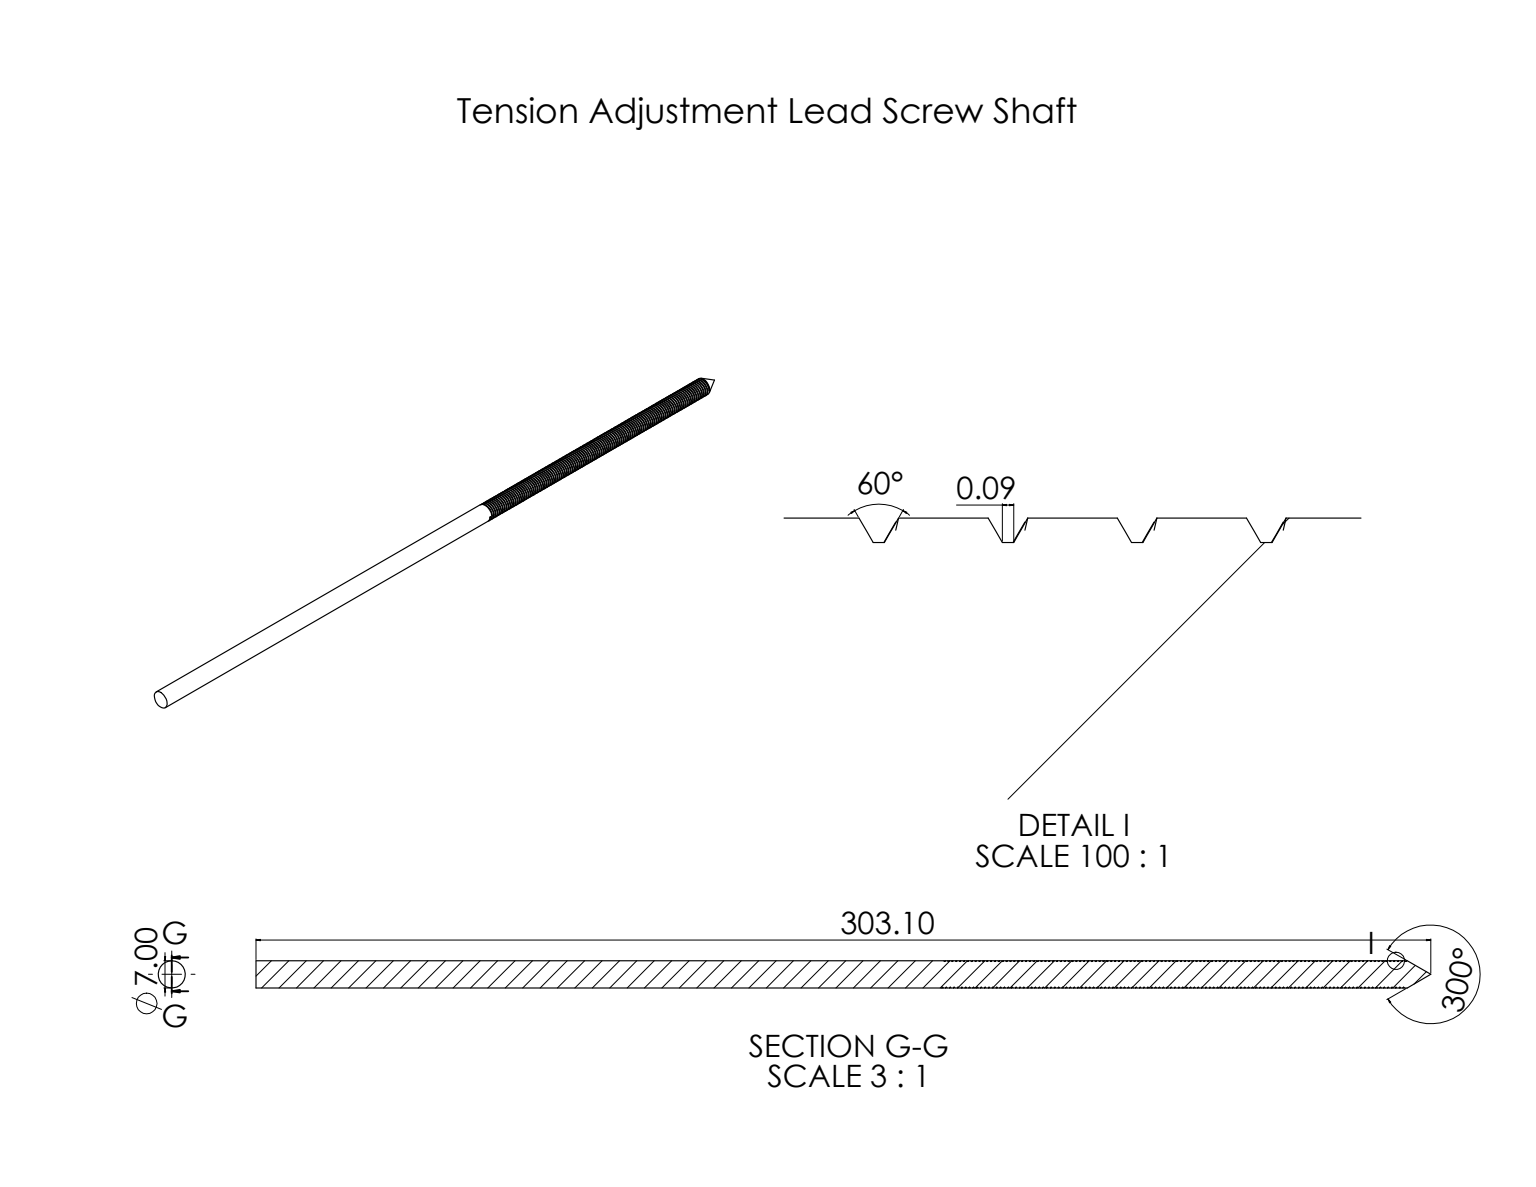
ISO-10303-21;
HEADER;
FILE_DESCRIPTION (('STEP AP214'),
    '1' );
FILE_NAME ('Tension Adjustment Lead Screw Shaft.step',
    '2026-10-25T21:42:00',
    ( '' ),
    ( '' ),
    'SwSTEP 2.0',
    'SolidWorks 2025',
    '' );
FILE_SCHEMA (( 'AUTOMOTIVE_DESIGN' ));
ENDSEC;

DATA;
#4=CARTESIAN_POINT ( 'NONE',  ( 1.655278471874998436, 14.63297358603754539, -90.43077246956613635 ) ) ;
#5=ORIENTED_EDGE ( 'NONE', *, *, #18600, .F. ) ;
#7=EDGE_LOOP ( 'NONE', ( #23173, #23553, #33553, #33564 ) ) ;
#9=CARTESIAN_POINT ( 'NONE',  ( -1.394453263437886604E-15, 14.00000000000001776, -84.40473080337743284 ) ) ;
#12=( BOUNDED_CURVE ( )  B_SPLINE_CURVE ( 2, ( #12979, #41701, #6799, #32739, #418, #13394, #26374, #31903, #3401 ),
 .UNSPECIFIED., .F., .F. ) 
 B_SPLINE_CURVE_WITH_KNOTS ( ( 3, 2, 2, 2, 3 ),
 ( 0.5229166666666666963, 0.5236111111111111382, 0.5250000000000000222, 0.5263888888888889062, 0.5270833333333333481 ),
 .UNSPECIFIED. ) 
 CURVE ( )  GEOMETRIC_REPRESENTATION_ITEM ( )  RATIONAL_B_SPLINE_CURVE ( ( 0.9330127018922194093, 0.9330127018922194093, 1.000000000000000000, 0.8660254037844387076, 1.000000000000000000, 0.8660254037844387076, 1.000000000000000000, 0.9330127018922194093, 0.9330127018922194093 ) ) 
 REPRESENTATION_ITEM ( '' )  );
#13=CARTESIAN_POINT ( 'NONE',  ( -0.9378221735089310451, 14.00000000000002309, -127.4493890021159359 ) ) ;
#14=CARTESIAN_POINT ( 'NONE',  ( 1.749999999999998224, 14.46891108675448656, -129.6276474690881741 ) ) ;
#15=CARTESIAN_POINT ( 'NONE',  ( -1.655278471874999990, 20.36702641396249902, -133.9307724695661364 ) ) ;
#17=CARTESIAN_POINT ( 'NONE',  ( 0.9378221735089302680, 14.00000000000002132, -139.3600726046389013 ) ) ;
#18=CARTESIAN_POINT ( 'NONE',  ( -3.310556943750002645, 15.58864905735837780, -117.7682724695661420 ) ) ;
#19=CARTESIAN_POINT ( 'NONE',  ( 3.310556943749999981, 15.58864905735836182, -51.43493913623279923 ) ) ;
#21=CARTESIAN_POINT ( 'NONE',  ( -3.500000000000000888, 19.52072594216371826, -128.7380641367107614 ) ) ;
#22=VECTOR ( 'NONE', #20923, 1000.000000000000000 ) ;
#23=CARTESIAN_POINT ( 'NONE',  ( 3.310556943750001313, 17.50000000000001421, -72.35160580289947063 ) ) ;
#24=CARTESIAN_POINT ( 'NONE',  ( 2.474675557024783212E-16, 21.54145188432740099, -122.2109808024215170 ) ) ;
#25=CARTESIAN_POINT ( 'NONE',  ( -1.655278471875002211, 14.63297358603754894, -108.5974391362328078 ) ) ;
#26=CARTESIAN_POINT ( 'NONE',  ( 1.750000000000001110, 20.53108891324555429, -92.98806413671076143 ) ) ;
#29=CARTESIAN_POINT ( 'NONE',  ( 3.500000000000001776, 19.52072594216371115, -75.37764746908818836 ) ) ;
#31=CARTESIAN_POINT ( 'NONE',  ( 3.310556943749999981, 15.58864905735836182, -44.34743913623280065 ) ) ;
#33=CARTESIAN_POINT ( 'NONE',  ( 1.655278471874998436, 14.63297358603754716, -97.51827246956612782 ) ) ;
#34=CARTESIAN_POINT ( 'NONE',  ( 0.9378221735089300459, 21.00000000000001421, -67.94938900211596433 ) ) ;
#35=CARTESIAN_POINT ( 'NONE',  ( 1.749999999999998224, 14.46891108675447768, -62.32139747004410424 ) ) ;
#38=CARTESIAN_POINT ( 'NONE',  ( 3.310556943750001313, 19.41135094264166838, -117.2682724695661278 ) ) ;
#44=CARTESIAN_POINT ( 'NONE',  ( 3.310556943750001313, 17.50000000000001776, -99.26410580289947916 ) ) ;
#45=CARTESIAN_POINT ( 'NONE',  ( 4.648177544792955347E-16, 21.00000000000001421, -63.21098080242150274 ) ) ;
#47=ORIENTED_EDGE ( 'NONE', *, *, #33783, .T. ) ;
#48=CARTESIAN_POINT ( 'NONE',  ( -7.460324959392693302E-14, 21.00000000000001776, -87.90473080337741862 ) ) ;
#49=CARTESIAN_POINT ( 'NONE',  ( -3.500000000000001332, 17.50000000000002132, -126.9609808024215170 ) ) ;
#50=DIRECTION ( 'NONE',  ( -0.000000000000000000, 1.259100132267607459E-16, -1.000000000000000000 ) ) ;
#53=CARTESIAN_POINT ( 'NONE',  ( 1.655278471875001101, 20.36702641396248481, -33.09743913623280775 ) ) ;
#54=CARTESIAN_POINT ( 'NONE',  ( -0.9378221735089310451, 14.00000000000002309, -109.4493890021159359 ) ) ;
#60=LINE ( 'NONE', #6452, #31415 ) ;
#61=( BOUNDED_CURVE ( )  B_SPLINE_CURVE ( 2, ( #20657, #17472, #30432, #1301, #10233, #7041, #1713, #24475, #37444 ),
 .UNSPECIFIED., .F., .T. ) 
 B_SPLINE_CURVE_WITH_KNOTS ( ( 3, 2, 2, 2, 3 ),
 ( 0.8270833333333332815, 0.8277777777777777235, 0.8291666666666667185, 0.8305555555555556024, 0.8312500000000000444 ),
 .UNSPECIFIED. ) 
 CURVE ( )  GEOMETRIC_REPRESENTATION_ITEM ( )  RATIONAL_B_SPLINE_CURVE ( ( 0.9330127018922194093, 0.9330127018922194093, 1.000000000000000000, 0.8660254037844387076, 1.000000000000000000, 0.8660254037844387076, 1.000000000000000000, 0.9330127018922194093, 0.9330127018922194093 ) ) 
 REPRESENTATION_ITEM ( '' )  );
#63=CARTESIAN_POINT ( 'NONE',  ( 4.648177544792955347E-16, 21.00000000000002132, -115.2109808024215027 ) ) ;
#64=CARTESIAN_POINT ( 'NONE',  ( 3.500000000000001332, 17.50000000000002487, -140.4609808024215170 ) ) ;
#65=CARTESIAN_POINT ( 'NONE',  ( -7.424026671074350129E-16, 13.45854811567263987, -118.4047308033774328 ) ) ;
#67=CARTESIAN_POINT ( 'NONE',  ( -1.655278471875002211, 14.63297358603755249, -134.6849391362327992 ) ) ;
#68=CARTESIAN_POINT ( 'NONE',  ( -3.500000000000000888, 19.52072594216370405, -34.04431413575484555 ) ) ;
#71=CARTESIAN_POINT ( 'NONE',  ( -1.394453263437886604E-15, 14.00000000000001421, -65.40473080337743284 ) ) ;
#73=CARTESIAN_POINT ( 'NONE',  ( -3.500000000000000888, 19.52072594216372181, -138.0443141357548598 ) ) ;
#74=CARTESIAN_POINT ( 'NONE',  ( 1.655278471874998436, 14.63297358603755072, -123.4307724695661506 ) ) ;
#77=CARTESIAN_POINT ( 'NONE',  ( -1.394453263437886604E-15, 14.00000000000001066, -46.40473080337741862 ) ) ;
#78=CARTESIAN_POINT ( 'NONE',  ( 1.749999999999998224, 14.46891108675448123, -92.62764746908815994 ) ) ;
#79=CARTESIAN_POINT ( 'NONE',  ( -3.500000000000001332, 17.50000000000001066, -45.65473080337742573 ) ) ;
#80=CARTESIAN_POINT ( 'NONE',  ( 3.310556943750001313, 17.50000000000001421, -58.26410580289947916 ) ) ;
#81=CARTESIAN_POINT ( 'NONE',  ( 1.655278471874998436, 14.63297358603754894, -119.5182724695661278 ) ) ;
#83=CARTESIAN_POINT ( 'NONE',  ( -3.500000000000002220, 15.47927405783632082, -30.57139747004410069 ) ) ;
#86=CARTESIAN_POINT ( 'NONE',  ( -7.022189441860112050E-16, 13.67729811471672896, -132.6016058028994564 ) ) ;
#90=CARTESIAN_POINT ( 'NONE',  ( -7.022189441860112050E-16, 13.67729811471672186, -70.60160580289947063 ) ) ;
#92=CARTESIAN_POINT ( 'NONE',  ( 3.310556943750001313, 17.50000000000001421, -65.26410580289946495 ) ) ;
#93=ORIENTED_EDGE ( 'NONE', *, *, #26909, .T. ) ;
#95=CARTESIAN_POINT ( 'NONE',  ( -1.655278471875002211, 14.63297358603754716, -83.68493913623278502 ) ) ;
#97=CARTESIAN_POINT ( 'NONE',  ( -1.394453263437886604E-15, 14.00000000000001066, -36.40473080337743284 ) ) ;
#99=CARTESIAN_POINT ( 'NONE',  ( -1.655278471874999990, 20.36702641396248836, -47.93077246956614346 ) ) ;
#100=EDGE_CURVE ( 'NONE', #30193, #39728, #5168, .T. ) ;
#102=CARTESIAN_POINT ( 'NONE',  ( 2.340729813953370519E-16, 21.32270188528331900, -105.0141058028994649 ) ) ;
#103=CARTESIAN_POINT ( 'NONE',  ( -3.500000000000000000, 19.52072594216370405, -36.04431413575484555 ) ) ;
#104=VERTEX_POINT ( 'NONE', #20780 ) ;
#109=CARTESIAN_POINT ( 'NONE',  ( 2.340729813953370519E-16, 21.32270188528330834, -56.01410580289947916 ) ) ;
#110=ORIENTED_EDGE ( 'NONE', *, *, #41716, .T. ) ;
#111=ORIENTED_EDGE ( 'NONE', *, *, #16123, .F. ) ;
#113=CARTESIAN_POINT ( 'NONE',  ( 4.648177544792955347E-16, 21.00000000000001421, -55.21098080242150274 ) ) ;
#116=CARTESIAN_POINT ( 'NONE',  ( -1.750000000000002220, 14.46891108675449011, -138.7943141357548313 ) ) ;
#117=CARTESIAN_POINT ( 'NONE',  ( -3.310556943750002201, 15.58864905735837780, -126.6807724695661364 ) ) ;
#118=EDGE_CURVE ( 'NONE', #7389, #10255, #33314, .T. ) ;
#120=VECTOR ( 'NONE', #13547, 1000.000000000000000 ) ;
#121=EDGE_CURVE ( 'NONE', #3869, #17551, #1003, .T. ) ;
#123=CARTESIAN_POINT ( 'NONE',  ( -3.310556943750002645, 15.58864905735836537, -33.76827246956613493 ) ) ;
#124=CARTESIAN_POINT ( 'NONE',  ( 1.655278471874998436, 14.63297358603753651, -25.51827246956613138 ) ) ;
#125=CARTESIAN_POINT ( 'NONE',  ( 3.310556943750001313, 19.41135094264166483, -85.26827246956612782 ) ) ;
#126=CARTESIAN_POINT ( 'NONE',  ( -3.310556943750000425, 19.41135094264167549, -139.8474391362327935 ) ) ;
#128=CARTESIAN_POINT ( 'NONE',  ( 3.405278471875001323, 17.50000000000001066, -23.20941830313845600 ) ) ;
#129=CARTESIAN_POINT ( 'NONE',  ( -1.394453263437886604E-15, 14.00000000000001421, -66.71098080242148853 ) ) ;
#130=CARTESIAN_POINT ( 'NONE',  ( -3.310556943750000425, 19.41135094264167549, -134.9349391362328277 ) ) ;
#131=CARTESIAN_POINT ( 'NONE',  ( 3.500000000000000000, 15.47927405783632437, -56.54431413575483845 ) ) ;
#132=CARTESIAN_POINT ( 'NONE',  ( 2.340729813953370519E-16, 21.32270188528331190, -94.01410580289947916 ) ) ;
#134=CARTESIAN_POINT ( 'NONE',  ( -0.9378221735089291577, 21.00000000000001776, -93.16632260368298546 ) ) ;
#135=CARTESIAN_POINT ( 'NONE',  ( 3.500000000000001776, 19.52072594216371115, -76.07139747004410424 ) ) ;
#136=AXIS2_PLACEMENT_3D ( 'NONE', #21819, #34790, #18632 ) ;
#137=CARTESIAN_POINT ( 'NONE',  ( -1.655278471874999990, 20.36702641396248836, -59.01827246956613493 ) ) ;
#141=AXIS2_PLACEMENT_3D ( 'NONE', #11011, #30148, #20585 ) ;
#142=CARTESIAN_POINT ( 'NONE',  ( 2.340729813953370519E-16, 21.32270188528331190, -84.10160580289945642 ) ) ;
#144=CARTESIAN_POINT ( 'NONE',  ( -1.655278471875002211, 14.63297358603755072, -115.5974391362327935 ) ) ;
#145=CARTESIAN_POINT ( 'NONE',  ( 2.340729813953370519E-16, 21.32270188528331190, -82.01410580289947916 ) ) ;
#146=CARTESIAN_POINT ( 'NONE',  ( -0.9378221735089291577, 21.00000000000001776, -96.86007260463890134 ) ) ;
#148=CARTESIAN_POINT ( 'NONE',  ( 2.340729813953370519E-16, 21.32270188528331190, -100.1016058028994706 ) ) ;
#149=CARTESIAN_POINT ( 'NONE',  ( -3.500000000000000888, 19.52072594216371826, -103.7380641367107614 ) ) ;
#152=CARTESIAN_POINT ( 'NONE',  ( 1.750000000000001110, 20.53108891324554719, -43.98806413671076143 ) ) ;
#153=CARTESIAN_POINT ( 'NONE',  ( 3.500000000000000000, 15.47927405783632082, -45.54431413575483845 ) ) ;
#155=CARTESIAN_POINT ( 'NONE',  ( 3.310556943750001313, 19.41135094264166483, -67.18077246956613635 ) ) ;
#156=ADVANCED_FACE ( 'NONE', ( #4604 ), #8574, .T. ) ;
#158=CARTESIAN_POINT ( 'NONE',  ( -3.310556943750000425, 19.41135094264166838, -119.8474391362328078 ) ) ;
#163=CARTESIAN_POINT ( 'NONE',  ( -3.500000000000001332, 17.50000000000001066, -42.96098080242151696 ) ) ;
#165=CARTESIAN_POINT ( 'NONE',  ( -7.022189441860112050E-16, 13.67729811471672186, -73.51410580289947916 ) ) ;
#166=EDGE_LOOP ( 'NONE', ( #29980, #17944, #31136, #21561 ) ) ;
#167=VERTEX_POINT ( 'NONE', #37923 ) ;
#173=CARTESIAN_POINT ( 'NONE',  ( -3.310556943750000425, 19.41135094264165772, -41.93493913623279212 ) ) ;
#174=CARTESIAN_POINT ( 'NONE',  ( 1.655278471875001101, 20.36702641396249547, -106.1849391362327992 ) ) ;
#176=ADVANCED_FACE ( 'NONE', ( #8782 ), #21755, .T. ) ;
#177=( BOUNDED_CURVE ( )  B_SPLINE_CURVE ( 2, ( #32647, #3511, #29666, #26491, #530, #13503, #39446, #10320, #20103 ),
 .UNSPECIFIED., .F., .T. ) 
 B_SPLINE_CURVE_WITH_KNOTS ( ( 3, 2, 2, 2, 3 ),
 ( 0.9312500000000000222, 0.9319444444444444642, 0.9333333333333333481, 0.9347222222222222321, 0.9354166666666666741 ),
 .UNSPECIFIED. ) 
 CURVE ( )  GEOMETRIC_REPRESENTATION_ITEM ( )  RATIONAL_B_SPLINE_CURVE ( ( 0.9330127018922194093, 0.9330127018922194093, 1.000000000000000000, 0.8660254037844387076, 1.000000000000000000, 0.8660254037844387076, 1.000000000000000000, 0.9330127018922194093, 0.9330127018922194093 ) ) 
 REPRESENTATION_ITEM ( '' )  );
#178=CARTESIAN_POINT ( 'NONE',  ( 1.655278471874998436, 14.63297358603753828, -27.43077246956614346 ) ) ;
#180=CARTESIAN_POINT ( 'NONE',  ( 1.750000000000001110, 20.53108891324555785, -104.2943141357548456 ) ) ;
#182=EDGE_CURVE ( 'NONE', #24979, #8593, #36724, .T. ) ;
#183=DIRECTION ( 'NONE',  ( -0.000000000000000000, 1.259100132267607459E-16, -1.000000000000000000 ) ) ;
#184=CARTESIAN_POINT ( 'NONE',  ( 3.500000000000001332, 17.50000000000001776, -91.15473080337743284 ) ) ;
#185=CARTESIAN_POINT ( 'NONE',  ( -3.500000000000001332, 17.50000000000001776, -77.96098080242150274 ) ) ;
#188=CARTESIAN_POINT ( 'NONE',  ( 1.749999999999998224, 14.46891108675447768, -59.62764746908817415 ) ) ;
#191=CARTESIAN_POINT ( 'NONE',  ( -3.500000000000000888, 19.52072594216370760, -46.73806413671076143 ) ) ;
#192=CARTESIAN_POINT ( 'NONE',  ( 1.655278471874998436, 14.63297358603753828, -29.51827246956613493 ) ) ;
#194=CARTESIAN_POINT ( 'NONE',  ( -1.394453263437886604E-15, 14.00000000000001421, -80.40473080337743284 ) ) ;
#197=DIRECTION ( 'NONE',  ( -0.000000000000000000, 1.259100132267607459E-16, -1.000000000000000000 ) ) ;
#199=CARTESIAN_POINT ( 'NONE',  ( -1.655278471874999990, 20.36702641396249192, -82.93077246956615056 ) ) ;
#201=CARTESIAN_POINT ( 'NONE',  ( 4.648177544792955347E-16, 21.00000000000001421, -52.21098080242150985 ) ) ;
#203=CARTESIAN_POINT ( 'NONE',  ( 0.9378221735089300459, 21.00000000000001066, -33.94938900211595012 ) ) ;
#205=CARTESIAN_POINT ( 'NONE',  ( 3.500000000000000000, 15.47927405783632793, -87.54431413575483134 ) ) ;
#208=CARTESIAN_POINT ( 'NONE',  ( 2.340729813953370519E-16, 21.32270188528331190, -89.01410580289947916 ) ) ;
#210=ORIENTED_EDGE ( 'NONE', *, *, #4786, .F. ) ;
#215=FACE_OUTER_BOUND ( 'NONE', #16259, .T. ) ;
#216=CARTESIAN_POINT ( 'NONE',  ( 1.655278471875001101, 20.36702641396249902, -134.0974391362328220 ) ) ;
#217=VERTEX_POINT ( 'NONE', #6222 ) ;
#218=AXIS2_PLACEMENT_3D ( 'NONE', #34519, #2189, #33537 ) ;
#220=VECTOR ( 'NONE', #24131, 1000.000000000000000 ) ;
#222=CARTESIAN_POINT ( 'NONE',  ( -1.655278471875002211, 14.63297358603755072, -118.6849391362327992 ) ) ;
#226=CARTESIAN_POINT ( 'NONE',  ( -3.500000000000002220, 15.47927405783633503, -129.5713974700440758 ) ) ;
#227=CARTESIAN_POINT ( 'NONE',  ( -7.022189441860112050E-16, 13.67729811471672186, -73.60160580289945642 ) ) ;
#228=CARTESIAN_POINT ( 'NONE',  ( -7.424026671074350129E-16, 13.45854811567263987, -120.7109808024215170 ) ) ;
#230=CARTESIAN_POINT ( 'NONE',  ( -7.022189441860112050E-16, 13.67729811471672541, -103.5141058028994649 ) ) ;
#232=CARTESIAN_POINT ( 'NONE',  ( -1.394453263437886604E-15, 14.00000000000001066, -31.71098080242150985 ) ) ;
#234=CARTESIAN_POINT ( 'NONE',  ( 3.500000000000000000, 15.47927405783632437, -75.54431413575484555 ) ) ;
#236=CARTESIAN_POINT ( 'NONE',  ( -7.022189441860112050E-16, 13.67729811471671475, -37.51410580289947205 ) ) ;
#237=CARTESIAN_POINT ( 'NONE',  ( 1.655278471874998436, 14.63297358603754716, -95.51827246956612782 ) ) ;
#238=CARTESIAN_POINT ( 'NONE',  ( -3.500000000000001332, 17.50000000000001421, -66.65473080337743284 ) ) ;
#240=CARTESIAN_POINT ( 'NONE',  ( -1.655278471875002211, 14.63297358603755072, -117.6849391362327850 ) ) ;
#247=CARTESIAN_POINT ( 'NONE',  ( -3.310556943750002201, 15.58864905735837425, -96.68077246956613635 ) ) ;
#250=ORIENTED_EDGE ( 'NONE', *, *, #32801, .F. ) ;
#252=CYLINDRICAL_SURFACE ( 'NONE', #19666, 3.499999999999999556 ) ;
#254=CARTESIAN_POINT ( 'NONE',  ( 4.648177544792955347E-16, 21.00000000000002132, -105.9047308033774186 ) ) ;
#259=CARTESIAN_POINT ( 'NONE',  ( -7.022189441860112050E-16, 13.67729811471671653, -26.51410580289948626 ) ) ;
#260=( BOUNDED_CURVE ( )  B_SPLINE_CURVE ( 2, ( #24634, #5264, #21631, #34609, #15269, #28228, #15689, #5055, #28645 ),
 .UNSPECIFIED., .F., .F. ) 
 B_SPLINE_CURVE_WITH_KNOTS ( ( 3, 2, 2, 2, 3 ),
 ( 0.05625000000000000139, 0.05694444444444444337, 0.05833333333333333426, 0.05972222222222222515, 0.06041666666666666713 ),
 .UNSPECIFIED. ) 
 CURVE ( )  GEOMETRIC_REPRESENTATION_ITEM ( )  RATIONAL_B_SPLINE_CURVE ( ( 0.9330127018922192983, 0.9330127018922196314, 1.000000000000000000, 0.8660254037844387076, 1.000000000000000000, 0.8660254037844387076, 1.000000000000000000, 0.9330127018922194093, 0.9330127018922194093 ) ) 
 REPRESENTATION_ITEM ( '' )  );
#263=VECTOR ( 'NONE', #2709, 1000.000000000000000 ) ;
#266=CARTESIAN_POINT ( 'NONE',  ( 4.648177544792955347E-16, 21.00000000000001421, -57.90473080337742573 ) ) ;
#267=ORIENTED_EDGE ( 'NONE', *, *, #5048, .F. ) ;
#270=CARTESIAN_POINT ( 'NONE',  ( -1.394453263437886604E-15, 14.00000000000001066, -31.40473080337742573 ) ) ;
#271=CARTESIAN_POINT ( 'NONE',  ( -3.500000000000002220, 15.47927405783633503, -118.5713974700441184 ) ) ;
#272=DIRECTION ( 'NONE',  ( 0.000000000000000000, 1.000000000000000000, 0.000000000000000000 ) ) ;
#273=CARTESIAN_POINT ( 'NONE',  ( 3.310556943750001313, 19.41135094264167549, -134.2682724695661420 ) ) ;
#274=CARTESIAN_POINT ( 'NONE',  ( -3.500000000000001332, 17.50000000000001066, -26.96098080242151340 ) ) ;
#276=DIRECTION ( 'NONE',  ( -0.000000000000000000, 1.259100132267607459E-16, -1.000000000000000000 ) ) ;
#278=CARTESIAN_POINT ( 'NONE',  ( -2.324088772396477673E-16, 14.00000000000002309, -142.7109808024215170 ) ) ;
#280=CARTESIAN_POINT ( 'NONE',  ( 3.500000000000001776, 19.52072594216372181, -140.3776474690881741 ) ) ;
#281=CARTESIAN_POINT ( 'NONE',  ( -1.655278471874999990, 20.36702641396249547, -117.9307724695661364 ) ) ;
#283=ORIENTED_EDGE ( 'NONE', *, *, #17861, .F. ) ;
#285=DIRECTION ( 'NONE',  ( -0.000000000000000000, 1.259100132267607459E-16, -1.000000000000000000 ) ) ;
#286=CARTESIAN_POINT ( 'NONE',  ( 1.750000000000001110, 20.53108891324555429, -91.29431413575484555 ) ) ;
#287=CARTESIAN_POINT ( 'NONE',  ( -0.9378221735089291577, 21.00000000000001066, -41.16632260368299256 ) ) ;
#288=CARTESIAN_POINT ( 'NONE',  ( -3.310556943750002645, 15.58864905735836714, -53.68077246956612925 ) ) ;
#289=CARTESIAN_POINT ( 'NONE',  ( -3.310556943750000425, 19.41135094264166838, -112.9349391362327992 ) ) ;
#290=DIRECTION ( 'NONE',  ( 0.000000000000000000, 1.000000000000000000, 0.000000000000000000 ) ) ;
#291=CARTESIAN_POINT ( 'NONE',  ( 3.500000000000000000, 15.47927405783632082, -32.23806413671076143 ) ) ;
#293=VECTOR ( 'NONE', #35770, 1000.000000000000000 ) ;
#295=CARTESIAN_POINT ( 'NONE',  ( 1.655278471874998436, 14.63297358603755249, -136.5182724695661420 ) ) ;
#296=EDGE_CURVE ( 'NONE', #3050, #12825, #3300, .T. ) ;
#300=CARTESIAN_POINT ( 'NONE',  ( 3.310556943750001313, 17.50000000000001421, -62.35160580289945642 ) ) ;
#302=CARTESIAN_POINT ( 'NONE',  ( 1.655278471875001101, 20.36702641396248836, -63.09743913623280775 ) ) ;
#304=CARTESIAN_POINT ( 'NONE',  ( 2.340729813953370519E-16, 21.32270188528331190, -88.10160580289947063 ) ) ;
#306=CARTESIAN_POINT ( 'NONE',  ( -3.500000000000001332, 17.50000000000002132, -103.6547308033774186 ) ) ;
#308=CARTESIAN_POINT ( 'NONE',  ( -1.655278471874999990, 20.36702641396248481, -43.93077246956614346 ) ) ;
#310=CARTESIAN_POINT ( 'NONE',  ( -3.310556943750000425, 19.41135094264166838, -107.8474391362328078 ) ) ;
#312=( BOUNDED_CURVE ( )  B_SPLINE_CURVE ( 2, ( #31832, #41215, #38439, #18665, #34822, #5896, #28021, #41000, #2494 ),
 .UNSPECIFIED., .F., .F. ) 
 B_SPLINE_CURVE_WITH_KNOTS ( ( 3, 2, 2, 2, 3 ),
 ( 0.3979166666666666963, 0.3986111111111111382, 0.4000000000000000222, 0.4013888888888889062, 0.4020833333333333481 ),
 .UNSPECIFIED. ) 
 CURVE ( )  GEOMETRIC_REPRESENTATION_ITEM ( )  RATIONAL_B_SPLINE_CURVE ( ( 0.9330127018922194093, 0.9330127018922220739, 1.000000000000000000, 0.8660254037844387076, 1.000000000000000000, 0.8660254037844387076, 1.000000000000000000, 0.9330127018922194093, 0.9330127018922194093 ) ) 
 REPRESENTATION_ITEM ( '' )  );
#319=CARTESIAN_POINT ( 'NONE',  ( -3.310556943750002645, 15.58864905735836892, -56.68077246956614346 ) ) ;
#320=ORIENTED_EDGE ( 'NONE', *, *, #14049, .F. ) ;
#322=CARTESIAN_POINT ( 'NONE',  ( 3.500000000000001332, 19.52072594216371115, -76.37764746908817415 ) ) ;
#323=AXIS2_PLACEMENT_3D ( 'NONE', #18071, #37633, #1287 ) ;
#324=CARTESIAN_POINT ( 'NONE',  ( -0.9378221735089291577, 21.00000000000001066, -40.86007260463890844 ) ) ;
#329=CARTESIAN_POINT ( 'NONE',  ( -4.648177544792955347E-16, 21.00000000000002487, -143.2109808024214885 ) ) ;
#330=CARTESIAN_POINT ( 'NONE',  ( -7.022189441860112050E-16, 13.67729811471672896, -127.5141058028994507 ) ) ;
#333=CARTESIAN_POINT ( 'NONE',  ( 3.310556943750001313, 17.50000000000001066, -33.35160580289946353 ) ) ;
#334=CARTESIAN_POINT ( 'NONE',  ( -7.022189441860112050E-16, 13.67729811471671297, -23.60160580289946353 ) ) ;
#335=CARTESIAN_POINT ( 'NONE',  ( -3.310556943750001313, 17.50000000000001776, -86.85160580289947063 ) ) ;
#336=CARTESIAN_POINT ( 'NONE',  ( 3.310556943749999981, 15.58864905735837780, -139.3474391362327935 ) ) ;
#339=CARTESIAN_POINT ( 'NONE',  ( 3.500000000000000000, 15.47927405783632082, -49.23806413671077564 ) ) ;
#340=CARTESIAN_POINT ( 'NONE',  ( 3.500000000000001332, 19.52072594216371826, -114.0713974700440900 ) ) ;
#342=CARTESIAN_POINT ( 'NONE',  ( 2.340729813953370519E-16, 21.32270188528331900, -129.1016058028994848 ) ) ;
#344=CARTESIAN_POINT ( 'NONE',  ( -1.394453263437886604E-15, 14.00000000000001776, -107.4047308033774328 ) ) ;
#345=CARTESIAN_POINT ( 'NONE',  ( 3.310556943749999981, 15.58864905735836892, -93.34743913623279354 ) ) ;
#346=CARTESIAN_POINT ( 'NONE',  ( -1.394453263437886604E-15, 14.00000000000000711, -24.71098080242150985 ) ) ;
#347=CARTESIAN_POINT ( 'NONE',  ( 4.648177544792955347E-16, 21.00000000000002132, -126.2109808024214885 ) ) ;
#349=CARTESIAN_POINT ( 'NONE',  ( -3.500000000000000888, 19.52072594216371115, -75.73806413671076143 ) ) ;
#350=CARTESIAN_POINT ( 'NONE',  ( -1.655278471875002211, 14.63297358603754361, -57.68493913623279212 ) ) ;
#352=CARTESIAN_POINT ( 'NONE',  ( 3.602337597214540226E-14, 14.00000000000002132, -117.4047308033774328 ) ) ;
#354=CARTESIAN_POINT ( 'NONE',  ( 1.655278471875001101, 20.36702641396249192, -86.18493913623278502 ) ) ;
#357=CARTESIAN_POINT ( 'NONE',  ( 1.655278471874998436, 14.63297358603754894, -111.4307724695661506 ) ) ;
#358=CARTESIAN_POINT ( 'NONE',  ( 3.310556943750001313, 19.41135094264166483, -80.18077246956613635 ) ) ;
#359=CARTESIAN_POINT ( 'NONE',  ( 0.9378221735089324884, 14.00000000000002665, -138.6663226036829997 ) ) ;
#362=CARTESIAN_POINT ( 'NONE',  ( -3.310556943750001313, 17.50000000000002132, -102.8516058028994564 ) ) ;
#363=CARTESIAN_POINT ( 'NONE',  ( -1.750000000000002220, 14.46891108675448478, -104.4880641367107614 ) ) ;
#366=CARTESIAN_POINT ( 'NONE',  ( -3.500000000000001332, 17.50000000000001776, -94.65473080337743284 ) ) ;
#367=CARTESIAN_POINT ( 'NONE',  ( 0.9378221735089300459, 21.00000000000001421, -53.94938900211595723 ) ) ;
#369=CARTESIAN_POINT ( 'NONE',  ( -1.655278471875002211, 14.63297358603754361, -60.59743913623280775 ) ) ;
#370=CARTESIAN_POINT ( 'NONE',  ( -1.394453263437886604E-15, 14.00000000000001066, -29.71098080242150985 ) ) ;
#371=ADVANCED_FACE ( 'NONE', ( #38132 ), #12394, .T. ) ;
#372=CARTESIAN_POINT ( 'NONE',  ( 3.310556943749999981, 15.58864905735837247, -120.3474391362328078 ) ) ;
#376=ORIENTED_EDGE ( 'NONE', *, *, #10155, .F. ) ;
#379=CARTESIAN_POINT ( 'NONE',  ( 1.750000000000001110, 20.53108891324555429, -78.98806413671076143 ) ) ;
#380=CARTESIAN_POINT ( 'NONE',  ( -1.655278471874999990, 20.36702641396248836, -72.93077246956613635 ) ) ;
#382=ORIENTED_EDGE ( 'NONE', *, *, #1692, .T. ) ;
#385=CARTESIAN_POINT ( 'NONE',  ( 4.286263797015737581E-16, 14.00000000000002487, -149.5231586289125687 ) ) ;
#386=EDGE_CURVE ( 'NONE', #5825, #2381, #41067, .T. ) ;
#388=CARTESIAN_POINT ( 'NONE',  ( 1.655278471875001101, 20.36702641396248481, -36.18493913623279923 ) ) ;
#389=CARTESIAN_POINT ( 'NONE',  ( -3.310556943750001313, 17.50000000000002132, -104.8516058028994564 ) ) ;
#391=EDGE_CURVE ( 'NONE', #32893, #8219, #9416, .T. ) ;
#392=CARTESIAN_POINT ( 'NONE',  ( -3.310556943750002645, 15.58864905735836537, -26.68077246956614346 ) ) ;
#393=CARTESIAN_POINT ( 'NONE',  ( 3.500000000000001332, 19.52072594216370760, -69.07139747004409003 ) ) ;
#394=CARTESIAN_POINT ( 'NONE',  ( 3.500000000000001776, 19.52072594216371826, -103.3776474690881599 ) ) ;
#396=CARTESIAN_POINT ( 'NONE',  ( 3.500000000000001332, 19.52072594216371826, -142.0713974700441042 ) ) ;
#397=CARTESIAN_POINT ( 'NONE',  ( -1.749999999999999778, 20.53108891324555429, -91.82139747004409003 ) ) ;
#402=CARTESIAN_POINT ( 'NONE',  ( -7.424026671074350129E-16, 13.45854811567263454, -54.71098080242152406 ) ) ;
#403=CARTESIAN_POINT ( 'NONE',  ( -1.749999999999999778, 20.53108891324554719, -30.82139747004410069 ) ) ;
#405=CARTESIAN_POINT ( 'NONE',  ( 2.474675557024783212E-16, 21.54145188432739033, -40.90473080337743284 ) ) ;
#407=CARTESIAN_POINT ( 'NONE',  ( -7.022189441860112050E-16, 13.67729811471671297, -25.60160580289946708 ) ) ;
#409=CARTESIAN_POINT ( 'NONE',  ( 4.648177544792955347E-16, 21.00000000000001066, -39.90473080337742573 ) ) ;
#410=CARTESIAN_POINT ( 'NONE',  ( -1.749999999999999778, 20.53108891324555074, -60.82139747004409713 ) ) ;
#412=CARTESIAN_POINT ( 'NONE',  ( -1.394453263437886604E-15, 14.00000000000001066, -33.40473080337742573 ) ) ;
#414=CARTESIAN_POINT ( 'NONE',  ( -1.655278471874999990, 20.36702641396249192, -81.93077246956615056 ) ) ;
#415=CARTESIAN_POINT ( 'NONE',  ( -1.750000000000002220, 14.46891108675449011, -141.4880641367107614 ) ) ;
#416=ORIENTED_EDGE ( 'NONE', *, *, #18320, .T. ) ;
#417=CARTESIAN_POINT ( 'NONE',  ( -1.750000000000002220, 14.46891108675447590, -35.48806413671076854 ) ) ;
#418=CARTESIAN_POINT ( 'NONE',  ( 3.500000000000001332, 17.50000000000001776, -80.46098080242150274 ) ) ;
#419=ORIENTED_EDGE ( 'NONE', *, *, #18485, .F. ) ;
#421=CARTESIAN_POINT ( 'NONE',  ( -3.310556943750000425, 19.41135094264166483, -89.84743913623280775 ) ) ;
#425=EDGE_CURVE ( 'NONE', #32425, #22611, #3648, .T. ) ;
#427=CARTESIAN_POINT ( 'NONE',  ( -1.394453263437886604E-15, 14.00000000000002132, -119.7109808024215170 ) ) ;
#428=( BOUNDED_CURVE ( )  B_SPLINE_CURVE ( 2, ( #7324, #1579, #20294, #4125, #14128, #14557, #1160, #17532, #11354 ),
 .UNSPECIFIED., .F., .F. ) 
 B_SPLINE_CURVE_WITH_KNOTS ( ( 3, 2, 2, 2, 3 ),
 ( 0.9729166666666666519, 0.9736111111111110938, 0.9749999999999999778, 0.9763888888888888618, 0.9770833333333333037 ),
 .UNSPECIFIED. ) 
 CURVE ( )  GEOMETRIC_REPRESENTATION_ITEM ( )  RATIONAL_B_SPLINE_CURVE ( ( 0.9330127018922194093, 0.9330127018922194093, 1.000000000000000000, 0.8660254037844387076, 1.000000000000000000, 0.8660254037844387076, 1.000000000000000000, 0.9330127018922194093, 0.9330127018922194093 ) ) 
 REPRESENTATION_ITEM ( '' )  );
#430=CARTESIAN_POINT ( 'NONE',  ( 3.310556943749999981, 15.58864905735837425, -127.3474391362328078 ) ) ;
#431=ORIENTED_EDGE ( 'NONE', *, *, #32696, .T. ) ;
#433=CARTESIAN_POINT ( 'NONE',  ( 1.655278471874998436, 14.63297358603754006, -52.51827246956612782 ) ) ;
#434=CARTESIAN_POINT ( 'NONE',  ( -1.655278471875002211, 14.63297358603755072, -121.6849391362327992 ) ) ;
#436=EDGE_CURVE ( 'NONE', #19172, #39176, #31243, .T. ) ;
#438=CARTESIAN_POINT ( 'NONE',  ( -3.500000000000000888, 19.52072594216372181, -131.7380641367107614 ) ) ;
#440=CARTESIAN_POINT ( 'NONE',  ( -3.310556943750000425, 19.41135094264166128, -72.93493913623278502 ) ) ;
#441=CARTESIAN_POINT ( 'NONE',  ( 2.474675557024783212E-16, 21.54145188432740099, -120.2109808024215027 ) ) ;
#442=CARTESIAN_POINT ( 'NONE',  ( -3.310556943750001313, 17.50000000000001776, -100.7641058028994792 ) ) ;
#444=CARTESIAN_POINT ( 'NONE',  ( 4.648177544792955347E-16, 21.00000000000002132, -105.2109808024215027 ) ) ;
#446=CARTESIAN_POINT ( 'NONE',  ( 1.750000000000001110, 20.53108891324555074, -69.29431413575484555 ) ) ;
#447=CARTESIAN_POINT ( 'NONE',  ( -3.500000000000002220, 15.47927405783632437, -50.87764746908815994 ) ) ;
#448=CARTESIAN_POINT ( 'NONE',  ( 3.310556943749999981, 15.58864905735836182, -39.34743913623282197 ) ) ;
#449=CARTESIAN_POINT ( 'NONE',  ( -7.022189441860112050E-16, 13.67729811471672541, -97.60160580289945642 ) ) ;
#450=CARTESIAN_POINT ( 'NONE',  ( -1.750000000000002220, 14.46891108675447946, -59.48806413671076143 ) ) ;
#452=CARTESIAN_POINT ( 'NONE',  ( 1.655278471875001101, 20.36702641396249547, -117.1849391362327850 ) ) ;
#454=CARTESIAN_POINT ( 'NONE',  ( 4.648177544792955347E-16, 21.00000000000001421, -61.21098080242150985 ) ) ;
#459=CARTESIAN_POINT ( 'NONE',  ( -1.655278471874999990, 20.36702641396249192, -96.93077246956613635 ) ) ;
#462=ORIENTED_EDGE ( 'NONE', *, *, #14219, .F. ) ;
#465=CARTESIAN_POINT ( 'NONE',  ( -0.9378221735089291577, 21.00000000000002132, -105.8600726046389013 ) ) ;
#466=VERTEX_POINT ( 'NONE', #16637 ) ;
#467=CARTESIAN_POINT ( 'NONE',  ( -1.749999999999999778, 20.53108891324556140, -135.1276474690881741 ) ) ;
#470=CARTESIAN_POINT ( 'NONE',  ( 1.655278471874998436, 14.63297358603753828, -31.43077246956614701 ) ) ;
#473=CARTESIAN_POINT ( 'NONE',  ( 0.000000000000000000, 17.50000000000002487, -149.5231586289125687 ) ) ;
#474=EDGE_CURVE ( 'NONE', #2381, #29038, #9270, .T. ) ;
#476=EDGE_CURVE ( 'NONE', #21056, #39932, #33207, .T. ) ;
#483=CARTESIAN_POINT ( 'NONE',  ( 1.750000000000001110, 20.53108891324555785, -119.9880641367107614 ) ) ;
#484=EDGE_CURVE ( 'NONE', #5180, #32296, #28511, .T. ) ;
#485=CARTESIAN_POINT ( 'NONE',  ( 0.000000000000000000, 17.50000000000002487, -149.5231586289125687 ) ) ;
#486=CARTESIAN_POINT ( 'NONE',  ( 3.310556943750001313, 19.41135094264167549, -136.2682724695661136 ) ) ;
#487=CARTESIAN_POINT ( 'NONE',  ( 3.500000000000000000, 15.47927405783631727, -25.54431413575483489 ) ) ;
#490=CARTESIAN_POINT ( 'NONE',  ( 1.750000000000001110, 20.53108891324555785, -105.9880641367107614 ) ) ;
#492=CARTESIAN_POINT ( 'NONE',  ( -3.500000000000002220, 15.47927405783633503, -131.8776474690881741 ) ) ;
#493=CARTESIAN_POINT ( 'NONE',  ( -1.655278471875002211, 14.63297358603755072, -117.5974391362328078 ) ) ;
#497=CARTESIAN_POINT ( 'NONE',  ( -7.424026671074350129E-16, 13.45854811567263631, -88.71098080242150274 ) ) ;
#498=CARTESIAN_POINT ( 'NONE',  ( 4.648177544792955347E-16, 21.00000000000001066, -32.90473080337742573 ) ) ;
#499=CARTESIAN_POINT ( 'NONE',  ( -3.310556943750000425, 19.41135094264166128, -50.84743913623280775 ) ) ;
#500=CARTESIAN_POINT ( 'NONE',  ( -7.022189441860112050E-16, 13.67729811471672718, -113.6016058028994564 ) ) ;
#502=CARTESIAN_POINT ( 'NONE',  ( -3.500000000000002220, 15.47927405783632082, -29.57139747004410069 ) ) ;
#504=CARTESIAN_POINT ( 'NONE',  ( -3.310556943750000425, 19.41135094264167549, -134.9349391362327992 ) ) ;
#508=CARTESIAN_POINT ( 'NONE',  ( 3.310556943749999981, 15.58864905735836537, -64.43493913623279923 ) ) ;
#510=CARTESIAN_POINT ( 'NONE',  ( 3.310556943750001313, 17.50000000000001421, -64.26410580289946495 ) ) ;
#511=ORIENTED_EDGE ( 'NONE', *, *, #12682, .F. ) ;
#512=CARTESIAN_POINT ( 'NONE',  ( -1.655278471874999990, 20.36702641396249192, -87.01827246956612782 ) ) ;
#517=CARTESIAN_POINT ( 'NONE',  ( 3.310556943749999981, 15.58864905735836182, -44.34743913623280065 ) ) ;
#519=CARTESIAN_POINT ( 'NONE',  ( 3.310556943749999981, 15.58864905735837070, -98.34743913623282197 ) ) ;
#520=CARTESIAN_POINT ( 'NONE',  ( -1.394453263437886604E-15, 14.00000000000001421, -74.71098080242151696 ) ) ;
#521=ORIENTED_EDGE ( 'NONE', *, *, #20165, .F. ) ;
#524=VERTEX_POINT ( 'NONE', #29379 ) ;
#526=CARTESIAN_POINT ( 'NONE',  ( -7.022189441860112050E-16, 13.67729811471671830, -55.51410580289947916 ) ) ;
#527=ORIENTED_EDGE ( 'NONE', *, *, #27991, .F. ) ;
#529=CARTESIAN_POINT ( 'NONE',  ( -1.394453263437886604E-15, 14.00000000000002132, -111.7109808024214885 ) ) ;
#530=CARTESIAN_POINT ( 'NONE',  ( 3.500000000000001332, 17.50000000000001066, -31.46098080242150274 ) ) ;
#533=CARTESIAN_POINT ( 'NONE',  ( 3.500000000000001332, 19.52072594216370760, -47.07139747004410424 ) ) ;
#537=CARTESIAN_POINT ( 'NONE',  ( -3.500000000000002220, 15.47927405783632260, -45.87764746908817415 ) ) ;
#538=CARTESIAN_POINT ( 'NONE',  ( 1.655278471875001101, 20.36702641396248481, -44.09743913623280775 ) ) ;
#539=CARTESIAN_POINT ( 'NONE',  ( 1.750000000000001110, 20.53108891324554719, -34.98806413671076854 ) ) ;
#540=CARTESIAN_POINT ( 'NONE',  ( 1.749999999999998224, 14.46891108675447235, -23.62764746908817415 ) ) ;
#542=CARTESIAN_POINT ( 'NONE',  ( 3.500000000000001332, 17.50000000000002487, -143.3078558028994394 ) ) ;
#544=CARTESIAN_POINT ( 'NONE',  ( -3.310556943750001313, 17.50000000000001066, -30.85160580289945997 ) ) ;
#545=CARTESIAN_POINT ( 'NONE',  ( -3.500000000000001332, 17.50000000000001776, -97.65473080337743284 ) ) ;
#546=CARTESIAN_POINT ( 'NONE',  ( 3.310556943749999981, 15.58864905735836892, -82.43493913623278502 ) ) ;
#547=CARTESIAN_POINT ( 'NONE',  ( 1.655278471874998436, 14.63297358603755249, -136.4307724695661364 ) ) ;
#550=CARTESIAN_POINT ( 'NONE',  ( -0.9378221735089310451, 14.00000000000001066, -34.44938900211595012 ) ) ;
#552=CARTESIAN_POINT ( 'NONE',  ( 3.310556943749999981, 15.58864905735837425, -129.4349391362327992 ) ) ;
#554=CARTESIAN_POINT ( 'NONE',  ( -3.310556943750002645, 15.58864905735837247, -92.68077246956613635 ) ) ;
#555=CARTESIAN_POINT ( 'NONE',  ( 4.648177544792955347E-16, 21.00000000000002132, -108.2109808024215170 ) ) ;
#557=CARTESIAN_POINT ( 'NONE',  ( 0.9378221735089281585, 14.00000000000002309, -126.6663226036829570 ) ) ;
#558=CARTESIAN_POINT ( 'NONE',  ( 1.750000000000001110, 20.53108891324555429, -74.98806413671076143 ) ) ;
#559=CARTESIAN_POINT ( 'NONE',  ( -1.655278471875002211, 14.63297358603754361, -60.68493913623279923 ) ) ;
#561=LINE ( 'NONE', #23108, #27221 ) ;
#562=CARTESIAN_POINT ( 'NONE',  ( 0.000000000000000000, 21.00000000000002487, -149.5231586289125687 ) ) ;
#563=CARTESIAN_POINT ( 'NONE',  ( -3.310556943750000425, 19.41135094264166483, -81.93493913623278502 ) ) ;
#566=CARTESIAN_POINT ( 'NONE',  ( 2.340729813953370519E-16, 21.32270188528331900, -107.0141058028994649 ) ) ;
#567=CARTESIAN_POINT ( 'NONE',  ( 1.655278471874998436, 14.63297358603754539, -82.43077246956615056 ) ) ;
#568=CARTESIAN_POINT ( 'NONE',  ( 0.9378221735089260491, 21.00000000000002842, -138.2556390011600058 ) ) ;
#570=CARTESIAN_POINT ( 'NONE',  ( -3.310556943750002201, 15.58864905735837425, -99.76827246956612782 ) ) ;
#571=CARTESIAN_POINT ( 'NONE',  ( -3.500000000000002220, 15.47927405783632970, -105.5713974700441042 ) ) ;
#574=CARTESIAN_POINT ( 'NONE',  ( 4.648177544792955347E-16, 21.00000000000001776, -95.90473080337744705 ) ) ;
#576=CARTESIAN_POINT ( 'NONE',  ( 3.310556943750001313, 17.50000000000001421, -62.26410580289947205 ) ) ;
#578=CARTESIAN_POINT ( 'NONE',  ( -3.310556943750002645, 15.58864905735837780, -120.6807724695661506 ) ) ;
#580=VECTOR ( 'NONE', #16145, 1000.000000000000000 ) ;
#582=ORIENTED_EDGE ( 'NONE', *, *, #38583, .T. ) ;
#583=EDGE_LOOP ( 'NONE', ( #13938, #30673, #809, #28014 ) ) ;
#586=CARTESIAN_POINT ( 'NONE',  ( 3.500000000000000000, 15.47927405783633503, -128.2380641367107614 ) ) ;
#587=CARTESIAN_POINT ( 'NONE',  ( 3.310556943750001313, 17.50000000000001421, -73.26410580289947916 ) ) ;
#588=ORIENTED_EDGE ( 'NONE', *, *, #38855, .T. ) ;
#589=ORIENTED_EDGE ( 'NONE', *, *, #296, .F. ) ;
#593=CARTESIAN_POINT ( 'NONE',  ( -1.655278471875002211, 14.63297358603755249, -133.5974391362328220 ) ) ;
#595=CARTESIAN_POINT ( 'NONE',  ( -3.500000000000001332, 17.50000000000002132, -110.9609808024215027 ) ) ;
#596=CARTESIAN_POINT ( 'NONE',  ( -1.655278471875002211, 14.63297358603754006, -35.68493913623279923 ) ) ;
#597=CARTESIAN_POINT ( 'NONE',  ( -3.310556943750001313, 17.50000000000001776, -100.8516058028994706 ) ) ;
#600=CARTESIAN_POINT ( 'NONE',  ( -7.022189441860112050E-16, 13.67729811471671297, -24.51410580289947561 ) ) ;
#602=CARTESIAN_POINT ( 'NONE',  ( 3.500000000000000000, 15.47927405783632793, -99.54431413575485976 ) ) ;
#605=CARTESIAN_POINT ( 'NONE',  ( -1.749999999999999778, 20.53108891324555429, -93.82139747004409003 ) ) ;
#609=CARTESIAN_POINT ( 'NONE',  ( 3.500000000000001776, 19.52072594216370760, -56.37764746908817415 ) ) ;
#611=CARTESIAN_POINT ( 'NONE',  ( -1.836030130193217234E-14, 21.00000000000002487, -134.9047308033774186 ) ) ;
#612=CARTESIAN_POINT ( 'NONE',  ( -3.500000000000002220, 15.47927405783632260, -44.57139747004409713 ) ) ;
#613=CARTESIAN_POINT ( 'NONE',  ( 0.9378221735089300459, 21.00000000000002132, -106.2556390011600342 ) ) ;
#614=CARTESIAN_POINT ( 'NONE',  ( -1.655278471874999990, 20.36702641396248481, -27.01827246956613138 ) ) ;
#616=CARTESIAN_POINT ( 'NONE',  ( 1.749999999999998224, 14.46891108675447946, -75.32139747004410424 ) ) ;
#619=CARTESIAN_POINT ( 'NONE',  ( 0.9378221735089300459, 21.00000000000002132, -101.9493890021159359 ) ) ;
#621=CARTESIAN_POINT ( 'NONE',  ( 1.655278471875001101, 20.36702641396249192, -75.09743913623280775 ) ) ;
#622=DIRECTION ( 'NONE',  ( 0.000000000000000000, 1.000000000000000000, 0.000000000000000000 ) ) ;
#628=CARTESIAN_POINT ( 'NONE',  ( 3.310556943749999981, 15.58864905735836892, -88.34743913623280775 ) ) ;
#629=EDGE_CURVE ( 'NONE', #8132, #26809, #35600, .T. ) ;
#630=( BOUNDED_CURVE ( )  B_SPLINE_CURVE ( 2, ( #41875, #28663, #35693, #35889, #39082, #22714, #6555, #31857, #3155 ),
 .UNSPECIFIED., .F., .T. ) 
 B_SPLINE_CURVE_WITH_KNOTS ( ( 3, 2, 2, 2, 3 ),
 ( 0.5979166666666666519, 0.5986111111111110938, 0.5999999999999999778, 0.6013888888888888618, 0.6020833333333333037 ),
 .UNSPECIFIED. ) 
 CURVE ( )  GEOMETRIC_REPRESENTATION_ITEM ( )  RATIONAL_B_SPLINE_CURVE ( ( 0.9330127018922194093, 0.9330127018922194093, 1.000000000000000000, 0.8660254037844387076, 1.000000000000000000, 0.8660254037844387076, 1.000000000000000000, 0.9330127018922194093, 0.9330127018922194093 ) ) 
 REPRESENTATION_ITEM ( '' )  );
#632=VERTEX_POINT ( 'NONE', #4709 ) ;
#634=EDGE_CURVE ( 'NONE', #26918, #3982, #37220, .T. ) ;
#637=CARTESIAN_POINT ( 'NONE',  ( 3.500000000000001332, 19.52072594216371826, -115.3776474690882168 ) ) ;
#639=CARTESIAN_POINT ( 'NONE',  ( 3.310556943750001313, 17.50000000000002132, -128.2641058028994792 ) ) ;
#642=CARTESIAN_POINT ( 'NONE',  ( 1.655278471875001101, 20.36702641396248836, -53.18493913623280633 ) ) ;
#643=CARTESIAN_POINT ( 'NONE',  ( 3.310556943750001313, 17.50000000000002132, -122.3516058028994706 ) ) ;
#644=VERTEX_POINT ( 'NONE', #27268 ) ;
#647=CARTESIAN_POINT ( 'NONE',  ( 3.500000000000000000, 15.47927405783633503, -124.2380641367107756 ) ) ;
#648=ADVANCED_FACE ( 'NONE', ( #21294 ), #37252, .T. ) ;
#649=CARTESIAN_POINT ( 'NONE',  ( -7.022189441860112050E-16, 13.67729811471671475, -37.51410580289947205 ) ) ;
#650=CARTESIAN_POINT ( 'NONE',  ( 3.310556943749999981, 15.58864905735836714, -71.43493913623278502 ) ) ;
#651=CARTESIAN_POINT ( 'NONE',  ( 3.500000000000001776, 19.52072594216371826, -120.3776474690881599 ) ) ;
#652=CARTESIAN_POINT ( 'NONE',  ( -3.310556943750002645, 15.58864905735837425, -103.6807724695661506 ) ) ;
#656=CARTESIAN_POINT ( 'NONE',  ( -3.500000000000001332, 17.50000000000001421, -67.96098080242150274 ) ) ;
#658=CARTESIAN_POINT ( 'NONE',  ( 0.000000000000000000, 17.50000000000002487, -149.5231586289125687 ) ) ;
#659=CARTESIAN_POINT ( 'NONE',  ( -1.655278471875002211, 14.63297358603754006, -35.59743913623280775 ) ) ;
#660=CARTESIAN_POINT ( 'NONE',  ( -3.310556943750002645, 15.58864905735837247, -94.76827246956611361 ) ) ;
#661=CARTESIAN_POINT ( 'NONE',  ( 3.500000000000001332, 17.50000000000001421, -60.15473080337743994 ) ) ;
#663=CARTESIAN_POINT ( 'NONE',  ( -1.655278471875002211, 14.63297358603755072, -110.6849391362327992 ) ) ;
#664=CARTESIAN_POINT ( 'NONE',  ( 3.310556943750001313, 19.41135094264166128, -44.26827246956613493 ) ) ;
#666=CARTESIAN_POINT ( 'NONE',  ( -1.394453263437886604E-15, 14.00000000000001421, -67.40473080337741862 ) ) ;
#671=CARTESIAN_POINT ( 'NONE',  ( -1.655278471874999990, 20.36702641396249192, -92.93077246956613635 ) ) ;
#672=CARTESIAN_POINT ( 'NONE',  ( -1.394453263437886604E-15, 14.00000000000001421, -62.71098080242150274 ) ) ;
#674=ORIENTED_EDGE ( 'NONE', *, *, #15576, .T. ) ;
#678=CARTESIAN_POINT ( 'NONE',  ( 0.9378221735089300459, 21.00000000000001066, -44.94938900211595012 ) ) ;
#683=CARTESIAN_POINT ( 'NONE',  ( 2.340729813953370519E-16, 21.32270188528330834, -30.01410580289948271 ) ) ;
#686=ORIENTED_EDGE ( 'NONE', *, *, #24192, .F. ) ;
#688=( BOUNDED_CURVE ( )  B_SPLINE_CURVE ( 2, ( #19679, #39449, #16709, #16300, #16506, #533, #29457, #10323, #23297 ),
 .UNSPECIFIED., .F., .F. ) 
 B_SPLINE_CURVE_WITH_KNOTS ( ( 3, 2, 2, 2, 3 ),
 ( 0.7979166666666667185, 0.7986111111111111605, 0.8000000000000000444, 0.8013888888888889284, 0.8020833333333333703 ),
 .UNSPECIFIED. ) 
 CURVE ( )  GEOMETRIC_REPRESENTATION_ITEM ( )  RATIONAL_B_SPLINE_CURVE ( ( 0.9330127018922194093, 0.9330127018922194093, 1.000000000000000000, 0.8660254037844387076, 1.000000000000000000, 0.8660254037844387076, 1.000000000000000000, 0.9330127018922194093, 0.9330127018922194093 ) ) 
 REPRESENTATION_ITEM ( '' )  );
#695=DIRECTION ( 'NONE',  ( 0.000000000000000000, 1.000000000000000000, 0.000000000000000000 ) ) ;
#697=CARTESIAN_POINT ( 'NONE',  ( -1.655278471874999990, 20.36702641396249902, -142.9307724695661364 ) ) ;
#698=CARTESIAN_POINT ( 'NONE',  ( 0.9378221735089281585, 14.00000000000001599, -68.66632260368298546 ) ) ;
#699=CARTESIAN_POINT ( 'NONE',  ( 4.648177544792955347E-16, 21.00000000000001776, -75.21098080242150274 ) ) ;
#700=CARTESIAN_POINT ( 'NONE',  ( -3.310556943750002645, 15.58864905735837958, -137.7682724695661420 ) ) ;
#701=CARTESIAN_POINT ( 'NONE',  ( -3.500000000000000888, 19.52072594216370405, -28.04431413575484200 ) ) ;
#703=CARTESIAN_POINT ( 'NONE',  ( 1.749999999999998224, 14.46891108675448834, -142.3213974700441042 ) ) ;
#706=CARTESIAN_POINT ( 'NONE',  ( -3.500000000000000888, 19.52072594216372181, -133.0443141357548313 ) ) ;
#707=CARTESIAN_POINT ( 'NONE',  ( 3.310556943750001313, 19.41135094264166838, -120.1807724695661506 ) ) ;
#710=CARTESIAN_POINT ( 'NONE',  ( 1.750000000000001110, 20.53108891324555785, -128.2943141357548313 ) ) ;
#711=CARTESIAN_POINT ( 'NONE',  ( 3.500000000000000000, 15.47927405783632615, -84.54431413575483134 ) ) ;
#713=CARTESIAN_POINT ( 'NONE',  ( 3.310556943750001313, 17.50000000000001421, -55.26410580289947916 ) ) ;
#714=CARTESIAN_POINT ( 'NONE',  ( -7.022189441860112050E-16, 13.67729811471672718, -112.6016058028994564 ) ) ;
#715=CARTESIAN_POINT ( 'NONE',  ( 1.749999999999998224, 14.46891108675447413, -38.62764746908817415 ) ) ;
#716=CARTESIAN_POINT ( 'NONE',  ( 2.474675557024783212E-16, 21.54145188432739033, -27.90473080337743639 ) ) ;
#720=CARTESIAN_POINT ( 'NONE',  ( 1.655278471875001101, 20.36702641396249902, -134.1849391362327992 ) ) ;
#722=CARTESIAN_POINT ( 'NONE',  ( 0.000000000000000000, 17.50000000000002487, -149.5231586289125687 ) ) ;
#723=CARTESIAN_POINT ( 'NONE',  ( 1.655278471875001101, 20.36702641396248836, -62.18493913623279923 ) ) ;
#724=AXIS2_PLACEMENT_3D ( 'NONE', #1922, #27871, #29076 ) ;
#726=CARTESIAN_POINT ( 'NONE',  ( 3.310556943749999981, 15.58864905735836537, -62.34743913623280775 ) ) ;
#728=CARTESIAN_POINT ( 'NONE',  ( 1.655278471874998436, 14.63297358603754539, -85.51827246956612782 ) ) ;
#734=CARTESIAN_POINT ( 'NONE',  ( 1.655278471874998436, 14.63297358603754006, -44.43077246956614346 ) ) ;
#736=CARTESIAN_POINT ( 'NONE',  ( -1.655278471875002211, 14.63297358603754894, -101.5974391362328078 ) ) ;
#737=CARTESIAN_POINT ( 'NONE',  ( -1.394453263437886604E-15, 14.00000000000001066, -53.40473080337743284 ) ) ;
#742=ORIENTED_EDGE ( 'NONE', *, *, #36802, .F. ) ;
#744=CARTESIAN_POINT ( 'NONE',  ( 2.340729813953370519E-16, 21.32270188528330834, -50.01410580289947205 ) ) ;
#745=VERTEX_POINT ( 'NONE', #11298 ) ;
#748=CARTESIAN_POINT ( 'NONE',  ( -3.500000000000001332, 17.50000000000001776, -95.96098080242150274 ) ) ;
#750=LINE ( 'NONE', #7342, #40816 ) ;
#753=CARTESIAN_POINT ( 'NONE',  ( -1.749999999999999778, 20.53108891324554719, -46.12764746908818125 ) ) ;
#754=CARTESIAN_POINT ( 'NONE',  ( -3.310556943750002645, 15.58864905735836714, -43.68077246956613635 ) ) ;
#755=CARTESIAN_POINT ( 'NONE',  ( 1.750000000000001110, 20.53108891324555785, -108.2943141357548456 ) ) ;
#756=CARTESIAN_POINT ( 'NONE',  ( 0.9378221735089300459, 21.00000000000001776, -96.94938900211595012 ) ) ;
#758=CARTESIAN_POINT ( 'NONE',  ( 4.648177544792955347E-16, 21.00000000000001776, -94.21098080242150274 ) ) ;
#760=CARTESIAN_POINT ( 'NONE',  ( 1.655278471875001101, 20.36702641396248481, -28.18493913623279568 ) ) ;
#762=CARTESIAN_POINT ( 'NONE',  ( -3.310556943750000425, 19.41135094264166483, -82.93493913623278502 ) ) ;
#763=CARTESIAN_POINT ( 'NONE',  ( 1.655278471874998436, 14.63297358603755072, -134.4307724695661364 ) ) ;
#769=CARTESIAN_POINT ( 'NONE',  ( 3.500000000000001332, 17.50000000000001776, -85.46098080242151696 ) ) ;
#770=CARTESIAN_POINT ( 'NONE',  ( -3.310556943750000425, 19.41135094264166838, -128.9349391362327992 ) ) ;
#771=CARTESIAN_POINT ( 'NONE',  ( 1.045839947578414805E-15, 14.00000000000002665, -141.4047308033774470 ) ) ;
#772=CARTESIAN_POINT ( 'NONE',  ( -7.022189441860112050E-16, 13.67729811471672363, -87.51410580289947916 ) ) ;
#773=CYLINDRICAL_SURFACE ( 'NONE', #21973, 3.499999999999999556 ) ;
#775=CARTESIAN_POINT ( 'NONE',  ( 0.000000000000000000, 17.50000000000002487, -149.5231586289125687 ) ) ;
#776=CARTESIAN_POINT ( 'NONE',  ( 2.474675557024783212E-16, 21.54145188432739744, -76.90473080337741862 ) ) ;
#777=CARTESIAN_POINT ( 'NONE',  ( 1.655278471875001101, 20.36702641396248836, -60.18493913623279923 ) ) ;
#781=CARTESIAN_POINT ( 'NONE',  ( 2.340729813953370519E-16, 21.32270188528331190, -78.10160580289945642 ) ) ;
#783=CARTESIAN_POINT ( 'NONE',  ( 1.655278471874998436, 14.63297358603755249, -142.5182724695661420 ) ) ;
#785=CARTESIAN_POINT ( 'NONE',  ( -3.310556943750002201, 15.58864905735837780, -110.6807724695661506 ) ) ;
#786=CARTESIAN_POINT ( 'NONE',  ( -1.655278471874999990, 20.36702641396249192, -79.93077246956615056 ) ) ;
#787=CARTESIAN_POINT ( 'NONE',  ( -8.715332896486792803E-15, 21.00000000000002842, -138.2109808024214601 ) ) ;
#789=CARTESIAN_POINT ( 'NONE',  ( 3.310556943749999981, 15.58864905735837070, -102.4349391362328134 ) ) ;
#790=CARTESIAN_POINT ( 'NONE',  ( -1.750000000000002220, 14.46891108675448478, -105.4880641367107614 ) ) ;
#793=CARTESIAN_POINT ( 'NONE',  ( 1.749999999999998224, 14.46891108675448123, -88.32139747004409003 ) ) ;
#794=CARTESIAN_POINT ( 'NONE',  ( 3.500000000000001332, 19.52072594216370760, -58.07139747004409713 ) ) ;
#797=CARTESIAN_POINT ( 'NONE',  ( 3.310556943750001313, 19.41135094264166483, -62.18077246956614346 ) ) ;
#799=CARTESIAN_POINT ( 'NONE',  ( 1.655278471875001101, 20.36702641396249547, -118.0974391362328078 ) ) ;
#800=CARTESIAN_POINT ( 'NONE',  ( 0.000000000000000000, 21.00000000000002487, -149.5231586289125687 ) ) ;
#803=ORIENTED_EDGE ( 'NONE', *, *, #36751, .T. ) ;
#807=CARTESIAN_POINT ( 'NONE',  ( -1.655278471875002211, 14.63297358603754361, -66.59743913623280775 ) ) ;
#809=ORIENTED_EDGE ( 'NONE', *, *, #121, .T. ) ;
#814=CARTESIAN_POINT ( 'NONE',  ( 1.655278471875001101, 20.36702641396249902, -137.0974391362328220 ) ) ;
#815=CARTESIAN_POINT ( 'NONE',  ( 0.9378221735089300459, 21.00000000000002487, -141.2556390011600058 ) ) ;
#816=( BOUNDED_CURVE ( )  B_SPLINE_CURVE ( 2, ( #4456, #5071, #20617, #30604, #17437, #30395, #8265, #14447, #22283 ),
 .UNSPECIFIED., .F., .T. ) 
 B_SPLINE_CURVE_WITH_KNOTS ( ( 3, 2, 2, 2, 3 ),
 ( 0.5562500000000000222, 0.5569444444444444642, 0.5583333333333333481, 0.5597222222222222321, 0.5604166666666666741 ),
 .UNSPECIFIED. ) 
 CURVE ( )  GEOMETRIC_REPRESENTATION_ITEM ( )  RATIONAL_B_SPLINE_CURVE ( ( 0.9330127018922194093, 0.9330127018922194093, 1.000000000000000000, 0.8660254037844387076, 1.000000000000000000, 0.8660254037844387076, 1.000000000000000000, 0.9330127018922194093, 0.9330127018922194093 ) ) 
 REPRESENTATION_ITEM ( '' )  );
#817=CARTESIAN_POINT ( 'NONE',  ( 3.310556943750001313, 17.50000000000001066, -45.35160580289947063 ) ) ;
#818=CARTESIAN_POINT ( 'NONE',  ( -3.310556943750002645, 15.58864905735836537, -39.76827246956612072 ) ) ;
#819=CARTESIAN_POINT ( 'NONE',  ( 1.655278471874998436, 14.63297358603754716, -96.51827246956612782 ) ) ;
#820=CIRCLE ( 'NONE', #24600, 3.499999999999999556 ) ;
#822=CARTESIAN_POINT ( 'NONE',  ( -3.310556943750002645, 15.58864905735836182, -25.68077246956613990 ) ) ;
#823=DIRECTION ( 'NONE',  ( -0.000000000000000000, 1.259100132267607459E-16, -1.000000000000000000 ) ) ;
#824=CARTESIAN_POINT ( 'NONE',  ( 1.750000000000001110, 20.53108891324555429, -99.29431413575484555 ) ) ;
#825=CARTESIAN_POINT ( 'NONE',  ( 4.648177544792955347E-16, 21.00000000000001421, -73.90473080337743284 ) ) ;
#827=CARTESIAN_POINT ( 'NONE',  ( -3.500000000000002220, 15.47927405783632793, -91.57139747004410424 ) ) ;
#832=CARTESIAN_POINT ( 'NONE',  ( 3.500000000000001776, 19.52072594216370760, -53.37764746908817415 ) ) ;
#833=CARTESIAN_POINT ( 'NONE',  ( -3.500000000000001332, 17.50000000000001066, -46.65473080337742573 ) ) ;
#834=CARTESIAN_POINT ( 'NONE',  ( 0.000000000000000000, 21.00000000000002487, -149.5231586289125687 ) ) ;
#837=CARTESIAN_POINT ( 'NONE',  ( -1.750000000000002220, 14.46891108675447768, -44.48806413671076143 ) ) ;
#838=CARTESIAN_POINT ( 'NONE',  ( 2.340729813953370519E-16, 21.32270188528330834, -29.10160580289947063 ) ) ;
#843=CARTESIAN_POINT ( 'NONE',  ( -1.394453263437886604E-15, 14.00000000000002132, -120.4047308033774328 ) ) ;
#845=CARTESIAN_POINT ( 'NONE',  ( 3.310556943749999981, 15.58864905735836714, -78.34743913623280775 ) ) ;
#846=CARTESIAN_POINT ( 'NONE',  ( 3.500000000000001332, 17.50000000000001421, -52.46098080242150985 ) ) ;
#847=ORIENTED_EDGE ( 'NONE', *, *, #31848, .F. ) ;
#849=CARTESIAN_POINT ( 'NONE',  ( 1.750000000000001110, 20.53108891324555429, -89.98806413671076143 ) ) ;
#852=CARTESIAN_POINT ( 'NONE',  ( -3.500000000000000000, 19.52072594216371115, -88.04431413575483134 ) ) ;
#853=CARTESIAN_POINT ( 'NONE',  ( -7.022189441860112050E-16, 13.67729811471672363, -92.51410580289949337 ) ) ;
#860=CARTESIAN_POINT ( 'NONE',  ( -3.310556943750000425, 19.41135094264166838, -125.8474391362328078 ) ) ;
#861=CARTESIAN_POINT ( 'NONE',  ( 1.750000000000001110, 20.53108891324555074, -63.98806413671076143 ) ) ;
#862=CARTESIAN_POINT ( 'NONE',  ( -3.310556943750002645, 15.58864905735836892, -54.76827246956612072 ) ) ;
#863=CARTESIAN_POINT ( 'NONE',  ( 1.655278471874998436, 14.63297358603754894, -113.5182724695661278 ) ) ;
#866=CARTESIAN_POINT ( 'NONE',  ( 1.749999999999998224, 14.46891108675448656, -127.3213974700440900 ) ) ;
#867=CARTESIAN_POINT ( 'NONE',  ( -3.310556943750002645, 15.58864905735836537, -37.68077246956613635 ) ) ;
#869=CARTESIAN_POINT ( 'NONE',  ( -1.655278471874999990, 20.36702641396248836, -64.01827246956614204 ) ) ;
#870=CARTESIAN_POINT ( 'NONE',  ( 1.750000000000001110, 20.53108891324555785, -115.2943141357548313 ) ) ;
#871=VECTOR ( 'NONE', #15495, 1000.000000000000000 ) ;
#872=EDGE_CURVE ( 'NONE', #11828, #29770, #20944, .T. ) ;
#873=CYLINDRICAL_SURFACE ( 'NONE', #32921, 3.499999999999999556 ) ;
#874=CYLINDRICAL_SURFACE ( 'NONE', #6894, 3.499999999999999556 ) ;
#877=CARTESIAN_POINT ( 'NONE',  ( -3.500000000000000888, 19.52072594216370760, -68.04431413575484555 ) ) ;
#878=DIRECTION ( 'NONE',  ( -0.000000000000000000, 1.259100132267607459E-16, -1.000000000000000000 ) ) ;
#879=CARTESIAN_POINT ( 'NONE',  ( 3.310556943750001313, 17.50000000000001066, -39.26410580289947916 ) ) ;
#880=CARTESIAN_POINT ( 'NONE',  ( -3.310556943750001313, 17.50000000000001776, -96.85160580289945642 ) ) ;
#881=CARTESIAN_POINT ( 'NONE',  ( -3.500000000000002220, 15.47927405783632437, -61.57139747004410424 ) ) ;
#883=CARTESIAN_POINT ( 'NONE',  ( -1.655278471875002211, 14.63297358603755072, -114.6849391362327850 ) ) ;
#884=CARTESIAN_POINT ( 'NONE',  ( 1.655278471875001101, 20.36702641396248481, -41.18493913623279212 ) ) ;
#890=DIRECTION ( 'NONE',  ( -0.000000000000000000, 1.259100132267607459E-16, -1.000000000000000000 ) ) ;
#891=CARTESIAN_POINT ( 'NONE',  ( -3.310556943750002201, 15.58864905735837247, -91.68077246956615056 ) ) ;
#892=( BOUNDED_CURVE ( )  B_SPLINE_CURVE ( 2, ( #9471, #18628, #40962, #21600, #41596, #25017, #32013, #28399, #25222 ),
 .UNSPECIFIED., .F., .F. ) 
 B_SPLINE_CURVE_WITH_KNOTS ( ( 3, 2, 2, 2, 3 ),
 ( 0.6312499999999999778, 0.6319444444444444198, 0.6333333333333333037, 0.6347222222222221877, 0.6354166666666666297 ),
 .UNSPECIFIED. ) 
 CURVE ( )  GEOMETRIC_REPRESENTATION_ITEM ( )  RATIONAL_B_SPLINE_CURVE ( ( 0.9330127018922194093, 0.9330127018922194093, 1.000000000000000000, 0.8660254037844387076, 1.000000000000000000, 0.8660254037844387076, 1.000000000000000000, 0.9330127018922194093, 0.9330127018922194093 ) ) 
 REPRESENTATION_ITEM ( '' )  );
#893=CARTESIAN_POINT ( 'NONE',  ( 0.9378221735089300459, 21.00000000000001421, -62.25563900116003424 ) ) ;
#896=CYLINDRICAL_SURFACE ( 'NONE', #17936, 3.499999999999999556 ) ;
#898=CARTESIAN_POINT ( 'NONE',  ( -3.500000000000001332, 17.50000000000002132, -105.6547308033774186 ) ) ;
#899=ORIENTED_EDGE ( 'NONE', *, *, #21977, .T. ) ;
#902=CARTESIAN_POINT ( 'NONE',  ( -7.022189441860112050E-16, 13.67729811471671653, -28.51410580289947916 ) ) ;
#904=EDGE_CURVE ( 'NONE', #21358, #2263, #12500, .T. ) ;
#911=ORIENTED_EDGE ( 'NONE', *, *, #18453, .F. ) ;
#917=CARTESIAN_POINT ( 'NONE',  ( -3.310556943750001313, 17.50000000000002132, -128.8516058028994564 ) ) ;
#918=CARTESIAN_POINT ( 'NONE',  ( 3.500000000000001776, 19.52072594216370405, -27.37764746908817415 ) ) ;
#920=ADVANCED_FACE ( 'NONE', ( #27823 ), #40387, .T. ) ;
#922=CARTESIAN_POINT ( 'NONE',  ( 3.500000000000000000, 15.47927405783633503, -140.2380641367107330 ) ) ;
#923=CARTESIAN_POINT ( 'NONE',  ( 0.9378221735089300459, 21.00000000000001066, -42.94938900211595012 ) ) ;
#925=CARTESIAN_POINT ( 'NONE',  ( 3.500000000000000000, 15.47927405783633503, -134.5443141357548313 ) ) ;
#926=CARTESIAN_POINT ( 'NONE',  ( 2.340729813953370519E-16, 21.32270188528331900, -118.0141058028994792 ) ) ;
#928=CARTESIAN_POINT ( 'NONE',  ( 1.749999999999998224, 14.46891108675448656, -128.6276474690881741 ) ) ;
#929=CARTESIAN_POINT ( 'NONE',  ( -3.500000000000000888, 19.52072594216371115, -87.04431413575483134 ) ) ;
#931=CARTESIAN_POINT ( 'NONE',  ( -7.022189441860112050E-16, 13.67729811471671653, -53.51410580289947205 ) ) ;
#933=CARTESIAN_POINT ( 'NONE',  ( -1.655278471875002211, 14.63297358603755072, -112.6849391362327992 ) ) ;
#934=CARTESIAN_POINT ( 'NONE',  ( 7.367361408496833051E-14, 14.00000000000001776, -93.71098080242150274 ) ) ;
#935=CARTESIAN_POINT ( 'NONE',  ( -1.749999999999999778, 20.53108891324554719, -28.82139747004410069 ) ) ;
#936=AXIS2_PLACEMENT_3D ( 'NONE', #19600, #32573, #3032 ) ;
#937=CARTESIAN_POINT ( 'NONE',  ( 0.9378221735089455890, 14.00000000000003197, -116.6663226036829712 ) ) ;
#939=CARTESIAN_POINT ( 'NONE',  ( -7.022189441860112050E-16, 13.67729811471672896, -129.6016058028994564 ) ) ;
#942=CARTESIAN_POINT ( 'NONE',  ( 0.9378221735089300459, 21.00000000000001421, -58.25563900116003424 ) ) ;
#943=CARTESIAN_POINT ( 'NONE',  ( -1.655278471874999990, 20.36702641396248836, -63.01827246956613493 ) ) ;
#945=ORIENTED_EDGE ( 'NONE', *, *, #3273, .T. ) ;
#947=CARTESIAN_POINT ( 'NONE',  ( 2.340729813953370519E-16, 21.32270188528331190, -80.10160580289944221 ) ) ;
#948=AXIS2_PLACEMENT_3D ( 'NONE', #27215, #8469, #2086 ) ;
#953=CARTESIAN_POINT ( 'NONE',  ( 1.655278471874998436, 14.63297358603754006, -47.43077246956614346 ) ) ;
#955=CARTESIAN_POINT ( 'NONE',  ( -1.655278471874999990, 20.36702641396249547, -102.9307724695661364 ) ) ;
#959=ORIENTED_EDGE ( 'NONE', *, *, #13559, .T. ) ;
#961=CARTESIAN_POINT ( 'NONE',  ( 3.310556943750001313, 19.41135094264166128, -55.18077246956614346 ) ) ;
#964=CARTESIAN_POINT ( 'NONE',  ( -1.394453263437886604E-15, 14.00000000000001066, -43.40473080337742573 ) ) ;
#967=VECTOR ( 'NONE', #19990, 1000.000000000000000 ) ;
#968=CARTESIAN_POINT ( 'NONE',  ( 4.286263797015737581E-16, 14.00000000000002487, -149.5231586289125687 ) ) ;
#969=EDGE_CURVE ( 'NONE', #11365, #23350, #22551, .T. ) ;
#970=ORIENTED_EDGE ( 'NONE', *, *, #24323, .T. ) ;
#972=CARTESIAN_POINT ( 'NONE',  ( -1.749999999999999778, 20.53108891324554719, -44.12764746908817415 ) ) ;
#974=CARTESIAN_POINT ( 'NONE',  ( -1.394453263437886604E-15, 14.00000000000002132, -119.4047308033774328 ) ) ;
#977=CARTESIAN_POINT ( 'NONE',  ( 3.310556943750001313, 17.50000000000001066, -28.35160580289947063 ) ) ;
#978=CARTESIAN_POINT ( 'NONE',  ( -3.500000000000000000, 19.52072594216371115, -97.73806413671076143 ) ) ;
#979=CARTESIAN_POINT ( 'NONE',  ( -3.310556943750001313, 17.50000000000001776, -81.85160580289945642 ) ) ;
#980=CARTESIAN_POINT ( 'NONE',  ( 3.310556943750001313, 17.50000000000002487, -133.2641058028994507 ) ) ;
#986=CARTESIAN_POINT ( 'NONE',  ( 1.749999999999998224, 14.46891108675448123, -85.62764746908817415 ) ) ;
#987=CARTESIAN_POINT ( 'NONE',  ( 3.310556943749999981, 15.58864905735837425, -130.4349391362327992 ) ) ;
#988=CARTESIAN_POINT ( 'NONE',  ( -1.749999999999999778, 20.53108891324555074, -69.12764746908817415 ) ) ;
#989=CARTESIAN_POINT ( 'NONE',  ( -3.310556943750001313, 17.50000000000001776, -86.76410580289947916 ) ) ;
#991=DIRECTION ( 'NONE',  ( 0.000000000000000000, -1.000000000000000000, -3.845925372767130591E-16 ) ) ;
#992=CARTESIAN_POINT ( 'NONE',  ( 1.750000000000001110, 20.53108891324555429, -88.98806413671076143 ) ) ;
#993=CARTESIAN_POINT ( 'NONE',  ( 3.500000000000001776, 19.52072594216370760, -68.07139747004409003 ) ) ;
#994=CARTESIAN_POINT ( 'NONE',  ( 3.310556943750001313, 19.41135094264166483, -56.26827246956613493 ) ) ;
#996=CARTESIAN_POINT ( 'NONE',  ( -8.715332896486792803E-15, 21.00000000000002842, -137.2109808024214885 ) ) ;
#998=CARTESIAN_POINT ( 'NONE',  ( -1.655278471875002211, 14.63297358603754539, -80.68493913623279923 ) ) ;
#999=CARTESIAN_POINT ( 'NONE',  ( 3.310556943750001313, 17.50000000000002487, -138.3516058028994564 ) ) ;
#1001=CARTESIAN_POINT ( 'NONE',  ( -3.310556943750000425, 19.41135094264166838, -107.8474391362328078 ) ) ;
#1002=CARTESIAN_POINT ( 'NONE',  ( 1.655278471875001101, 20.36702641396248836, -73.09743913623280775 ) ) ;
#1003=LINE ( 'NONE', #37719, #16554 ) ;
#1005=CARTESIAN_POINT ( 'NONE',  ( -3.310556943750001313, 17.50000000000001776, -100.8516058028994706 ) ) ;
#1006=CARTESIAN_POINT ( 'NONE',  ( 2.474675557024783212E-16, 21.54145188432740099, -103.9047308033774186 ) ) ;
#1009=CARTESIAN_POINT ( 'NONE',  ( 4.648177544792955347E-16, 21.00000000000001776, -86.90473080337741862 ) ) ;
#1010=DIRECTION ( 'NONE',  ( -0.000000000000000000, 1.259100132267607459E-16, -1.000000000000000000 ) ) ;
#1012=CARTESIAN_POINT ( 'NONE',  ( 2.340729813953370519E-16, 21.32270188528331190, -63.01410580289947205 ) ) ;
#1013=CARTESIAN_POINT ( 'NONE',  ( -1.749999999999999778, 20.53108891324555785, -125.1276474690881599 ) ) ;
#1014=CARTESIAN_POINT ( 'NONE',  ( 3.310556943750001313, 19.41135094264166838, -117.1807724695661506 ) ) ;
#1015=CARTESIAN_POINT ( 'NONE',  ( 4.648177544792955347E-16, 21.00000000000001066, -43.90473080337743284 ) ) ;
#1017=VERTEX_POINT ( 'NONE', #18880 ) ;
#1023=CARTESIAN_POINT ( 'NONE',  ( -3.310556943750000425, 19.41135094264166128, -66.84743913623280775 ) ) ;
#1031=ORIENTED_EDGE ( 'NONE', *, *, #6803, .T. ) ;
#1032=CARTESIAN_POINT ( 'NONE',  ( -7.022189441860112050E-16, 13.67729811471672896, -133.5141058028994507 ) ) ;
#1034=CARTESIAN_POINT ( 'NONE',  ( 3.310556943749999981, 15.58864905735836182, -44.43493913623279923 ) ) ;
#1035=CARTESIAN_POINT ( 'NONE',  ( -7.022189441860112050E-16, 13.67729811471671653, -40.60160580289947063 ) ) ;
#1036=EDGE_CURVE ( 'NONE', #15782, #34588, #31429, .T. ) ;
#1037=CARTESIAN_POINT ( 'NONE',  ( 3.310556943749999981, 15.58864905735837070, -99.43493913623281344 ) ) ;
#1039=CARTESIAN_POINT ( 'NONE',  ( -1.655278471874999990, 20.36702641396249902, -143.0182724695661420 ) ) ;
#1042=CARTESIAN_POINT ( 'NONE',  ( 3.500000000000001332, 17.50000000000001776, -101.4609808024215170 ) ) ;
#1043=CARTESIAN_POINT ( 'NONE',  ( 1.750000000000001110, 20.53108891324555429, -99.98806413671077564 ) ) ;
#1044=CARTESIAN_POINT ( 'NONE',  ( -3.500000000000000000, 19.52072594216370760, -61.73806413671076143 ) ) ;
#1045=CARTESIAN_POINT ( 'NONE',  ( 2.474675557024783212E-16, 21.54145188432739744, -88.90473080337743284 ) ) ;
#1048=CARTESIAN_POINT ( 'NONE',  ( 3.500000000000000000, 15.47927405783632793, -84.23806413671076143 ) ) ;
#1051=CARTESIAN_POINT ( 'NONE',  ( 3.500000000000001332, 17.50000000000001421, -53.46098080242150985 ) ) ;
#1053=ORIENTED_EDGE ( 'NONE', *, *, #24174, .T. ) ;
#1054=CARTESIAN_POINT ( 'NONE',  ( -1.749999999999999778, 20.53108891324554719, -43.82139747004409713 ) ) ;
#1056=CARTESIAN_POINT ( 'NONE',  ( 3.310556943750001313, 17.50000000000001066, -27.35160580289947063 ) ) ;
#1057=CARTESIAN_POINT ( 'NONE',  ( 0.9378221735089300459, 21.00000000000001776, -74.94938900211595012 ) ) ;
#1058=CARTESIAN_POINT ( 'NONE',  ( -3.500000000000002220, 15.47927405783632615, -60.57139747004410424 ) ) ;
#1060=CARTESIAN_POINT ( 'NONE',  ( -3.500000000000001332, 17.50000000000002132, -106.9609808024215027 ) ) ;
#1062=CARTESIAN_POINT ( 'NONE',  ( -3.310556943750002201, 15.58864905735837070, -76.68077246956615056 ) ) ;
#1063=CARTESIAN_POINT ( 'NONE',  ( 4.648177544792955347E-16, 21.00000000000002487, -134.2109808024215170 ) ) ;
#1067=ORIENTED_EDGE ( 'NONE', *, *, #121, .F. ) ;
#1068=EDGE_CURVE ( 'NONE', #8756, #20830, #39701, .T. ) ;
#1069=CARTESIAN_POINT ( 'NONE',  ( 4.648177544792955347E-16, 21.00000000000001421, -64.21098080242150274 ) ) ;
#1070=CARTESIAN_POINT ( 'NONE',  ( -7.022189441860112050E-16, 13.67729811471672363, -84.51410580289947916 ) ) ;
#1072=EDGE_LOOP ( 'NONE', ( #30028, #15668, #19364, #28617 ) ) ;
#1074=( BOUNDED_CURVE ( )  B_SPLINE_CURVE ( 2, ( #22833, #35801, #16666, #29624, #9236, #6039, #19016, #30474, #1344 ),
 .UNSPECIFIED., .F., .F. ) 
 B_SPLINE_CURVE_WITH_KNOTS ( ( 3, 2, 2, 2, 3 ),
 ( 0.8812499999999999778, 0.8819444444444444198, 0.8833333333333333037, 0.8847222222222221877, 0.8854166666666666297 ),
 .UNSPECIFIED. ) 
 CURVE ( )  GEOMETRIC_REPRESENTATION_ITEM ( )  RATIONAL_B_SPLINE_CURVE ( ( 0.9330127018922194093, 0.9330127018922194093, 1.000000000000000000, 0.8660254037844387076, 1.000000000000000000, 0.8660254037844387076, 1.000000000000000000, 0.9330127018922194093, 0.9330127018922194093 ) ) 
 REPRESENTATION_ITEM ( '' )  );
#1075=VECTOR ( 'NONE', #40792, 1000.000000000000000 ) ;
#1079=CARTESIAN_POINT ( 'NONE',  ( -3.310556943750001313, 17.50000000000002132, -128.7641058028994792 ) ) ;
#1082=CARTESIAN_POINT ( 'NONE',  ( -3.310556943750002645, 15.58864905735836892, -55.76827246956613493 ) ) ;
#1084=CARTESIAN_POINT ( 'NONE',  ( -3.310556943750001313, 17.50000000000002132, -114.8516058028994706 ) ) ;
#1085=ORIENTED_EDGE ( 'NONE', *, *, #5156, .T. ) ;
#1087=CARTESIAN_POINT ( 'NONE',  ( -3.500000000000001332, 17.50000000000002132, -124.6547308033774186 ) ) ;
#1088=CARTESIAN_POINT ( 'NONE',  ( -1.655278471875002211, 14.63297358603754006, -39.59743913623281486 ) ) ;
#1089=CARTESIAN_POINT ( 'NONE',  ( -1.655278471874999990, 20.36702641396248836, -66.01827246956612782 ) ) ;
#1090=CARTESIAN_POINT ( 'NONE',  ( 2.474675557024783212E-16, 21.54145188432740099, -116.2109808024215170 ) ) ;
#1091=CARTESIAN_POINT ( 'NONE',  ( 3.310556943749999981, 15.58864905735837070, -101.3474391362328220 ) ) ;
#1092=FACE_OUTER_BOUND ( 'NONE', #39121, .T. ) ;
#1094=CARTESIAN_POINT ( 'NONE',  ( -1.394453263437886604E-15, 14.00000000000001066, -26.40473080337743284 ) ) ;
#1096=CARTESIAN_POINT ( 'NONE',  ( 2.474675557024783212E-16, 21.54145188432739388, -68.21098080242150274 ) ) ;
#1097=CARTESIAN_POINT ( 'NONE',  ( -1.394453263437886604E-15, 14.00000000000001776, -100.7109808024215027 ) ) ;
#1098=CARTESIAN_POINT ( 'NONE',  ( 1.655278471875001101, 20.36702641396248481, -38.09743913623281486 ) ) ;
#1099=CARTESIAN_POINT ( 'NONE',  ( 3.310556943750001313, 19.41135094264166483, -93.26827246956611361 ) ) ;
#1100=CARTESIAN_POINT ( 'NONE',  ( -1.749999999999999778, 20.53108891324555074, -59.82139747004409713 ) ) ;
#1101=CARTESIAN_POINT ( 'NONE',  ( -3.310556943750002201, 15.58864905735837780, -114.7682724695661278 ) ) ;
#1102=CARTESIAN_POINT ( 'NONE',  ( -1.655278471875002211, 14.63297358603754184, -44.68493913623279923 ) ) ;
#1109=CARTESIAN_POINT ( 'NONE',  ( -3.310556943750001313, 17.50000000000001776, -94.76410580289946495 ) ) ;
#1110=CARTESIAN_POINT ( 'NONE',  ( 3.500000000000001332, 19.52072594216370405, -39.07139747004409713 ) ) ;
#1115=CARTESIAN_POINT ( 'NONE',  ( -3.500000000000001332, 17.50000000000001776, -78.96098080242150274 ) ) ;
#1116=VERTEX_POINT ( 'NONE', #21442 ) ;
#1119=CARTESIAN_POINT ( 'NONE',  ( -3.500000000000000000, 19.52072594216371826, -133.0443141357548598 ) ) ;
#1120=ORIENTED_EDGE ( 'NONE', *, *, #7412, .F. ) ;
#1121=CARTESIAN_POINT ( 'NONE',  ( -1.394453263437886604E-15, 14.00000000000001421, -65.40473080337743284 ) ) ;
#1125=VERTEX_POINT ( 'NONE', #5907 ) ;
#1126=CARTESIAN_POINT ( 'NONE',  ( 4.648177544792955347E-16, 21.00000000000001421, -54.21098080242150985 ) ) ;
#1130=CARTESIAN_POINT ( 'NONE',  ( 3.500000000000001332, 17.50000000000001421, -68.46098080242150274 ) ) ;
#1131=CARTESIAN_POINT ( 'NONE',  ( 4.648177544792955347E-16, 21.00000000000001421, -56.21098080242150985 ) ) ;
#1132=CARTESIAN_POINT ( 'NONE',  ( -7.022189441860112050E-16, 13.67729811471672718, -132.6016058028994564 ) ) ;
#1133=CARTESIAN_POINT ( 'NONE',  ( 3.500000000000000000, 15.47927405783632082, -30.54431413575483845 ) ) ;
#1135=CARTESIAN_POINT ( 'NONE',  ( -3.500000000000001332, 17.50000000000002487, -140.6547308033774186 ) ) ;
#1138=CARTESIAN_POINT ( 'NONE',  ( -1.749999999999999778, 20.53108891324556140, -131.1276474690881741 ) ) ;
#1139=CARTESIAN_POINT ( 'NONE',  ( -3.310556943750001313, 17.50000000000002132, -116.7641058028994792 ) ) ;
#1141=( BOUNDED_CURVE ( )  B_SPLINE_CURVE ( 2, ( #9959, #22919, #6748, #35883, #39492, #23341, #32690, #367, #3552 ),
 .UNSPECIFIED., .F., .F. ) 
 B_SPLINE_CURVE_WITH_KNOTS ( ( 3, 2, 2, 2, 3 ),
 ( 0.7395833333333333703, 0.7402777777777778123, 0.7416666666666666963, 0.7430555555555555802, 0.7437500000000000222 ),
 .UNSPECIFIED. ) 
 CURVE ( )  GEOMETRIC_REPRESENTATION_ITEM ( )  RATIONAL_B_SPLINE_CURVE ( ( 0.9330127018922194093, 0.9330127018922194093, 1.000000000000000000, 0.8660254037844387076, 1.000000000000000000, 0.8660254037844387076, 1.000000000000000000, 0.9330127018922194093, 0.9330127018922194093 ) ) 
 REPRESENTATION_ITEM ( '' )  );
#1143=CARTESIAN_POINT ( 'NONE',  ( -7.424026671074350129E-16, 13.45854811567263631, -83.71098080242151696 ) ) ;
#1144=CARTESIAN_POINT ( 'NONE',  ( -1.394453263437886604E-15, 14.00000000000001776, -92.40473080337741862 ) ) ;
#1145=CARTESIAN_POINT ( 'NONE',  ( -1.655278471874999990, 20.36702641396248836, -54.93077246956613635 ) ) ;
#1146=CARTESIAN_POINT ( 'NONE',  ( -3.310556943750001313, 17.50000000000002132, -109.8516058028994564 ) ) ;
#1151=CARTESIAN_POINT ( 'NONE',  ( 3.310556943750001313, 19.41135094264167549, -130.2682724695661136 ) ) ;
#1154=CARTESIAN_POINT ( 'NONE',  ( 1.749999999999998224, 14.46891108675448123, -83.32139747004410424 ) ) ;
#1155=LINE ( 'NONE', #36667, #41452 ) ;
#1156=CARTESIAN_POINT ( 'NONE',  ( -3.310556943750000425, 19.41135094264166128, -65.93493913623279923 ) ) ;
#1158=CARTESIAN_POINT ( 'NONE',  ( 1.655278471875001101, 20.36702641396249192, -83.18493913623278502 ) ) ;
#1159=CARTESIAN_POINT ( 'NONE',  ( 3.500000000000000000, 15.47927405783632615, -77.23806413671076143 ) ) ;
#1160=CARTESIAN_POINT ( 'NONE',  ( 1.750000000000001110, 20.53108891324554719, -25.98806413671075788 ) ) ;
#1163=CARTESIAN_POINT ( 'NONE',  ( -3.310556943750000425, 19.41135094264166128, -43.84743913623280775 ) ) ;
#1164=CARTESIAN_POINT ( 'NONE',  ( -1.655278471875002211, 14.63297358603754894, -98.59743913623280775 ) ) ;
#1170=CARTESIAN_POINT ( 'NONE',  ( 3.310556943750001313, 19.41135094264166128, -53.18077246956613635 ) ) ;
#1173=ORIENTED_EDGE ( 'NONE', *, *, #18911, .F. ) ;
#1174=CARTESIAN_POINT ( 'NONE',  ( -1.750000000000002220, 14.46891108675447768, -43.48806413671076143 ) ) ;
#1175=CARTESIAN_POINT ( 'NONE',  ( -0.9378221735089291577, 21.00000000000001776, -91.86007260463891555 ) ) ;
#1180=CARTESIAN_POINT ( 'NONE',  ( 2.474675557024783212E-16, 21.54145188432739033, -43.21098080242151696 ) ) ;
#1183=CARTESIAN_POINT ( 'NONE',  ( 3.310556943749999981, 15.58864905735836182, -30.43493913623279568 ) ) ;
#1184=DIRECTION ( 'NONE',  ( 0.000000000000000000, 1.000000000000000000, 0.000000000000000000 ) ) ;
#1185=CARTESIAN_POINT ( 'NONE',  ( -3.310556943750001313, 17.50000000000001776, -84.85160580289947063 ) ) ;
#1186=CARTESIAN_POINT ( 'NONE',  ( -7.022189441860112050E-16, 13.67729811471672718, -133.5141058028994507 ) ) ;
#1192=( BOUNDED_CURVE ( )  B_SPLINE_CURVE ( 2, ( #9962, #16342, #23126, #3768, #16752, #19725, #16549, #29500, #370 ),
 .UNSPECIFIED., .F., .T. ) 
 B_SPLINE_CURVE_WITH_KNOTS ( ( 3, 2, 2, 2, 3 ),
 ( 0.9437499999999999778, 0.9444444444444444198, 0.9458333333333333037, 0.9472222222222221877, 0.9479166666666666297 ),
 .UNSPECIFIED. ) 
 CURVE ( )  GEOMETRIC_REPRESENTATION_ITEM ( )  RATIONAL_B_SPLINE_CURVE ( ( 0.9330127018922194093, 0.9330127018922194093, 1.000000000000000000, 0.8660254037844387076, 1.000000000000000000, 0.8660254037844387076, 1.000000000000000000, 0.9330127018922194093, 0.9330127018922194093 ) ) 
 REPRESENTATION_ITEM ( '' )  );
#1193=CARTESIAN_POINT ( 'NONE',  ( 1.655278471875001101, 20.36702641396249547, -129.1849391362327992 ) ) ;
#1194=EDGE_CURVE ( 'NONE', #524, #35484, #21192, .T. ) ;
#1195=CARTESIAN_POINT ( 'NONE',  ( -3.500000000000001332, 17.50000000000001421, -68.96098080242150274 ) ) ;
#1196=CARTESIAN_POINT ( 'NONE',  ( 1.655278471874998436, 14.63297358603754539, -86.43077246956613635 ) ) ;
#1198=DIRECTION ( 'NONE',  ( -0.000000000000000000, 1.259100132267607459E-16, -1.000000000000000000 ) ) ;
#1200=CARTESIAN_POINT ( 'NONE',  ( 3.500000000000000000, 15.47927405783632437, -71.23806413671076143 ) ) ;
#1201=CARTESIAN_POINT ( 'NONE',  ( 1.655278471874998436, 14.63297358603754184, -55.51827246956612782 ) ) ;
#1203=CARTESIAN_POINT ( 'NONE',  ( 0.000000000000000000, 17.50000000000002487, -149.5231586289125687 ) ) ;
#1205=CARTESIAN_POINT ( 'NONE',  ( -3.310556943750000425, 19.41135094264166483, -78.93493913623279923 ) ) ;
#1206=CARTESIAN_POINT ( 'NONE',  ( 1.655278471874998436, 14.63297358603755249, -140.5182724695661420 ) ) ;
#1208=CARTESIAN_POINT ( 'NONE',  ( -3.310556943750001313, 17.50000000000002132, -108.7641058028994649 ) ) ;
#1209=CARTESIAN_POINT ( 'NONE',  ( -1.655278471875002211, 14.63297358603754539, -77.59743913623280775 ) ) ;
#1212=CARTESIAN_POINT ( 'NONE',  ( -1.655278471874999990, 20.36702641396249192, -98.01827246956612782 ) ) ;
#1213=CARTESIAN_POINT ( 'NONE',  ( -3.500000000000002220, 15.47927405783632970, -99.57139747004409003 ) ) ;
#1216=CARTESIAN_POINT ( 'NONE',  ( 0.9378221735089281585, 14.00000000000000888, -26.66632260368299256 ) ) ;
#1218=CARTESIAN_POINT ( 'NONE',  ( -3.310556943750002201, 15.58864905735836892, -63.68077246956614346 ) ) ;
#1219=CARTESIAN_POINT ( 'NONE',  ( -1.750000000000002220, 14.46891108675448656, -112.7943141357548456 ) ) ;
#1220=CARTESIAN_POINT ( 'NONE',  ( -3.310556943750002645, 15.58864905735837780, -116.6807724695661506 ) ) ;
#1221=CARTESIAN_POINT ( 'NONE',  ( 1.749999999999998224, 14.46891108675447413, -36.62764746908816704 ) ) ;
#1224=VERTEX_POINT ( 'NONE', #33101 ) ;
#1226=CARTESIAN_POINT ( 'NONE',  ( 1.750000000000001110, 20.53108891324556140, -130.9880641367107614 ) ) ;
#1227=CARTESIAN_POINT ( 'NONE',  ( 1.749999999999998224, 14.46891108675447413, -33.62764746908818125 ) ) ;
#1228=CARTESIAN_POINT ( 'NONE',  ( 3.310556943750001313, 17.50000000000001421, -66.26410580289947916 ) ) ;
#1229=EDGE_CURVE ( 'NONE', #19472, #41304, #25292, .T. ) ;
#1231=ORIENTED_EDGE ( 'NONE', *, *, #7811, .T. ) ;
#1239=CARTESIAN_POINT ( 'NONE',  ( -3.310556943750002201, 15.58864905735837958, -136.6807724695661364 ) ) ;
#1241=CARTESIAN_POINT ( 'NONE',  ( -3.310556943750000425, 19.41135094264166128, -46.93493913623279923 ) ) ;
#1242=DIRECTION ( 'NONE',  ( -0.000000000000000000, 1.259100132267607459E-16, -1.000000000000000000 ) ) ;
#1243=CARTESIAN_POINT ( 'NONE',  ( -3.310556943750001313, 17.50000000000001066, -39.85160580289947063 ) ) ;
#1244=CARTESIAN_POINT ( 'NONE',  ( -3.310556943750001313, 17.50000000000001776, -96.85160580289945642 ) ) ;
#1246=CARTESIAN_POINT ( 'NONE',  ( 2.340729813953370519E-16, 21.32270188528332255, -142.1016058028994564 ) ) ;
#1248=CARTESIAN_POINT ( 'NONE',  ( 1.749999999999998224, 14.46891108675448123, -94.62764746908815994 ) ) ;
#1250=CARTESIAN_POINT ( 'NONE',  ( 1.045839947578414805E-15, 14.00000000000002665, -141.7109808024215170 ) ) ;
#1251=CARTESIAN_POINT ( 'NONE',  ( -3.500000000000002220, 15.47927405783632793, -84.57139747004410424 ) ) ;
#1252=CARTESIAN_POINT ( 'NONE',  ( 1.655278471875001101, 20.36702641396248836, -72.18493913623279923 ) ) ;
#1254=CARTESIAN_POINT ( 'NONE',  ( -3.500000000000002220, 15.47927405783633503, -111.5713974700441042 ) ) ;
#1256=CARTESIAN_POINT ( 'NONE',  ( 0.000000000000000000, 21.00000000000002487, -149.5231586289125687 ) ) ;
#1257=CARTESIAN_POINT ( 'NONE',  ( 3.500000000000001776, 19.52072594216370760, -51.37764746908816704 ) ) ;
#1258=VECTOR ( 'NONE', #27166, 1000.000000000000000 ) ;
#1259=CARTESIAN_POINT ( 'NONE',  ( -0.9378221735089310451, 14.00000000000001066, -46.44938900211595012 ) ) ;
#1261=CARTESIAN_POINT ( 'NONE',  ( 0.9378221735089281585, 14.00000000000002132, -103.6663226036829855 ) ) ;
#1263=VERTEX_POINT ( 'NONE', #12921 ) ;
#1264=CARTESIAN_POINT ( 'NONE',  ( 3.500000000000001332, 17.50000000000001066, -43.15473080337743284 ) ) ;
#1266=ADVANCED_FACE ( 'NONE', ( #9741 ), #6543, .T. ) ;
#1267=CARTESIAN_POINT ( 'NONE',  ( 3.310556943749999981, 15.58864905735836004, -24.43493913623280633 ) ) ;
#1269=CARTESIAN_POINT ( 'NONE',  ( -0.9378221735089310451, 14.00000000000002132, -90.44938900211595012 ) ) ;
#1272=CARTESIAN_POINT ( 'NONE',  ( -1.655278471874999990, 20.36702641396249192, -76.93077246956615056 ) ) ;
#1275=CARTESIAN_POINT ( 'NONE',  ( -3.500000000000000000, 19.52072594216370760, -54.73806413671076143 ) ) ;
#1276=EDGE_LOOP ( 'NONE', ( #19469, #40505, #2270, #9866 ) ) ;
#1278=CARTESIAN_POINT ( 'NONE',  ( -0.9378221735089291577, 21.00000000000002132, -120.8600726046389013 ) ) ;
#1279=CARTESIAN_POINT ( 'NONE',  ( -1.655278471875002211, 14.63297358603754716, -86.59743913623280775 ) ) ;
#1280=ORIENTED_EDGE ( 'NONE', *, *, #4389, .T. ) ;
#1281=ORIENTED_EDGE ( 'NONE', *, *, #19694, .F. ) ;
#1284=CARTESIAN_POINT ( 'NONE',  ( 4.648177544792955347E-16, 21.00000000000001066, -41.90473080337742573 ) ) ;
#1286=CARTESIAN_POINT ( 'NONE',  ( 3.310556943750001313, 17.50000000000002132, -126.2641058028994792 ) ) ;
#1287=DIRECTION ( 'NONE',  ( 0.000000000000000000, -1.000000000000000000, -1.259100132267607459E-16 ) ) ;
#1288=CARTESIAN_POINT ( 'NONE',  ( -3.310556943750000425, 19.41135094264166128, -55.93493913623279212 ) ) ;
#1289=CARTESIAN_POINT ( 'NONE',  ( 2.340729813953370519E-16, 21.32270188528331900, -112.1016058028994706 ) ) ;
#1290=EDGE_LOOP ( 'NONE', ( #1483, #38521, #40780, #14470 ) ) ;
#1291=CARTESIAN_POINT ( 'NONE',  ( -3.500000000000001332, 17.50000000000002132, -125.6547308033774470 ) ) ;
#1292=CARTESIAN_POINT ( 'NONE',  ( 1.655278471874998436, 14.63297358603753828, -39.43077246956613635 ) ) ;
#1293=CARTESIAN_POINT ( 'NONE',  ( 3.310556943750001313, 19.41135094264166128, -67.26827246956612782 ) ) ;
#1294=CARTESIAN_POINT ( 'NONE',  ( -3.500000000000002220, 15.47927405783633503, -109.8776474690881884 ) ) ;
#1295=CARTESIAN_POINT ( 'NONE',  ( 3.310556943750001313, 19.41135094264166483, -99.18077246956613635 ) ) ;
#1298=CARTESIAN_POINT ( 'NONE',  ( -3.500000000000000000, 19.52072594216370760, -70.73806413671076143 ) ) ;
#1300=CARTESIAN_POINT ( 'NONE',  ( 1.750000000000001110, 20.53108891324555074, -70.29431413575484555 ) ) ;
#1301=CARTESIAN_POINT ( 'NONE',  ( -3.500000000000000000, 19.52072594216370405, -44.04431413575483845 ) ) ;
#1302=CARTESIAN_POINT ( 'NONE',  ( 3.310556943750001313, 17.50000000000001066, -34.26410580289947205 ) ) ;
#1303=CARTESIAN_POINT ( 'NONE',  ( 1.655278471875001101, 20.36702641396249192, -90.18493913623279923 ) ) ;
#1304=CARTESIAN_POINT ( 'NONE',  ( 2.474675557024783212E-16, 21.54145188432739388, -57.90473080337743994 ) ) ;
#1305=CARTESIAN_POINT ( 'NONE',  ( 3.500000000000001332, 17.50000000000001776, -92.46098080242151696 ) ) ;
#1306=CARTESIAN_POINT ( 'NONE',  ( 2.340729813953370519E-16, 21.32270188528331900, -114.1016058028994706 ) ) ;
#1307=CARTESIAN_POINT ( 'NONE',  ( -1.655278471875002211, 14.63297358603754184, -41.68493913623279212 ) ) ;
#1313=CARTESIAN_POINT ( 'NONE',  ( 0.9378221735089300459, 21.00000000000001421, -61.25563900116002714 ) ) ;
#1314=CARTESIAN_POINT ( 'NONE',  ( 1.655278471875001101, 20.36702641396249192, -93.09743913623280775 ) ) ;
#1321=( BOUNDED_CURVE ( )  B_SPLINE_CURVE ( 2, ( #19059, #324, #13303, #9489, #9919, #19478, #6707, #35433, #32029 ),
 .UNSPECIFIED., .F., .F. ) 
 B_SPLINE_CURVE_WITH_KNOTS ( ( 3, 2, 2, 2, 3 ),
 ( 0.8520833333333333037, 0.8527777777777777457, 0.8541666666666666297, 0.8555555555555555136, 0.8562499999999999556 ),
 .UNSPECIFIED. ) 
 CURVE ( )  GEOMETRIC_REPRESENTATION_ITEM ( )  RATIONAL_B_SPLINE_CURVE ( ( 0.9330127018922194093, 0.9330127018922194093, 1.000000000000000000, 0.8660254037844387076, 1.000000000000000000, 0.8660254037844387076, 1.000000000000000000, 0.9330127018922194093, 0.9330127018922194093 ) ) 
 REPRESENTATION_ITEM ( '' )  );
#1322=CARTESIAN_POINT ( 'NONE',  ( -1.394453263437886604E-15, 14.00000000000001421, -78.71098080242148853 ) ) ;
#1325=EDGE_CURVE ( 'NONE', #18479, #10589, #1930, .T. ) ;
#1328=CARTESIAN_POINT ( 'NONE',  ( 0.9378221735089281585, 14.00000000000001776, -82.36007260463891555 ) ) ;
#1329=VECTOR ( 'NONE', #6784, 1000.000000000000000 ) ;
#1334=CARTESIAN_POINT ( 'NONE',  ( 1.743066579297357930E-14, 14.00000000000002132, -135.4047308033774186 ) ) ;
#1336=CARTESIAN_POINT ( 'NONE',  ( -3.310556943750002645, 15.58864905735837958, -140.6807724695661364 ) ) ;
#1337=CARTESIAN_POINT ( 'NONE',  ( -1.394453263437886604E-15, 14.00000000000001776, -100.4047308033774328 ) ) ;
#1338=DIRECTION ( 'NONE',  ( 0.000000000000000000, 1.000000000000000000, 0.000000000000000000 ) ) ;
#1339=CARTESIAN_POINT ( 'NONE',  ( -3.310556943750001313, 17.50000000000002487, -130.8516058028994564 ) ) ;
#1340=CARTESIAN_POINT ( 'NONE',  ( 2.340729813953370519E-16, 21.32270188528330834, -55.10160580289946353 ) ) ;
#1343=CARTESIAN_POINT ( 'NONE',  ( -7.424026671074350129E-16, 13.45854811567264164, -139.4047308033774186 ) ) ;
#1344=CARTESIAN_POINT ( 'NONE',  ( 4.648177544792955347E-16, 21.00000000000001066, -36.90473080337743284 ) ) ;
#1346=CARTESIAN_POINT ( 'NONE',  ( 3.500000000000001332, 17.50000000000002487, -132.4609808024214885 ) ) ;
#1347=CARTESIAN_POINT ( 'NONE',  ( 3.310556943749999981, 15.58864905735837247, -114.3474391362328078 ) ) ;
#1350=CARTESIAN_POINT ( 'NONE',  ( 2.474675557024783212E-16, 21.54145188432739744, -88.21098080242151696 ) ) ;
#1352=CARTESIAN_POINT ( 'NONE',  ( -1.655278471874999990, 20.36702641396248481, -45.93077246956614346 ) ) ;
#1353=CARTESIAN_POINT ( 'NONE',  ( 3.310556943749999981, 15.58864905735837070, -108.4349391362327850 ) ) ;
#1354=CARTESIAN_POINT ( 'NONE',  ( 0.9378221735089281585, 14.00000000000002132, -111.3600726046389013 ) ) ;
#1357=CARTESIAN_POINT ( 'NONE',  ( -1.655278471875002211, 14.63297358603755249, -127.6849391362327992 ) ) ;
#1360=CARTESIAN_POINT ( 'NONE',  ( 1.750000000000001110, 20.53108891324554719, -27.29431413575483845 ) ) ;
#1362=CARTESIAN_POINT ( 'NONE',  ( -7.022189441860112050E-16, 13.67729811471671830, -59.60160580289947063 ) ) ;
#1365=CARTESIAN_POINT ( 'NONE',  ( 1.655278471875001101, 20.36702641396249192, -80.18493913623279923 ) ) ;
#1370=CARTESIAN_POINT ( 'NONE',  ( -1.655278471875002211, 14.63297358603754006, -38.59743913623281486 ) ) ;
#1371=CARTESIAN_POINT ( 'NONE',  ( -3.310556943750001313, 17.50000000000001776, -101.7641058028994792 ) ) ;
#1374=EDGE_LOOP ( 'NONE', ( #38526, #20793, #39327, #32437 ) ) ;
#1376=CARTESIAN_POINT ( 'NONE',  ( -7.022189441860112050E-16, 13.67729811471671830, -54.51410580289947205 ) ) ;
#1377=ORIENTED_EDGE ( 'NONE', *, *, #12387, .F. ) ;
#1379=CARTESIAN_POINT ( 'NONE',  ( 1.749999999999998224, 14.46891108675448123, -93.62764746908815994 ) ) ;
#1381=CARTESIAN_POINT ( 'NONE',  ( -3.500000000000002220, 15.47927405783632970, -91.57139747004410424 ) ) ;
#1387=CARTESIAN_POINT ( 'NONE',  ( 3.500000000000000000, 15.47927405783632082, -42.54431413575484555 ) ) ;
#1388=( BOUNDED_CURVE ( )  B_SPLINE_CURVE ( 2, ( #34011, #4863, #21447, #11654, #24652, #37613, #2301, #15289, #31644 ),
 .UNSPECIFIED., .F., .T. ) 
 B_SPLINE_CURVE_WITH_KNOTS ( ( 3, 2, 2, 2, 3 ),
 ( 0.8812499999999999778, 0.8819444444444444198, 0.8833333333333333037, 0.8847222222222221877, 0.8854166666666666297 ),
 .UNSPECIFIED. ) 
 CURVE ( )  GEOMETRIC_REPRESENTATION_ITEM ( )  RATIONAL_B_SPLINE_CURVE ( ( 0.9330127018922194093, 0.9330127018922194093, 1.000000000000000000, 0.8660254037844387076, 1.000000000000000000, 0.8660254037844387076, 1.000000000000000000, 0.9330127018922194093, 0.9330127018922194093 ) ) 
 REPRESENTATION_ITEM ( '' )  );
#1389=LINE ( 'NONE', #17349, #14634 ) ;
#1390=CARTESIAN_POINT ( 'NONE',  ( 0.9378221735089300459, 21.00000000000002132, -118.9493890021159501 ) ) ;
#1392=CARTESIAN_POINT ( 'NONE',  ( 3.310556943750001313, 19.41135094264165772, -30.26827246956613493 ) ) ;
#1393=CARTESIAN_POINT ( 'NONE',  ( 0.9378221735089300459, 21.00000000000002132, -121.9493890021159501 ) ) ;
#1394=CARTESIAN_POINT ( 'NONE',  ( -1.655278471874999990, 20.36702641396249192, -81.01827246956614204 ) ) ;
#1395=CARTESIAN_POINT ( 'NONE',  ( -1.655278471874999990, 20.36702641396249902, -134.9307724695661364 ) ) ;
#1398=CARTESIAN_POINT ( 'NONE',  ( -3.500000000000000000, 19.52072594216370405, -38.73806413671076143 ) ) ;
#1400=CARTESIAN_POINT ( 'NONE',  ( 1.655278471874998436, 14.63297358603755072, -124.5182724695661278 ) ) ;
#1402=CARTESIAN_POINT ( 'NONE',  ( 2.340729813953370519E-16, 21.32270188528331190, -88.01410580289947916 ) ) ;
#1403=CARTESIAN_POINT ( 'NONE',  ( 3.500000000000001332, 17.50000000000001066, -46.15473080337742573 ) ) ;
#1405=CARTESIAN_POINT ( 'NONE',  ( -3.500000000000000888, 19.52072594216370760, -69.73806413671076143 ) ) ;
#1406=ADVANCED_FACE ( 'NONE', ( #25798 ), #16028, .T. ) ;
#1407=CARTESIAN_POINT ( 'NONE',  ( -7.022189441860112050E-16, 13.67729811471672186, -54.60160580289946353 ) ) ;
#1411=CARTESIAN_POINT ( 'NONE',  ( 3.310556943750001313, 17.50000000000001776, -82.35160580289945642 ) ) ;
#1412=CARTESIAN_POINT ( 'NONE',  ( 3.310556943749999981, 15.58864905735837780, -140.4349391362327992 ) ) ;
#1414=CARTESIAN_POINT ( 'NONE',  ( -3.310556943750002201, 15.58864905735837425, -103.6807724695661364 ) ) ;
#1415=CARTESIAN_POINT ( 'NONE',  ( 1.655278471875001101, 20.36702641396249192, -76.09743913623280775 ) ) ;
#1416=CARTESIAN_POINT ( 'NONE',  ( -1.750000000000002220, 14.46891108675448656, -115.4880641367107614 ) ) ;
#1419=CARTESIAN_POINT ( 'NONE',  ( 1.655278471875001101, 20.36702641396249192, -96.18493913623279923 ) ) ;
#1421=CARTESIAN_POINT ( 'NONE',  ( 3.500000000000000000, 15.47927405783632793, -91.54431413575483134 ) ) ;
#1422=LINE ( 'NONE', #40344, #4371 ) ;
#1424=CARTESIAN_POINT ( 'NONE',  ( -1.655278471875002211, 14.63297358603754361, -55.59743913623280065 ) ) ;
#1425=CARTESIAN_POINT ( 'NONE',  ( -0.9378221735089310451, 14.00000000000001599, -68.44938900211596433 ) ) ;
#1426=CARTESIAN_POINT ( 'NONE',  ( -1.655278471875002211, 14.63297358603755072, -117.5974391362328078 ) ) ;
#1433=CARTESIAN_POINT ( 'NONE',  ( 2.340729813953370519E-16, 21.32270188528330834, -67.01410580289947916 ) ) ;
#1434=ORIENTED_EDGE ( 'NONE', *, *, #32747, .F. ) ;
#1435=VERTEX_POINT ( 'NONE', #32783 ) ;
#1436=EDGE_CURVE ( 'NONE', #9822, #11775, #29623, .T. ) ;
#1438=CARTESIAN_POINT ( 'NONE',  ( -3.500000000000000000, 19.52072594216371826, -131.0443141357548598 ) ) ;
#1440=EDGE_CURVE ( 'NONE', #13926, #18853, #20038, .T. ) ;
#1443=ORIENTED_EDGE ( 'NONE', *, *, #17415, .F. ) ;
#1445=FACE_OUTER_BOUND ( 'NONE', #12256, .T. ) ;
#1446=CARTESIAN_POINT ( 'NONE',  ( -3.310556943750001313, 17.50000000000002487, -133.7641058028994507 ) ) ;
#1447=CARTESIAN_POINT ( 'NONE',  ( 4.648177544792955347E-16, 21.00000000000001421, -62.90473080337742573 ) ) ;
#1448=( BOUNDED_CURVE ( )  B_SPLINE_CURVE ( 2, ( #17430, #14229, #20189, #26787, #833, #23160, #16582, #1259, #27207 ),
 .UNSPECIFIED., .F., .T. ) 
 B_SPLINE_CURVE_WITH_KNOTS ( ( 3, 2, 2, 2, 3 ),
 ( 0.8020833333333333703, 0.8027777777777778123, 0.8041666666666666963, 0.8055555555555555802, 0.8062500000000000222 ),
 .UNSPECIFIED. ) 
 CURVE ( )  GEOMETRIC_REPRESENTATION_ITEM ( )  RATIONAL_B_SPLINE_CURVE ( ( 0.9330127018922194093, 0.9330127018922194093, 1.000000000000000000, 0.8660254037844387076, 1.000000000000000000, 0.8660254037844387076, 1.000000000000000000, 0.9330127018922194093, 0.9330127018922194093 ) ) 
 REPRESENTATION_ITEM ( '' )  );
#1450=CARTESIAN_POINT ( 'NONE',  ( 1.749999999999998224, 14.46891108675448301, -96.62764746908817415 ) ) ;
#1451=CARTESIAN_POINT ( 'NONE',  ( -1.655278471875002211, 14.63297358603754006, -33.68493913623279923 ) ) ;
#1452=CARTESIAN_POINT ( 'NONE',  ( 1.655278471874998436, 14.63297358603754716, -97.51827246956612782 ) ) ;
#1454=CARTESIAN_POINT ( 'NONE',  ( 3.310556943749999981, 15.58864905735837780, -141.4349391362327992 ) ) ;
#1455=CARTESIAN_POINT ( 'NONE',  ( 0.000000000000000000, 17.50000000000002487, -149.5231586289125687 ) ) ;
#1456=CARTESIAN_POINT ( 'NONE',  ( -3.500000000000002220, 15.47927405783632793, -93.87764746908817415 ) ) ;
#1459=CARTESIAN_POINT ( 'NONE',  ( 1.750000000000001110, 20.53108891324555429, -85.98806413671076143 ) ) ;
#1460=CARTESIAN_POINT ( 'NONE',  ( -1.655278471875002211, 14.63297358603754539, -69.68493913623279923 ) ) ;
#1465=CARTESIAN_POINT ( 'NONE',  ( 3.500000000000001332, 17.50000000000001421, -48.46098080242150274 ) ) ;
#1466=CARTESIAN_POINT ( 'NONE',  ( -3.310556943750001313, 17.50000000000002132, -117.7641058028994792 ) ) ;
#1467=CARTESIAN_POINT ( 'NONE',  ( -1.750000000000002220, 14.46891108675448123, -79.48806413671076143 ) ) ;
#1469=EDGE_CURVE ( 'NONE', #36297, #19989, #16640, .T. ) ;
#1470=CARTESIAN_POINT ( 'NONE',  ( -7.424026671074350129E-16, 13.45854811567263987, -114.4047308033774328 ) ) ;
#1471=CARTESIAN_POINT ( 'NONE',  ( 4.286263797015737581E-16, 14.00000000000002487, -149.5231586289125687 ) ) ;
#1473=DIRECTION ( 'NONE',  ( -0.000000000000000000, 1.259100132267607459E-16, -1.000000000000000000 ) ) ;
#1476=CARTESIAN_POINT ( 'NONE',  ( -3.310556943750000425, 19.41135094264166838, -77.84743913623280775 ) ) ;
#1477=CARTESIAN_POINT ( 'NONE',  ( -3.500000000000001332, 17.50000000000001776, -96.96098080242150274 ) ) ;
#1478=VECTOR ( 'NONE', #38060, 1000.000000000000000 ) ;
#1481=CARTESIAN_POINT ( 'NONE',  ( -3.500000000000002220, 15.47927405783632615, -63.87764746908818125 ) ) ;
#1482=CARTESIAN_POINT ( 'NONE',  ( 2.340729813953370519E-16, 21.32270188528331190, -86.01410580289946495 ) ) ;
#1483=ORIENTED_EDGE ( 'NONE', *, *, #41454, .F. ) ;
#1484=ORIENTED_EDGE ( 'NONE', *, *, #476, .F. ) ;
#1488=EDGE_CURVE ( 'NONE', #4210, #9158, #9523, .T. ) ;
#1491=CARTESIAN_POINT ( 'NONE',  ( -1.655278471875002211, 14.63297358603754184, -46.68493913623279923 ) ) ;
#1492=CARTESIAN_POINT ( 'NONE',  ( -7.022189441860112050E-16, 13.67729811471672718, -115.6016058028994706 ) ) ;
#1494=CARTESIAN_POINT ( 'NONE',  ( -3.500000000000000888, 19.52072594216371826, -122.7380641367107472 ) ) ;
#1496=CARTESIAN_POINT ( 'NONE',  ( 3.310556943750001313, 19.41135094264165772, -39.18077246956613635 ) ) ;
#1497=CARTESIAN_POINT ( 'NONE',  ( -7.022189441860112050E-16, 13.67729811471671830, -64.60160580289945642 ) ) ;
#1498=CARTESIAN_POINT ( 'NONE',  ( -1.749999999999999778, 20.53108891324555785, -115.1276474690881741 ) ) ;
#1500=CARTESIAN_POINT ( 'NONE',  ( -3.310556943750000425, 19.41135094264166483, -97.84743913623280775 ) ) ;
#1502=CARTESIAN_POINT ( 'NONE',  ( 1.750000000000001110, 20.53108891324555429, -97.98806413671076143 ) ) ;
#1503=CARTESIAN_POINT ( 'NONE',  ( 3.500000000000001332, 19.52072594216370760, -52.07139747004409003 ) ) ;
#1504=DIRECTION ( 'NONE',  ( -0.000000000000000000, 1.259100132267607459E-16, -1.000000000000000000 ) ) ;
#1506=CARTESIAN_POINT ( 'NONE',  ( 1.749999999999998224, 14.46891108675447768, -63.62764746908818125 ) ) ;
#1507=LINE ( 'NONE', #17259, #3358 ) ;
#1508=CARTESIAN_POINT ( 'NONE',  ( 3.310556943750001313, 17.50000000000001066, -30.26410580289948271 ) ) ;
#1509=CARTESIAN_POINT ( 'NONE',  ( -1.655278471875002211, 14.63297358603754716, -92.68493913623279923 ) ) ;
#1510=EDGE_CURVE ( 'NONE', #27884, #36364, #13866, .T. ) ;
#1511=CARTESIAN_POINT ( 'NONE',  ( 2.474675557024783212E-16, 21.54145188432739388, -51.90473080337743284 ) ) ;
#1512=CARTESIAN_POINT ( 'NONE',  ( -1.394453263437886604E-15, 14.00000000000001066, -52.71098080242150985 ) ) ;
#1513=CARTESIAN_POINT ( 'NONE',  ( -1.655278471874999990, 20.36702641396249547, -115.0182724695661278 ) ) ;
#1514=CARTESIAN_POINT ( 'NONE',  ( -1.655278471874999990, 20.36702641396248481, -39.01827246956612782 ) ) ;
#1521=CARTESIAN_POINT ( 'NONE',  ( -1.750000000000002220, 14.46891108675447413, -23.48806413671077209 ) ) ;
#1522=CARTESIAN_POINT ( 'NONE',  ( -3.310556943750002201, 15.58864905735837247, -94.68077246956613635 ) ) ;
#1525=EDGE_LOOP ( 'NONE', ( #8854, #431, #2531, #34189 ) ) ;
#1528=DIRECTION ( 'NONE',  ( 0.000000000000000000, 1.000000000000000000, 0.000000000000000000 ) ) ;
#1529=EDGE_LOOP ( 'NONE', ( #2417, #3619, #29274, #32745, #21102, #899, #4712, #40188, #12265, #40994, #6077, #27593, #21932, #33226, #12987, #1928, #25087, #26603, #19155, #34796, #27274, #13183, #35526, #21564, #42035, #14250, #2886, #21927, #8849, #41493, #13606, #27586, #803, #6704, #32737, #24872, #17801, #32961, #5543, #34166, #40340, #9667, #33657, #8234, #31139, #30285, #41122, #20169, #30301, #12499, #35838, #22782, #39938, #40557, #28111, #39486, #31284, #33334, #37692, #15891, #28200, #35311, #35124, #12037, #27930, #7550, #37156, #34273, #33776, #16183, #11618, #13717, #39641, #26910, #41381, #4253, #33716, #7876, #29121, #4566, #29861, #30568, #15566, #9008, #22022, #23932, #26277, #26587, #25652, #1085, #33283, #33825, #38777, #34326, #15189, #110, #22484, #15756, #19733, #23570, #5332, #19888, #8331, #7374, #11221, #3196, #22346, #35307, #11215, #8173, #1031, #2635, #17712, #26951, #35215, #22777, #26267, #2048, #18064, #8489, #14194, #17018, #4015, #34794, #11564, #24833, #32023, #970, #18529, #27903, #12043, #4716, #33610, #26976, #18847, #24755, #19831, #8376, #23785, #9369, #32222, #17604, #32352, #14141, #29658, #4046, #20364, #34677, #15226, #31037, #38603, #23758, #39089, #30453, #4357, #22764, #39926, #16905, #28346, #14246, #34686, #15147, #29778, #3160, #30627, #15885, #41022, #37117, #5483, #9645, #674, #18251, #23506, #382, #38561, #41028, #2519, #26646, #24882, #14409, #21919, #3655, #27628, #27070, #27550, #27283, #18127, #34492, #39754, #26429, #40861, #35120, #25044, #3625, #15492, #26282, #31859, #25513, #20893, #17247, #10167, #11890, #11619, #25235, #41647, #16864, #30601, #8947, #34165, #4885, #27122, #47, #34693, #35695, #41934, #6843, #9916, #9742, #20628, #28148, #21656, #10433, #31665, #11879, #24086, #26850, #11843, #21509, #28446, #8316, #3442, #36102, #29449, #31220, #41011, #588, #15264, #32586, #38511, #30253, #24911, #18894, #25336, #32968 ) ) ;
#1538=ORIENTED_EDGE ( 'NONE', *, *, #12855, .T. ) ;
#1539=CARTESIAN_POINT ( 'NONE',  ( 0.000000000000000000, 17.50000000000002487, -149.5231586289125687 ) ) ;
#1540=CARTESIAN_POINT ( 'NONE',  ( -3.310556943750001313, 17.50000000000002487, -141.7641058028994792 ) ) ;
#1541=VECTOR ( 'NONE', #19945, 1000.000000000000000 ) ;
#1544=VECTOR ( 'NONE', #14822, 1000.000000000000000 ) ;
#1545=CARTESIAN_POINT ( 'NONE',  ( -1.749999999999999778, 20.53108891324554719, -26.82139747004409713 ) ) ;
#1546=CARTESIAN_POINT ( 'NONE',  ( 3.310556943750001313, 17.50000000000002487, -130.3516058028994564 ) ) ;
#1547=CARTESIAN_POINT ( 'NONE',  ( -1.655278471875002211, 14.63297358603754361, -56.68493913623279212 ) ) ;
#1551=CARTESIAN_POINT ( 'NONE',  ( 3.500000000000001776, 19.52072594216372181, -142.0713974700441042 ) ) ;
#1554=CARTESIAN_POINT ( 'NONE',  ( 1.749999999999998224, 14.46891108675448656, -127.6276474690881741 ) ) ;
#1555=CARTESIAN_POINT ( 'NONE',  ( -3.310556943750002645, 15.58864905735837780, -111.6807724695661506 ) ) ;
#1558=CARTESIAN_POINT ( 'NONE',  ( 3.500000000000000000, 15.47927405783633503, -128.5443141357548313 ) ) ;
#1559=CARTESIAN_POINT ( 'NONE',  ( 2.474675557024783212E-16, 21.54145188432739744, -86.21098080242151696 ) ) ;
#1560=( BOUNDED_CURVE ( )  B_SPLINE_CURVE ( 2, ( #31557, #18801, #28366, #24563, #2427, #37526, #35167, #1799, #31761 ),
 .UNSPECIFIED., .F., .F. ) 
 B_SPLINE_CURVE_WITH_KNOTS ( ( 3, 2, 2, 2, 3 ),
 ( 0.3187499999999999778, 0.3194444444444444198, 0.3208333333333333592, 0.3222222222222222432, 0.3229166666666666852 ),
 .UNSPECIFIED. ) 
 CURVE ( )  GEOMETRIC_REPRESENTATION_ITEM ( )  RATIONAL_B_SPLINE_CURVE ( ( 0.9330127018922194093, 0.9330127018922194093, 1.000000000000000000, 0.8660254037844387076, 1.000000000000000000, 0.8660254037844387076, 1.000000000000000000, 0.9330127018922194093, 0.9330127018922194093 ) ) 
 REPRESENTATION_ITEM ( '' )  );
#1561=CARTESIAN_POINT ( 'NONE',  ( -1.836030130193217234E-14, 21.00000000000002132, -128.9047308033774470 ) ) ;
#1562=CARTESIAN_POINT ( 'NONE',  ( 3.310556943750001313, 19.41135094264166128, -47.18077246956614346 ) ) ;
#1563=CARTESIAN_POINT ( 'NONE',  ( -7.022189441860112050E-16, 13.67729811471672541, -106.6016058028994564 ) ) ;
#1564=( BOUNDED_CURVE ( )  B_SPLINE_CURVE ( 2, ( #19063, #32033, #25242, #37792, #31616, #2900, #15892, #28420, #8438 ),
 .UNSPECIFIED., .F., .T. ) 
 B_SPLINE_CURVE_WITH_KNOTS ( ( 3, 2, 2, 2, 3 ),
 ( 0.7354166666666667185, 0.7361111111111111605, 0.7375000000000000444, 0.7388888888888889284, 0.7395833333333333703 ),
 .UNSPECIFIED. ) 
 CURVE ( )  GEOMETRIC_REPRESENTATION_ITEM ( )  RATIONAL_B_SPLINE_CURVE ( ( 0.9330127018922194093, 0.9330127018922194093, 1.000000000000000000, 0.8660254037844387076, 1.000000000000000000, 0.8660254037844387076, 1.000000000000000000, 0.9330127018922194093, 0.9330127018922194093 ) ) 
 REPRESENTATION_ITEM ( '' )  );
#1565=CARTESIAN_POINT ( 'NONE',  ( -1.749999999999999778, 20.53108891324556140, -130.1276474690881741 ) ) ;
#1566=DIRECTION ( 'NONE',  ( -0.000000000000000000, 1.259100132267607459E-16, -1.000000000000000000 ) ) ;
#1568=DIRECTION ( 'NONE',  ( -0.000000000000000000, 1.259100132267607459E-16, -1.000000000000000000 ) ) ;
#1569=CARTESIAN_POINT ( 'NONE',  ( 2.340729813953370519E-16, 21.32270188528331900, -126.1016058028994706 ) ) ;
#1572=CARTESIAN_POINT ( 'NONE',  ( 0.9378221735089300459, 21.00000000000001776, -82.94938900211595012 ) ) ;
#1573=LINE ( 'NONE', #40280, #17675 ) ;
#1574=CARTESIAN_POINT ( 'NONE',  ( 3.310556943750001313, 19.41135094264166128, -61.26827246956612782 ) ) ;
#1576=CARTESIAN_POINT ( 'NONE',  ( 1.655278471875001101, 20.36702641396249192, -78.18493913623279923 ) ) ;
#1579=CARTESIAN_POINT ( 'NONE',  ( 0.9378221735089281585, 14.00000000000000888, -26.36007260463891555 ) ) ;
#1582=CARTESIAN_POINT ( 'NONE',  ( 2.340729813953370519E-16, 21.32270188528330834, -40.01410580289947916 ) ) ;
#1583=CARTESIAN_POINT ( 'NONE',  ( -3.310556943750002645, 15.58864905735837247, -92.68077246956613635 ) ) ;
#1588=CARTESIAN_POINT ( 'NONE',  ( 1.655278471875001101, 20.36702641396248836, -53.09743913623281486 ) ) ;
#1589=ORIENTED_EDGE ( 'NONE', *, *, #40242, .F. ) ;
#1594=DIRECTION ( 'NONE',  ( -0.000000000000000000, 1.259100132267607459E-16, -1.000000000000000000 ) ) ;
#1595=VERTEX_POINT ( 'NONE', #39166 ) ;
#1596=CARTESIAN_POINT ( 'NONE',  ( 3.500000000000001332, 17.50000000000001066, -43.46098080242151696 ) ) ;
#1597=CARTESIAN_POINT ( 'NONE',  ( 3.500000000000001332, 17.50000000000001066, -37.46098080242150985 ) ) ;
#1599=CARTESIAN_POINT ( 'NONE',  ( -3.500000000000000000, 19.52072594216371826, -110.7380641367107472 ) ) ;
#1601=CARTESIAN_POINT ( 'NONE',  ( 3.310556943750001313, 19.41135094264165772, -26.26827246956613138 ) ) ;
#1602=CARTESIAN_POINT ( 'NONE',  ( -3.500000000000001332, 17.50000000000002132, -106.6547308033774186 ) ) ;
#1603=CARTESIAN_POINT ( 'NONE',  ( 1.655278471875001101, 20.36702641396249547, -127.0974391362328078 ) ) ;
#1607=CARTESIAN_POINT ( 'NONE',  ( -0.9378221735089291577, 21.00000000000001066, -38.86007260463890844 ) ) ;
#1608=CARTESIAN_POINT ( 'NONE',  ( 3.310556943750001313, 17.50000000000002132, -124.3516058028994564 ) ) ;
#1610=CARTESIAN_POINT ( 'NONE',  ( -7.424026671074350129E-16, 13.45854811567263098, -39.40473080337742573 ) ) ;
#1614=CARTESIAN_POINT ( 'NONE',  ( 3.310556943750001313, 17.50000000000002487, -142.3516058028994564 ) ) ;
#1615=CARTESIAN_POINT ( 'NONE',  ( -1.750000000000002220, 14.46891108675448123, -68.48806413671077564 ) ) ;
#1616=CARTESIAN_POINT ( 'NONE',  ( 1.655278471875001101, 20.36702641396248836, -55.18493913623280633 ) ) ;
#1618=DIRECTION ( 'NONE',  ( -0.000000000000000000, 1.259100132267607459E-16, -1.000000000000000000 ) ) ;
#1619=CARTESIAN_POINT ( 'NONE',  ( -7.022189441860112050E-16, 13.67729811471672186, -75.60160580289944221 ) ) ;
#1621=CARTESIAN_POINT ( 'NONE',  ( 1.655278471874998436, 14.63297358603754716, -105.4307724695661364 ) ) ;
#1622=CARTESIAN_POINT ( 'NONE',  ( 1.655278471875001101, 20.36702641396249192, -77.09743913623280775 ) ) ;
#1624=CARTESIAN_POINT ( 'NONE',  ( -1.655278471874999990, 20.36702641396249192, -96.01827246956612782 ) ) ;
#1627=DIRECTION ( 'NONE',  ( -0.000000000000000000, 1.259100132267607459E-16, -1.000000000000000000 ) ) ;
#1628=CARTESIAN_POINT ( 'NONE',  ( -1.655278471874999990, 20.36702641396248836, -55.93077246956613635 ) ) ;
#1630=CARTESIAN_POINT ( 'NONE',  ( -3.310556943750001313, 17.50000000000002132, -114.7641058028994792 ) ) ;
#1635=ORIENTED_EDGE ( 'NONE', *, *, #33469, .F. ) ;
#1636=CARTESIAN_POINT ( 'NONE',  ( -1.394453263437886604E-15, 14.00000000000001066, -33.71098080242150985 ) ) ;
#1637=CARTESIAN_POINT ( 'NONE',  ( 3.310556943749999981, 15.58864905735836714, -69.34743913623282197 ) ) ;
#1638=( BOUNDED_CURVE ( )  B_SPLINE_CURVE ( 2, ( #1854, #11627, #37586, #8440, #40151, #14632, #7835, #11019, #34184 ),
 .UNSPECIFIED., .F., .F. ) 
 B_SPLINE_CURVE_WITH_KNOTS ( ( 3, 2, 2, 2, 3 ),
 ( 0.2270833333333333315, 0.2277777777777777735, 0.2291666666666666574, 0.2305555555555555691, 0.2312500000000000111 ),
 .UNSPECIFIED. ) 
 CURVE ( )  GEOMETRIC_REPRESENTATION_ITEM ( )  RATIONAL_B_SPLINE_CURVE ( ( 0.9330127018922194093, 0.9330127018922194093, 1.000000000000000000, 0.8660254037844387076, 1.000000000000000000, 0.8660254037844387076, 1.000000000000000000, 0.9330127018922194093, 0.9330127018922194093 ) ) 
 REPRESENTATION_ITEM ( '' )  );
#1639=ORIENTED_EDGE ( 'NONE', *, *, #3802, .T. ) ;
#1640=ORIENTED_EDGE ( 'NONE', *, *, #39167, .F. ) ;
#1641=CARTESIAN_POINT ( 'NONE',  ( -1.394453263437886604E-15, 14.00000000000001066, -32.71098080242150274 ) ) ;
#1648=CARTESIAN_POINT ( 'NONE',  ( -7.022189441860112050E-16, 13.67729811471672896, -129.5141058028994507 ) ) ;
#1649=CARTESIAN_POINT ( 'NONE',  ( 3.500000000000000000, 15.47927405783633326, -119.5443141357548313 ) ) ;
#1650=CARTESIAN_POINT ( 'NONE',  ( 3.310556943750001313, 17.50000000000001421, -47.35160580289946353 ) ) ;
#1651=CARTESIAN_POINT ( 'NONE',  ( 3.310556943749999981, 15.58864905735836182, -35.43493913623279923 ) ) ;
#1652=CARTESIAN_POINT ( 'NONE',  ( -1.655278471875002211, 14.63297358603754894, -95.68493913623279923 ) ) ;
#1653=CARTESIAN_POINT ( 'NONE',  ( 3.310556943750001313, 17.50000000000002487, -143.2641058028994792 ) ) ;
#1655=CARTESIAN_POINT ( 'NONE',  ( -3.310556943750002645, 15.58864905735837958, -140.7682724695661136 ) ) ;
#1657=DIRECTION ( 'NONE',  ( 0.000000000000000000, 1.000000000000000000, 0.000000000000000000 ) ) ;
#1658=CARTESIAN_POINT ( 'NONE',  ( -1.750000000000002220, 14.46891108675448478, -96.79431413575484555 ) ) ;
#1659=CARTESIAN_POINT ( 'NONE',  ( 3.500000000000001332, 19.52072594216371826, -132.3776474690881741 ) ) ;
#1661=CARTESIAN_POINT ( 'NONE',  ( 3.500000000000001776, 19.52072594216371115, -84.07139747004411845 ) ) ;
#1662=CARTESIAN_POINT ( 'NONE',  ( 1.655278471874998436, 14.63297358603754361, -71.51827246956612782 ) ) ;
#1665=ADVANCED_FACE ( 'NONE', ( #33429 ), #17692, .T. ) ;
#1668=CARTESIAN_POINT ( 'NONE',  ( 3.500000000000000000, 15.47927405783632082, -48.54431413575484555 ) ) ;
#1669=CARTESIAN_POINT ( 'NONE',  ( 3.310556943749999981, 15.58864905735837247, -119.3474391362328078 ) ) ;
#1670=CARTESIAN_POINT ( 'NONE',  ( 4.648177544792955347E-16, 21.00000000000001776, -79.90473080337741862 ) ) ;
#1671=CARTESIAN_POINT ( 'NONE',  ( 4.648177544792955347E-16, 21.00000000000001066, -35.21098080242151696 ) ) ;
#1674=CARTESIAN_POINT ( 'NONE',  ( 3.500000000000001332, 17.50000000000002132, -113.1547308033774328 ) ) ;
#1676=AXIS2_PLACEMENT_3D ( 'NONE', #31634, #34616, #2500 ) ;
#1677=CARTESIAN_POINT ( 'NONE',  ( 4.648177544792955347E-16, 21.00000000000001421, -47.90473080337742573 ) ) ;
#1681=CARTESIAN_POINT ( 'NONE',  ( -3.310556943750002201, 15.58864905735837070, -73.68077246956615056 ) ) ;
#1683=CARTESIAN_POINT ( 'NONE',  ( -1.394453263437886604E-15, 14.00000000000002132, -114.7109808024214885 ) ) ;
#1684=VERTEX_POINT ( 'NONE', #26846 ) ;
#1685=CARTESIAN_POINT ( 'NONE',  ( 4.648177544792955347E-16, 21.00000000000002487, -136.2109808024215170 ) ) ;
#1686=CARTESIAN_POINT ( 'NONE',  ( -1.655278471875002211, 14.63297358603754716, -84.59743913623279354 ) ) ;
#1687=ORIENTED_EDGE ( 'NONE', *, *, #40455, .F. ) ;
#1688=ORIENTED_EDGE ( 'NONE', *, *, #38166, .F. ) ;
#1689=( BOUNDED_CURVE ( )  B_SPLINE_CURVE ( 2, ( #2520, #5081, #18059, #24660, #15933, #25709, #39085, #13354, #22718 ),
 .UNSPECIFIED., .F., .F. ) 
 B_SPLINE_CURVE_WITH_KNOTS ( ( 3, 2, 2, 2, 3 ),
 ( 0.3270833333333333370, 0.3277777777777777790, 0.3291666666666666630, 0.3305555555555555469, 0.3312499999999999889 ),
 .UNSPECIFIED. ) 
 CURVE ( )  GEOMETRIC_REPRESENTATION_ITEM ( )  RATIONAL_B_SPLINE_CURVE ( ( 0.9330127018922194093, 0.9330127018922194093, 1.000000000000000000, 0.8660254037844387076, 1.000000000000000000, 0.8660254037844387076, 1.000000000000000000, 0.9330127018922194093, 0.9330127018922194093 ) ) 
 REPRESENTATION_ITEM ( '' )  );
#1690=VECTOR ( 'NONE', #19584, 1000.000000000000000 ) ;
#1692=EDGE_CURVE ( 'NONE', #16103, #14931, #2178, .T. ) ;
#1695=CARTESIAN_POINT ( 'NONE',  ( 1.749999999999998224, 14.46891108675448301, -102.6276474690881741 ) ) ;
#1697=ADVANCED_FACE ( 'NONE', ( #23876 ), #896, .T. ) ;
#1699=FACE_OUTER_BOUND ( 'NONE', #31204, .T. ) ;
#1700=CARTESIAN_POINT ( 'NONE',  ( -1.655278471874999990, 20.36702641396248836, -49.01827246956613493 ) ) ;
#1701=CARTESIAN_POINT ( 'NONE',  ( -7.022189441860112050E-16, 13.67729811471672718, -113.6016058028994564 ) ) ;
#1702=ORIENTED_EDGE ( 'NONE', *, *, #15434, .F. ) ;
#1703=CARTESIAN_POINT ( 'NONE',  ( 2.474675557024783212E-16, 21.54145188432740099, -121.9047308033774328 ) ) ;
#1704=CARTESIAN_POINT ( 'NONE',  ( 2.340729813953370519E-16, 21.32270188528330479, -32.01410580289947205 ) ) ;
#1705=CARTESIAN_POINT ( 'NONE',  ( 2.340729813953370519E-16, 21.32270188528330834, -65.10160580289947063 ) ) ;
#1706=CARTESIAN_POINT ( 'NONE',  ( 3.500000000000001776, 19.52072594216371826, -112.3776474690881741 ) ) ;
#1708=CARTESIAN_POINT ( 'NONE',  ( -3.310556943750002645, 15.58864905735837425, -97.68077246956613635 ) ) ;
#1710=CARTESIAN_POINT ( 'NONE',  ( 3.500000000000001332, 17.50000000000001776, -85.15473080337743284 ) ) ;
#1712=CARTESIAN_POINT ( 'NONE',  ( 1.750000000000001110, 20.53108891324555074, -64.29431413575484555 ) ) ;
#1713=CARTESIAN_POINT ( 'NONE',  ( -1.750000000000002220, 14.46891108675447768, -43.79431413575483845 ) ) ;
#1714=CARTESIAN_POINT ( 'NONE',  ( -3.310556943750002645, 15.58864905735836537, -33.68077246956615056 ) ) ;
#1715=CARTESIAN_POINT ( 'NONE',  ( 3.310556943750001313, 19.41135094264166483, -90.26827246956612782 ) ) ;
#1718=CARTESIAN_POINT ( 'NONE',  ( 3.500000000000001776, 19.52072594216370760, -54.07139747004409713 ) ) ;
#1719=CARTESIAN_POINT ( 'NONE',  ( -3.500000000000001332, 17.50000000000002487, -137.9609808024214885 ) ) ;
#1720=CARTESIAN_POINT ( 'NONE',  ( 3.310556943750001313, 19.41135094264166838, -105.2682724695661278 ) ) ;
#1721=CARTESIAN_POINT ( 'NONE',  ( 3.310556943750001313, 19.41135094264166128, -39.26827246956613493 ) ) ;
#1723=FACE_OUTER_BOUND ( 'NONE', #33866, .T. ) ;
#1729=CARTESIAN_POINT ( 'NONE',  ( -3.310556943750001313, 17.50000000000001776, -89.76410580289947916 ) ) ;
#1732=ORIENTED_EDGE ( 'NONE', *, *, #31639, .F. ) ;
#1734=CARTESIAN_POINT ( 'NONE',  ( 4.648177544792955347E-16, 21.00000000000002132, -109.2109808024215170 ) ) ;
#1735=VECTOR ( 'NONE', #15616, 1000.000000000000000 ) ;
#1736=ORIENTED_EDGE ( 'NONE', *, *, #30611, .F. ) ;
#1744=CYLINDRICAL_SURFACE ( 'NONE', #29193, 3.499999999999999556 ) ;
#1748=VERTEX_POINT ( 'NONE', #11707 ) ;
#1749=CARTESIAN_POINT ( 'NONE',  ( 3.500000000000000000, 15.47927405783633326, -109.2380641367107472 ) ) ;
#1750=CARTESIAN_POINT ( 'NONE',  ( 1.749999999999998224, 14.46891108675448834, -140.3213974700441042 ) ) ;
#1752=CARTESIAN_POINT ( 'NONE',  ( 3.310556943749999981, 15.58864905735837780, -137.3474391362328220 ) ) ;
#1753=CARTESIAN_POINT ( 'NONE',  ( 1.749999999999998224, 14.46891108675448301, -104.3213974700441042 ) ) ;
#1754=CARTESIAN_POINT ( 'NONE',  ( -0.9378221735089310451, 14.00000000000001066, -26.44938900211595367 ) ) ;
#1755=CARTESIAN_POINT ( 'NONE',  ( 3.310556943749999981, 15.58864905735837425, -128.4349391362327992 ) ) ;
#1756=CARTESIAN_POINT ( 'NONE',  ( -1.655278471874999990, 20.36702641396248836, -54.01827246956612782 ) ) ;
#1757=ORIENTED_EDGE ( 'NONE', *, *, #9355, .T. ) ;
#1759=CARTESIAN_POINT ( 'NONE',  ( -7.424026671074350129E-16, 13.45854811567264164, -134.4047308033774186 ) ) ;
#1762=CARTESIAN_POINT ( 'NONE',  ( -1.749999999999999778, 20.53108891324555785, -128.1276474690881741 ) ) ;
#1763=CARTESIAN_POINT ( 'NONE',  ( 3.310556943750001313, 19.41135094264166838, -110.1807724695661364 ) ) ;
#1767=CARTESIAN_POINT ( 'NONE',  ( 2.474675557024783212E-16, 21.54145188432739744, -82.21098080242150274 ) ) ;
#1768=CARTESIAN_POINT ( 'NONE',  ( 1.750000000000001110, 20.53108891324555074, -51.29431413575484555 ) ) ;
#1769=CARTESIAN_POINT ( 'NONE',  ( 1.655278471875001101, 20.36702641396248836, -47.09743913623280775 ) ) ;
#1770=CARTESIAN_POINT ( 'NONE',  ( -3.310556943750000425, 19.41135094264166838, -107.9349391362327992 ) ) ;
#1773=CARTESIAN_POINT ( 'NONE',  ( -3.500000000000001332, 17.50000000000001776, -88.96098080242151696 ) ) ;
#1774=CARTESIAN_POINT ( 'NONE',  ( -3.310556943750001313, 17.50000000000002132, -125.8516058028994706 ) ) ;
#1777=CARTESIAN_POINT ( 'NONE',  ( -3.500000000000000000, 19.52072594216371826, -117.0443141357548313 ) ) ;
#1778=CARTESIAN_POINT ( 'NONE',  ( -0.9378221735089310451, 14.00000000000001599, -71.44938900211596433 ) ) ;
#1779=CARTESIAN_POINT ( 'NONE',  ( -7.022189441860112050E-16, 13.67729811471671830, -58.60160580289947063 ) ) ;
#1781=CARTESIAN_POINT ( 'NONE',  ( 3.310556943749999981, 15.58864905735836892, -82.43493913623278502 ) ) ;
#1783=LINE ( 'NONE', #27726, #35217 ) ;
#1784=CARTESIAN_POINT ( 'NONE',  ( -0.9378221735089313782, 21.00000000000002132, -139.8600726046389013 ) ) ;
#1787=CARTESIAN_POINT ( 'NONE',  ( 3.310556943750001313, 17.50000000000001066, -40.26410580289947916 ) ) ;
#1794=CARTESIAN_POINT ( 'NONE',  ( 1.655278471874998436, 14.63297358603754006, -48.43077246956614346 ) ) ;
#1797=DIRECTION ( 'NONE',  ( -0.000000000000000000, 1.259100132267607459E-16, -1.000000000000000000 ) ) ;
#1799=CARTESIAN_POINT ( 'NONE',  ( -0.9378221735089310451, 14.00000000000002132, -104.4493890021159501 ) ) ;
#1800=ORIENTED_EDGE ( 'NONE', *, *, #21707, .F. ) ;
#1801=CYLINDRICAL_SURFACE ( 'NONE', #22044, 3.499999999999999556 ) ;
#1802=CARTESIAN_POINT ( 'NONE',  ( -3.500000000000002220, 15.47927405783632082, -39.87764746908817415 ) ) ;
#1803=DIRECTION ( 'NONE',  ( 0.000000000000000000, 1.000000000000000000, 0.000000000000000000 ) ) ;
#1805=( BOUNDED_CURVE ( )  B_SPLINE_CURVE ( 2, ( #26011, #22811, #467, #32582, #3447, #26222, #26423, #39380, #10256 ),
 .UNSPECIFIED., .F., .T. ) 
 B_SPLINE_CURVE_WITH_KNOTS ( ( 3, 2, 2, 2, 3 ),
 ( 0.06875000000000000555, 0.06944444444444444753, 0.07083333333333333148, 0.07222222222222221544, 0.07291666666666667129 ),
 .UNSPECIFIED. ) 
 CURVE ( )  GEOMETRIC_REPRESENTATION_ITEM ( )  RATIONAL_B_SPLINE_CURVE ( ( 0.9330127018922194093, 0.9330127018922200755, 1.000000000000000000, 0.8660254037844387076, 1.000000000000000000, 0.8660254037844387076, 1.000000000000000000, 0.9330127018922187432, 0.9330127018922194093 ) ) 
 REPRESENTATION_ITEM ( '' )  );
#1807=CARTESIAN_POINT ( 'NONE',  ( 2.474675557024783212E-16, 21.54145188432740810, -143.2109808024215170 ) ) ;
#1808=CARTESIAN_POINT ( 'NONE',  ( -3.500000000000000000, 19.52072594216370760, -59.73806413671076143 ) ) ;
#1809=CARTESIAN_POINT ( 'NONE',  ( -3.310556943750000425, 19.41135094264166838, -126.8474391362328078 ) ) ;
#1812=DIRECTION ( 'NONE',  ( 0.000000000000000000, 1.000000000000000000, 0.000000000000000000 ) ) ;
#1813=CARTESIAN_POINT ( 'NONE',  ( -3.310556943750000425, 19.41135094264166838, -121.9349391362327850 ) ) ;
#1815=CARTESIAN_POINT ( 'NONE',  ( -1.749999999999999778, 20.53108891324554719, -38.82139747004409713 ) ) ;
#1817=CARTESIAN_POINT ( 'NONE',  ( 3.500000000000001332, 17.50000000000002487, -130.4609808024214885 ) ) ;
#1818=CARTESIAN_POINT ( 'NONE',  ( 3.500000000000000000, 15.47927405783632793, -89.23806413671076143 ) ) ;
#1820=CARTESIAN_POINT ( 'NONE',  ( 2.474675557024783212E-16, 21.54145188432739388, -68.90473080337743284 ) ) ;
#1822=CARTESIAN_POINT ( 'NONE',  ( 1.655278471875001101, 20.36702641396248836, -56.18493913623279212 ) ) ;
#1824=FACE_OUTER_BOUND ( 'NONE', #10588, .T. ) ;
#1825=CARTESIAN_POINT ( 'NONE',  ( -3.310556943750000425, 19.41135094264166128, -73.93493913623278502 ) ) ;
#1827=CARTESIAN_POINT ( 'NONE',  ( -3.310556943750002201, 15.58864905735837425, -104.6807724695661364 ) ) ;
#1828=CARTESIAN_POINT ( 'NONE',  ( -3.310556943750002645, 15.58864905735837070, -75.68077246956613635 ) ) ;
#1830=CARTESIAN_POINT ( 'NONE',  ( -3.310556943750001313, 17.50000000000001776, -98.85160580289947063 ) ) ;
#1832=CARTESIAN_POINT ( 'NONE',  ( -1.750000000000002220, 14.46891108675447590, -32.79431413575484555 ) ) ;
#1833=CARTESIAN_POINT ( 'NONE',  ( -3.500000000000002220, 15.47927405783632970, -81.57139747004410424 ) ) ;
#1835=CARTESIAN_POINT ( 'NONE',  ( 1.655278471874998436, 14.63297358603754184, -57.43077246956614346 ) ) ;
#1837=CARTESIAN_POINT ( 'NONE',  ( 3.310556943750001313, 19.41135094264166838, -110.1807724695661364 ) ) ;
#1843=EDGE_CURVE ( 'NONE', #11917, #41462, #6545, .T. ) ;
#1844=CARTESIAN_POINT ( 'NONE',  ( 1.655278471875001101, 20.36702641396248836, -61.09743913623280775 ) ) ;
#1845=ORIENTED_EDGE ( 'NONE', *, *, #25952, .T. ) ;
#1846=ORIENTED_EDGE ( 'NONE', *, *, #21839, .T. ) ;
#1847=CARTESIAN_POINT ( 'NONE',  ( -1.394453263437886604E-15, 14.00000000000002132, -130.7109808024214885 ) ) ;
#1848=CARTESIAN_POINT ( 'NONE',  ( -4.648177544792955347E-16, 21.00000000000002487, -142.9047308033773902 ) ) ;
#1853=CARTESIAN_POINT ( 'NONE',  ( -1.655278471874999990, 20.36702641396249902, -129.9307724695661364 ) ) ;
#1854=CARTESIAN_POINT ( 'NONE',  ( 4.648177544792955347E-16, 21.00000000000002132, -116.2109808024215027 ) ) ;
#1855=CARTESIAN_POINT ( 'NONE',  ( -3.310556943750002645, 15.58864905735836714, -41.76827246956612782 ) ) ;
#1856=CARTESIAN_POINT ( 'NONE',  ( 3.310556943750001313, 17.50000000000001066, -31.35160580289945997 ) ) ;
#1857=CARTESIAN_POINT ( 'NONE',  ( -1.655278471874999990, 20.36702641396249192, -91.01827246956612782 ) ) ;
#1858=CARTESIAN_POINT ( 'NONE',  ( 3.310556943749999981, 15.58864905735837780, -142.3474391362327935 ) ) ;
#1861=CARTESIAN_POINT ( 'NONE',  ( 3.310556943750001313, 19.41135094264167549, -139.2682724695661420 ) ) ;
#1863=CARTESIAN_POINT ( 'NONE',  ( 3.500000000000000000, 15.47927405783632615, -94.54431413575484555 ) ) ;
#1866=CARTESIAN_POINT ( 'NONE',  ( 3.500000000000001332, 17.50000000000001776, -88.15473080337743284 ) ) ;
#1867=CARTESIAN_POINT ( 'NONE',  ( -3.310556943750001313, 17.50000000000001421, -68.85160580289947063 ) ) ;
#1870=CARTESIAN_POINT ( 'NONE',  ( -1.749999999999999778, 20.53108891324555785, -120.1276474690881741 ) ) ;
#1871=CARTESIAN_POINT ( 'NONE',  ( 3.500000000000001332, 17.50000000000001421, -47.46098080242150274 ) ) ;
#1872=CARTESIAN_POINT ( 'NONE',  ( -7.022189441860112050E-16, 13.67729811471672896, -121.5141058028994792 ) ) ;
#1874=CARTESIAN_POINT ( 'NONE',  ( 3.500000000000001332, 17.50000000000001776, -95.46098080242150274 ) ) ;
#1876=CARTESIAN_POINT ( 'NONE',  ( -3.500000000000000888, 19.52072594216371826, -113.7380641367107472 ) ) ;
#1879=DIRECTION ( 'NONE',  ( -0.000000000000000000, 1.259100132267607459E-16, -1.000000000000000000 ) ) ;
#1882=CARTESIAN_POINT ( 'NONE',  ( -3.310556943750000425, 19.41135094264166483, -70.84743913623280775 ) ) ;
#1883=( BOUNDED_CURVE ( )  B_SPLINE_CURVE ( 2, ( #29831, #698, #39610, #14309, #1130, #17294, #13669, #40252, #37076 ),
 .UNSPECIFIED., .F., .T. ) 
 B_SPLINE_CURVE_WITH_KNOTS ( ( 3, 2, 2, 2, 3 ),
 ( 0.6229166666666666741, 0.6236111111111111160, 0.6250000000000000000, 0.6263888888888888840, 0.6270833333333333259 ),
 .UNSPECIFIED. ) 
 CURVE ( )  GEOMETRIC_REPRESENTATION_ITEM ( )  RATIONAL_B_SPLINE_CURVE ( ( 0.9330127018922194093, 0.9330127018922194093, 1.000000000000000000, 0.8660254037844387076, 1.000000000000000000, 0.8660254037844387076, 1.000000000000000000, 0.9330127018922194093, 0.9330127018922194093 ) ) 
 REPRESENTATION_ITEM ( '' )  );
#1885=CARTESIAN_POINT ( 'NONE',  ( -1.394453263437886604E-15, 14.00000000000001421, -72.71098080242151696 ) ) ;
#1887=CARTESIAN_POINT ( 'NONE',  ( -3.310556943750000425, 19.41135094264166128, -24.84743913623281486 ) ) ;
#1888=CARTESIAN_POINT ( 'NONE',  ( 3.500000000000001332, 17.50000000000001066, -25.46098080242151340 ) ) ;
#1889=CARTESIAN_POINT ( 'NONE',  ( -3.310556943750000425, 19.41135094264166483, -82.84743913623279354 ) ) ;
#1890=ORIENTED_EDGE ( 'NONE', *, *, #17860, .T. ) ;
#1891=VERTEX_POINT ( 'NONE', #12122 ) ;
#1897=CARTESIAN_POINT ( 'NONE',  ( 3.310556943749999981, 15.58864905735836182, -48.43493913623279923 ) ) ;
#1898=CARTESIAN_POINT ( 'NONE',  ( 3.310556943750001313, 17.50000000000002132, -109.3516058028994564 ) ) ;
#1900=CARTESIAN_POINT ( 'NONE',  ( -1.655278471875002211, 14.63297358603754006, -34.59743913623280775 ) ) ;
#1901=CARTESIAN_POINT ( 'NONE',  ( -1.655278471874999990, 20.36702641396248836, -59.01827246956613493 ) ) ;
#1902=CARTESIAN_POINT ( 'NONE',  ( 1.749999999999998224, 14.46891108675448478, -113.6276474690881741 ) ) ;
#1904=CARTESIAN_POINT ( 'NONE',  ( -1.655278471875002211, 14.63297358603754894, -98.59743913623280775 ) ) ;
#1905=CARTESIAN_POINT ( 'NONE',  ( 0.9378221735089300459, 21.00000000000001776, -97.94938900211596433 ) ) ;
#1909=CARTESIAN_POINT ( 'NONE',  ( 1.749999999999998224, 14.46891108675447768, -62.62764746908818125 ) ) ;
#1911=CARTESIAN_POINT ( 'NONE',  ( -3.310556943750000425, 19.41135094264165772, -29.84743913623280420 ) ) ;
#1912=CARTESIAN_POINT ( 'NONE',  ( 3.310556943749999981, 15.58864905735836892, -88.43493913623279923 ) ) ;
#1914=CARTESIAN_POINT ( 'NONE',  ( 1.750000000000001110, 20.53108891324555074, -52.98806413671076854 ) ) ;
#1915=CARTESIAN_POINT ( 'NONE',  ( -7.022189441860112050E-16, 13.67729811471672541, -108.6016058028994706 ) ) ;
#1916=CARTESIAN_POINT ( 'NONE',  ( 3.310556943749999981, 15.58864905735836182, -40.43493913623279212 ) ) ;
#1922=CARTESIAN_POINT ( 'NONE',  ( 0.000000000000000000, 17.50000000000002487, -149.5231586289125687 ) ) ;
#1925=CARTESIAN_POINT ( 'NONE',  ( 1.655278471875001101, 20.36702641396249192, -88.09743913623280775 ) ) ;
#1928=ORIENTED_EDGE ( 'NONE', *, *, #1488, .T. ) ;
#1930=( BOUNDED_CURVE ( )  B_SPLINE_CURVE ( 2, ( #13761, #19509, #3757, #20141, #39485, #7170, #26740, #9521, #19200 ),
 .UNSPECIFIED., .F., .F. ) 
 B_SPLINE_CURVE_WITH_KNOTS ( ( 3, 2, 2, 2, 3 ),
 ( 0.7145833333333333481, 0.7152777777777777901, 0.7166666666666666741, 0.7180555555555555580, 0.7187500000000000000 ),
 .UNSPECIFIED. ) 
 CURVE ( )  GEOMETRIC_REPRESENTATION_ITEM ( )  RATIONAL_B_SPLINE_CURVE ( ( 0.9330127018922194093, 0.9330127018922194093, 1.000000000000000000, 0.8660254037844387076, 1.000000000000000000, 0.8660254037844387076, 1.000000000000000000, 0.9330127018922194093, 0.9330127018922194093 ) ) 
 REPRESENTATION_ITEM ( '' )  );
#1932=VERTEX_POINT ( 'NONE', #41700 ) ;
#1937=CARTESIAN_POINT ( 'NONE',  ( 3.500000000000001332, 19.52072594216371826, -118.0713974700440900 ) ) ;
#1938=ORIENTED_EDGE ( 'NONE', *, *, #36533, .F. ) ;
#1944=ORIENTED_EDGE ( 'NONE', *, *, #28872, .F. ) ;
#1946=CARTESIAN_POINT ( 'NONE',  ( 1.750000000000001110, 20.53108891324555785, -108.9880641367107614 ) ) ;
#1947=CARTESIAN_POINT ( 'NONE',  ( -1.394453263437886604E-15, 14.00000000000001776, -96.40473080337741862 ) ) ;
#1948=EDGE_CURVE ( 'NONE', #38620, #21195, #15238, .T. ) ;
#1949=CARTESIAN_POINT ( 'NONE',  ( 3.310556943750001313, 17.50000000000002487, -136.2641058028994792 ) ) ;
#1950=CARTESIAN_POINT ( 'NONE',  ( 3.500000000000001332, 17.50000000000002132, -104.1547308033774186 ) ) ;
#1952=CARTESIAN_POINT ( 'NONE',  ( 3.310556943750001313, 17.50000000000002132, -126.3516058028994706 ) ) ;
#1953=CARTESIAN_POINT ( 'NONE',  ( 3.310556943750001313, 19.41135094264166128, -58.26827246956613493 ) ) ;
#1956=CARTESIAN_POINT ( 'NONE',  ( 3.500000000000000000, 15.47927405783633503, -135.2380641367107614 ) ) ;
#1958=CARTESIAN_POINT ( 'NONE',  ( 2.474675557024783212E-16, 21.54145188432740099, -128.2109808024214885 ) ) ;
#1959=CARTESIAN_POINT ( 'NONE',  ( -7.022189441860112050E-16, 13.67729811471672718, -110.5141058028994792 ) ) ;
#1963=CARTESIAN_POINT ( 'NONE',  ( 3.500000000000001776, 19.52072594216371115, -82.37764746908817415 ) ) ;
#1966=CARTESIAN_POINT ( 'NONE',  ( -3.310556943750000425, 19.41135094264166128, -47.84743913623280775 ) ) ;
#1967=CARTESIAN_POINT ( 'NONE',  ( 3.310556943750001313, 19.41135094264166838, -109.2682724695661278 ) ) ;
#1969=CARTESIAN_POINT ( 'NONE',  ( 4.286263797015737581E-16, 14.00000000000002487, -149.5231586289125687 ) ) ;
#1970=CARTESIAN_POINT ( 'NONE',  ( -3.310556943750002201, 15.58864905735837780, -122.7682724695661278 ) ) ;
#1973=CARTESIAN_POINT ( 'NONE',  ( 3.500000000000001332, 17.50000000000001066, -27.46098080242151340 ) ) ;
#1974=CARTESIAN_POINT ( 'NONE',  ( 4.648177544792955347E-16, 21.00000000000002132, -111.2109808024214885 ) ) ;
#1975=ADVANCED_FACE ( 'NONE', ( #41918 ), #12766, .T. ) ;
#1976=CARTESIAN_POINT ( 'NONE',  ( -3.310556943750002645, 15.58864905735836892, -60.76827246956613493 ) ) ;
#1977=EDGE_CURVE ( 'NONE', #29219, #3982, #6798, .T. ) ;
#1979=CARTESIAN_POINT ( 'NONE',  ( -3.310556943750001313, 17.50000000000001776, -75.85160580289945642 ) ) ;
#1981=EDGE_CURVE ( 'NONE', #4297, #35835, #6285, .T. ) ;
#1983=CARTESIAN_POINT ( 'NONE',  ( 4.648177544792955347E-16, 21.00000000000001776, -76.90473080337740441 ) ) ;
#1984=CARTESIAN_POINT ( 'NONE',  ( -1.750000000000002220, 14.46891108675447946, -55.79431413575483845 ) ) ;
#1988=CARTESIAN_POINT ( 'NONE',  ( -1.655278471874999990, 20.36702641396248481, -37.93077246956613635 ) ) ;
#1994=CARTESIAN_POINT ( 'NONE',  ( 2.340729813953370519E-16, 21.32270188528330479, -45.01410580289947916 ) ) ;
#2000=CARTESIAN_POINT ( 'NONE',  ( 3.500000000000001776, 19.52072594216370405, -25.37764746908817415 ) ) ;
#2002=CARTESIAN_POINT ( 'NONE',  ( -1.394453263437886604E-15, 14.00000000000001066, -43.40473080337743284 ) ) ;
#2003=CARTESIAN_POINT ( 'NONE',  ( 0.000000000000000000, 17.50000000000002487, -149.5231586289125687 ) ) ;
#2004=CARTESIAN_POINT ( 'NONE',  ( -1.750000000000002220, 14.46891108675447590, -39.79431413575484555 ) ) ;
#2005=CARTESIAN_POINT ( 'NONE',  ( 4.286263797015737581E-16, 14.00000000000002487, -149.5231586289125687 ) ) ;
#2009=CARTESIAN_POINT ( 'NONE',  ( -7.022189441860112050E-16, 13.67729811471671475, -26.60160580289946708 ) ) ;
#2010=EDGE_CURVE ( 'NONE', #644, #9807, #23940, .T. ) ;
#2011=CARTESIAN_POINT ( 'NONE',  ( -1.749999999999999778, 20.53108891324555074, -59.82139747004409713 ) ) ;
#2012=CARTESIAN_POINT ( 'NONE',  ( 3.310556943749999981, 15.58864905735837425, -129.3474391362328220 ) ) ;
#2015=LINE ( 'NONE', #14998, #22505 ) ;
#2016=CARTESIAN_POINT ( 'NONE',  ( 1.655278471874998436, 14.63297358603755072, -123.5182724695661278 ) ) ;
#2017=DIRECTION ( 'NONE',  ( 0.000000000000000000, 1.000000000000000000, 0.000000000000000000 ) ) ;
#2018=CARTESIAN_POINT ( 'NONE',  ( 3.500000000000000000, 15.47927405783632082, -37.23806413671077564 ) ) ;
#2019=CARTESIAN_POINT ( 'NONE',  ( -1.394453263437886604E-15, 14.00000000000001066, -49.40473080337742573 ) ) ;
#2021=CARTESIAN_POINT ( 'NONE',  ( -1.655278471875002211, 14.63297358603755427, -136.6849391362327992 ) ) ;
#2022=EDGE_CURVE ( 'NONE', #18659, #38292, #33987, .T. ) ;
#2023=CYLINDRICAL_SURFACE ( 'NONE', #33426, 3.499999999999999556 ) ;
#2024=CARTESIAN_POINT ( 'NONE',  ( 1.655278471874998436, 14.63297358603754006, -47.51827246956613493 ) ) ;
#2026=CARTESIAN_POINT ( 'NONE',  ( -0.9378221735089310451, 14.00000000000001066, -41.44938900211595012 ) ) ;
#2027=CARTESIAN_POINT ( 'NONE',  ( 3.310556943750001313, 17.50000000000001421, -73.35160580289947063 ) ) ;
#2030=CARTESIAN_POINT ( 'NONE',  ( 3.310556943750001313, 17.50000000000002132, -102.2641058028994649 ) ) ;
#2031=CARTESIAN_POINT ( 'NONE',  ( 3.310556943750001313, 17.50000000000001421, -70.26410580289947916 ) ) ;
#2033=CARTESIAN_POINT ( 'NONE',  ( -3.310556943750001313, 17.50000000000001776, -94.85160580289945642 ) ) ;
#2037=DIRECTION ( 'NONE',  ( 0.000000000000000000, 1.000000000000000000, 0.000000000000000000 ) ) ;
#2039=CARTESIAN_POINT ( 'NONE',  ( -7.022189441860112050E-16, 13.67729811471672186, -56.51410580289948626 ) ) ;
#2040=CARTESIAN_POINT ( 'NONE',  ( 1.655278471874998436, 14.63297358603754894, -113.4307724695661364 ) ) ;
#2047=CARTESIAN_POINT ( 'NONE',  ( -7.022189441860112050E-16, 13.67729811471671830, -65.51410580289946495 ) ) ;
#2048=ORIENTED_EDGE ( 'NONE', *, *, #6979, .T. ) ;
#2050=( BOUNDED_CURVE ( )  B_SPLINE_CURVE ( 2, ( #25906, #31853, #32486, #6551, #35473, #31645, #12930, #25067, #19517 ),
 .UNSPECIFIED., .F., .F. ) 
 B_SPLINE_CURVE_WITH_KNOTS ( ( 3, 2, 2, 2, 3 ),
 ( 0.6479166666666666963, 0.6486111111111111382, 0.6500000000000000222, 0.6513888888888889062, 0.6520833333333333481 ),
 .UNSPECIFIED. ) 
 CURVE ( )  GEOMETRIC_REPRESENTATION_ITEM ( )  RATIONAL_B_SPLINE_CURVE ( ( 0.9330127018922194093, 0.9330127018922194093, 1.000000000000000000, 0.8660254037844387076, 1.000000000000000000, 0.8660254037844387076, 1.000000000000000000, 0.9330127018922194093, 0.9330127018922194093 ) ) 
 REPRESENTATION_ITEM ( '' )  );
#2051=DIRECTION ( 'NONE',  ( -0.000000000000000000, 1.259100132267607459E-16, -1.000000000000000000 ) ) ;
#2054=DIRECTION ( 'NONE',  ( -0.000000000000000000, 1.259100132267607459E-16, -1.000000000000000000 ) ) ;
#2057=CARTESIAN_POINT ( 'NONE',  ( 3.310556943750001313, 19.41135094264166838, -129.1807724695661364 ) ) ;
#2060=CARTESIAN_POINT ( 'NONE',  ( -1.655278471874999990, 20.36702641396248481, -42.01827246956612782 ) ) ;
#2061=CARTESIAN_POINT ( 'NONE',  ( -3.310556943750000425, 19.41135094264165772, -33.93493913623279923 ) ) ;
#2062=CARTESIAN_POINT ( 'NONE',  ( 3.310556943750001313, 19.41135094264166483, -93.26827246956611361 ) ) ;
#2063=CARTESIAN_POINT ( 'NONE',  ( 3.500000000000001776, 19.52072594216370405, -24.07139747004409358 ) ) ;
#2064=ORIENTED_EDGE ( 'NONE', *, *, #9722, .F. ) ;
#2067=CARTESIAN_POINT ( 'NONE',  ( 1.655278471875001101, 20.36702641396249902, -137.1849391362327992 ) ) ;
#2070=CARTESIAN_POINT ( 'NONE',  ( 2.340729813953370519E-16, 21.32270188528330834, -60.01410580289947916 ) ) ;
#2071=CARTESIAN_POINT ( 'NONE',  ( -3.500000000000000000, 19.52072594216371826, -122.7380641367107756 ) ) ;
#2072=CARTESIAN_POINT ( 'NONE',  ( 1.750000000000001110, 20.53108891324555429, -86.98806413671076143 ) ) ;
#2074=CARTESIAN_POINT ( 'NONE',  ( -3.310556943750001313, 17.50000000000001421, -62.85160580289946353 ) ) ;
#2078=CARTESIAN_POINT ( 'NONE',  ( 4.648177544792955347E-16, 21.00000000000002132, -116.9047308033774328 ) ) ;
#2079=CARTESIAN_POINT ( 'NONE',  ( -1.749999999999999778, 20.53108891324555074, -50.12764746908818125 ) ) ;
#2080=CARTESIAN_POINT ( 'NONE',  ( 2.340729813953370519E-16, 21.32270188528331900, -119.0141058028994792 ) ) ;
#2082=DIRECTION ( 'NONE',  ( -0.000000000000000000, 1.259100132267607459E-16, -1.000000000000000000 ) ) ;
#2083=ORIENTED_EDGE ( 'NONE', *, *, #7117, .T. ) ;
#2084=CARTESIAN_POINT ( 'NONE',  ( 3.500000000000001776, 19.52072594216371826, -116.0713974700440900 ) ) ;
#2086=DIRECTION ( 'NONE',  ( 0.000000000000000000, 1.000000000000000000, 0.000000000000000000 ) ) ;
#2090=CARTESIAN_POINT ( 'NONE',  ( -3.310556943750001313, 17.50000000000001421, -69.76410580289947916 ) ) ;
#2091=DIRECTION ( 'NONE',  ( -0.000000000000000000, 1.259100132267607459E-16, -1.000000000000000000 ) ) ;
#2095=CARTESIAN_POINT ( 'NONE',  ( -1.655278471874999990, 20.36702641396248481, -23.93077246956613990 ) ) ;
#2097=CARTESIAN_POINT ( 'NONE',  ( 1.655278471874998436, 14.63297358603754539, -81.43077246956615056 ) ) ;
#2104=ADVANCED_FACE ( 'NONE', ( #4665 ), #39766, .T. ) ;
#2108=CARTESIAN_POINT ( 'NONE',  ( 3.310556943749999981, 15.58864905735836182, -51.43493913623279923 ) ) ;
#2109=CARTESIAN_POINT ( 'NONE',  ( -7.022189441860112050E-16, 13.67729811471672541, -108.6016058028994422 ) ) ;
#2111=AXIS2_PLACEMENT_3D ( 'NONE', #34529, #41337, #12186 ) ;
#2112=CARTESIAN_POINT ( 'NONE',  ( 1.655278471874998436, 14.63297358603753828, -34.43077246956615056 ) ) ;
#2113=CARTESIAN_POINT ( 'NONE',  ( -3.310556943750002645, 15.58864905735836892, -58.76827246956612782 ) ) ;
#2114=CARTESIAN_POINT ( 'NONE',  ( -1.750000000000002220, 14.46891108675448656, -110.7943141357548456 ) ) ;
#2116=CARTESIAN_POINT ( 'NONE',  ( 3.310556943749999981, 15.58864905735837070, -98.34743913623282197 ) ) ;
#2117=EDGE_CURVE ( 'NONE', #22032, #8132, #20415, .T. ) ;
#2118=CARTESIAN_POINT ( 'NONE',  ( 0.9378221735089300459, 21.00000000000001421, -51.94938900211595012 ) ) ;
#2119=CARTESIAN_POINT ( 'NONE',  ( -1.836030130193217234E-14, 21.00000000000002487, -134.9047308033774186 ) ) ;
#2121=CARTESIAN_POINT ( 'NONE',  ( -3.500000000000001332, 17.50000000000001421, -63.96098080242150274 ) ) ;
#2122=CARTESIAN_POINT ( 'NONE',  ( 0.000000000000000000, 17.50000000000002487, -149.5231586289125687 ) ) ;
#2123=CARTESIAN_POINT ( 'NONE',  ( -3.310556943750000425, 19.41135094264165772, -30.84743913623280775 ) ) ;
#2125=CARTESIAN_POINT ( 'NONE',  ( 1.750000000000001110, 20.53108891324555074, -54.98806413671076854 ) ) ;
#2127=CARTESIAN_POINT ( 'NONE',  ( -1.655278471875002211, 14.63297358603755072, -109.6849391362327992 ) ) ;
#2128=CARTESIAN_POINT ( 'NONE',  ( 3.310556943750001313, 19.41135094264166128, -40.26827246956612782 ) ) ;
#2130=CARTESIAN_POINT ( 'NONE',  ( 0.9378221735089300459, 21.00000000000001421, -53.25563900116003424 ) ) ;
#2136=CARTESIAN_POINT ( 'NONE',  ( 3.310556943749999981, 15.58864905735836892, -88.34743913623282197 ) ) ;
#2138=CARTESIAN_POINT ( 'NONE',  ( -1.394453263437886604E-15, 14.00000000000000711, -23.71098080242150985 ) ) ;
#2145=CARTESIAN_POINT ( 'NONE',  ( -1.394453263437886604E-15, 14.00000000000001776, -91.71098080242150274 ) ) ;
#2151=ORIENTED_EDGE ( 'NONE', *, *, #26639, .T. ) ;
#2152=CARTESIAN_POINT ( 'NONE',  ( 1.750000000000001110, 20.53108891324555429, -90.98806413671076143 ) ) ;
#2153=VECTOR ( 'NONE', #30379, 1000.000000000000000 ) ;
#2154=CARTESIAN_POINT ( 'NONE',  ( 0.000000000000000000, 17.50000000000002487, -149.5231586289125687 ) ) ;
#2155=CARTESIAN_POINT ( 'NONE',  ( 1.655278471875001101, 20.36702641396249902, -135.0974391362328220 ) ) ;
#2156=CARTESIAN_POINT ( 'NONE',  ( -1.394453263437886604E-15, 14.00000000000001066, -38.40473080337743284 ) ) ;
#2157=EDGE_LOOP ( 'NONE', ( #2899, #35197, #8588, #16807 ) ) ;
#2158=DIRECTION ( 'NONE',  ( -0.000000000000000000, 1.259100132267607459E-16, -1.000000000000000000 ) ) ;
#2159=CARTESIAN_POINT ( 'NONE',  ( 1.655278471874998436, 14.63297358603755072, -126.5182724695661278 ) ) ;
#2160=CARTESIAN_POINT ( 'NONE',  ( -3.310556943750002645, 15.58864905735836892, -56.76827246956612782 ) ) ;
#2162=EDGE_CURVE ( 'NONE', #18376, #11548, #17230, .T. ) ;
#2164=CARTESIAN_POINT ( 'NONE',  ( -1.749999999999999778, 20.53108891324556140, -136.8213974700441042 ) ) ;
#2167=CARTESIAN_POINT ( 'NONE',  ( -3.310556943750002645, 15.58864905735837070, -76.76827246956612782 ) ) ;
#2168=CARTESIAN_POINT ( 'NONE',  ( -7.424026671074350129E-16, 13.45854811567264164, -130.7109808024214885 ) ) ;
#2169=CARTESIAN_POINT ( 'NONE',  ( 3.310556943749999981, 15.58864905735837247, -112.3474391362328078 ) ) ;
#2175=CARTESIAN_POINT ( 'NONE',  ( -3.500000000000001332, 17.50000000000001776, -77.96098080242150274 ) ) ;
#2176=CARTESIAN_POINT ( 'NONE',  ( 3.500000000000000000, 15.47927405783632082, -51.54431413575484555 ) ) ;
#2177=CARTESIAN_POINT ( 'NONE',  ( 3.310556943750001313, 19.41135094264165772, -46.18077246956615056 ) ) ;
#2178=( BOUNDED_CURVE ( )  B_SPLINE_CURVE ( 2, ( #17275, #4917, #33654, #39816, #14085, #27271, #24284, #20881, #21087 ),
 .UNSPECIFIED., .F., .T. ) 
 B_SPLINE_CURVE_WITH_KNOTS ( ( 3, 2, 2, 2, 3 ),
 ( 0.7145833333333333481, 0.7152777777777777901, 0.7166666666666666741, 0.7180555555555555580, 0.7187500000000000000 ),
 .UNSPECIFIED. ) 
 CURVE ( )  GEOMETRIC_REPRESENTATION_ITEM ( )  RATIONAL_B_SPLINE_CURVE ( ( 0.9330127018922194093, 0.9330127018922194093, 1.000000000000000000, 0.8660254037844387076, 1.000000000000000000, 0.8660254037844387076, 1.000000000000000000, 0.9330127018922194093, 0.9330127018922194093 ) ) 
 REPRESENTATION_ITEM ( '' )  );
#2179=CARTESIAN_POINT ( 'NONE',  ( 3.310556943750001313, 19.41135094264166838, -105.2682724695661278 ) ) ;
#2182=CARTESIAN_POINT ( 'NONE',  ( -0.9378221735089291577, 21.00000000000001421, -72.86007260463891555 ) ) ;
#2183=CARTESIAN_POINT ( 'NONE',  ( -3.310556943750001313, 17.50000000000002132, -121.8516058028994706 ) ) ;
#2187=CARTESIAN_POINT ( 'NONE',  ( 3.500000000000000000, 15.47927405783632082, -50.54431413575484555 ) ) ;
#2188=CARTESIAN_POINT ( 'NONE',  ( 1.750000000000001110, 20.53108891324556140, -129.9880641367107614 ) ) ;
#2189=DIRECTION ( 'NONE',  ( -0.000000000000000000, 1.259100132267607459E-16, -1.000000000000000000 ) ) ;
#2191=ORIENTED_EDGE ( 'NONE', *, *, #21268, .T. ) ;
#2192=CARTESIAN_POINT ( 'NONE',  ( 3.310556943750001313, 17.50000000000001776, -76.35160580289945642 ) ) ;
#2194=DIRECTION ( 'NONE',  ( 0.000000000000000000, 1.000000000000000000, 0.000000000000000000 ) ) ;
#2195=CARTESIAN_POINT ( 'NONE',  ( 1.750000000000001110, 20.53108891324555429, -79.98806413671076143 ) ) ;
#2196=CARTESIAN_POINT ( 'NONE',  ( -1.749999999999999778, 20.53108891324555074, -56.12764746908817415 ) ) ;
#2198=CARTESIAN_POINT ( 'NONE',  ( 1.749999999999998224, 14.46891108675447946, -74.32139747004410424 ) ) ;
#2200=CARTESIAN_POINT ( 'NONE',  ( 3.310556943749999981, 15.58864905735836182, -41.34743913623280065 ) ) ;
#2201=CARTESIAN_POINT ( 'NONE',  ( -1.750000000000002220, 14.46891108675448301, -93.48806413671076143 ) ) ;
#2202=VECTOR ( 'NONE', #25074, 1000.000000000000000 ) ;
#2204=EDGE_LOOP ( 'NONE', ( #35792, #16999, #11972, #23181 ) ) ;
#2207=CARTESIAN_POINT ( 'NONE',  ( -3.310556943750000425, 19.41135094264166128, -47.84743913623280775 ) ) ;
#2208=ADVANCED_FACE ( 'NONE', ( #39542 ), #10840, .T. ) ;
#2210=AXIS2_PLACEMENT_3D ( 'NONE', #33065, #3932, #26698 ) ;
#2211=VERTEX_POINT ( 'NONE', #17445 ) ;
#2213=CARTESIAN_POINT ( 'NONE',  ( 4.286263797015737581E-16, 14.00000000000002487, -149.5231586289125687 ) ) ;
#2216=EDGE_CURVE ( 'NONE', #18853, #23290, #10643, .T. ) ;
#2217=CARTESIAN_POINT ( 'NONE',  ( 1.749999999999998224, 14.46891108675448478, -112.6276474690881884 ) ) ;
#2218=CARTESIAN_POINT ( 'NONE',  ( -1.749999999999999778, 20.53108891324554719, -41.12764746908817415 ) ) ;
#2219=DIRECTION ( 'NONE',  ( -0.000000000000000000, 1.259100132267607459E-16, -1.000000000000000000 ) ) ;
#2220=CARTESIAN_POINT ( 'NONE',  ( 4.648177544792955347E-16, 21.00000000000001421, -64.90473080337743284 ) ) ;
#2224=CARTESIAN_POINT ( 'NONE',  ( -3.310556943750002645, 15.58864905735836182, -25.76827246956613138 ) ) ;
#2225=CARTESIAN_POINT ( 'NONE',  ( -1.749999999999999778, 20.53108891324555429, -100.8213974700440900 ) ) ;
#2226=CARTESIAN_POINT ( 'NONE',  ( 1.655278471874998436, 14.63297358603755072, -128.4307724695661364 ) ) ;
#2229=CARTESIAN_POINT ( 'NONE',  ( -3.500000000000002220, 15.47927405783632793, -76.57139747004410424 ) ) ;
#2230=CARTESIAN_POINT ( 'NONE',  ( -3.310556943750001313, 17.50000000000002132, -121.8516058028994706 ) ) ;
#2231=CARTESIAN_POINT ( 'NONE',  ( -3.500000000000000000, 19.52072594216370760, -55.73806413671075433 ) ) ;
#2232=CARTESIAN_POINT ( 'NONE',  ( -3.500000000000001332, 17.50000000000001066, -37.65473080337743284 ) ) ;
#2233=CARTESIAN_POINT ( 'NONE',  ( -3.500000000000000000, 19.52072594216370760, -49.73806413671076854 ) ) ;
#2234=CARTESIAN_POINT ( 'NONE',  ( 3.500000000000001332, 19.52072594216371826, -130.3776474690881741 ) ) ;
#2235=CARTESIAN_POINT ( 'NONE',  ( -3.310556943750002201, 15.58864905735837958, -140.7682724695661420 ) ) ;
#2238=CARTESIAN_POINT ( 'NONE',  ( -7.022189441860112050E-16, 13.67729811471671830, -50.60160580289946353 ) ) ;
#2240=LINE ( 'NONE', #15009, #20413 ) ;
#2241=AXIS2_PLACEMENT_3D ( 'NONE', #23409, #14254, #14051 ) ;
#2242=CARTESIAN_POINT ( 'NONE',  ( -3.310556943750002645, 15.58864905735837070, -72.76827246956612782 ) ) ;
#2244=CARTESIAN_POINT ( 'NONE',  ( -1.655278471874999990, 20.36702641396249547, -103.9307724695661364 ) ) ;
#2245=CARTESIAN_POINT ( 'NONE',  ( -1.655278471875002211, 14.63297358603754539, -71.59743913623280775 ) ) ;
#2247=CARTESIAN_POINT ( 'NONE',  ( 2.340729813953370519E-16, 21.32270188528331190, -89.10160580289947063 ) ) ;
#2250=CARTESIAN_POINT ( 'NONE',  ( 4.648177544792955347E-16, 21.00000000000002487, -130.9047308033774186 ) ) ;
#2252=CARTESIAN_POINT ( 'NONE',  ( 3.310556943749999981, 15.58864905735836537, -57.34743913623279354 ) ) ;
#2253=( BOUNDED_CURVE ( )  B_SPLINE_CURVE ( 2, ( #18947, #31911, #15764, #25337, #12352, #38295, #9162, #2781, #41501 ),
 .UNSPECIFIED., .F., .T. ) 
 B_SPLINE_CURVE_WITH_KNOTS ( ( 3, 2, 2, 2, 3 ),
 ( 0.03125000000000000000, 0.03194444444444444198, 0.03333333333333333287, 0.03472222222222222376, 0.03541666666666666574 ),
 .UNSPECIFIED. ) 
 CURVE ( )  GEOMETRIC_REPRESENTATION_ITEM ( )  RATIONAL_B_SPLINE_CURVE ( ( 0.9330127018922194093, 0.9330127018922195203, 1.000000000000000000, 0.8660254037844387076, 1.000000000000000000, 0.8660254037844387076, 1.000000000000000000, 0.9330127018922194093, 0.9330127018922194093 ) ) 
 REPRESENTATION_ITEM ( '' )  );
#2254=DIRECTION ( 'NONE',  ( 0.000000000000000000, 1.000000000000000000, 0.000000000000000000 ) ) ;
#2255=CARTESIAN_POINT ( 'NONE',  ( 1.655278471875001101, 20.36702641396249547, -113.0974391362328078 ) ) ;
#2256=EDGE_LOOP ( 'NONE', ( #11249, #24395, #23716, #17186 ) ) ;
#2258=EDGE_CURVE ( 'NONE', #35892, #32425, #29254, .T. ) ;
#2262=CARTESIAN_POINT ( 'NONE',  ( -3.310556943750001313, 17.50000000000001421, -62.76410580289947205 ) ) ;
#2263=VERTEX_POINT ( 'NONE', #13107 ) ;
#2264=ORIENTED_EDGE ( 'NONE', *, *, #22908, .F. ) ;
#2269=CYLINDRICAL_SURFACE ( 'NONE', #14293, 3.499999999999999556 ) ;
#2270=ORIENTED_EDGE ( 'NONE', *, *, #19694, .T. ) ;
#2271=EDGE_CURVE ( 'NONE', #24713, #17107, #14982, .T. ) ;
#2274=CARTESIAN_POINT ( 'NONE',  ( -3.310556943750001313, 17.50000000000002132, -127.7641058028994792 ) ) ;
#2275=CARTESIAN_POINT ( 'NONE',  ( -3.500000000000002220, 15.47927405783633326, -102.8776474690881884 ) ) ;
#2277=CARTESIAN_POINT ( 'NONE',  ( -1.655278471874999990, 20.36702641396248481, -40.01827246956612782 ) ) ;
#2278=CARTESIAN_POINT ( 'NONE',  ( -3.310556943750002645, 15.58864905735836537, -31.76827246956613493 ) ) ;
#2279=CARTESIAN_POINT ( 'NONE',  ( 3.310556943749999981, 15.58864905735836892, -91.43493913623279923 ) ) ;
#2280=CARTESIAN_POINT ( 'NONE',  ( -1.750000000000002220, 14.46891108675447413, -25.48806413671075788 ) ) ;
#2281=ORIENTED_EDGE ( 'NONE', *, *, #17448, .F. ) ;
#2283=CARTESIAN_POINT ( 'NONE',  ( 1.655278471874998436, 14.63297358603755249, -136.5182724695661420 ) ) ;
#2286=CARTESIAN_POINT ( 'NONE',  ( 1.749999999999998224, 14.46891108675448656, -132.3213974700441042 ) ) ;
#2287=CARTESIAN_POINT ( 'NONE',  ( 1.750000000000001110, 20.53108891324555429, -81.98806413671074722 ) ) ;
#2288=CARTESIAN_POINT ( 'NONE',  ( 1.655278471874998436, 14.63297358603754184, -65.51827246956614204 ) ) ;
#2291=LINE ( 'NONE', #41858, #25457 ) ;
#2292=CARTESIAN_POINT ( 'NONE',  ( 0.000000000000000000, 21.00000000000002487, -149.5231586289125687 ) ) ;
#2293=ORIENTED_EDGE ( 'NONE', *, *, #9047, .F. ) ;
#2294=CARTESIAN_POINT ( 'NONE',  ( 3.310556943750001313, 17.50000000000002132, -118.2641058028994792 ) ) ;
#2296=EDGE_LOOP ( 'NONE', ( #5660, #1687, #8983, #35625 ) ) ;
#2297=CARTESIAN_POINT ( 'NONE',  ( 1.749999999999998224, 14.46891108675448301, -106.3213974700441042 ) ) ;
#2300=CARTESIAN_POINT ( 'NONE',  ( -0.9378221735089291577, 21.00000000000001421, -68.16632260368298546 ) ) ;
#2301=CARTESIAN_POINT ( 'NONE',  ( 1.750000000000001110, 20.53108891324554719, -37.29431413575484555 ) ) ;
#2304=CARTESIAN_POINT ( 'NONE',  ( 3.310556943749999981, 15.58864905735836714, -72.34743913623280775 ) ) ;
#2305=DIRECTION ( 'NONE',  ( 0.000000000000000000, 1.000000000000000000, 0.000000000000000000 ) ) ;
#2307=( BOUNDED_CURVE ( )  B_SPLINE_CURVE ( 2, ( #12458, #28614, #34376, #22029, #28195, #15022, #41183, #8631, #37776 ),
 .UNSPECIFIED., .F., .F. ) 
 B_SPLINE_CURVE_WITH_KNOTS ( ( 3, 2, 2, 2, 3 ),
 ( 0.04375000000000000416, 0.04444444444444444614, 0.04583333333333333010, 0.04722222222222222099, 0.04791666666666666990 ),
 .UNSPECIFIED. ) 
 CURVE ( )  GEOMETRIC_REPRESENTATION_ITEM ( )  RATIONAL_B_SPLINE_CURVE ( ( 0.9330127018922192983, 0.9330127018922196314, 1.000000000000000000, 0.8660254037844387076, 1.000000000000000000, 0.8660254037844387076, 1.000000000000000000, 0.9330127018922189652, 0.9330127018922192983 ) ) 
 REPRESENTATION_ITEM ( '' )  );
#2309=CARTESIAN_POINT ( 'NONE',  ( 3.500000000000000000, 15.47927405783632615, -72.54431413575483134 ) ) ;
#2312=CARTESIAN_POINT ( 'NONE',  ( -0.9378221735089291577, 21.00000000000002487, -133.1663226036829712 ) ) ;
#2313=CARTESIAN_POINT ( 'NONE',  ( -3.500000000000000000, 19.52072594216371826, -105.0443141357548313 ) ) ;
#2314=CARTESIAN_POINT ( 'NONE',  ( -1.655278471875002211, 14.63297358603754539, -79.59743913623280775 ) ) ;
#2315=ORIENTED_EDGE ( 'NONE', *, *, #8557, .T. ) ;
#2316=ORIENTED_EDGE ( 'NONE', *, *, #39186, .F. ) ;
#2318=ADVANCED_FACE ( 'NONE', ( #3737 ), #32257, .T. ) ;
#2324=CARTESIAN_POINT ( 'NONE',  ( 1.655278471875001101, 20.36702641396248836, -49.18493913623279923 ) ) ;
#2325=CARTESIAN_POINT ( 'NONE',  ( -3.310556943750002645, 15.58864905735837425, -107.7682724695661420 ) ) ;
#2326=EDGE_LOOP ( 'NONE', ( #23177, #31347, #7426, #30093 ) ) ;
#2327=CARTESIAN_POINT ( 'NONE',  ( 3.310556943749999981, 15.58864905735836182, -35.34743913623280775 ) ) ;
#2328=CARTESIAN_POINT ( 'NONE',  ( -7.022189441860112050E-16, 13.67729811471671830, -62.60160580289946353 ) ) ;
#2329=CARTESIAN_POINT ( 'NONE',  ( -3.500000000000001332, 17.50000000000002132, -107.9609808024215027 ) ) ;
#2331=CARTESIAN_POINT ( 'NONE',  ( -1.655278471875002211, 14.63297358603754716, -93.59743913623280775 ) ) ;
#2332=CARTESIAN_POINT ( 'NONE',  ( -3.500000000000000888, 19.52072594216371115, -97.73806413671077564 ) ) ;
#2333=CARTESIAN_POINT ( 'NONE',  ( 4.648177544792955347E-16, 21.00000000000001421, -63.21098080242150274 ) ) ;
#2336=CARTESIAN_POINT ( 'NONE',  ( -1.750000000000002220, 14.46891108675447946, -66.79431413575484555 ) ) ;
#2338=CARTESIAN_POINT ( 'NONE',  ( -1.655278471875002211, 14.63297358603754006, -28.59743913623280420 ) ) ;
#2339=CARTESIAN_POINT ( 'NONE',  ( 3.500000000000001332, 17.50000000000001421, -53.15473080337743284 ) ) ;
#2340=CARTESIAN_POINT ( 'NONE',  ( -1.394453263437886604E-15, 14.00000000000001421, -77.71098080242148853 ) ) ;
#2341=CARTESIAN_POINT ( 'NONE',  ( 3.310556943750001313, 19.41135094264166838, -106.2682724695661278 ) ) ;
#2343=CARTESIAN_POINT ( 'NONE',  ( -3.310556943750002201, 15.58864905735836537, -36.76827246956612782 ) ) ;
#2348=CYLINDRICAL_SURFACE ( 'NONE', #22459, 3.499999999999999556 ) ;
#2350=CARTESIAN_POINT ( 'NONE',  ( -3.310556943750001313, 17.50000000000001776, -85.76410580289947916 ) ) ;
#2352=CARTESIAN_POINT ( 'NONE',  ( -1.749999999999999778, 20.53108891324554719, -25.82139747004409713 ) ) ;
#2353=ORIENTED_EDGE ( 'NONE', *, *, #33385, .F. ) ;
#2355=CARTESIAN_POINT ( 'NONE',  ( 4.648177544792955347E-16, 21.00000000000001066, -26.21098080242150985 ) ) ;
#2356=AXIS2_PLACEMENT_3D ( 'NONE', #37032, #20653, #33631 ) ;
#2359=CARTESIAN_POINT ( 'NONE',  ( 1.655278471875001101, 20.36702641396249192, -95.09743913623280775 ) ) ;
#2362=CARTESIAN_POINT ( 'NONE',  ( 0.000000000000000000, 17.50000000000002487, -149.5231586289125687 ) ) ;
#2364=AXIS2_PLACEMENT_3D ( 'NONE', #21316, #2158, #5566 ) ;
#2365=AXIS2_PLACEMENT_3D ( 'NONE', #25629, #35183, #290 ) ;
#2372=EDGE_CURVE ( 'NONE', #30409, #41237, #20700, .T. ) ;
#2373=CARTESIAN_POINT ( 'NONE',  ( 0.9378221735089213862, 21.00000000000003197, -134.9493890021159075 ) ) ;
#2374=FACE_OUTER_BOUND ( 'NONE', #2407, .T. ) ;
#2375=CARTESIAN_POINT ( 'NONE',  ( -3.310556943750002645, 15.58864905735837780, -134.6807724695661364 ) ) ;
#2376=CARTESIAN_POINT ( 'NONE',  ( 3.500000000000000000, 15.47927405783632615, -78.54431413575483134 ) ) ;
#2379=CARTESIAN_POINT ( 'NONE',  ( 1.655278471875001101, 20.36702641396249547, -123.1849391362327992 ) ) ;
#2380=CARTESIAN_POINT ( 'NONE',  ( 2.340729813953370519E-16, 21.32270188528330834, -50.10160580289946353 ) ) ;
#2381=VERTEX_POINT ( 'NONE', #38900 ) ;
#2383=CARTESIAN_POINT ( 'NONE',  ( -3.500000000000002220, 15.47927405783633503, -137.5713974700441042 ) ) ;
#2386=CARTESIAN_POINT ( 'NONE',  ( -7.022189441860112050E-16, 13.67729811471672186, -77.60160580289947063 ) ) ;
#2387=CARTESIAN_POINT ( 'NONE',  ( 1.749999999999998224, 14.46891108675448656, -130.6276474690881741 ) ) ;
#2388=CARTESIAN_POINT ( 'NONE',  ( 1.655278471875001101, 20.36702641396249547, -108.0974391362328078 ) ) ;
#2389=CYLINDRICAL_SURFACE ( 'NONE', #28849, 3.499999999999999556 ) ;
#2392=CARTESIAN_POINT ( 'NONE',  ( -3.500000000000001332, 17.50000000000001776, -78.96098080242150274 ) ) ;
#2393=CARTESIAN_POINT ( 'NONE',  ( -7.022189441860112050E-16, 13.67729811471671653, -40.51410580289947916 ) ) ;
#2394=CARTESIAN_POINT ( 'NONE',  ( -1.655278471874999990, 20.36702641396249192, -100.0182724695661278 ) ) ;
#2395=CARTESIAN_POINT ( 'NONE',  ( -3.500000000000001332, 17.50000000000002487, -130.6547308033774186 ) ) ;
#2396=CARTESIAN_POINT ( 'NONE',  ( 1.750000000000001110, 20.53108891324554719, -39.29431413575484555 ) ) ;
#2399=CARTESIAN_POINT ( 'NONE',  ( -3.310556943750002201, 15.58864905735837780, -125.7682724695661278 ) ) ;
#2403=CARTESIAN_POINT ( 'NONE',  ( 3.500000000000001332, 19.52072594216370760, -50.37764746908818125 ) ) ;
#2404=CARTESIAN_POINT ( 'NONE',  ( 3.500000000000001332, 19.52072594216371826, -130.0713974700441042 ) ) ;
#2405=CARTESIAN_POINT ( 'NONE',  ( -0.9378221735089291577, 21.00000000000002132, -115.8600726046389013 ) ) ;
#2407=EDGE_LOOP ( 'NONE', ( #4877, #18521, #20401, #29558 ) ) ;
#2408=CARTESIAN_POINT ( 'NONE',  ( -7.022189441860112050E-16, 13.67729811471672186, -75.60160580289944221 ) ) ;
#2409=FACE_OUTER_BOUND ( 'NONE', #24251, .T. ) ;
#2414=CARTESIAN_POINT ( 'NONE',  ( -7.022189441860112050E-16, 13.67729811471671653, -32.51410580289947205 ) ) ;
#2415=CARTESIAN_POINT ( 'NONE',  ( 3.500000000000001332, 19.52072594216370760, -72.07139747004409003 ) ) ;
#2417=ORIENTED_EDGE ( 'NONE', *, *, #32801, .T. ) ;
#2419=CARTESIAN_POINT ( 'NONE',  ( 3.310556943749999981, 15.58864905735836182, -45.34743913623280775 ) ) ;
#2422=CARTESIAN_POINT ( 'NONE',  ( 3.500000000000000000, 15.47927405783632437, -56.23806413671076143 ) ) ;
#2423=CARTESIAN_POINT ( 'NONE',  ( 1.749999999999998224, 14.46891108675447235, -24.62764746908817415 ) ) ;
#2424=PRODUCT ( 'Tension Adjustment Lead Screw Shaft', 'Tension Adjustment Lead Screw Shaft', '', ( #6905 ) ) ;
#2426=( BOUNDED_CURVE ( )  B_SPLINE_CURVE ( 2, ( #19191, #41746, #15590, #35353, #15802, #12390, #32163, #3026, #29373 ),
 .UNSPECIFIED., .F., .T. ) 
 B_SPLINE_CURVE_WITH_KNOTS ( ( 3, 2, 2, 2, 3 ),
 ( 0.9604166666666666963, 0.9611111111111111382, 0.9625000000000000222, 0.9638888888888889062, 0.9645833333333333481 ),
 .UNSPECIFIED. ) 
 CURVE ( )  GEOMETRIC_REPRESENTATION_ITEM ( )  RATIONAL_B_SPLINE_CURVE ( ( 0.9330127018922194093, 0.9330127018922194093, 1.000000000000000000, 0.8660254037844387076, 1.000000000000000000, 0.8660254037844387076, 1.000000000000000000, 0.9330127018922194093, 0.9330127018922194093 ) ) 
 REPRESENTATION_ITEM ( '' )  );
#2427=CARTESIAN_POINT ( 'NONE',  ( -3.500000000000001332, 17.50000000000002132, -104.6547308033774186 ) ) ;
#2428=AXIS2_PLACEMENT_3D ( 'NONE', #23111, #10143, #26522 ) ;
#2429=CARTESIAN_POINT ( 'NONE',  ( -1.394453263437886604E-15, 14.00000000000001066, -43.71098080242150985 ) ) ;
#2430=CARTESIAN_POINT ( 'NONE',  ( 1.749999999999998224, 14.46891108675447590, -40.62764746908817415 ) ) ;
#2432=CARTESIAN_POINT ( 'NONE',  ( 1.750000000000001110, 20.53108891324555429, -82.29431413575483134 ) ) ;
#2433=EDGE_CURVE ( 'NONE', #36594, #20942, #13371, .T. ) ;
#2436=CARTESIAN_POINT ( 'NONE',  ( -1.750000000000002220, 14.46891108675449011, -142.7943141357548313 ) ) ;
#2437=CARTESIAN_POINT ( 'NONE',  ( -1.394453263437886604E-15, 14.00000000000002132, -120.7109808024215170 ) ) ;
#2438=CARTESIAN_POINT ( 'NONE',  ( 3.310556943750001313, 17.50000000000002487, -131.2641058028994507 ) ) ;
#2441=CARTESIAN_POINT ( 'NONE',  ( -0.9378221735089310451, 14.00000000000001599, -76.44938900211593591 ) ) ;
#2442=CARTESIAN_POINT ( 'NONE',  ( -3.310556943750002645, 15.58864905735837780, -114.7682724695661278 ) ) ;
#2443=CARTESIAN_POINT ( 'NONE',  ( 1.749999999999998224, 14.46891108675448656, -134.3213974700441042 ) ) ;
#2444=CARTESIAN_POINT ( 'NONE',  ( 3.500000000000001332, 17.50000000000001066, -38.15473080337743284 ) ) ;
#2445=CARTESIAN_POINT ( 'NONE',  ( -3.500000000000002220, 15.47927405783633503, -121.5713974700441042 ) ) ;
#2447=CARTESIAN_POINT ( 'NONE',  ( -3.310556943750002201, 15.58864905735837958, -139.7682724695661420 ) ) ;
#2450=CARTESIAN_POINT ( 'NONE',  ( 3.310556943750001313, 19.41135094264166483, -51.26827246956612782 ) ) ;
#2452=CARTESIAN_POINT ( 'NONE',  ( 2.340729813953370519E-16, 21.32270188528330834, -72.10160580289947063 ) ) ;
#2454=CARTESIAN_POINT ( 'NONE',  ( 1.655278471875001101, 20.36702641396248836, -70.09743913623280775 ) ) ;
#2456=CARTESIAN_POINT ( 'NONE',  ( 2.340729813953370519E-16, 21.32270188528331190, -92.10160580289947063 ) ) ;
#2457=AXIS2_PLACEMENT_3D ( 'NONE', #2154, #28104, #3211 ) ;
#2460=DIRECTION ( 'NONE',  ( -0.000000000000000000, 1.259100132267607459E-16, -1.000000000000000000 ) ) ;
#2461=CARTESIAN_POINT ( 'NONE',  ( -0.9378221735089291577, 21.00000000000001066, -42.16632260368299256 ) ) ;
#2462=CARTESIAN_POINT ( 'NONE',  ( -7.022189441860112050E-16, 13.67729811471671830, -51.51410580289947205 ) ) ;
#2463=ADVANCED_FACE ( 'NONE', ( #20390 ), #17205, .T. ) ;
#2464=CARTESIAN_POINT ( 'NONE',  ( -0.9378221735089310451, 14.00000000000000888, -24.44938900211595367 ) ) ;
#2465=CARTESIAN_POINT ( 'NONE',  ( 3.310556943750001313, 17.50000000000002132, -113.2641058028994792 ) ) ;
#2467=EDGE_LOOP ( 'NONE', ( #34470, #39231, #32494, #37263 ) ) ;
#2470=VERTEX_POINT ( 'NONE', #4223 ) ;
#2472=CARTESIAN_POINT ( 'NONE',  ( -1.655278471875002211, 14.63297358603754361, -61.59743913623280775 ) ) ;
#2473=ORIENTED_EDGE ( 'NONE', *, *, #24609, .F. ) ;
#2478=DIRECTION ( 'NONE',  ( -0.000000000000000000, 1.259100132267607459E-16, -1.000000000000000000 ) ) ;
#2481=CARTESIAN_POINT ( 'NONE',  ( -3.310556943750001313, 17.50000000000002487, -129.7641058028994507 ) ) ;
#2482=EDGE_CURVE ( 'NONE', #21056, #15782, #19075, .T. ) ;
#2483=CARTESIAN_POINT ( 'NONE',  ( 1.743066579297357930E-14, 14.00000000000002132, -128.4047308033774186 ) ) ;
#2485=CARTESIAN_POINT ( 'NONE',  ( 2.340729813953370519E-16, 21.32270188528330479, -39.10160580289947063 ) ) ;
#2486=CARTESIAN_POINT ( 'NONE',  ( -3.310556943750000425, 19.41135094264165772, -29.93493913623279568 ) ) ;
#2487=CARTESIAN_POINT ( 'NONE',  ( 3.310556943750001313, 19.41135094264166483, -94.26827246956612782 ) ) ;
#2488=CARTESIAN_POINT ( 'NONE',  ( 3.500000000000001332, 17.50000000000001066, -23.15473080337743284 ) ) ;
#2491=CARTESIAN_POINT ( 'NONE',  ( -3.310556943750001313, 17.50000000000002487, -133.8516058028994564 ) ) ;
#2494=CARTESIAN_POINT ( 'NONE',  ( 4.648177544792955347E-16, 21.00000000000001776, -94.90473080337743284 ) ) ;
#2495=CARTESIAN_POINT ( 'NONE',  ( 3.500000000000000000, 15.47927405783632615, -81.23806413671077564 ) ) ;
#2496=CARTESIAN_POINT ( 'NONE',  ( 3.310556943750001313, 17.50000000000001421, -64.35160580289945642 ) ) ;
#2497=( BOUNDED_CURVE ( )  B_SPLINE_CURVE ( 2, ( #3299, #41393, #3099, #15876, #22659, #6497, #12879, #15450, #16091 ),
 .UNSPECIFIED., .F., .F. ) 
 B_SPLINE_CURVE_WITH_KNOTS ( ( 3, 2, 2, 2, 3 ),
 ( 0.3895833333333333370, 0.3902777777777777790, 0.3916666666666666630, 0.3930555555555555469, 0.3937499999999999889 ),
 .UNSPECIFIED. ) 
 CURVE ( )  GEOMETRIC_REPRESENTATION_ITEM ( )  RATIONAL_B_SPLINE_CURVE ( ( 0.9330127018922194093, 0.9330127018922194093, 1.000000000000000000, 0.8660254037844387076, 1.000000000000000000, 0.8660254037844387076, 1.000000000000000000, 0.9330127018922194093, 0.9330127018922194093 ) ) 
 REPRESENTATION_ITEM ( '' )  );
#2500=DIRECTION ( 'NONE',  ( 0.000000000000000000, 1.000000000000000000, 0.000000000000000000 ) ) ;
#2502=ORIENTED_EDGE ( 'NONE', *, *, #28510, .T. ) ;
#2503=CARTESIAN_POINT ( 'NONE',  ( -3.310556943750001313, 17.50000000000002132, -113.7641058028994792 ) ) ;
#2504=CARTESIAN_POINT ( 'NONE',  ( -1.394453263437886604E-15, 14.00000000000002132, -124.7109808024214885 ) ) ;
#2506=VERTEX_POINT ( 'NONE', #39520 ) ;
#2507=CARTESIAN_POINT ( 'NONE',  ( 3.500000000000001332, 17.50000000000002132, -109.1547308033774186 ) ) ;
#2508=CARTESIAN_POINT ( 'NONE',  ( -3.500000000000001332, 17.50000000000002487, -139.9609808024215170 ) ) ;
#2510=CARTESIAN_POINT ( 'NONE',  ( 3.500000000000001332, 17.50000000000001421, -59.15473080337743994 ) ) ;
#2512=CARTESIAN_POINT ( 'NONE',  ( 3.310556943750001313, 19.41135094264166483, -73.18077246956613635 ) ) ;
#2514=ADVANCED_FACE ( 'NONE', ( #23592 ), #32511, .T. ) ;
#2516=DIRECTION ( 'NONE',  ( -0.000000000000000000, 1.259100132267607459E-16, -1.000000000000000000 ) ) ;
#2518=CARTESIAN_POINT ( 'NONE',  ( 0.000000000000000000, 17.50000000000002487, -149.5231586289125687 ) ) ;
#2519=ORIENTED_EDGE ( 'NONE', *, *, #12891, .T. ) ;
#2520=CARTESIAN_POINT ( 'NONE',  ( 4.648177544792955347E-16, 21.00000000000002132, -104.2109808024215027 ) ) ;
#2522=CARTESIAN_POINT ( 'NONE',  ( -1.655278471874999990, 20.36702641396249192, -80.93077246956615056 ) ) ;
#2525=CARTESIAN_POINT ( 'NONE',  ( -1.749999999999999778, 20.53108891324555785, -128.1276474690881741 ) ) ;
#2527=CARTESIAN_POINT ( 'NONE',  ( 0.9378221735089213862, 21.00000000000002487, -128.9493890021159359 ) ) ;
#2528=CYLINDRICAL_SURFACE ( 'NONE', #19365, 3.499999999999999556 ) ;
#2529=CARTESIAN_POINT ( 'NONE',  ( 3.310556943749999981, 15.58864905735836182, -45.43493913623279212 ) ) ;
#2530=CARTESIAN_POINT ( 'NONE',  ( -3.310556943750001313, 17.50000000000002132, -109.8516058028994564 ) ) ;
#2531=ORIENTED_EDGE ( 'NONE', *, *, #31848, .T. ) ;
#2532=ADVANCED_FACE ( 'NONE', ( #35911 ), #12956, .T. ) ;
#2533=CARTESIAN_POINT ( 'NONE',  ( -3.310556943750002645, 15.58864905735836537, -32.68077246956614346 ) ) ;
#2534=CARTESIAN_POINT ( 'NONE',  ( -1.655278471874999990, 20.36702641396248836, -60.01827246956613493 ) ) ;
#2535=CARTESIAN_POINT ( 'NONE',  ( -1.749999999999999778, 20.53108891324555785, -105.1276474690881741 ) ) ;
#2536=EDGE_CURVE ( 'NONE', #40555, #6853, #19750, .T. ) ;
#2538=CARTESIAN_POINT ( 'NONE',  ( -3.310556943750001313, 17.50000000000001776, -93.76410580289947916 ) ) ;
#2539=CARTESIAN_POINT ( 'NONE',  ( -3.500000000000002220, 15.47927405783632970, -95.57139747004409003 ) ) ;
#2540=DIRECTION ( 'NONE',  ( 0.000000000000000000, 1.000000000000000000, 0.000000000000000000 ) ) ;
#2541=CARTESIAN_POINT ( 'NONE',  ( -3.500000000000001332, 17.50000000000001421, -56.65473080337743284 ) ) ;
#2543=CARTESIAN_POINT ( 'NONE',  ( 3.500000000000001332, 17.50000000000001421, -59.46098080242151696 ) ) ;
#2544=CARTESIAN_POINT ( 'NONE',  ( -1.394453263437886604E-15, 14.00000000000002132, -115.7109808024214885 ) ) ;
#2545=CARTESIAN_POINT ( 'NONE',  ( 3.310556943750001313, 17.50000000000001066, -27.26410580289947916 ) ) ;
#2547=CARTESIAN_POINT ( 'NONE',  ( -1.750000000000002220, 14.46891108675447768, -46.48806413671076143 ) ) ;
#2549=CARTESIAN_POINT ( 'NONE',  ( -3.310556943750002201, 15.58864905735837780, -109.7682724695661420 ) ) ;
#2550=CARTESIAN_POINT ( 'NONE',  ( -3.310556943750001313, 17.50000000000001066, -33.85160580289946353 ) ) ;
#2553=CARTESIAN_POINT ( 'NONE',  ( 4.648177544792955347E-16, 21.00000000000001421, -57.21098080242150274 ) ) ;
#2554=EDGE_CURVE ( 'NONE', #23350, #41433, #39951, .T. ) ;
#2558=CARTESIAN_POINT ( 'NONE',  ( 1.655278471875001101, 20.36702641396249192, -89.09743913623280775 ) ) ;
#2560=CARTESIAN_POINT ( 'NONE',  ( 3.500000000000001332, 17.50000000000001066, -23.15473080337743284 ) ) ;
#2563=CARTESIAN_POINT ( 'NONE',  ( 3.500000000000001332, 17.50000000000002132, -109.4609808024215027 ) ) ;
#2567=CARTESIAN_POINT ( 'NONE',  ( 3.310556943749999981, 15.58864905735837070, -96.34743913623280775 ) ) ;
#2570=DIRECTION ( 'NONE',  ( 0.000000000000000000, 1.000000000000000000, 0.000000000000000000 ) ) ;
#2577=CARTESIAN_POINT ( 'NONE',  ( 1.749999999999998224, 14.46891108675448478, -109.3213974700441042 ) ) ;
#2579=CARTESIAN_POINT ( 'NONE',  ( 1.655278471875001101, 20.36702641396249902, -138.0974391362327935 ) ) ;
#2581=ORIENTED_EDGE ( 'NONE', *, *, #38377, .F. ) ;
#2582=CARTESIAN_POINT ( 'NONE',  ( -3.500000000000002220, 15.47927405783633503, -140.8776474690881741 ) ) ;
#2583=CARTESIAN_POINT ( 'NONE',  ( 3.310556943750001313, 19.41135094264166838, -124.2682724695661278 ) ) ;
#2584=CARTESIAN_POINT ( 'NONE',  ( 3.310556943749999981, 15.58864905735836182, -49.43493913623279212 ) ) ;
#2585=ORIENTED_EDGE ( 'NONE', *, *, #40135, .F. ) ;
#2586=CARTESIAN_POINT ( 'NONE',  ( 2.474675557024783212E-16, 21.54145188432740810, -135.9047308033774186 ) ) ;
#2589=CARTESIAN_POINT ( 'NONE',  ( 3.310556943750001313, 17.50000000000001776, -78.35160580289945642 ) ) ;
#2590=CARTESIAN_POINT ( 'NONE',  ( -3.500000000000000888, 19.52072594216371826, -122.0443141357548456 ) ) ;
#2591=CARTESIAN_POINT ( 'NONE',  ( 2.340729813953370519E-16, 21.32270188528331900, -107.0141058028994649 ) ) ;
#2594=CARTESIAN_POINT ( 'NONE',  ( 3.500000000000000000, 15.47927405783632437, -72.54431413575484555 ) ) ;
#2595=CARTESIAN_POINT ( 'NONE',  ( 0.000000000000000000, 21.00000000000002487, -149.5231586289125687 ) ) ;
#2596=CARTESIAN_POINT ( 'NONE',  ( 3.310556943750001313, 19.41135094264165772, -40.18077246956614346 ) ) ;
#2597=CARTESIAN_POINT ( 'NONE',  ( 3.310556943750001313, 19.41135094264166483, -101.2682724695661278 ) ) ;
#2598=CARTESIAN_POINT ( 'NONE',  ( -1.750000000000002220, 14.46891108675448301, -82.79431413575483134 ) ) ;
#2599=CARTESIAN_POINT ( 'NONE',  ( 3.500000000000001332, 17.50000000000001421, -63.15473080337742573 ) ) ;
#2602=CARTESIAN_POINT ( 'NONE',  ( 3.310556943749999981, 15.58864905735837247, -121.4349391362327992 ) ) ;
#2607=DIRECTION ( 'NONE',  ( 0.000000000000000000, 1.000000000000000000, 0.000000000000000000 ) ) ;
#2613=CARTESIAN_POINT ( 'NONE',  ( 3.310556943750001313, 19.41135094264166483, -73.26827246956612782 ) ) ;
#2614=DIRECTION ( 'NONE',  ( -0.000000000000000000, 1.259100132267607459E-16, -1.000000000000000000 ) ) ;
#2615=CARTESIAN_POINT ( 'NONE',  ( 3.500000000000001332, 17.50000000000001066, -45.15473080337743994 ) ) ;
#2616=CARTESIAN_POINT ( 'NONE',  ( -3.500000000000002220, 15.47927405783632615, -55.87764746908817415 ) ) ;
#2618=DIRECTION ( 'NONE',  ( -0.000000000000000000, 1.259100132267607459E-16, -1.000000000000000000 ) ) ;
#2620=CARTESIAN_POINT ( 'NONE',  ( 3.310556943750001313, 17.50000000000001066, -35.26410580289947205 ) ) ;
#2623=VERTEX_POINT ( 'NONE', #1250 ) ;
#2625=CARTESIAN_POINT ( 'NONE',  ( 3.310556943750001313, 19.41135094264166128, -48.18077246956614346 ) ) ;
#2627=ORIENTED_EDGE ( 'NONE', *, *, #4668, .T. ) ;
#2629=DIRECTION ( 'NONE',  ( -0.000000000000000000, 1.259100132267607459E-16, -1.000000000000000000 ) ) ;
#2633=CARTESIAN_POINT ( 'NONE',  ( -7.424026671074350129E-16, 13.45854811567263098, -35.71098080242150985 ) ) ;
#2635=ORIENTED_EDGE ( 'NONE', *, *, #9086, .T. ) ;
#2640=CARTESIAN_POINT ( 'NONE',  ( -7.424026671074350129E-16, 13.45854811567264164, -141.7109808024214885 ) ) ;
#2641=CARTESIAN_POINT ( 'NONE',  ( -1.394453263437886604E-15, 14.00000000000001421, -57.40473080337742573 ) ) ;
#2642=CARTESIAN_POINT ( 'NONE',  ( 1.655278471875001101, 20.36702641396249547, -123.0974391362328078 ) ) ;
#2645=DIRECTION ( 'NONE',  ( -0.8660254037844367092, -0.000000000000000000, 0.5000000000000034417 ) ) ;
#2646=CARTESIAN_POINT ( 'NONE',  ( -3.500000000000000888, 19.52072594216371115, -96.04431413575483134 ) ) ;
#2647=CARTESIAN_POINT ( 'NONE',  ( -3.310556943750002645, 15.58864905735837780, -117.7682724695661420 ) ) ;
#2648=FACE_OUTER_BOUND ( 'NONE', #33271, .T. ) ;
#2649=CARTESIAN_POINT ( 'NONE',  ( 3.500000000000001332, 17.50000000000001066, -35.15473080337742573 ) ) ;
#2650=CARTESIAN_POINT ( 'NONE',  ( 4.648177544792955347E-16, 21.00000000000002132, -121.9047308033774044 ) ) ;
#2652=CARTESIAN_POINT ( 'NONE',  ( -7.022189441860112050E-16, 13.67729811471673074, -138.6016058028994564 ) ) ;
#2656=CARTESIAN_POINT ( 'NONE',  ( -1.655278471875002211, 14.63297358603754184, -47.68493913623279923 ) ) ;
#2658=CARTESIAN_POINT ( 'NONE',  ( -3.500000000000000000, 19.52072594216370405, -41.73806413671076143 ) ) ;
#2659=CARTESIAN_POINT ( 'NONE',  ( -7.022189441860112050E-16, 13.67729811471672186, -71.60160580289947063 ) ) ;
#2661=CARTESIAN_POINT ( 'NONE',  ( 3.310556943749999981, 15.58864905735836714, -70.34743913623280775 ) ) ;
#2663=CARTESIAN_POINT ( 'NONE',  ( 1.655278471875001101, 20.36702641396249192, -91.18493913623279923 ) ) ;
#2665=CARTESIAN_POINT ( 'NONE',  ( -1.394453263437886604E-15, 14.00000000000002132, -121.4047308033774328 ) ) ;
#2666=CARTESIAN_POINT ( 'NONE',  ( -3.500000000000002220, 15.47927405783633326, -105.8776474690881741 ) ) ;
#2668=CARTESIAN_POINT ( 'NONE',  ( 2.340729813953370519E-16, 21.32270188528331190, -50.01410580289946495 ) ) ;
#2669=EDGE_CURVE ( 'NONE', #40609, #25349, #10390, .T. ) ;
#2671=CARTESIAN_POINT ( 'NONE',  ( -3.310556943750000425, 19.41135094264166838, -104.8474391362328078 ) ) ;
#2674=ORIENTED_EDGE ( 'NONE', *, *, #38832, .T. ) ;
#2675=( BOUNDED_CURVE ( )  B_SPLINE_CURVE ( 2, ( #16381, #32524, #616, #26365, #10627, #39758, #27004, #1057, #36131 ),
 .UNSPECIFIED., .F., .F. ) 
 B_SPLINE_CURVE_WITH_KNOTS ( ( 3, 2, 2, 2, 3 ),
 ( 0.5645833333333333259, 0.5652777777777777679, 0.5666666666666666519, 0.5680555555555555358, 0.5687499999999999778 ),
 .UNSPECIFIED. ) 
 CURVE ( )  GEOMETRIC_REPRESENTATION_ITEM ( )  RATIONAL_B_SPLINE_CURVE ( ( 0.9330127018922194093, 0.9330127018922194093, 1.000000000000000000, 0.8660254037844387076, 1.000000000000000000, 0.8660254037844387076, 1.000000000000000000, 0.9330127018922194093, 0.9330127018922194093 ) ) 
 REPRESENTATION_ITEM ( '' )  );
#2680=CARTESIAN_POINT ( 'NONE',  ( -1.655278471874999990, 20.36702641396248836, -63.93077246956614346 ) ) ;
#2684=AXIS2_PLACEMENT_3D ( 'NONE', #33925, #30096, #37329 ) ;
#2685=DIRECTION ( 'NONE',  ( -0.000000000000000000, 1.259100132267607459E-16, -1.000000000000000000 ) ) ;
#2687=CYLINDRICAL_SURFACE ( 'NONE', #11566, 3.499999999999999556 ) ;
#2690=CARTESIAN_POINT ( 'NONE',  ( 1.655278471874998436, 14.63297358603755072, -124.4307724695661364 ) ) ;
#2691=CARTESIAN_POINT ( 'NONE',  ( 3.310556943749999981, 15.58864905735836182, -38.43493913623279923 ) ) ;
#2692=CARTESIAN_POINT ( 'NONE',  ( -3.310556943750001313, 17.50000000000001066, -27.85160580289947063 ) ) ;
#2693=CARTESIAN_POINT ( 'NONE',  ( -7.022189441860112050E-16, 13.67729811471672363, -85.60160580289947063 ) ) ;
#2694=CARTESIAN_POINT ( 'NONE',  ( -1.655278471875002211, 14.63297358603755427, -139.5974391362327935 ) ) ;
#2696=ADVANCED_FACE ( 'NONE', ( #8249 ), #30590, .T. ) ;
#2699=CARTESIAN_POINT ( 'NONE',  ( 1.655278471874998436, 14.63297358603755072, -133.5182724695661420 ) ) ;
#2702=AXIS2_PLACEMENT_3D ( 'NONE', #35781, #36412, #29601 ) ;
#2703=CARTESIAN_POINT ( 'NONE',  ( -1.394453263437886604E-15, 14.00000000000001776, -84.40473080337743284 ) ) ;
#2704=CARTESIAN_POINT ( 'NONE',  ( 4.648177544792955347E-16, 21.00000000000001421, -52.21098080242150985 ) ) ;
#2705=CARTESIAN_POINT ( 'NONE',  ( -3.500000000000000888, 19.52072594216371115, -82.73806413671074722 ) ) ;
#2706=CARTESIAN_POINT ( 'NONE',  ( 3.310556943750001313, 19.41135094264166483, -63.26827246956613493 ) ) ;
#2709=DIRECTION ( 'NONE',  ( -0.000000000000000000, 1.259100132267607459E-16, -1.000000000000000000 ) ) ;
#2710=CARTESIAN_POINT ( 'NONE',  ( -1.655278471874999990, 20.36702641396249192, -83.01827246956614204 ) ) ;
#2711=CARTESIAN_POINT ( 'NONE',  ( -3.500000000000002220, 15.47927405783632437, -47.87764746908818125 ) ) ;
#2712=CARTESIAN_POINT ( 'NONE',  ( 3.310556943750001313, 19.41135094264166838, -114.1807724695661364 ) ) ;
#2713=FACE_OUTER_BOUND ( 'NONE', #41825, .T. ) ;
#2717=CARTESIAN_POINT ( 'NONE',  ( 3.500000000000001332, 17.50000000000002132, -110.1547308033774328 ) ) ;
#2719=CARTESIAN_POINT ( 'NONE',  ( -1.749999999999999778, 20.53108891324555429, -82.82139747004410424 ) ) ;
#2720=CARTESIAN_POINT ( 'NONE',  ( 4.648177544792955347E-16, 21.00000000000001066, -27.21098080242150985 ) ) ;
#2723=CARTESIAN_POINT ( 'NONE',  ( 1.655278471875001101, 20.36702641396248836, -65.09743913623280775 ) ) ;
#2724=CARTESIAN_POINT ( 'NONE',  ( 3.500000000000000000, 15.47927405783632437, -59.54431413575483845 ) ) ;
#2729=ORIENTED_EDGE ( 'NONE', *, *, #38846, .F. ) ;
#2730=CARTESIAN_POINT ( 'NONE',  ( -1.394453263437886604E-15, 14.00000000000001776, -92.71098080242150274 ) ) ;
#2732=CARTESIAN_POINT ( 'NONE',  ( -3.310556943750001313, 17.50000000000001776, -79.76410580289946495 ) ) ;
#2733=VERTEX_POINT ( 'NONE', #24636 ) ;
#2735=CARTESIAN_POINT ( 'NONE',  ( -0.9378221735089291577, 21.00000000000001421, -53.86007260463891555 ) ) ;
#2738=VECTOR ( 'NONE', #22249, 1000.000000000000000 ) ;
#2739=CARTESIAN_POINT ( 'NONE',  ( -3.500000000000001332, 17.50000000000002132, -113.6547308033774328 ) ) ;
#2740=CARTESIAN_POINT ( 'NONE',  ( -1.655278471875002211, 14.63297358603754184, -44.68493913623279923 ) ) ;
#2741=CARTESIAN_POINT ( 'NONE',  ( -1.655278471874999990, 20.36702641396249547, -110.0182724695661420 ) ) ;
#2743=( BOUNDED_CURVE ( )  B_SPLINE_CURVE ( 2, ( #6516, #16106, #23087, #42044, #26709, #6299, #23305, #13513, #758 ),
 .UNSPECIFIED., .F., .T. ) 
 B_SPLINE_CURVE_WITH_KNOTS ( ( 3, 2, 2, 2, 3 ),
 ( 0.4062500000000000000, 0.4069444444444444420, 0.4083333333333333259, 0.4097222222222222099, 0.4104166666666666519 ),
 .UNSPECIFIED. ) 
 CURVE ( )  GEOMETRIC_REPRESENTATION_ITEM ( )  RATIONAL_B_SPLINE_CURVE ( ( 0.9330127018922194093, 0.9330127018922194093, 1.000000000000000000, 0.8660254037844387076, 1.000000000000000000, 0.8660254037844387076, 1.000000000000000000, 0.9330127018922194093, 0.9330127018922194093 ) ) 
 REPRESENTATION_ITEM ( '' )  );
#2745=CARTESIAN_POINT ( 'NONE',  ( 1.655278471874998436, 14.63297358603753828, -30.43077246956614346 ) ) ;
#2746=CARTESIAN_POINT ( 'NONE',  ( 1.655278471874998436, 14.63297358603754184, -61.51827246956613493 ) ) ;
#2747=CARTESIAN_POINT ( 'NONE',  ( -1.750000000000002220, 14.46891108675448478, -104.7943141357548313 ) ) ;
#2749=CARTESIAN_POINT ( 'NONE',  ( -1.749999999999999778, 20.53108891324555429, -97.82139747004409003 ) ) ;
#2750=CARTESIAN_POINT ( 'NONE',  ( 4.648177544792955347E-16, 21.00000000000002487, -141.2109808024214885 ) ) ;
#2753=CARTESIAN_POINT ( 'NONE',  ( -1.750000000000002220, 14.46891108675447946, -56.79431413575483845 ) ) ;
#2756=CARTESIAN_POINT ( 'NONE',  ( 3.310556943749999981, 15.58864905735836004, -25.34743913623280420 ) ) ;
#2757=CARTESIAN_POINT ( 'NONE',  ( 1.749999999999998224, 14.46891108675447590, -48.32139747004410424 ) ) ;
#2758=CARTESIAN_POINT ( 'NONE',  ( 3.500000000000001332, 17.50000000000001776, -77.46098080242150274 ) ) ;
#2759=CARTESIAN_POINT ( 'NONE',  ( 1.655278471875001101, 20.36702641396248481, -34.18493913623279923 ) ) ;
#2761=CARTESIAN_POINT ( 'NONE',  ( 0.000000000000000000, 21.00000000000002487, -149.5231586289125687 ) ) ;
#2764=CARTESIAN_POINT ( 'NONE',  ( 4.648177544792955347E-16, 21.00000000000001421, -65.90473080337741862 ) ) ;
#2766=CARTESIAN_POINT ( 'NONE',  ( 2.340729813953370519E-16, 21.32270188528331190, -83.01410580289947916 ) ) ;
#2767=VERTEX_POINT ( 'NONE', #8044 ) ;
#2771=AXIS2_PLACEMENT_3D ( 'NONE', #33720, #4571, #33281 ) ;
#2776=CARTESIAN_POINT ( 'NONE',  ( -7.022189441860112050E-16, 13.67729811471672541, -97.51410580289947916 ) ) ;
#2778=ORIENTED_EDGE ( 'NONE', *, *, #5392, .F. ) ;
#2779=CARTESIAN_POINT ( 'NONE',  ( 4.648177544792955347E-16, 21.00000000000002132, -128.2109808024214885 ) ) ;
#2781=CARTESIAN_POINT ( 'NONE',  ( 0.9378221735089300459, 21.00000000000002487, -139.2556390011600342 ) ) ;
#2782=EDGE_CURVE ( 'NONE', #20830, #15608, #20445, .T. ) ;
#2788=ORIENTED_EDGE ( 'NONE', *, *, #25102, .F. ) ;
#2790=DIRECTION ( 'NONE',  ( -0.000000000000000000, 1.259100132267607459E-16, -1.000000000000000000 ) ) ;
#2791=DIRECTION ( 'NONE',  ( -0.000000000000000000, 1.259100132267607459E-16, -1.000000000000000000 ) ) ;
#2792=CARTESIAN_POINT ( 'NONE',  ( 3.310556943750001313, 17.50000000000002487, -130.2641058028994507 ) ) ;
#2795=CARTESIAN_POINT ( 'NONE',  ( 1.749999999999998224, 14.46891108675447413, -28.62764746908817770 ) ) ;
#2796=CARTESIAN_POINT ( 'NONE',  ( -7.022189441860112050E-16, 13.67729811471672718, -126.6016058028994848 ) ) ;
#2797=CARTESIAN_POINT ( 'NONE',  ( -1.655278471874999990, 20.36702641396248836, -53.01827246956612782 ) ) ;
#2799=CARTESIAN_POINT ( 'NONE',  ( -1.749999999999999778, 20.53108891324555785, -128.8213974700441042 ) ) ;
#2800=( BOUNDED_CURVE ( )  B_SPLINE_CURVE ( 2, ( #31323, #2182, #18145, #33892, #11541, #28129, #11750, #24956, #4751 ),
 .UNSPECIFIED., .F., .T. ) 
 B_SPLINE_CURVE_WITH_KNOTS ( ( 3, 2, 2, 2, 3 ),
 ( 0.5854166666666666963, 0.5861111111111111382, 0.5875000000000000222, 0.5888888888888889062, 0.5895833333333333481 ),
 .UNSPECIFIED. ) 
 CURVE ( )  GEOMETRIC_REPRESENTATION_ITEM ( )  RATIONAL_B_SPLINE_CURVE ( ( 0.9330127018922194093, 0.9330127018922194093, 1.000000000000000000, 0.8660254037844387076, 1.000000000000000000, 0.8660254037844387076, 1.000000000000000000, 0.9330127018922194093, 0.9330127018922194093 ) ) 
 REPRESENTATION_ITEM ( '' )  );
#2804=CARTESIAN_POINT ( 'NONE',  ( 1.655278471875001101, 20.36702641396249192, -76.18493913623279923 ) ) ;
#2805=CARTESIAN_POINT ( 'NONE',  ( -3.500000000000000888, 19.52072594216371826, -121.0443141357548598 ) ) ;
#2806=CARTESIAN_POINT ( 'NONE',  ( -1.655278471874999990, 20.36702641396249547, -107.9307724695661506 ) ) ;
#2807=CARTESIAN_POINT ( 'NONE',  ( 0.9378221735089300459, 21.00000000000001776, -92.94938900211593591 ) ) ;
#2810=CARTESIAN_POINT ( 'NONE',  ( 3.500000000000001776, 19.52072594216370760, -74.37764746908817415 ) ) ;
#2812=CARTESIAN_POINT ( 'NONE',  ( 3.310556943750001313, 17.50000000000001066, -41.26410580289947916 ) ) ;
#2813=CARTESIAN_POINT ( 'NONE',  ( -3.310556943750000425, 19.41135094264166483, -99.93493913623281344 ) ) ;
#2814=CARTESIAN_POINT ( 'NONE',  ( 1.750000000000001110, 20.53108891324555074, -73.29431413575483134 ) ) ;
#2815=CARTESIAN_POINT ( 'NONE',  ( 3.500000000000001776, 19.52072594216370760, -67.07139747004409003 ) ) ;
#2817=ORIENTED_EDGE ( 'NONE', *, *, #21766, .F. ) ;
#2818=CARTESIAN_POINT ( 'NONE',  ( 2.340729813953370519E-16, 21.32270188528331900, -116.1016058028994564 ) ) ;
#2821=CARTESIAN_POINT ( 'NONE',  ( 3.500000000000000000, 15.47927405783632082, -32.23806413671076143 ) ) ;
#2826=CARTESIAN_POINT ( 'NONE',  ( -3.310556943750002201, 15.58864905735837070, -76.76827246956612782 ) ) ;
#2829=CARTESIAN_POINT ( 'NONE',  ( -1.394453263437886604E-15, 14.00000000000002132, -122.4047308033774044 ) ) ;
#2832=CARTESIAN_POINT ( 'NONE',  ( 1.655278471874998436, 14.63297358603753828, -34.43077246956615056 ) ) ;
#2833=CARTESIAN_POINT ( 'NONE',  ( 0.000000000000000000, 17.50000000000002487, -149.5231586289125687 ) ) ;
#2843=CARTESIAN_POINT ( 'NONE',  ( 1.749999999999998224, 14.46891108675448834, -140.6276474690881741 ) ) ;
#2844=CARTESIAN_POINT ( 'NONE',  ( -1.750000000000002220, 14.46891108675448656, -117.4880641367107614 ) ) ;
#2846=LINE ( 'NONE', #15836, #27486 ) ;
#2847=CARTESIAN_POINT ( 'NONE',  ( 3.500000000000000000, 15.47927405783632082, -35.54431413575484555 ) ) ;
#2848=CARTESIAN_POINT ( 'NONE',  ( -1.394453263437886604E-15, 14.00000000000001776, -88.40473080337740441 ) ) ;
#2849=CARTESIAN_POINT ( 'NONE',  ( 1.750000000000001110, 20.53108891324555074, -70.29431413575484555 ) ) ;
#2850=CARTESIAN_POINT ( 'NONE',  ( 0.9378221735089300459, 21.00000000000002132, -105.9493890021159501 ) ) ;
#2852=CARTESIAN_POINT ( 'NONE',  ( -3.500000000000000888, 19.52072594216372181, -137.0443141357548598 ) ) ;
#2853=CARTESIAN_POINT ( 'NONE',  ( 3.500000000000000000, 15.47927405783633326, -120.5443141357548171 ) ) ;
#2854=CARTESIAN_POINT ( 'NONE',  ( 3.310556943750001313, 19.41135094264166838, -124.1807724695661364 ) ) ;
#2858=CARTESIAN_POINT ( 'NONE',  ( 2.474675557024783212E-16, 21.54145188432739744, -92.21098080242151696 ) ) ;
#2860=CARTESIAN_POINT ( 'NONE',  ( 3.310556943750001313, 17.50000000000001421, -61.26410580289946495 ) ) ;
#2861=CARTESIAN_POINT ( 'NONE',  ( -3.310556943750002645, 15.58864905735837780, -116.7682724695661278 ) ) ;
#2863=CARTESIAN_POINT ( 'NONE',  ( -3.500000000000002220, 15.47927405783632082, -34.57139747004410424 ) ) ;
#2866=CARTESIAN_POINT ( 'NONE',  ( 3.310556943750001313, 17.50000000000002487, -140.3516058028994564 ) ) ;
#2868=CARTESIAN_POINT ( 'NONE',  ( 0.9378221735089260491, 21.00000000000002842, -137.9493890021159928 ) ) ;
#2869=CARTESIAN_POINT ( 'NONE',  ( 1.655278471875001101, 20.36702641396248836, -49.18493913623279923 ) ) ;
#2871=CARTESIAN_POINT ( 'NONE',  ( 4.648177544792955347E-16, 21.00000000000001066, -41.90473080337742573 ) ) ;
#2872=CARTESIAN_POINT ( 'NONE',  ( -7.022189441860112050E-16, 13.67729811471672186, -68.60160580289945642 ) ) ;
#2874=CARTESIAN_POINT ( 'NONE',  ( -7.022189441860112050E-16, 13.67729811471672186, -68.51410580289947916 ) ) ;
#2876=CARTESIAN_POINT ( 'NONE',  ( 3.310556943749999981, 15.58864905735836892, -89.43493913623278502 ) ) ;
#2879=FACE_OUTER_BOUND ( 'NONE', #34439, .T. ) ;
#2882=CARTESIAN_POINT ( 'NONE',  ( 3.310556943750001313, 17.50000000000001421, -50.26410580289947205 ) ) ;
#2885=CARTESIAN_POINT ( 'NONE',  ( 1.655278471874998436, 14.63297358603754716, -104.4307724695661364 ) ) ;
#2886=ORIENTED_EDGE ( 'NONE', *, *, #13735, .T. ) ;
#2891=CARTESIAN_POINT ( 'NONE',  ( 1.655278471874998436, 14.63297358603754184, -55.43077246956613635 ) ) ;
#2897=FACE_OUTER_BOUND ( 'NONE', #17691, .T. ) ;
#2898=EDGE_CURVE ( 'NONE', #11548, #21198, #312, .T. ) ;
#2899=ORIENTED_EDGE ( 'NONE', *, *, #29730, .F. ) ;
#2900=CARTESIAN_POINT ( 'NONE',  ( -3.500000000000002220, 15.47927405783632615, -54.87764746908817415 ) ) ;
#2901=CARTESIAN_POINT ( 'NONE',  ( -1.655278471875002211, 14.63297358603755072, -122.5974391362328078 ) ) ;
#2903=VECTOR ( 'NONE', #10498, 1000.000000000000000 ) ;
#2905=CARTESIAN_POINT ( 'NONE',  ( 3.310556943750001313, 19.41135094264165772, -32.26827246956613493 ) ) ;
#2906=CARTESIAN_POINT ( 'NONE',  ( -3.310556943750000425, 19.41135094264165772, -26.93493913623279568 ) ) ;
#2908=CARTESIAN_POINT ( 'NONE',  ( 3.310556943749999981, 15.58864905735836892, -89.43493913623278502 ) ) ;
#2909=CARTESIAN_POINT ( 'NONE',  ( 2.340729813953370519E-16, 21.32270188528332255, -137.0141058028994792 ) ) ;
#2913=CARTESIAN_POINT ( 'NONE',  ( -1.655278471875002211, 14.63297358603755249, -134.6849391362327992 ) ) ;
#2914=CARTESIAN_POINT ( 'NONE',  ( 4.648177544792955347E-16, 21.00000000000001421, -69.90473080337741862 ) ) ;
#2918=CARTESIAN_POINT ( 'NONE',  ( -1.750000000000002220, 14.46891108675448123, -80.48806413671076143 ) ) ;
#2919=CARTESIAN_POINT ( 'NONE',  ( 1.655278471875001101, 20.36702641396248836, -62.18493913623279923 ) ) ;
#2923=CARTESIAN_POINT ( 'NONE',  ( -1.655278471874999990, 20.36702641396249192, -86.01827246956612782 ) ) ;
#2924=CARTESIAN_POINT ( 'NONE',  ( 1.655278471875001101, 20.36702641396249547, -113.0974391362328078 ) ) ;
#2926=( BOUNDED_CURVE ( )  B_SPLINE_CURVE ( 2, ( #18382, #11991, #21779, #41984, #31975, #13042, #39187, #16244, #6455 ),
 .UNSPECIFIED., .F., .T. ) 
 B_SPLINE_CURVE_WITH_KNOTS ( ( 3, 2, 2, 2, 3 ),
 ( 0.1937500000000000056, 0.1944444444444444475, 0.1958333333333333315, 0.1972222222222222154, 0.1979166666666666574 ),
 .UNSPECIFIED. ) 
 CURVE ( )  GEOMETRIC_REPRESENTATION_ITEM ( )  RATIONAL_B_SPLINE_CURVE ( ( 0.9330127018922194093, 0.9330127018922194093, 1.000000000000000000, 0.8660254037844387076, 1.000000000000000000, 0.8660254037844387076, 1.000000000000000000, 0.9330127018922194093, 0.9330127018922194093 ) ) 
 REPRESENTATION_ITEM ( '' )  );
#2928=ORIENTED_EDGE ( 'NONE', *, *, #24556, .T. ) ;
#2929=CARTESIAN_POINT ( 'NONE',  ( -1.750000000000002220, 14.46891108675448478, -108.4880641367107614 ) ) ;
#2930=CARTESIAN_POINT ( 'NONE',  ( -1.749999999999999778, 20.53108891324556140, -140.1276474690881741 ) ) ;
#2931=( BOUNDED_CURVE ( )  B_SPLINE_CURVE ( 2, ( #4541, #1354, #17520, #19855, #40684, #24531, #12168, #33889, #28334 ),
 .UNSPECIFIED., .F., .F. ) 
 B_SPLINE_CURVE_WITH_KNOTS ( ( 3, 2, 2, 2, 3 ),
 ( 0.2645833333333333370, 0.2652777777777777790, 0.2666666666666666630, 0.2680555555555555469, 0.2687499999999999889 ),
 .UNSPECIFIED. ) 
 CURVE ( )  GEOMETRIC_REPRESENTATION_ITEM ( )  RATIONAL_B_SPLINE_CURVE ( ( 0.9330127018922194093, 0.9330127018922194093, 1.000000000000000000, 0.8660254037844387076, 1.000000000000000000, 0.8660254037844387076, 1.000000000000000000, 0.9330127018922194093, 0.9330127018922194093 ) ) 
 REPRESENTATION_ITEM ( '' )  );
#2933=DIRECTION ( 'NONE',  ( -0.000000000000000000, 1.259100132267607459E-16, -1.000000000000000000 ) ) ;
#2934=CARTESIAN_POINT ( 'NONE',  ( -1.394453263437886604E-15, 14.00000000000001066, -45.71098080242149564 ) ) ;
#2935=CARTESIAN_POINT ( 'NONE',  ( 7.367361408496833051E-14, 14.00000000000002132, -110.7109808024214885 ) ) ;
#2937=CARTESIAN_POINT ( 'NONE',  ( -3.310556943750000425, 19.41135094264166483, -68.84743913623280775 ) ) ;
#2939=CARTESIAN_POINT ( 'NONE',  ( 3.310556943750001313, 19.41135094264166838, -119.1807724695661364 ) ) ;
#2942=ORIENTED_EDGE ( 'NONE', *, *, #38583, .F. ) ;
#2944=CARTESIAN_POINT ( 'NONE',  ( 4.648177544792955347E-16, 21.00000000000001066, -32.21098080242150274 ) ) ;
#2945=CARTESIAN_POINT ( 'NONE',  ( 3.310556943750001313, 17.50000000000001776, -78.26410580289946495 ) ) ;
#2946=AXIS2_PLACEMENT_3D ( 'NONE', #15361, #8956, #32134 ) ;
#2947=EDGE_LOOP ( 'NONE', ( #10904, #31624, #25030, #16540 ) ) ;
#2948=VERTEX_POINT ( 'NONE', #2704 ) ;
#2949=CARTESIAN_POINT ( 'NONE',  ( -1.750000000000002220, 14.46891108675447768, -53.48806413671076854 ) ) ;
#2950=CARTESIAN_POINT ( 'NONE',  ( -3.310556943750001313, 17.50000000000002487, -141.7641058028994792 ) ) ;
#2953=CARTESIAN_POINT ( 'NONE',  ( -1.655278471874999990, 20.36702641396248481, -45.01827246956613493 ) ) ;
#2954=CARTESIAN_POINT ( 'NONE',  ( 1.655278471875001101, 20.36702641396249547, -103.1849391362327992 ) ) ;
#2958=CARTESIAN_POINT ( 'NONE',  ( -1.655278471874999990, 20.36702641396248481, -30.93077246956614346 ) ) ;
#2960=CARTESIAN_POINT ( 'NONE',  ( -3.500000000000000888, 19.52072594216371826, -106.0443141357548313 ) ) ;
#2963=CARTESIAN_POINT ( 'NONE',  ( -3.500000000000001332, 17.50000000000001776, -98.65473080337743284 ) ) ;
#2966=CARTESIAN_POINT ( 'NONE',  ( 2.474675557024783212E-16, 21.54145188432739388, -60.21098080242151696 ) ) ;
#2968=CARTESIAN_POINT ( 'NONE',  ( 3.310556943750001313, 17.50000000000001066, -25.26410580289947916 ) ) ;
#2969=CARTESIAN_POINT ( 'NONE',  ( 3.500000000000001332, 17.50000000000001421, -48.15473080337742573 ) ) ;
#2970=CARTESIAN_POINT ( 'NONE',  ( -1.394453263437886604E-15, 14.00000000000001066, -45.71098080242149564 ) ) ;
#2972=CARTESIAN_POINT ( 'NONE',  ( 1.655278471874998436, 14.63297358603753828, -33.51827246956613493 ) ) ;
#2975=CARTESIAN_POINT ( 'NONE',  ( -1.394453263437886604E-15, 14.00000000000001066, -50.40473080337741862 ) ) ;
#2979=CARTESIAN_POINT ( 'NONE',  ( -1.655278471875002211, 14.63297358603754716, -82.59743913623279354 ) ) ;
#2980=CARTESIAN_POINT ( 'NONE',  ( -3.500000000000001332, 17.50000000000001066, -25.65473080337743284 ) ) ;
#2986=CARTESIAN_POINT ( 'NONE',  ( -1.655278471874999990, 20.36702641396249192, -93.93077246956613635 ) ) ;
#2988=ADVANCED_FACE ( 'NONE', ( #38012 ), #12272, .T. ) ;
#2989=ORIENTED_EDGE ( 'NONE', *, *, #4527, .T. ) ;
#2992=EDGE_CURVE ( 'NONE', #39978, #13141, #23427, .T. ) ;
#2994=APPLICATION_CONTEXT ( 'automotive_design' ) ;
#2995=CARTESIAN_POINT ( 'NONE',  ( 4.648177544792955347E-16, 21.00000000000001421, -66.21098080242148853 ) ) ;
#2997=( BOUNDED_CURVE ( )  B_SPLINE_CURVE ( 2, ( #2720, #35472, #34837, #41652, #12507, #18682, #5915, #25492, #6332 ),
 .UNSPECIFIED., .F., .F. ) 
 B_SPLINE_CURVE_WITH_KNOTS ( ( 3, 2, 2, 2, 3 ),
 ( 0.9687500000000000000, 0.9694444444444444420, 0.9708333333333333259, 0.9722222222222222099, 0.9729166666666666519 ),
 .UNSPECIFIED. ) 
 CURVE ( )  GEOMETRIC_REPRESENTATION_ITEM ( )  RATIONAL_B_SPLINE_CURVE ( ( 0.9330127018922194093, 0.9330127018922194093, 1.000000000000000000, 0.8660254037844387076, 1.000000000000000000, 0.8660254037844387076, 1.000000000000000000, 0.9330127018922194093, 0.9330127018922194093 ) ) 
 REPRESENTATION_ITEM ( '' )  );
#2999=CARTESIAN_POINT ( 'NONE',  ( -1.394453263437886604E-15, 14.00000000000002132, -127.4047308033774186 ) ) ;
#3000=DIRECTION ( 'NONE',  ( 0.000000000000000000, 1.000000000000000000, 0.000000000000000000 ) ) ;
#3001=CARTESIAN_POINT ( 'NONE',  ( 1.655278471875001101, 20.36702641396249902, -132.0974391362328220 ) ) ;
#3003=CARTESIAN_POINT ( 'NONE',  ( 3.500000000000001332, 17.50000000000002487, -141.4609808024215170 ) ) ;
#3005=CARTESIAN_POINT ( 'NONE',  ( 3.500000000000001332, 17.50000000000002487, -139.1547308033774186 ) ) ;
#3006=CARTESIAN_POINT ( 'NONE',  ( -1.655278471875002211, 14.63297358603755072, -117.6849391362327850 ) ) ;
#3007=CARTESIAN_POINT ( 'NONE',  ( 1.655278471875001101, 20.36702641396248836, -53.18493913623280633 ) ) ;
#3009=CARTESIAN_POINT ( 'NONE',  ( -1.750000000000002220, 14.46891108675448834, -132.4880641367107614 ) ) ;
#3012=CARTESIAN_POINT ( 'NONE',  ( 3.310556943749999981, 15.58864905735836714, -75.43493913623281344 ) ) ;
#3013=CARTESIAN_POINT ( 'NONE',  ( -3.500000000000001332, 17.50000000000002132, -121.9609808024215170 ) ) ;
#3014=CARTESIAN_POINT ( 'NONE',  ( -3.310556943750002645, 15.58864905735837780, -109.6807724695661364 ) ) ;
#3015=DIRECTION ( 'NONE',  ( -0.000000000000000000, 1.259100132267607459E-16, -1.000000000000000000 ) ) ;
#3018=CARTESIAN_POINT ( 'NONE',  ( -1.749999999999999778, 20.53108891324555429, -75.12764746908817415 ) ) ;
#3020=CARTESIAN_POINT ( 'NONE',  ( 2.340729813953370519E-16, 21.32270188528330479, -44.01410580289947916 ) ) ;
#3021=CARTESIAN_POINT ( 'NONE',  ( 3.310556943749999981, 15.58864905735837070, -103.4349391362327992 ) ) ;
#3022=CARTESIAN_POINT ( 'NONE',  ( 1.749999999999998224, 14.46891108675447768, -63.32139747004410424 ) ) ;
#3024=VERTEX_POINT ( 'NONE', #22472 ) ;
#3025=CARTESIAN_POINT ( 'NONE',  ( 3.310556943750001313, 19.41135094264166838, -119.2682724695661278 ) ) ;
#3026=CARTESIAN_POINT ( 'NONE',  ( -0.9378221735089310451, 14.00000000000001066, -27.75563900116003069 ) ) ;
#3029=CARTESIAN_POINT ( 'NONE',  ( -1.394453263437886604E-15, 14.00000000000001066, -50.71098080242150274 ) ) ;
#3031=CARTESIAN_POINT ( 'NONE',  ( 3.310556943750001313, 17.50000000000001776, -100.2641058028994792 ) ) ;
#3032=DIRECTION ( 'NONE',  ( 0.000000000000000000, 1.000000000000000000, 0.000000000000000000 ) ) ;
#3035=CARTESIAN_POINT ( 'NONE',  ( -0.9378221735089310451, 14.00000000000001066, -28.75563900116003069 ) ) ;
#3036=CARTESIAN_POINT ( 'NONE',  ( 4.648177544792955347E-16, 21.00000000000002132, -118.9047308033774328 ) ) ;
#3038=CARTESIAN_POINT ( 'NONE',  ( -1.394453263437886604E-15, 14.00000000000001066, -40.40473080337743284 ) ) ;
#3042=CARTESIAN_POINT ( 'NONE',  ( -3.310556943750001313, 17.50000000000001066, -33.76410580289947205 ) ) ;
#3044=DIRECTION ( 'NONE',  ( 0.000000000000000000, 1.000000000000000000, 0.000000000000000000 ) ) ;
#3045=EDGE_CURVE ( 'NONE', #15247, #28708, #13110, .T. ) ;
#3047=ORIENTED_EDGE ( 'NONE', *, *, #30708, .F. ) ;
#3050=VERTEX_POINT ( 'NONE', #10347 ) ;
#3052=( BOUNDED_CURVE ( )  B_SPLINE_CURVE ( 2, ( #19851, #287, #32818, #3688, #10285, #36221, #7095, #20072, #15849 ),
 .UNSPECIFIED., .F., .T. ) 
 B_SPLINE_CURVE_WITH_KNOTS ( ( 3, 2, 2, 2, 3 ),
 ( 0.8520833333333333037, 0.8527777777777777457, 0.8541666666666666297, 0.8555555555555555136, 0.8562499999999999556 ),
 .UNSPECIFIED. ) 
 CURVE ( )  GEOMETRIC_REPRESENTATION_ITEM ( )  RATIONAL_B_SPLINE_CURVE ( ( 0.9330127018922194093, 0.9330127018922194093, 1.000000000000000000, 0.8660254037844387076, 1.000000000000000000, 0.8660254037844387076, 1.000000000000000000, 0.9330127018922194093, 0.9330127018922194093 ) ) 
 REPRESENTATION_ITEM ( '' )  );
#3053=CARTESIAN_POINT ( 'NONE',  ( 4.286263797015737581E-16, 14.00000000000002487, -149.5231586289125687 ) ) ;
#3055=DIRECTION ( 'NONE',  ( 0.000000000000000000, 1.000000000000000000, 0.000000000000000000 ) ) ;
#3056=CARTESIAN_POINT ( 'NONE',  ( 3.500000000000000000, 15.47927405783632970, -117.2380641367107614 ) ) ;
#3058=CARTESIAN_POINT ( 'NONE',  ( -1.749999999999999778, 20.53108891324554719, -33.12764746908818125 ) ) ;
#3059=CARTESIAN_POINT ( 'NONE',  ( 4.648177544792955347E-16, 21.00000000000001421, -50.21098080242150985 ) ) ;
#3060=CARTESIAN_POINT ( 'NONE',  ( -0.9378221735089291577, 21.00000000000001066, -44.86007260463891555 ) ) ;
#3062=CARTESIAN_POINT ( 'NONE',  ( -1.394453263437886604E-15, 14.00000000000001066, -41.71098080242150274 ) ) ;
#3064=CARTESIAN_POINT ( 'NONE',  ( 1.750000000000001110, 20.53108891324556140, -139.2943141357548313 ) ) ;
#3065=CARTESIAN_POINT ( 'NONE',  ( -3.500000000000001332, 17.50000000000001421, -52.96098080242150985 ) ) ;
#3066=CARTESIAN_POINT ( 'NONE',  ( 3.310556943749999981, 15.58864905735837247, -121.3474391362328078 ) ) ;
#3069=CARTESIAN_POINT ( 'NONE',  ( -3.500000000000000000, 19.52072594216371115, -82.04431413575483134 ) ) ;
#3070=CARTESIAN_POINT ( 'NONE',  ( -7.424026671074350129E-16, 13.45854811567263631, -90.71098080242151696 ) ) ;
#3072=CARTESIAN_POINT ( 'NONE',  ( -1.750000000000002220, 14.46891108675447768, -45.48806413671076143 ) ) ;
#3073=CARTESIAN_POINT ( 'NONE',  ( -1.655278471874999990, 20.36702641396248836, -60.93077246956614346 ) ) ;
#3074=CARTESIAN_POINT ( 'NONE',  ( -1.655278471875002211, 14.63297358603755072, -118.6849391362327992 ) ) ;
#3076=CARTESIAN_POINT ( 'NONE',  ( -7.424026671074350129E-16, 13.45854811567263098, -34.40473080337742573 ) ) ;
#3077=CARTESIAN_POINT ( 'NONE',  ( -1.394453263437886604E-15, 14.00000000000001776, -92.40473080337741862 ) ) ;
#3079=ADVANCED_FACE ( 'NONE', ( #35864 ), #32881, .T. ) ;
#3080=CARTESIAN_POINT ( 'NONE',  ( -1.655278471874999990, 20.36702641396249902, -133.0182724695661420 ) ) ;
#3082=CARTESIAN_POINT ( 'NONE',  ( -0.9378221735089310451, 14.00000000000001599, -66.44938900211595012 ) ) ;
#3083=CARTESIAN_POINT ( 'NONE',  ( -1.655278471874999990, 20.36702641396248481, -44.01827246956613493 ) ) ;
#3085=CARTESIAN_POINT ( 'NONE',  ( -1.655278471874999990, 20.36702641396248836, -67.01827246956612782 ) ) ;
#3087=CARTESIAN_POINT ( 'NONE',  ( -3.310556943750001313, 17.50000000000001421, -64.76410580289946495 ) ) ;
#3088=ORIENTED_EDGE ( 'NONE', *, *, #34190, .F. ) ;
#3089=CARTESIAN_POINT ( 'NONE',  ( 3.310556943750001313, 19.41135094264166838, -86.26827246956612782 ) ) ;
#3092=DIRECTION ( 'NONE',  ( 0.000000000000000000, 1.000000000000000000, 0.000000000000000000 ) ) ;
#3096=CARTESIAN_POINT ( 'NONE',  ( 3.310556943750001313, 19.41135094264166483, -50.18077246956615056 ) ) ;
#3098=CARTESIAN_POINT ( 'NONE',  ( 3.310556943750001313, 19.41135094264166838, -104.1807724695661221 ) ) ;
#3099=CARTESIAN_POINT ( 'NONE',  ( 1.749999999999998224, 14.46891108675448301, -96.32139747004409003 ) ) ;
#3102=VECTOR ( 'NONE', #24226, 1000.000000000000000 ) ;
#3106=CARTESIAN_POINT ( 'NONE',  ( 1.655278471875001101, 20.36702641396248836, -56.09743913623280065 ) ) ;
#3108=ORIENTED_EDGE ( 'NONE', *, *, #3274, .F. ) ;
#3109=CARTESIAN_POINT ( 'NONE',  ( 3.500000000000000000, 15.47927405783632615, -76.54431413575485976 ) ) ;
#3110=CARTESIAN_POINT ( 'NONE',  ( 0.000000000000000000, 17.50000000000002487, -149.5231586289125687 ) ) ;
#3115=CARTESIAN_POINT ( 'NONE',  ( 1.655278471875001101, 20.36702641396249547, -125.0974391362328078 ) ) ;
#3117=CARTESIAN_POINT ( 'NONE',  ( -3.310556943750001313, 17.50000000000001066, -33.85160580289946353 ) ) ;
#3119=CARTESIAN_POINT ( 'NONE',  ( -3.310556943750002645, 15.58864905735836182, -25.76827246956613138 ) ) ;
#3120=CARTESIAN_POINT ( 'NONE',  ( 3.310556943749999981, 15.58864905735836892, -90.43493913623278502 ) ) ;
#3121=CARTESIAN_POINT ( 'NONE',  ( 3.310556943750001313, 19.41135094264167549, -141.1807724695661648 ) ) ;
#3123=CARTESIAN_POINT ( 'NONE',  ( 0.000000000000000000, 17.50000000000002487, -149.5231586289125687 ) ) ;
#3126=CARTESIAN_POINT ( 'NONE',  ( -1.655278471875002211, 14.63297358603755249, -135.6849391362327992 ) ) ;
#3127=AXIS2_PLACEMENT_3D ( 'NONE', #25399, #19833, #22197 ) ;
#3130=CARTESIAN_POINT ( 'NONE',  ( -0.9378221735089291577, 21.00000000000002132, -126.1663226036829855 ) ) ;
#3131=CARTESIAN_POINT ( 'NONE',  ( -1.975475456537005874E-15, 21.00000000000002487, -142.2109808024214885 ) ) ;
#3132=CARTESIAN_POINT ( 'NONE',  ( 3.500000000000001332, 17.50000000000001776, -79.15473080337743284 ) ) ;
#3133=CARTESIAN_POINT ( 'NONE',  ( 3.310556943750001313, 19.41135094264166483, -57.26827246956612782 ) ) ;
#3136=CARTESIAN_POINT ( 'NONE',  ( -0.9378221735089291577, 21.00000000000002487, -129.8600726046389013 ) ) ;
#3137=CARTESIAN_POINT ( 'NONE',  ( 3.310556943749999981, 15.58864905735836892, -85.43493913623278502 ) ) ;
#3139=CARTESIAN_POINT ( 'NONE',  ( -3.500000000000001332, 17.50000000000001776, -77.65473080337741862 ) ) ;
#3140=CARTESIAN_POINT ( 'NONE',  ( -1.655278471874999990, 20.36702641396249547, -114.9307724695661364 ) ) ;
#3141=CARTESIAN_POINT ( 'NONE',  ( -3.310556943750001313, 17.50000000000001776, -78.76410580289946495 ) ) ;
#3144=CARTESIAN_POINT ( 'NONE',  ( -3.500000000000000888, 19.52072594216371826, -106.7380641367107614 ) ) ;
#3148=CARTESIAN_POINT ( 'NONE',  ( 1.749999999999998224, 14.46891108675447590, -45.62764746908818125 ) ) ;
#3149=EDGE_CURVE ( 'NONE', #14304, #27997, #6029, .T. ) ;
#3150=CARTESIAN_POINT ( 'NONE',  ( -1.394453263437886604E-15, 14.00000000000001066, -32.40473080337742573 ) ) ;
#3152=CARTESIAN_POINT ( 'NONE',  ( 3.310556943749999981, 15.58864905735836537, -64.34743913623280775 ) ) ;
#3154=CARTESIAN_POINT ( 'NONE',  ( 3.310556943749999981, 15.58864905735837425, -123.3474391362327935 ) ) ;
#3155=CARTESIAN_POINT ( 'NONE',  ( 4.648177544792955347E-16, 21.00000000000001421, -70.90473080337743284 ) ) ;
#3158=CARTESIAN_POINT ( 'NONE',  ( 0.9378221735089281585, 14.00000000000001599, -79.36007260463891555 ) ) ;
#3159=CARTESIAN_POINT ( 'NONE',  ( -3.310556943750000425, 19.41135094264166483, -74.84743913623280775 ) ) ;
#3160=ORIENTED_EDGE ( 'NONE', *, *, #474, .T. ) ;
#3164=CARTESIAN_POINT ( 'NONE',  ( 1.655278471875001101, 20.36702641396249902, -141.0974391362327935 ) ) ;
#3165=CARTESIAN_POINT ( 'NONE',  ( -1.836030130193217234E-14, 21.00000000000002132, -129.2109808024214601 ) ) ;
#3167=CARTESIAN_POINT ( 'NONE',  ( 3.310556943749999981, 15.58864905735836182, -44.43493913623279923 ) ) ;
#3168=CARTESIAN_POINT ( 'NONE',  ( 1.655278471874998436, 14.63297358603754716, -104.5182724695661278 ) ) ;
#3170=( BOUNDED_CURVE ( )  B_SPLINE_CURVE ( 2, ( #5145, #21309, #2577, #1749, #38100, #31294, #1946, #31709, #24721 ),
 .UNSPECIFIED., .F., .F. ) 
 B_SPLINE_CURVE_WITH_KNOTS ( ( 3, 2, 2, 2, 3 ),
 ( 0.2812500000000000000, 0.2819444444444444420, 0.2833333333333333259, 0.2847222222222222099, 0.2854166666666666519 ),
 .UNSPECIFIED. ) 
 CURVE ( )  GEOMETRIC_REPRESENTATION_ITEM ( )  RATIONAL_B_SPLINE_CURVE ( ( 0.9330127018922194093, 0.9330127018922194093, 1.000000000000000000, 0.8660254037844387076, 1.000000000000000000, 0.8660254037844387076, 1.000000000000000000, 0.9330127018922194093, 0.9330127018922194093 ) ) 
 REPRESENTATION_ITEM ( '' )  );
#3172=CARTESIAN_POINT ( 'NONE',  ( 2.340729813953370519E-16, 21.32270188528330479, -29.01410580289947916 ) ) ;
#3173=CARTESIAN_POINT ( 'NONE',  ( -3.500000000000002220, 15.47927405783633503, -111.8776474690881884 ) ) ;
#3174=CARTESIAN_POINT ( 'NONE',  ( 3.500000000000000000, 15.47927405783632793, -107.5443141357548456 ) ) ;
#3177=CARTESIAN_POINT ( 'NONE',  ( 1.749999999999998224, 14.46891108675448123, -94.32139747004409003 ) ) ;
#3178=FACE_OUTER_BOUND ( 'NONE', #22499, .T. ) ;
#3181=ADVANCED_FACE ( 'NONE', ( #23103 ), #13748, .T. ) ;
#3182=CARTESIAN_POINT ( 'NONE',  ( -3.500000000000001332, 17.50000000000001421, -60.96098080242150274 ) ) ;
#3183=CARTESIAN_POINT ( 'NONE',  ( -1.749999999999999778, 20.53108891324555074, -47.12764746908818125 ) ) ;
#3184=CARTESIAN_POINT ( 'NONE',  ( 3.310556943750001313, 19.41135094264165772, -28.18077246956614346 ) ) ;
#3185=CARTESIAN_POINT ( 'NONE',  ( 3.500000000000001776, 19.52072594216370760, -49.07139747004409713 ) ) ;
#3186=CARTESIAN_POINT ( 'NONE',  ( -3.695301148110399846E-14, 21.00000000000002132, -125.2109808024214885 ) ) ;
#3187=CARTESIAN_POINT ( 'NONE',  ( -7.022189441860112050E-16, 13.67729811471671653, -30.60160580289945997 ) ) ;
#3190=CARTESIAN_POINT ( 'NONE',  ( -3.500000000000001332, 17.50000000000002132, -120.9609808024215170 ) ) ;
#3194=CARTESIAN_POINT ( 'NONE',  ( 2.340729813953370519E-16, 21.32270188528331190, -82.01410580289947916 ) ) ;
#3196=ORIENTED_EDGE ( 'NONE', *, *, #28978, .T. ) ;
#3198=CARTESIAN_POINT ( 'NONE',  ( -1.394453263437886604E-15, 14.00000000000001421, -64.71098080242150274 ) ) ;
#3199=VERTEX_POINT ( 'NONE', #29477 ) ;
#3202=CARTESIAN_POINT ( 'NONE',  ( -1.655278471875002211, 14.63297358603754716, -87.59743913623280775 ) ) ;
#3203=ORIENTED_EDGE ( 'NONE', *, *, #31226, .F. ) ;
#3209=VERTEX_POINT ( 'NONE', #6531 ) ;
#3210=FACE_OUTER_BOUND ( 'NONE', #40613, .T. ) ;
#3211=DIRECTION ( 'NONE',  ( 0.000000000000000000, 1.000000000000000000, 0.000000000000000000 ) ) ;
#3212=CARTESIAN_POINT ( 'NONE',  ( 3.310556943750001313, 17.50000000000002132, -129.2641058028994507 ) ) ;
#3213=VERTEX_POINT ( 'NONE', #13326 ) ;
#3214=CARTESIAN_POINT ( 'NONE',  ( 1.655278471875001101, 20.36702641396249547, -119.1849391362327992 ) ) ;
#3215=CARTESIAN_POINT ( 'NONE',  ( 1.655278471875001101, 20.36702641396248836, -49.18493913623279923 ) ) ;
#3217=CARTESIAN_POINT ( 'NONE',  ( -3.500000000000001332, 17.50000000000002487, -129.6547308033774186 ) ) ;
#3218=CARTESIAN_POINT ( 'NONE',  ( -1.655278471874999990, 20.36702641396248836, -73.01827246956612782 ) ) ;
#3219=CARTESIAN_POINT ( 'NONE',  ( -3.500000000000001332, 17.50000000000002132, -124.9609808024215027 ) ) ;
#3220=CARTESIAN_POINT ( 'NONE',  ( 1.655278471875001101, 20.36702641396249547, -105.0974391362328078 ) ) ;
#3222=CARTESIAN_POINT ( 'NONE',  ( -3.500000000000001332, 17.50000000000002132, -107.6547308033774186 ) ) ;
#3225=CARTESIAN_POINT ( 'NONE',  ( 3.500000000000001776, 19.52072594216371115, -76.37764746908817415 ) ) ;
#3227=CARTESIAN_POINT ( 'NONE',  ( -1.655278471874999990, 20.36702641396248481, -42.93077246956614346 ) ) ;
#3228=CARTESIAN_POINT ( 'NONE',  ( -7.022189441860112050E-16, 13.67729811471672363, -94.60160580289945642 ) ) ;
#3229=CARTESIAN_POINT ( 'NONE',  ( 1.749999999999998224, 14.46891108675447946, -68.32139747004409003 ) ) ;
#3230=CARTESIAN_POINT ( 'NONE',  ( -3.500000000000001332, 17.50000000000001421, -63.65473080337742573 ) ) ;
#3231=LINE ( 'NONE', #12169, #23238 ) ;
#3232=VERTEX_POINT ( 'NONE', #3131 ) ;
#3233=CARTESIAN_POINT ( 'NONE',  ( 1.655278471874998436, 14.63297358603754894, -120.5182724695661278 ) ) ;
#3234=CARTESIAN_POINT ( 'NONE',  ( -3.500000000000000000, 19.52072594216371826, -136.7380641367107614 ) ) ;
#3238=CARTESIAN_POINT ( 'NONE',  ( 1.655278471875001101, 20.36702641396249192, -100.0974391362328078 ) ) ;
#3242=CARTESIAN_POINT ( 'NONE',  ( 0.000000000000000000, 21.00000000000002487, -149.5231586289125687 ) ) ;
#3248=CARTESIAN_POINT ( 'NONE',  ( 3.310556943749999981, 15.58864905735836182, -33.34743913623280775 ) ) ;
#3249=( BOUNDED_CURVE ( )  B_SPLINE_CURVE ( 2, ( #19285, #32258, #16115, #19909, #19695, #6721, #35449, #550, #26508 ),
 .UNSPECIFIED., .F., .T. ) 
 B_SPLINE_CURVE_WITH_KNOTS ( ( 3, 2, 2, 2, 3 ),
 ( 0.9020833333333333481, 0.9027777777777777901, 0.9041666666666666741, 0.9055555555555555580, 0.9062500000000000000 ),
 .UNSPECIFIED. ) 
 CURVE ( )  GEOMETRIC_REPRESENTATION_ITEM ( )  RATIONAL_B_SPLINE_CURVE ( ( 0.9330127018922194093, 0.9330127018922194093, 1.000000000000000000, 0.8660254037844387076, 1.000000000000000000, 0.8660254037844387076, 1.000000000000000000, 0.9330127018922194093, 0.9330127018922194093 ) ) 
 REPRESENTATION_ITEM ( '' )  );
#3252=EDGE_CURVE ( 'NONE', #13926, #32798, #30761, .T. ) ;
#3253=VECTOR ( 'NONE', #29761, 1000.000000000000000 ) ;
#3258=CARTESIAN_POINT ( 'NONE',  ( -1.750000000000002220, 14.46891108675447590, -37.48806413671076854 ) ) ;
#3260=CARTESIAN_POINT ( 'NONE',  ( 3.310556943750001313, 17.50000000000001066, -23.35160580289946708 ) ) ;
#3261=CARTESIAN_POINT ( 'NONE',  ( 1.750000000000001110, 20.53108891324555785, -117.9880641367107614 ) ) ;
#3263=CARTESIAN_POINT ( 'NONE',  ( -3.310556943750001313, 17.50000000000002487, -133.8516058028994564 ) ) ;
#3264=CARTESIAN_POINT ( 'NONE',  ( 3.500000000000001332, 17.50000000000001066, -34.46098080242150985 ) ) ;
#3267=CARTESIAN_POINT ( 'NONE',  ( -1.749999999999999778, 20.53108891324555074, -65.82139747004409003 ) ) ;
#3269=CARTESIAN_POINT ( 'NONE',  ( 3.500000000000001332, 17.50000000000002487, -137.4609808024214885 ) ) ;
#3270=CARTESIAN_POINT ( 'NONE',  ( -1.655278471875002211, 14.63297358603755072, -121.5974391362328078 ) ) ;
#3273=EDGE_CURVE ( 'NONE', #18937, #2506, #13364, .T. ) ;
#3274=EDGE_CURVE ( 'NONE', #37632, #34378, #29368, .T. ) ;
#3275=DIRECTION ( 'NONE',  ( 0.000000000000000000, 1.000000000000000000, 0.000000000000000000 ) ) ;
#3276=CARTESIAN_POINT ( 'NONE',  ( 3.500000000000001776, 19.52072594216371115, -92.37764746908815994 ) ) ;
#3277=CARTESIAN_POINT ( 'NONE',  ( 1.655278471875001101, 20.36702641396248836, -61.09743913623280775 ) ) ;
#3278=EDGE_CURVE ( 'NONE', #15800, #4141, #33752, .T. ) ;
#3279=CARTESIAN_POINT ( 'NONE',  ( 3.310556943750001313, 17.50000000000002132, -116.3516058028994706 ) ) ;
#3281=CARTESIAN_POINT ( 'NONE',  ( 3.500000000000001332, 17.50000000000001066, -34.15473080337742573 ) ) ;
#3282=CARTESIAN_POINT ( 'NONE',  ( 4.648177544792955347E-16, 21.00000000000001776, -91.90473080337741862 ) ) ;
#3284=CARTESIAN_POINT ( 'NONE',  ( 3.310556943750001313, 19.41135094264167549, -136.2682724695661420 ) ) ;
#3288=CARTESIAN_POINT ( 'NONE',  ( 3.310556943750001313, 17.50000000000001421, -68.35160580289947063 ) ) ;
#3290=CARTESIAN_POINT ( 'NONE',  ( -1.655278471875002211, 14.63297358603754361, -63.59743913623280775 ) ) ;
#3292=CARTESIAN_POINT ( 'NONE',  ( -1.655278471875002211, 14.63297358603754716, -86.68493913623278502 ) ) ;
#3295=CYLINDRICAL_SURFACE ( 'NONE', #15773, 3.499999999999999556 ) ;
#3296=CARTESIAN_POINT ( 'NONE',  ( 1.655278471875001101, 20.36702641396248836, -52.09743913623281486 ) ) ;
#3298=CARTESIAN_POINT ( 'NONE',  ( 3.310556943750001313, 19.41135094264166838, -103.1807724695661506 ) ) ;
#3299=CARTESIAN_POINT ( 'NONE',  ( -1.394453263437886604E-15, 14.00000000000001776, -96.40473080337741862 ) ) ;
#3300=( BOUNDED_CURVE ( )  B_SPLINE_CURVE ( 2, ( #12177, #29167, #28344, #19404, #32168, #38340, #22178, #22594, #41963 ),
 .UNSPECIFIED., .F., .T. ) 
 B_SPLINE_CURVE_WITH_KNOTS ( ( 3, 2, 2, 2, 3 ),
 ( 0.7520833333333333259, 0.7527777777777777679, 0.7541666666666666519, 0.7555555555555555358, 0.7562499999999999778 ),
 .UNSPECIFIED. ) 
 CURVE ( )  GEOMETRIC_REPRESENTATION_ITEM ( )  RATIONAL_B_SPLINE_CURVE ( ( 0.9330127018922194093, 0.9330127018922194093, 1.000000000000000000, 0.8660254037844387076, 1.000000000000000000, 0.8660254037844387076, 1.000000000000000000, 0.9330127018922194093, 0.9330127018922194093 ) ) 
 REPRESENTATION_ITEM ( '' )  );
#3301=ORIENTED_EDGE ( 'NONE', *, *, #20192, .F. ) ;
#3303=ORIENTED_EDGE ( 'NONE', *, *, #26427, .F. ) ;
#3305=CARTESIAN_POINT ( 'NONE',  ( -7.022189441860112050E-16, 13.67729811471671830, -58.51410580289947916 ) ) ;
#3307=ORIENTED_EDGE ( 'NONE', *, *, #8709, .T. ) ;
#3309=AXIS2_PLACEMENT_3D ( 'NONE', #26067, #25443, #34792 ) ;
#3310=PLANE ( 'NONE',  #36167 ) ;
#3312=CARTESIAN_POINT ( 'NONE',  ( 0.9378221735089300459, 21.00000000000001421, -55.25563900116002714 ) ) ;
#3314=CARTESIAN_POINT ( 'NONE',  ( -1.749999999999999778, 20.53108891324556140, -140.8213974700441042 ) ) ;
#3316=ORIENTED_EDGE ( 'NONE', *, *, #14999, .F. ) ;
#3317=DIRECTION ( 'NONE',  ( -0.000000000000000000, 1.259100132267607459E-16, -1.000000000000000000 ) ) ;
#3318=CARTESIAN_POINT ( 'NONE',  ( -3.310556943750002201, 15.58864905735837780, -125.6807724695661364 ) ) ;
#3320=CARTESIAN_POINT ( 'NONE',  ( -1.655278471875002211, 14.63297358603754006, -35.68493913623279923 ) ) ;
#3321=CARTESIAN_POINT ( 'NONE',  ( 3.310556943749999981, 15.58864905735836182, -26.43493913623279212 ) ) ;
#3322=ADVANCED_FACE ( 'NONE', ( #14379 ), #20336, .T. ) ;
#3323=CARTESIAN_POINT ( 'NONE',  ( -1.655278471875002211, 14.63297358603754716, -85.68493913623278502 ) ) ;
#3324=CARTESIAN_POINT ( 'NONE',  ( 1.655278471874998436, 14.63297358603755249, -139.4307724695661364 ) ) ;
#3327=CARTESIAN_POINT ( 'NONE',  ( -3.500000000000000000, 19.52072594216370760, -67.04431413575484555 ) ) ;
#3328=EDGE_CURVE ( 'NONE', #18011, #23461, #17573, .T. ) ;
#3329=CARTESIAN_POINT ( 'NONE',  ( -3.310556943750001313, 17.50000000000002487, -135.8516058028994564 ) ) ;
#3331=CARTESIAN_POINT ( 'NONE',  ( -1.655278471875002211, 14.63297358603754716, -91.59743913623280775 ) ) ;
#3332=CARTESIAN_POINT ( 'NONE',  ( 3.500000000000000000, 15.47927405783632082, -28.23806413671076143 ) ) ;
#3334=CARTESIAN_POINT ( 'NONE',  ( 1.749999999999998224, 14.46891108675447946, -73.32139747004410424 ) ) ;
#3335=CARTESIAN_POINT ( 'NONE',  ( 1.655278471874998436, 14.63297358603754184, -59.51827246956613493 ) ) ;
#3337=CARTESIAN_POINT ( 'NONE',  ( 0.000000000000000000, 21.00000000000002487, -149.5231586289125687 ) ) ;
#3339=CARTESIAN_POINT ( 'NONE',  ( 1.655278471874998436, 14.63297358603754539, -86.51827246956612782 ) ) ;
#3340=CARTESIAN_POINT ( 'NONE',  ( -3.310556943750001313, 17.50000000000002487, -142.8516058028994564 ) ) ;
#3342=CARTESIAN_POINT ( 'NONE',  ( 3.310556943750001313, 17.50000000000002132, -114.2641058028994792 ) ) ;
#3343=CARTESIAN_POINT ( 'NONE',  ( 3.310556943749999981, 15.58864905735836892, -81.34743913623280775 ) ) ;
#3344=CARTESIAN_POINT ( 'NONE',  ( -1.750000000000002220, 14.46891108675448478, -96.48806413671076143 ) ) ;
#3345=VERTEX_POINT ( 'NONE', #20768 ) ;
#3346=CARTESIAN_POINT ( 'NONE',  ( -7.022189441860112050E-16, 13.67729811471672541, -102.6016058028994706 ) ) ;
#3347=CARTESIAN_POINT ( 'NONE',  ( 1.749999999999998224, 14.46891108675448301, -103.3213974700440900 ) ) ;
#3349=CARTESIAN_POINT ( 'NONE',  ( 3.369928719974892676E-15, 14.00000000000002309, -139.4047308033773902 ) ) ;
#3350=CARTESIAN_POINT ( 'NONE',  ( 0.9378221735089281585, 14.00000000000001066, -44.36007260463891555 ) ) ;
#3351=DIRECTION ( 'NONE',  ( -0.000000000000000000, 1.259100132267607459E-16, -1.000000000000000000 ) ) ;
#3354=CARTESIAN_POINT ( 'NONE',  ( 3.310556943749999981, 15.58864905735836714, -68.34743913623280775 ) ) ;
#3356=CARTESIAN_POINT ( 'NONE',  ( 1.655278471875001101, 20.36702641396249547, -121.0974391362328078 ) ) ;
#3358=VECTOR ( 'NONE', #20864, 1000.000000000000000 ) ;
#3364=CARTESIAN_POINT ( 'NONE',  ( -3.310556943750002645, 15.58864905735837070, -72.68077246956613635 ) ) ;
#3368=EDGE_CURVE ( 'NONE', #13507, #18006, #17715, .T. ) ;
#3369=( BOUNDED_CURVE ( )  B_SPLINE_CURVE ( 2, ( #17362, #7359, #11187, #30323, #36926, #7789, #17774, #30745, #13523 ),
 .UNSPECIFIED., .F., .T. ) 
 B_SPLINE_CURVE_WITH_KNOTS ( ( 3, 2, 2, 2, 3 ),
 ( 0.8395833333333333481, 0.8402777777777777901, 0.8416666666666666741, 0.8430555555555555580, 0.8437500000000000000 ),
 .UNSPECIFIED. ) 
 CURVE ( )  GEOMETRIC_REPRESENTATION_ITEM ( )  RATIONAL_B_SPLINE_CURVE ( ( 0.9330127018922194093, 0.9330127018922194093, 1.000000000000000000, 0.8660254037844387076, 1.000000000000000000, 0.8660254037844387076, 1.000000000000000000, 0.9330127018922194093, 0.9330127018922194093 ) ) 
 REPRESENTATION_ITEM ( '' )  );
#3370=CARTESIAN_POINT ( 'NONE',  ( -7.022189441860112050E-16, 13.67729811471673074, -139.5141058028994792 ) ) ;
#3372=CARTESIAN_POINT ( 'NONE',  ( 4.648177544792955347E-16, 21.00000000000001421, -51.90473080337743284 ) ) ;
#3374=CARTESIAN_POINT ( 'NONE',  ( -3.310556943750002645, 15.58864905735836714, -44.76827246956613493 ) ) ;
#3375=ADVANCED_FACE ( 'NONE', ( #19179 ), #2389, .T. ) ;
#3376=CARTESIAN_POINT ( 'NONE',  ( -3.310556943750000425, 19.41135094264166483, -101.9349391362327992 ) ) ;
#3378=CARTESIAN_POINT ( 'NONE',  ( -1.655278471874999990, 20.36702641396248481, -27.93077246956614346 ) ) ;
#3380=CARTESIAN_POINT ( 'NONE',  ( 3.500000000000001776, 19.52072594216371115, -101.3776474690881741 ) ) ;
#3382=CARTESIAN_POINT ( 'NONE',  ( -3.500000000000001332, 17.50000000000001776, -92.65473080337743284 ) ) ;
#3383=CARTESIAN_POINT ( 'NONE',  ( -3.500000000000002220, 15.47927405783632793, -77.87764746908817415 ) ) ;
#3386=CARTESIAN_POINT ( 'NONE',  ( -1.750000000000002220, 14.46891108675447946, -61.79431413575483845 ) ) ;
#3388=LINE ( 'NONE', #834, #12208 ) ;
#3389=CARTESIAN_POINT ( 'NONE',  ( -1.749999999999999778, 20.53108891324555074, -48.82139747004410424 ) ) ;
#3390=CARTESIAN_POINT ( 'NONE',  ( 4.648177544792955347E-16, 21.00000000000002487, -132.2109808024214885 ) ) ;
#3391=CARTESIAN_POINT ( 'NONE',  ( -1.655278471875002211, 14.63297358603754006, -26.68493913623279212 ) ) ;
#3397=CARTESIAN_POINT ( 'NONE',  ( -3.310556943750001313, 17.50000000000001776, -84.76410580289947916 ) ) ;
#3398=CARTESIAN_POINT ( 'NONE',  ( 1.749999999999998224, 14.46891108675447590, -52.62764746908817415 ) ) ;
#3400=CARTESIAN_POINT ( 'NONE',  ( -1.749999999999999778, 20.53108891324555785, -124.1276474690881599 ) ) ;
#3401=CARTESIAN_POINT ( 'NONE',  ( 4.648177544792955347E-16, 21.00000000000001776, -80.21098080242148853 ) ) ;
#3403=CARTESIAN_POINT ( 'NONE',  ( 4.648177544792955347E-16, 21.00000000000002132, -123.2109808024214885 ) ) ;
#3404=ORIENTED_EDGE ( 'NONE', *, *, #6401, .F. ) ;
#3406=VECTOR ( 'NONE', #37790, 1000.000000000000000 ) ;
#3409=CARTESIAN_POINT ( 'NONE',  ( -3.500000000000002220, 15.47927405783632970, -88.57139747004409003 ) ) ;
#3410=( BOUNDED_CURVE ( )  B_SPLINE_CURVE ( 2, ( #19421, #9430, #19002, #16041, #12827, #19618, #22396, #26232, #9647 ),
 .UNSPECIFIED., .F., .T. ) 
 B_SPLINE_CURVE_WITH_KNOTS ( ( 3, 2, 2, 2, 3 ),
 ( 0.3604166666666666630, 0.3611111111111111049, 0.3624999999999999889, 0.3638888888888888729, 0.3645833333333333148 ),
 .UNSPECIFIED. ) 
 CURVE ( )  GEOMETRIC_REPRESENTATION_ITEM ( )  RATIONAL_B_SPLINE_CURVE ( ( 0.9330127018922194093, 0.9330127018922194093, 1.000000000000000000, 0.8660254037844387076, 1.000000000000000000, 0.8660254037844387076, 1.000000000000000000, 0.9330127018922194093, 0.9330127018922194093 ) ) 
 REPRESENTATION_ITEM ( '' )  );
#3411=CYLINDRICAL_SURFACE ( 'NONE', #23507, 3.499999999999999556 ) ;
#3412=CARTESIAN_POINT ( 'NONE',  ( 2.340729813953370519E-16, 21.32270188528332255, -132.0141058028994507 ) ) ;
#3414=VERTEX_POINT ( 'NONE', #31723 ) ;
#3415=CARTESIAN_POINT ( 'NONE',  ( 0.9378221735089281585, 14.00000000000000888, -28.66632260368298546 ) ) ;
#3416=EDGE_CURVE ( 'NONE', #37593, #33117, #39435, .T. ) ;
#3417=CARTESIAN_POINT ( 'NONE',  ( -1.655278471875002211, 14.63297358603755072, -119.6849391362327992 ) ) ;
#3418=EDGE_LOOP ( 'NONE', ( #15996, #15727, #32786, #27893 ) ) ;
#3419=CARTESIAN_POINT ( 'NONE',  ( -7.424026671074350129E-16, 13.45854811567264164, -130.4047308033774186 ) ) ;
#3420=CARTESIAN_POINT ( 'NONE',  ( -3.310556943750002645, 15.58864905735837070, -73.76827246956612782 ) ) ;
#3421=CARTESIAN_POINT ( 'NONE',  ( -1.749999999999999778, 20.53108891324555785, -121.1276474690881741 ) ) ;
#3422=CARTESIAN_POINT ( 'NONE',  ( -3.310556943750000425, 19.41135094264166838, -103.8474391362328220 ) ) ;
#3426=CARTESIAN_POINT ( 'NONE',  ( 1.749999999999998224, 14.46891108675447946, -73.62764746908817415 ) ) ;
#3427=CARTESIAN_POINT ( 'NONE',  ( -0.9378221735089291577, 21.00000000000001421, -51.16632260368298546 ) ) ;
#3428=CARTESIAN_POINT ( 'NONE',  ( 3.310556943750001313, 19.41135094264165772, -35.18077246956615056 ) ) ;
#3430=CARTESIAN_POINT ( 'NONE',  ( -3.310556943750000425, 19.41135094264166483, -95.93493913623279923 ) ) ;
#3431=CARTESIAN_POINT ( 'NONE',  ( -1.749999999999999778, 20.53108891324555074, -64.82139747004410424 ) ) ;
#3433=CARTESIAN_POINT ( 'NONE',  ( -3.310556943750002201, 15.58864905735837780, -119.7682724695661278 ) ) ;
#3439=CARTESIAN_POINT ( 'NONE',  ( -1.655278471875002211, 14.63297358603754894, -97.59743913623280775 ) ) ;
#3442=ORIENTED_EDGE ( 'NONE', *, *, #1510, .T. ) ;
#3443=CARTESIAN_POINT ( 'NONE',  ( 3.500000000000000000, 15.47927405783633503, -136.5443141357548598 ) ) ;
#3445=CARTESIAN_POINT ( 'NONE',  ( 3.500000000000001332, 17.50000000000002132, -123.1547308033774186 ) ) ;
#3447=CARTESIAN_POINT ( 'NONE',  ( -3.500000000000001332, 17.50000000000002487, -134.9609808024214885 ) ) ;
#3450=CARTESIAN_POINT ( 'NONE',  ( 1.655278471875001101, 20.36702641396248481, -28.09743913623280420 ) ) ;
#3456=CARTESIAN_POINT ( 'NONE',  ( 4.648177544792955347E-16, 21.00000000000001421, -58.21098080242150985 ) ) ;
#3457=EDGE_CURVE ( 'NONE', #19673, #31249, #23175, .T. ) ;
#3458=ORIENTED_EDGE ( 'NONE', *, *, #11550, .T. ) ;
#3461=CARTESIAN_POINT ( 'NONE',  ( -1.394453263437886604E-15, 14.00000000000001421, -70.40473080337741862 ) ) ;
#3462=CARTESIAN_POINT ( 'NONE',  ( 3.500000000000001776, 19.52072594216371826, -121.0713974700440900 ) ) ;
#3464=CARTESIAN_POINT ( 'NONE',  ( 1.655278471874998436, 14.63297358603755072, -135.5182724695661420 ) ) ;
#3465=CARTESIAN_POINT ( 'NONE',  ( 3.500000000000001332, 17.50000000000001066, -32.46098080242150274 ) ) ;
#3467=CARTESIAN_POINT ( 'NONE',  ( 1.750000000000001110, 20.53108891324554719, -32.29431413575484555 ) ) ;
#3468=CARTESIAN_POINT ( 'NONE',  ( 3.500000000000001332, 17.50000000000002132, -118.4609808024215170 ) ) ;
#3470=CARTESIAN_POINT ( 'NONE',  ( 1.750000000000001110, 20.53108891324556140, -140.2943141357548313 ) ) ;
#3471=CARTESIAN_POINT ( 'NONE',  ( -1.655278471874999990, 20.36702641396249547, -120.9307724695661364 ) ) ;
#3474=EDGE_CURVE ( 'NONE', #15451, #217, #22787, .T. ) ;
#3475=CARTESIAN_POINT ( 'NONE',  ( 4.648177544792955347E-16, 21.00000000000001776, -87.21098080242151696 ) ) ;
#3476=CARTESIAN_POINT ( 'NONE',  ( 2.474675557024783212E-16, 21.54145188432739744, -93.21098080242150274 ) ) ;
#3477=CARTESIAN_POINT ( 'NONE',  ( -3.500000000000000000, 19.52072594216370405, -37.04431413575484555 ) ) ;
#3478=CARTESIAN_POINT ( 'NONE',  ( -1.655278471875002211, 14.63297358603754184, -51.59743913623281486 ) ) ;
#3479=CARTESIAN_POINT ( 'NONE',  ( 3.310556943749999981, 15.58864905735837247, -109.4349391362327992 ) ) ;
#3480=EDGE_CURVE ( 'NONE', #17696, #12883, #14488, .T. ) ;
#3482=CARTESIAN_POINT ( 'NONE',  ( -1.749999999999999778, 20.53108891324554719, -33.82139747004410424 ) ) ;
#3485=CARTESIAN_POINT ( 'NONE',  ( 1.655278471874998436, 14.63297358603755072, -135.5182724695661420 ) ) ;
#3487=CARTESIAN_POINT ( 'NONE',  ( 0.9378221735089324884, 14.00000000000002665, -138.3600726046389298 ) ) ;
#3489=CARTESIAN_POINT ( 'NONE',  ( -3.310556943750000425, 19.41135094264166128, -69.93493913623279923 ) ) ;
#3491=CARTESIAN_POINT ( 'NONE',  ( 3.310556943750001313, 17.50000000000001421, -63.26410580289947205 ) ) ;
#3493=AXIS2_PLACEMENT_3D ( 'NONE', #4004, #11432, #36337 ) ;
#3494=CARTESIAN_POINT ( 'NONE',  ( 3.310556943749999981, 15.58864905735836892, -88.43493913623279923 ) ) ;
#3496=CARTESIAN_POINT ( 'NONE',  ( -1.749999999999999778, 20.53108891324555785, -103.8213974700440900 ) ) ;
#3498=CARTESIAN_POINT ( 'NONE',  ( -7.022189441860112050E-16, 13.67729811471671830, -44.51410580289947205 ) ) ;
#3500=CARTESIAN_POINT ( 'NONE',  ( 3.310556943750001313, 19.41135094264166838, -105.1807724695661364 ) ) ;
#3501=CARTESIAN_POINT ( 'NONE',  ( 4.648177544792955347E-16, 21.00000000000001421, -52.90473080337743284 ) ) ;
#3505=ADVANCED_FACE ( 'NONE', ( #31520 ), #15379, .T. ) ;
#3507=CARTESIAN_POINT ( 'NONE',  ( -3.310556943750002645, 15.58864905735836892, -59.68077246956615056 ) ) ;
#3511=CARTESIAN_POINT ( 'NONE',  ( 0.9378221735089281585, 14.00000000000000888, -31.66632260368298901 ) ) ;
#3512=EDGE_CURVE ( 'NONE', #27672, #23073, #16006, .T. ) ;
#3515=CARTESIAN_POINT ( 'NONE',  ( 3.369928719974892676E-15, 14.00000000000002309, -140.4047308033774186 ) ) ;
#3516=VERTEX_POINT ( 'NONE', #9613 ) ;
#3517=CARTESIAN_POINT ( 'NONE',  ( -1.394453263437886604E-15, 14.00000000000001066, -35.40473080337743284 ) ) ;
#3518=CARTESIAN_POINT ( 'NONE',  ( 1.655278471874998436, 14.63297358603755072, -125.4307724695661364 ) ) ;
#3521=CARTESIAN_POINT ( 'NONE',  ( 3.310556943749999981, 15.58864905735836182, -33.43493913623279923 ) ) ;
#3522=CARTESIAN_POINT ( 'NONE',  ( 3.310556943749999981, 15.58864905735836004, -24.43493913623280633 ) ) ;
#3523=CARTESIAN_POINT ( 'NONE',  ( -3.310556943750001313, 17.50000000000001776, -88.85160580289947063 ) ) ;
#3524=CARTESIAN_POINT ( 'NONE',  ( -3.310556943750000425, 19.41135094264167549, -140.8474391362327935 ) ) ;
#3528=CARTESIAN_POINT ( 'NONE',  ( 3.310556943750001313, 19.41135094264167549, -130.2682724695661136 ) ) ;
#3529=CARTESIAN_POINT ( 'NONE',  ( -3.310556943750000425, 19.41135094264166483, -89.84743913623280775 ) ) ;
#3530=CARTESIAN_POINT ( 'NONE',  ( 1.749999999999998224, 14.46891108675447413, -28.32139747004410069 ) ) ;
#3533=CARTESIAN_POINT ( 'NONE',  ( -3.500000000000000888, 19.52072594216371115, -77.73806413671076143 ) ) ;
#3535=CARTESIAN_POINT ( 'NONE',  ( 3.310556943749999981, 15.58864905735836537, -59.43493913623279212 ) ) ;
#3538=CARTESIAN_POINT ( 'NONE',  ( 4.286263797015737581E-16, 14.00000000000002487, -149.5231586289125687 ) ) ;
#3540=CARTESIAN_POINT ( 'NONE',  ( 3.310556943750001313, 19.41135094264166483, -85.26827246956612782 ) ) ;
#3543=CARTESIAN_POINT ( 'NONE',  ( 3.310556943750001313, 19.41135094264166838, -107.1807724695661364 ) ) ;
#3544=CARTESIAN_POINT ( 'NONE',  ( -1.655278471875002211, 14.63297358603754539, -80.59743913623280775 ) ) ;
#3546=CARTESIAN_POINT ( 'NONE',  ( 1.655278471875001101, 20.36702641396249547, -102.1849391362327992 ) ) ;
#3547=CARTESIAN_POINT ( 'NONE',  ( 2.474675557024783212E-16, 21.54145188432739744, -100.9047308033774328 ) ) ;
#3550=CARTESIAN_POINT ( 'NONE',  ( -3.500000000000000000, 19.52072594216371115, -94.73806413671074722 ) ) ;
#3551=CARTESIAN_POINT ( 'NONE',  ( -1.749999999999999778, 20.53108891324555429, -95.82139747004409003 ) ) ;
#3552=CARTESIAN_POINT ( 'NONE',  ( 4.648177544792955347E-16, 21.00000000000001421, -53.90473080337743284 ) ) ;
#3554=CARTESIAN_POINT ( 'NONE',  ( 1.655278471874998436, 14.63297358603754184, -65.43077246956615056 ) ) ;
#3556=CARTESIAN_POINT ( 'NONE',  ( 2.340729813953370519E-16, 21.32270188528331900, -123.0141058028994792 ) ) ;
#3557=CARTESIAN_POINT ( 'NONE',  ( -1.394453263437886604E-15, 14.00000000000001776, -106.4047308033774328 ) ) ;
#3560=CARTESIAN_POINT ( 'NONE',  ( 0.9378221735089281585, 14.00000000000002132, -99.66632260368297125 ) ) ;
#3561=CARTESIAN_POINT ( 'NONE',  ( 1.750000000000001110, 20.53108891324555785, -127.9880641367107614 ) ) ;
#3562=CARTESIAN_POINT ( 'NONE',  ( -1.655278471875002211, 14.63297358603754539, -71.59743913623280775 ) ) ;
#3563=ADVANCED_FACE ( 'NONE', ( #35552 ), #6414, .T. ) ;
#3565=ORIENTED_EDGE ( 'NONE', *, *, #26395, .F. ) ;
#3570=VECTOR ( 'NONE', #10318, 1000.000000000000000 ) ;
#3571=CARTESIAN_POINT ( 'NONE',  ( 3.310556943749999981, 15.58864905735837780, -141.3474391362327935 ) ) ;
#3573=CARTESIAN_POINT ( 'NONE',  ( 4.648177544792955347E-16, 21.00000000000001066, -42.90473080337742573 ) ) ;
#3574=CARTESIAN_POINT ( 'NONE',  ( -3.310556943750002645, 15.58864905735836537, -36.76827246956612782 ) ) ;
#3575=CARTESIAN_POINT ( 'NONE',  ( -3.310556943750002645, 15.58864905735837425, -102.7682724695661278 ) ) ;
#3576=CARTESIAN_POINT ( 'NONE',  ( -3.310556943750000425, 19.41135094264165772, -26.84743913623280420 ) ) ;
#3578=CARTESIAN_POINT ( 'NONE',  ( 1.749999999999998224, 14.46891108675448301, -101.6276474690881741 ) ) ;
#3580=DIRECTION ( 'NONE',  ( -0.000000000000000000, 1.259100132267607459E-16, -1.000000000000000000 ) ) ;
#3581=CARTESIAN_POINT ( 'NONE',  ( 1.750000000000001110, 20.53108891324555429, -91.98806413671076143 ) ) ;
#3586=CARTESIAN_POINT ( 'NONE',  ( 2.474675557024783212E-16, 21.54145188432739388, -54.21098080242150985 ) ) ;
#3588=DIRECTION ( 'NONE',  ( -0.000000000000000000, 1.259100132267607459E-16, -1.000000000000000000 ) ) ;
#3589=ADVANCED_FACE ( 'NONE', ( #4271 ), #873, .T. ) ;
#3590=CARTESIAN_POINT ( 'NONE',  ( 3.500000000000001776, 19.52072594216370405, -44.07139747004410424 ) ) ;
#3592=EDGE_CURVE ( 'NONE', #5926, #13090, #10229, .T. ) ;
#3593=CARTESIAN_POINT ( 'NONE',  ( -3.310556943750002201, 15.58864905735836537, -28.76827246956614559 ) ) ;
#3599=CARTESIAN_POINT ( 'NONE',  ( 3.500000000000001332, 19.52072594216371826, -102.0713974700440758 ) ) ;
#3601=CARTESIAN_POINT ( 'NONE',  ( -3.310556943750000425, 19.41135094264166838, -80.84743913623280775 ) ) ;
#3604=VERTEX_POINT ( 'NONE', #23422 ) ;
#3605=CARTESIAN_POINT ( 'NONE',  ( -0.9378221735089291577, 21.00000000000001066, -35.86007260463890844 ) ) ;
#3606=CARTESIAN_POINT ( 'NONE',  ( 3.500000000000001332, 19.52072594216371115, -87.37764746908817415 ) ) ;
#3610=CARTESIAN_POINT ( 'NONE',  ( -3.310556943750001313, 17.50000000000001776, -89.76410580289947916 ) ) ;
#3611=( BOUNDED_CURVE ( )  B_SPLINE_CURVE ( 2, ( #15437, #31786, #22018, #8619, #12445, #28391, #5855, #25428, #40953 ),
 .UNSPECIFIED., .F., .T. ) 
 B_SPLINE_CURVE_WITH_KNOTS ( ( 3, 2, 2, 2, 3 ),
 ( 0.2354166666666666630, 0.2361111111111111049, 0.2374999999999999889, 0.2388888888888889006, 0.2395833333333333426 ),
 .UNSPECIFIED. ) 
 CURVE ( )  GEOMETRIC_REPRESENTATION_ITEM ( )  RATIONAL_B_SPLINE_CURVE ( ( 0.9330127018922194093, 0.9330127018922194093, 1.000000000000000000, 0.8660254037844387076, 1.000000000000000000, 0.8660254037844387076, 1.000000000000000000, 0.9330127018922194093, 0.9330127018922194093 ) ) 
 REPRESENTATION_ITEM ( '' )  );
#3613=ORIENTED_EDGE ( 'NONE', *, *, #31825, .T. ) ;
#3615=CARTESIAN_POINT ( 'NONE',  ( -3.500000000000001332, 17.50000000000002132, -127.6547308033774186 ) ) ;
#3616=CARTESIAN_POINT ( 'NONE',  ( -2.324088772396477673E-16, 14.00000000000002309, -142.7109808024215170 ) ) ;
#3617=CARTESIAN_POINT ( 'NONE',  ( -3.310556943750000425, 19.41135094264167549, -130.8474391362328220 ) ) ;
#3618=VERTEX_POINT ( 'NONE', #26825 ) ;
#3619=ORIENTED_EDGE ( 'NONE', *, *, #36533, .T. ) ;
#3622=CARTESIAN_POINT ( 'NONE',  ( 3.310556943749999981, 15.58864905735837247, -120.4349391362327850 ) ) ;
#3623=ORIENTED_EDGE ( 'NONE', *, *, #41512, .T. ) ;
#3625=ORIENTED_EDGE ( 'NONE', *, *, #39475, .T. ) ;
#3626=CARTESIAN_POINT ( 'NONE',  ( -1.749999999999999778, 20.53108891324556140, -130.8213974700441042 ) ) ;
#3627=AXIS2_PLACEMENT_3D ( 'NONE', #29452, #6081, #32242 ) ;
#3628=CARTESIAN_POINT ( 'NONE',  ( -1.655278471874999990, 20.36702641396248836, -71.01827246956612782 ) ) ;
#3629=CARTESIAN_POINT ( 'NONE',  ( 1.750000000000001110, 20.53108891324555785, -118.2943141357548313 ) ) ;
#3631=CARTESIAN_POINT ( 'NONE',  ( -1.655278471874999990, 20.36702641396249192, -99.93077246956613635 ) ) ;
#3632=DIRECTION ( 'NONE',  ( 0.000000000000000000, 1.000000000000000000, 0.000000000000000000 ) ) ;
#3633=CARTESIAN_POINT ( 'NONE',  ( 3.500000000000001332, 19.52072594216371826, -105.3776474690881599 ) ) ;
#3635=CARTESIAN_POINT ( 'NONE',  ( -3.500000000000000888, 19.52072594216370760, -70.04431413575484555 ) ) ;
#3637=CARTESIAN_POINT ( 'NONE',  ( 3.310556943750001313, 19.41135094264165772, -39.18077246956613635 ) ) ;
#3638=CARTESIAN_POINT ( 'NONE',  ( 2.340729813953370519E-16, 21.32270188528331190, -98.10160580289947063 ) ) ;
#3639=CARTESIAN_POINT ( 'NONE',  ( 3.500000000000000000, 15.47927405783632260, -59.23806413671076854 ) ) ;
#3640=CARTESIAN_POINT ( 'NONE',  ( -1.655278471874999990, 20.36702641396249547, -116.0182724695661278 ) ) ;
#3645=CARTESIAN_POINT ( 'NONE',  ( 0.9378221735089300459, 21.00000000000001776, -79.25563900116003424 ) ) ;
#3647=CARTESIAN_POINT ( 'NONE',  ( -7.022189441860112050E-16, 13.67729811471672541, -99.51410580289947916 ) ) ;
#3648=LINE ( 'NONE', #29807, #35575 ) ;
#3650=EDGE_LOOP ( 'NONE', ( #22980, #10148, #13657, #21090 ) ) ;
#3651=CARTESIAN_POINT ( 'NONE',  ( -1.749999999999999778, 20.53108891324555429, -87.82139747004409003 ) ) ;
#3652=CARTESIAN_POINT ( 'NONE',  ( -0.9378221735089310451, 14.00000000000002309, -118.4493890021159501 ) ) ;
#3654=CARTESIAN_POINT ( 'NONE',  ( -0.9378221735089291577, 21.00000000000001421, -71.16632260368299967 ) ) ;
#3655=ORIENTED_EDGE ( 'NONE', *, *, #37800, .T. ) ;
#3658=EDGE_CURVE ( 'NONE', #28199, #28655, #13626, .T. ) ;
#3660=CARTESIAN_POINT ( 'NONE',  ( -1.655278471874999990, 20.36702641396248481, -28.93077246956614346 ) ) ;
#3661=VERTEX_POINT ( 'NONE', #19795 ) ;
#3663=( BOUNDED_CURVE ( )  B_SPLINE_CURVE ( 2, ( #11006, #40759, #37169, #20995, #33966, #24399, #5029, #11616, #20367 ),
 .UNSPECIFIED., .F., .T. ) 
 B_SPLINE_CURVE_WITH_KNOTS ( ( 3, 2, 2, 2, 3 ),
 ( 0.2770833333333333481, 0.2777777777777777901, 0.2791666666666666741, 0.2805555555555555580, 0.2812500000000000000 ),
 .UNSPECIFIED. ) 
 CURVE ( )  GEOMETRIC_REPRESENTATION_ITEM ( )  RATIONAL_B_SPLINE_CURVE ( ( 0.9330127018922194093, 0.9330127018922194093, 1.000000000000000000, 0.8660254037844387076, 1.000000000000000000, 0.8660254037844387076, 1.000000000000000000, 0.9330127018922194093, 0.9330127018922194093 ) ) 
 REPRESENTATION_ITEM ( '' )  );
#3664=VECTOR ( 'NONE', #2933, 1000.000000000000000 ) ;
#3667=CARTESIAN_POINT ( 'NONE',  ( 4.648177544792955347E-16, 21.00000000000002487, -138.9047308033774186 ) ) ;
#3670=CYLINDRICAL_SURFACE ( 'NONE', #3127, 3.499999999999999556 ) ;
#3671=CARTESIAN_POINT ( 'NONE',  ( 0.9378221735089302680, 14.00000000000002132, -140.6663226036829712 ) ) ;
#3672=CARTESIAN_POINT ( 'NONE',  ( 3.500000000000001332, 17.50000000000002132, -121.1547308033774328 ) ) ;
#3674=CARTESIAN_POINT ( 'NONE',  ( -7.022189441860112050E-16, 13.67729811471672718, -133.6016058028994564 ) ) ;
#3675=CARTESIAN_POINT ( 'NONE',  ( 1.749999999999998224, 14.46891108675447413, -26.62764746908817415 ) ) ;
#3678=CARTESIAN_POINT ( 'NONE',  ( 4.648177544792955347E-16, 21.00000000000001066, -32.21098080242150274 ) ) ;
#3680=CARTESIAN_POINT ( 'NONE',  ( 1.750000000000001110, 20.53108891324556140, -142.2943141357548313 ) ) ;
#3682=CARTESIAN_POINT ( 'NONE',  ( 3.500000000000000000, 15.47927405783633503, -131.5443141357548313 ) ) ;
#3683=CARTESIAN_POINT ( 'NONE',  ( 3.310556943750001313, 17.50000000000002132, -118.2641058028994792 ) ) ;
#3686=CARTESIAN_POINT ( 'NONE',  ( 4.648177544792955347E-16, 21.00000000000001066, -36.90473080337743284 ) ) ;
#3687=CARTESIAN_POINT ( 'NONE',  ( -3.500000000000000888, 19.52072594216371115, -89.04431413575484555 ) ) ;
#3688=CARTESIAN_POINT ( 'NONE',  ( -3.500000000000000000, 19.52072594216370405, -41.04431413575483845 ) ) ;
#3689=CARTESIAN_POINT ( 'NONE',  ( -3.310556943750002645, 15.58864905735836892, -54.68077246956613635 ) ) ;
#3690=CARTESIAN_POINT ( 'NONE',  ( 3.310556943750001313, 19.41135094264166838, -113.2682724695661562 ) ) ;
#3692=CARTESIAN_POINT ( 'NONE',  ( 1.750000000000001110, 20.53108891324554719, -29.98806413671076143 ) ) ;
#3695=CARTESIAN_POINT ( 'NONE',  ( -7.022189441860112050E-16, 13.67729811471672896, -131.6016058028994564 ) ) ;
#3697=DIRECTION ( 'NONE',  ( -0.000000000000000000, 1.259100132267607459E-16, -1.000000000000000000 ) ) ;
#3699=CARTESIAN_POINT ( 'NONE',  ( 2.340729813953370519E-16, 21.32270188528330834, -64.10160580289945642 ) ) ;
#3701=CARTESIAN_POINT ( 'NONE',  ( 3.310556943750001313, 17.50000000000001421, -66.26410580289947916 ) ) ;
#3703=CARTESIAN_POINT ( 'NONE',  ( -1.655278471874999990, 20.36702641396249192, -84.01827246956614204 ) ) ;
#3705=CARTESIAN_POINT ( 'NONE',  ( -0.9378221735089310451, 14.00000000000002132, -103.4493890021159501 ) ) ;
#3707=CARTESIAN_POINT ( 'NONE',  ( -3.310556943750002201, 15.58864905735836714, -46.68077246956614346 ) ) ;
#3709=CARTESIAN_POINT ( 'NONE',  ( -7.022189441860112050E-16, 13.67729811471672541, -98.51410580289947916 ) ) ;
#3710=DIRECTION ( 'NONE',  ( -0.000000000000000000, 1.259100132267607459E-16, -1.000000000000000000 ) ) ;
#3715=CARTESIAN_POINT ( 'NONE',  ( 3.310556943750001313, 19.41135094264166128, -56.18077246956613635 ) ) ;
#3716=EDGE_LOOP ( 'NONE', ( #23019, #38721 ) ) ;
#3721=EDGE_CURVE ( 'NONE', #12825, #37421, #24808, .T. ) ;
#3724=CARTESIAN_POINT ( 'NONE',  ( -0.9378221735089288247, 14.00000000000002309, -140.4493890021159643 ) ) ;
#3726=VERTEX_POINT ( 'NONE', #21477 ) ;
#3727=CARTESIAN_POINT ( 'NONE',  ( 2.474675557024783212E-16, 21.54145188432739033, -44.21098080242150985 ) ) ;
#3728=CARTESIAN_POINT ( 'NONE',  ( -1.655278471874999990, 20.36702641396248481, -43.93077246956614346 ) ) ;
#3729=CARTESIAN_POINT ( 'NONE',  ( -3.500000000000000000, 19.52072594216370405, -39.04431413575484555 ) ) ;
#3730=CARTESIAN_POINT ( 'NONE',  ( 0.000000000000000000, 21.00000000000002487, -149.5231586289125687 ) ) ;
#3732=CARTESIAN_POINT ( 'NONE',  ( -7.022189441860112050E-16, 13.67729811471671475, -32.60160580289946353 ) ) ;
#3734=CARTESIAN_POINT ( 'NONE',  ( -3.310556943750002645, 15.58864905735837247, -82.76827246956615625 ) ) ;
#3735=CARTESIAN_POINT ( 'NONE',  ( -3.310556943750000425, 19.41135094264167549, -131.8474391362327935 ) ) ;
#3737=FACE_OUTER_BOUND ( 'NONE', #35980, .T. ) ;
#3738=CARTESIAN_POINT ( 'NONE',  ( -1.749999999999999778, 20.53108891324555074, -67.12764746908817415 ) ) ;
#3739=CARTESIAN_POINT ( 'NONE',  ( 3.310556943750001313, 17.50000000000002132, -129.3516058028994564 ) ) ;
#3742=CARTESIAN_POINT ( 'NONE',  ( -1.655278471874999990, 20.36702641396249192, -88.93077246956613635 ) ) ;
#3744=CARTESIAN_POINT ( 'NONE',  ( -3.500000000000000000, 19.52072594216371826, -126.0443141357548456 ) ) ;
#3746=CARTESIAN_POINT ( 'NONE',  ( -1.750000000000002220, 14.46891108675448123, -76.48806413671076143 ) ) ;
#3748=CARTESIAN_POINT ( 'NONE',  ( -1.655278471874999990, 20.36702641396248836, -60.01827246956613493 ) ) ;
#3752=CARTESIAN_POINT ( 'NONE',  ( -3.310556943750001313, 17.50000000000001776, -80.85160580289945642 ) ) ;
#3753=CARTESIAN_POINT ( 'NONE',  ( 0.000000000000000000, 17.50000000000002487, -149.5231586289125687 ) ) ;
#3755=CARTESIAN_POINT ( 'NONE',  ( -3.310556943750000425, 19.41135094264166838, -109.8474391362328220 ) ) ;
#3756=CARTESIAN_POINT ( 'NONE',  ( -1.655278471875002211, 14.63297358603754539, -78.59743913623280775 ) ) ;
#3757=CARTESIAN_POINT ( 'NONE',  ( 1.749999999999998224, 14.46891108675447768, -57.32139747004409713 ) ) ;
#3758=ORIENTED_EDGE ( 'NONE', *, *, #38327, .F. ) ;
#3759=CARTESIAN_POINT ( 'NONE',  ( 3.310556943750001313, 19.41135094264166838, -100.2682724695661278 ) ) ;
#3761=CARTESIAN_POINT ( 'NONE',  ( 1.749999999999998224, 14.46891108675448301, -104.3213974700441042 ) ) ;
#3763=CARTESIAN_POINT ( 'NONE',  ( 0.9378221735089300459, 21.00000000000001421, -71.25563900116000582 ) ) ;
#3764=CARTESIAN_POINT ( 'NONE',  ( -0.9378221735089291577, 21.00000000000001066, -38.16632260368297835 ) ) ;
#3767=CARTESIAN_POINT ( 'NONE',  ( 3.310556943750001313, 17.50000000000001421, -63.26410580289947205 ) ) ;
#3768=CARTESIAN_POINT ( 'NONE',  ( -3.500000000000000000, 19.52072594216370405, -30.04431413575484200 ) ) ;
#3769=CARTESIAN_POINT ( 'NONE',  ( 1.655278471874998436, 14.63297358603754894, -121.4307724695661364 ) ) ;
#3770=LINE ( 'NONE', #800, #36623 ) ;
#3773=ORIENTED_EDGE ( 'NONE', *, *, #20326, .T. ) ;
#3775=CARTESIAN_POINT ( 'NONE',  ( -1.394453263437886604E-15, 14.00000000000002132, -131.4047308033774186 ) ) ;
#3776=CARTESIAN_POINT ( 'NONE',  ( 4.648177544792955347E-16, 21.00000000000001776, -78.90473080337741862 ) ) ;
#3778=CARTESIAN_POINT ( 'NONE',  ( 1.655278471874998436, 14.63297358603754361, -76.43077246956615056 ) ) ;
#3779=ORIENTED_EDGE ( 'NONE', *, *, #15735, .F. ) ;
#3780=VERTEX_POINT ( 'NONE', #41045 ) ;
#3781=EDGE_CURVE ( 'NONE', #24201, #10062, #16116, .T. ) ;
#3783=ADVANCED_FACE ( 'NONE', ( #8088 ), #21065, .T. ) ;
#3785=CARTESIAN_POINT ( 'NONE',  ( 2.340729813953370519E-16, 21.32270188528332255, -139.0141058028994792 ) ) ;
#3786=LINE ( 'NONE', #19958, #17636 ) ;
#3787=( BOUNDED_CURVE ( )  B_SPLINE_CURVE ( 2, ( #15513, #28468, #41459, #19959, #16980, #29303, #3789, #13791, #19533 ),
 .UNSPECIFIED., .F., .T. ) 
 B_SPLINE_CURVE_WITH_KNOTS ( ( 3, 2, 2, 2, 3 ),
 ( 0.4437499999999999778, 0.4444444444444444198, 0.4458333333333333592, 0.4472222222222222432, 0.4479166666666666852 ),
 .UNSPECIFIED. ) 
 CURVE ( )  GEOMETRIC_REPRESENTATION_ITEM ( )  RATIONAL_B_SPLINE_CURVE ( ( 0.9330127018922194093, 0.9330127018922194093, 1.000000000000000000, 0.8660254037844387076, 1.000000000000000000, 0.8660254037844387076, 1.000000000000000000, 0.9330127018922194093, 0.9330127018922194093 ) ) 
 REPRESENTATION_ITEM ( '' )  );
#3788=VECTOR ( 'NONE', #21311, 1000.000000000000000 ) ;
#3789=CARTESIAN_POINT ( 'NONE',  ( -1.750000000000002220, 14.46891108675448301, -89.48806413671076143 ) ) ;
#3790=CARTESIAN_POINT ( 'NONE',  ( -3.310556943750000425, 19.41135094264165772, -35.93493913623279923 ) ) ;
#3791=CARTESIAN_POINT ( 'NONE',  ( 3.310556943750001313, 19.41135094264166838, -102.2682724695661278 ) ) ;
#3793=CARTESIAN_POINT ( 'NONE',  ( -1.655278471875002211, 14.63297358603755427, -141.6849391362327708 ) ) ;
#3795=CARTESIAN_POINT ( 'NONE',  ( -1.749999999999999778, 20.53108891324555429, -100.1276474690881741 ) ) ;
#3798=CARTESIAN_POINT ( 'NONE',  ( -1.749999999999999778, 20.53108891324555429, -92.82139747004409003 ) ) ;
#3802=EDGE_CURVE ( 'NONE', #12140, #34390, #14740, .T. ) ;
#3804=CARTESIAN_POINT ( 'NONE',  ( -3.500000000000000888, 19.52072594216370760, -56.04431413575484555 ) ) ;
#3808=CARTESIAN_POINT ( 'NONE',  ( 2.474675557024783212E-16, 21.54145188432739033, -44.90473080337743994 ) ) ;
#3810=ADVANCED_FACE ( 'NONE', ( #40832 ), #5310, .T. ) ;
#3811=CARTESIAN_POINT ( 'NONE',  ( -1.655278471875002211, 14.63297358603754006, -28.68493913623279568 ) ) ;
#3814=CARTESIAN_POINT ( 'NONE',  ( -3.500000000000001332, 17.50000000000001421, -60.65473080337742573 ) ) ;
#3818=CARTESIAN_POINT ( 'NONE',  ( 2.340729813953370519E-16, 21.32270188528331190, -76.01410580289945074 ) ) ;
#3819=CARTESIAN_POINT ( 'NONE',  ( -3.500000000000002220, 15.47927405783633503, -141.5713974700441042 ) ) ;
#3824=VERTEX_POINT ( 'NONE', #4486 ) ;
#3826=CARTESIAN_POINT ( 'NONE',  ( -3.310556943750002645, 15.58864905735837247, -89.68077246956615056 ) ) ;
#3827=EDGE_LOOP ( 'NONE', ( #28927, #37999, #4469, #32499 ) ) ;
#3834=CARTESIAN_POINT ( 'NONE',  ( -1.655278471875002211, 14.63297358603755249, -124.5974391362328078 ) ) ;
#3837=CARTESIAN_POINT ( 'NONE',  ( 3.310556943749999981, 15.58864905735836537, -56.43493913623279212 ) ) ;
#3838=CARTESIAN_POINT ( 'NONE',  ( -3.310556943750001313, 17.50000000000002132, -121.8516058028994706 ) ) ;
#3841=CARTESIAN_POINT ( 'NONE',  ( -1.750000000000002220, 14.46891108675448834, -124.4880641367107614 ) ) ;
#3842=CARTESIAN_POINT ( 'NONE',  ( 3.310556943750001313, 17.50000000000001066, -41.26410580289947916 ) ) ;
#3843=CARTESIAN_POINT ( 'NONE',  ( -7.022189441860112050E-16, 13.67729811471672186, -72.60160580289947063 ) ) ;
#3844=CARTESIAN_POINT ( 'NONE',  ( 3.500000000000000000, 15.47927405783632970, -116.5443141357548456 ) ) ;
#3845=CARTESIAN_POINT ( 'NONE',  ( 2.340729813953370519E-16, 21.32270188528331900, -103.0141058028994792 ) ) ;
#3846=ADVANCED_FACE ( 'NONE', ( #31881 ), #15733, .T. ) ;
#3850=CARTESIAN_POINT ( 'NONE',  ( 1.750000000000001110, 20.53108891324555074, -68.29431413575484555 ) ) ;
#3851=CARTESIAN_POINT ( 'NONE',  ( 3.500000000000000000, 15.47927405783632970, -100.5443141357548456 ) ) ;
#3852=CARTESIAN_POINT ( 'NONE',  ( -7.022189441860112050E-16, 13.67729811471671475, -36.51410580289947205 ) ) ;
#3853=CARTESIAN_POINT ( 'NONE',  ( -3.310556943750001313, 17.50000000000001776, -93.85160580289947063 ) ) ;
#3855=CARTESIAN_POINT ( 'NONE',  ( 1.749999999999998224, 14.46891108675447768, -60.32139747004409713 ) ) ;
#3857=CARTESIAN_POINT ( 'NONE',  ( 3.310556943749999981, 15.58864905735837247, -112.4349391362327992 ) ) ;
#3858=CARTESIAN_POINT ( 'NONE',  ( -7.022189441860112050E-16, 13.67729811471671830, -43.60160580289947063 ) ) ;
#3865=CARTESIAN_POINT ( 'NONE',  ( -3.310556943750000425, 19.41135094264166838, -100.8474391362328220 ) ) ;
#3866=( BOUNDED_CURVE ( )  B_SPLINE_CURVE ( 2, ( #15593, #41540, #22177, #5595, #17942, #5806, #24963, #1778, #14761 ),
 .UNSPECIFIED., .F., .F. ) 
 B_SPLINE_CURVE_WITH_KNOTS ( ( 3, 2, 2, 2, 3 ),
 ( 0.5937500000000000000, 0.5944444444444444420, 0.5958333333333333259, 0.5972222222222222099, 0.5979166666666666519 ),
 .UNSPECIFIED. ) 
 CURVE ( )  GEOMETRIC_REPRESENTATION_ITEM ( )  RATIONAL_B_SPLINE_CURVE ( ( 0.9330127018922194093, 0.9330127018922194093, 1.000000000000000000, 0.8660254037844387076, 1.000000000000000000, 0.8660254037844387076, 1.000000000000000000, 0.9330127018922194093, 0.9330127018922194093 ) ) 
 REPRESENTATION_ITEM ( '' )  );
#3869=VERTEX_POINT ( 'NONE', #32096 ) ;
#3870=CARTESIAN_POINT ( 'NONE',  ( 3.500000000000001332, 17.50000000000002487, -136.4609808024214885 ) ) ;
#3872=CYLINDRICAL_SURFACE ( 'NONE', #2702, 3.499999999999999556 ) ;
#3877=CARTESIAN_POINT ( 'NONE',  ( 2.340729813953370519E-16, 21.32270188528330834, -31.01410580289946850 ) ) ;
#3879=CARTESIAN_POINT ( 'NONE',  ( 4.286263797015737581E-16, 14.00000000000002487, -149.5231586289125687 ) ) ;
#3886=CARTESIAN_POINT ( 'NONE',  ( 2.340729813953370519E-16, 21.32270188528332255, -141.0141058028994792 ) ) ;
#3888=CARTESIAN_POINT ( 'NONE',  ( 2.340729813953370519E-16, 21.32270188528332255, -135.1016058028994564 ) ) ;
#3889=CARTESIAN_POINT ( 'NONE',  ( 1.750000000000001110, 20.53108891324554719, -29.29431413575483845 ) ) ;
#3891=CARTESIAN_POINT ( 'NONE',  ( -1.749999999999999778, 20.53108891324556140, -140.8213974700441042 ) ) ;
#3893=CARTESIAN_POINT ( 'NONE',  ( 3.500000000000001332, 17.50000000000002487, -135.4609808024214885 ) ) ;
#3894=CARTESIAN_POINT ( 'NONE',  ( -3.310556943750000425, 19.41135094264166838, -117.8474391362327935 ) ) ;
#3899=CARTESIAN_POINT ( 'NONE',  ( -1.750000000000002220, 14.46891108675448301, -84.79431413575483134 ) ) ;
#3900=DIRECTION ( 'NONE',  ( -0.000000000000000000, 1.259100132267607459E-16, -1.000000000000000000 ) ) ;
#3901=CARTESIAN_POINT ( 'NONE',  ( 3.310556943749999981, 15.58864905735836182, -53.34743913623280775 ) ) ;
#3902=CARTESIAN_POINT ( 'NONE',  ( 3.310556943750001313, 17.50000000000002132, -110.3516058028994564 ) ) ;
#3903=CARTESIAN_POINT ( 'NONE',  ( 4.286263797015737581E-16, 14.00000000000002487, -149.5231586289125687 ) ) ;
#3904=CARTESIAN_POINT ( 'NONE',  ( -1.750000000000002220, 14.46891108675447590, -28.48806413671076143 ) ) ;
#3907=CARTESIAN_POINT ( 'NONE',  ( 1.655278471875001101, 20.36702641396249902, -136.1849391362327992 ) ) ;
#3910=CYLINDRICAL_SURFACE ( 'NONE', #37379, 3.499999999999999556 ) ;
#3911=CARTESIAN_POINT ( 'NONE',  ( 3.310556943750001313, 17.50000000000001421, -63.35160580289946353 ) ) ;
#3913=CARTESIAN_POINT ( 'NONE',  ( 1.655278471875001101, 20.36702641396248836, -64.09743913623280775 ) ) ;
#3915=( BOUNDED_CURVE ( )  B_SPLINE_CURVE ( 2, ( #24195, #4408, #1013, #10783, #37162, #40551, #7814, #30768, #39711 ),
 .UNSPECIFIED., .F., .T. ) 
 B_SPLINE_CURVE_WITH_KNOTS ( ( 3, 2, 2, 2, 3 ),
 ( 0.1520833333333333481, 0.1527777777777777901, 0.1541666666666666741, 0.1555555555555555580, 0.1562500000000000000 ),
 .UNSPECIFIED. ) 
 CURVE ( )  GEOMETRIC_REPRESENTATION_ITEM ( )  RATIONAL_B_SPLINE_CURVE ( ( 0.9330127018922194093, 0.9330127018922207416, 1.000000000000000000, 0.8660254037844387076, 1.000000000000000000, 0.8660254037844387076, 1.000000000000000000, 0.9330127018922194093, 0.9330127018922194093 ) ) 
 REPRESENTATION_ITEM ( '' )  );
#3916=CARTESIAN_POINT ( 'NONE',  ( 3.310556943749999981, 15.58864905735836892, -85.43493913623277081 ) ) ;
#3918=CARTESIAN_POINT ( 'NONE',  ( -1.394453263437886604E-15, 14.00000000000001066, -44.71098080242150985 ) ) ;
#3920=CARTESIAN_POINT ( 'NONE',  ( 3.310556943749999981, 15.58864905735836182, -45.34743913623280775 ) ) ;
#3922=CARTESIAN_POINT ( 'NONE',  ( -1.655278471875002211, 14.63297358603754894, -99.59743913623280775 ) ) ;
#3924=EDGE_LOOP ( 'NONE', ( #6907, #12342, #36973, #11987 ) ) ;
#3927=EDGE_CURVE ( 'NONE', #9764, #25787, #26171, .T. ) ;
#3929=CARTESIAN_POINT ( 'NONE',  ( 3.310556943750001313, 17.50000000000001421, -50.26410580289947205 ) ) ;
#3930=ORIENTED_EDGE ( 'NONE', *, *, #27776, .T. ) ;
#3932=DIRECTION ( 'NONE',  ( -0.000000000000000000, 1.259100132267607459E-16, -1.000000000000000000 ) ) ;
#3935=CARTESIAN_POINT ( 'NONE',  ( -0.9378221735089291577, 21.00000000000002487, -140.8600726046389013 ) ) ;
#3938=CARTESIAN_POINT ( 'NONE',  ( 1.750000000000001110, 20.53108891324554719, -43.29431413575483845 ) ) ;
#3939=CARTESIAN_POINT ( 'NONE',  ( 2.340729813953370519E-16, 21.32270188528330479, -44.01410580289947916 ) ) ;
#3940=CARTESIAN_POINT ( 'NONE',  ( 4.648177544792955347E-16, 21.00000000000001066, -34.90473080337743284 ) ) ;
#3941=CARTESIAN_POINT ( 'NONE',  ( -1.394453263437886604E-15, 14.00000000000002132, -133.4047308033774186 ) ) ;
#3943=CARTESIAN_POINT ( 'NONE',  ( 1.655278471875001101, 20.36702641396248481, -31.18493913623279923 ) ) ;
#3944=CARTESIAN_POINT ( 'NONE',  ( -3.310556943750000425, 19.41135094264165772, -23.93493913623280278 ) ) ;
#3945=CARTESIAN_POINT ( 'NONE',  ( 2.340729813953370519E-16, 21.32270188528331190, -80.10160580289947063 ) ) ;
#3946=CARTESIAN_POINT ( 'NONE',  ( -3.310556943750000425, 19.41135094264167549, -132.8474391362328220 ) ) ;
#3951=VECTOR ( 'NONE', #13807, 1000.000000000000000 ) ;
#3952=CARTESIAN_POINT ( 'NONE',  ( -3.310556943750002645, 15.58864905735837780, -126.7682724695661420 ) ) ;
#3953=DIRECTION ( 'NONE',  ( 0.000000000000000000, 1.000000000000000000, 0.000000000000000000 ) ) ;
#3954=CARTESIAN_POINT ( 'NONE',  ( -3.310556943750001313, 17.50000000000001776, -84.76410580289947916 ) ) ;
#3955=FACE_OUTER_BOUND ( 'NONE', #26193, .T. ) ;
#3958=CARTESIAN_POINT ( 'NONE',  ( -3.500000000000002220, 15.47927405783632615, -77.57139747004410424 ) ) ;
#3959=CARTESIAN_POINT ( 'NONE',  ( -1.655278471875002211, 14.63297358603754361, -59.68493913623279212 ) ) ;
#3963=CARTESIAN_POINT ( 'NONE',  ( 1.655278471875001101, 20.36702641396249192, -81.18493913623279923 ) ) ;
#3964=CARTESIAN_POINT ( 'NONE',  ( 1.655278471875001101, 20.36702641396249902, -142.1849391362327992 ) ) ;
#3966=CARTESIAN_POINT ( 'NONE',  ( 3.310556943750001313, 19.41135094264166838, -108.1807724695661648 ) ) ;
#3967=CARTESIAN_POINT ( 'NONE',  ( 1.655278471875001101, 20.36702641396249192, -79.09743913623280775 ) ) ;
#3970=CARTESIAN_POINT ( 'NONE',  ( 2.340729813953370519E-16, 21.32270188528331900, -104.1016058028994422 ) ) ;
#3971=CARTESIAN_POINT ( 'NONE',  ( 1.749999999999998224, 14.46891108675448301, -105.3213974700441042 ) ) ;
#3976=CARTESIAN_POINT ( 'NONE',  ( 1.655278471875001101, 20.36702641396248836, -62.09743913623280775 ) ) ;
#3978=CARTESIAN_POINT ( 'NONE',  ( -7.022189441860112050E-16, 13.67729811471672718, -116.5141058028994792 ) ) ;
#3979=DIRECTION ( 'NONE',  ( -0.000000000000000000, 1.259100132267607459E-16, -1.000000000000000000 ) ) ;
#3980=AXIS2_PLACEMENT_3D ( 'NONE', #12513, #22924, #25276 ) ;
#3982=VERTEX_POINT ( 'NONE', #22520 ) ;
#3986=CARTESIAN_POINT ( 'NONE',  ( 1.743066579297357930E-14, 14.00000000000002132, -128.4047308033774186 ) ) ;
#3987=CARTESIAN_POINT ( 'NONE',  ( 3.310556943750001313, 17.50000000000001421, -67.26410580289947916 ) ) ;
#3989=VERTEX_POINT ( 'NONE', #21682 ) ;
#3992=VERTEX_POINT ( 'NONE', #2750 ) ;
#3994=CARTESIAN_POINT ( 'NONE',  ( -7.022189441860112050E-16, 13.67729811471673074, -137.5141058028994792 ) ) ;
#3996=CARTESIAN_POINT ( 'NONE',  ( 3.310556943750001313, 19.41135094264165772, -44.26827246956613493 ) ) ;
#3997=CARTESIAN_POINT ( 'NONE',  ( 3.310556943750001313, 17.50000000000001066, -36.35160580289946353 ) ) ;
#3998=CARTESIAN_POINT ( 'NONE',  ( -7.022189441860112050E-16, 13.67729811471672541, -98.60160580289947063 ) ) ;
#4001=CARTESIAN_POINT ( 'NONE',  ( -7.022189441860112050E-16, 13.67729811471671297, -25.51410580289947916 ) ) ;
#4002=CARTESIAN_POINT ( 'NONE',  ( 1.750000000000001110, 20.53108891324555785, -121.2943141357548313 ) ) ;
#4003=CARTESIAN_POINT ( 'NONE',  ( 3.500000000000001332, 17.50000000000002132, -104.4609808024215027 ) ) ;
#4004=CARTESIAN_POINT ( 'NONE',  ( 0.000000000000000000, 17.50000000000002487, -149.5231586289125687 ) ) ;
#4005=CARTESIAN_POINT ( 'NONE',  ( 0.9378221735089290467, 21.00000000000002842, -141.9493890021159643 ) ) ;
#4006=CARTESIAN_POINT ( 'NONE',  ( 1.749999999999998224, 14.46891108675448123, -93.32139747004409003 ) ) ;
#4012=CARTESIAN_POINT ( 'NONE',  ( -3.500000000000002220, 15.47927405783632437, -54.87764746908817415 ) ) ;
#4014=CARTESIAN_POINT ( 'NONE',  ( -3.500000000000001332, 17.50000000000002487, -134.6547308033774186 ) ) ;
#4015=ORIENTED_EDGE ( 'NONE', *, *, #34112, .T. ) ;
#4017=CARTESIAN_POINT ( 'NONE',  ( -3.500000000000002220, 15.47927405783632260, -42.57139747004410424 ) ) ;
#4018=CARTESIAN_POINT ( 'NONE',  ( -3.500000000000000000, 19.52072594216371826, -132.0443141357548598 ) ) ;
#4019=CARTESIAN_POINT ( 'NONE',  ( -3.310556943750000425, 19.41135094264166128, -24.93493913623280633 ) ) ;
#4020=CARTESIAN_POINT ( 'NONE',  ( 0.000000000000000000, 17.50000000000002487, -149.5231586289125687 ) ) ;
#4021=CARTESIAN_POINT ( 'NONE',  ( -1.394453263437886604E-15, 14.00000000000001776, -90.40473080337741862 ) ) ;
#4023=CARTESIAN_POINT ( 'NONE',  ( 4.648177544792955347E-16, 21.00000000000002132, -107.2109808024215027 ) ) ;
#4025=CARTESIAN_POINT ( 'NONE',  ( 1.655278471874998436, 14.63297358603754361, -76.43077246956615056 ) ) ;
#4026=DIRECTION ( 'NONE',  ( -0.000000000000000000, 1.259100132267607459E-16, -1.000000000000000000 ) ) ;
#4027=ORIENTED_EDGE ( 'NONE', *, *, #6716, .T. ) ;
#4029=CARTESIAN_POINT ( 'NONE',  ( 4.648177544792955347E-16, 21.00000000000001421, -54.90473080337742573 ) ) ;
#4032=CARTESIAN_POINT ( 'NONE',  ( 4.648177544792955347E-16, 21.00000000000002132, -127.2109808024214885 ) ) ;
#4033=CARTESIAN_POINT ( 'NONE',  ( -7.022189441860112050E-16, 13.67729811471672363, -87.51410580289947916 ) ) ;
#4034=VERTEX_POINT ( 'NONE', #6362 ) ;
#4037=( BOUNDED_CURVE ( )  B_SPLINE_CURVE ( 2, ( #278, #23035, #41782, #41993, #9878, #38576, #3680, #22204, #29409 ),
 .UNSPECIFIED., .F., .F. ) 
 B_SPLINE_CURVE_WITH_KNOTS ( ( 3, 2, 2, 2, 3 ),
 ( 0.006250000000000000347, 0.006944444444444444059, 0.008333333333333333218, 0.009722222222222222376, 0.01041666666666666782 ),
 .UNSPECIFIED. ) 
 CURVE ( )  GEOMETRIC_REPRESENTATION_ITEM ( )  RATIONAL_B_SPLINE_CURVE ( ( 0.9330127018922194093, 0.9330127018922194093, 1.000000000000000000, 0.8660254037844387076, 1.000000000000000000, 0.8660254037844387076, 1.000000000000000000, 0.9330127018922191873, 0.9330127018922192983 ) ) 
 REPRESENTATION_ITEM ( '' )  );
#4040=AXIS2_PLACEMENT_3D ( 'NONE', #27898, #8751, #11726 ) ;
#4041=ADVANCED_FACE ( 'NONE', ( #3178 ), #29106, .T. ) ;
#4042=CARTESIAN_POINT ( 'NONE',  ( -1.655278471874999990, 20.36702641396249547, -124.9307724695661364 ) ) ;
#4044=CARTESIAN_POINT ( 'NONE',  ( 3.310556943750001313, 17.50000000000001421, -52.35160580289946353 ) ) ;
#4045=CARTESIAN_POINT ( 'NONE',  ( 3.310556943750001313, 17.50000000000002132, -114.3516058028994706 ) ) ;
#4046=ORIENTED_EDGE ( 'NONE', *, *, #28793, .T. ) ;
#4047=EDGE_LOOP ( 'NONE', ( #34121, #34379, #41451, #28630 ) ) ;
#4048=CARTESIAN_POINT ( 'NONE',  ( -3.500000000000002220, 15.47927405783633503, -125.5713974700440758 ) ) ;
#4049=CARTESIAN_POINT ( 'NONE',  ( 3.310556943749999981, 15.58864905735836182, -40.34743913623281486 ) ) ;
#4050=CARTESIAN_POINT ( 'NONE',  ( -3.310556943750001313, 17.50000000000001421, -73.85160580289947063 ) ) ;
#4051=CARTESIAN_POINT ( 'NONE',  ( 3.500000000000001332, 17.50000000000002132, -120.4609808024215170 ) ) ;
#4052=CARTESIAN_POINT ( 'NONE',  ( -7.022189441860112050E-16, 13.67729811471672541, -101.5141058028994792 ) ) ;
#4053=CARTESIAN_POINT ( 'NONE',  ( 0.000000000000000000, 17.50000000000002487, -149.5231586289125687 ) ) ;
#4054=DIRECTION ( 'NONE',  ( -0.000000000000000000, 1.259100132267607459E-16, -1.000000000000000000 ) ) ;
#4056=CARTESIAN_POINT ( 'NONE',  ( 3.500000000000000000, 15.47927405783632260, -67.54431413575484555 ) ) ;
#4058=DIRECTION ( 'NONE',  ( -0.000000000000000000, 1.259100132267607459E-16, -1.000000000000000000 ) ) ;
#4059=CARTESIAN_POINT ( 'NONE',  ( -1.655278471874999990, 20.36702641396248481, -39.93077246956613635 ) ) ;
#4060=CARTESIAN_POINT ( 'NONE',  ( -3.310556943750002645, 15.58864905735837247, -93.76827246956612782 ) ) ;
#4061=CARTESIAN_POINT ( 'NONE',  ( -3.500000000000000888, 19.52072594216370760, -58.73806413671076143 ) ) ;
#4062=CARTESIAN_POINT ( 'NONE',  ( 1.655278471875001101, 20.36702641396249547, -113.1849391362327992 ) ) ;
#4063=CARTESIAN_POINT ( 'NONE',  ( 3.310556943750001313, 19.41135094264166128, -43.26827246956613493 ) ) ;
#4065=CARTESIAN_POINT ( 'NONE',  ( 0.9378221735089281585, 14.00000000000002309, -127.6663226036829855 ) ) ;
#4069=CYLINDRICAL_SURFACE ( 'NONE', #6818, 3.499999999999999556 ) ;
#4070=CARTESIAN_POINT ( 'NONE',  ( 1.655278471874998436, 14.63297358603754539, -90.43077246956613635 ) ) ;
#4071=CARTESIAN_POINT ( 'NONE',  ( 1.750000000000001110, 20.53108891324554719, -38.98806413671076854 ) ) ;
#4078=CARTESIAN_POINT ( 'NONE',  ( 3.500000000000001332, 19.52072594216370405, -45.07139747004409713 ) ) ;
#4079=ORIENTED_EDGE ( 'NONE', *, *, #5726, .T. ) ;
#4080=EDGE_CURVE ( 'NONE', #22966, #5825, #27774, .T. ) ;
#4083=CARTESIAN_POINT ( 'NONE',  ( -7.022189441860112050E-16, 13.67729811471671653, -30.51410580289946495 ) ) ;
#4084=ORIENTED_EDGE ( 'NONE', *, *, #18356, .F. ) ;
#4091=CARTESIAN_POINT ( 'NONE',  ( -1.394453263437886604E-15, 14.00000000000001421, -63.40473080337742573 ) ) ;
#4092=EDGE_CURVE ( 'NONE', #34018, #26292, #15320, .T. ) ;
#4096=CARTESIAN_POINT ( 'NONE',  ( 1.655278471875001101, 20.36702641396249902, -138.1849391362327992 ) ) ;
#4097=CARTESIAN_POINT ( 'NONE',  ( 2.474675557024783212E-16, 21.54145188432739033, -29.21098080242151696 ) ) ;
#4100=CARTESIAN_POINT ( 'NONE',  ( -3.500000000000002220, 15.47927405783633503, -140.5713974700441042 ) ) ;
#4101=CARTESIAN_POINT ( 'NONE',  ( 3.500000000000001332, 19.52072594216370405, -43.07139747004409713 ) ) ;
#4103=CARTESIAN_POINT ( 'NONE',  ( -7.424026671074350129E-16, 13.45854811567264164, -132.7109808024214885 ) ) ;
#4104=CARTESIAN_POINT ( 'NONE',  ( 2.340729813953370519E-16, 21.32270188528331900, -120.0141058028994792 ) ) ;
#4106=( BOUNDED_CURVE ( )  B_SPLINE_CURVE ( 2, ( #11920, #21298, #41279, #8939, #31279, #21911, #18733, #8318, #31695 ),
 .UNSPECIFIED., .F., .T. ) 
 B_SPLINE_CURVE_WITH_KNOTS ( ( 3, 2, 2, 2, 3 ),
 ( 0.5729166666666666297, 0.5736111111111110716, 0.5749999999999999556, 0.5763888888888888395, 0.5770833333333332815 ),
 .UNSPECIFIED. ) 
 CURVE ( )  GEOMETRIC_REPRESENTATION_ITEM ( )  RATIONAL_B_SPLINE_CURVE ( ( 0.9330127018922194093, 0.9330127018922194093, 1.000000000000000000, 0.8660254037844387076, 1.000000000000000000, 0.8660254037844387076, 1.000000000000000000, 0.9330127018922194093, 0.9330127018922194093 ) ) 
 REPRESENTATION_ITEM ( '' )  );
#4107=FACE_OUTER_BOUND ( 'NONE', #24822, .T. ) ;
#4108=CARTESIAN_POINT ( 'NONE',  ( -3.500000000000000888, 19.52072594216371115, -84.04431413575483134 ) ) ;
#4110=CARTESIAN_POINT ( 'NONE',  ( 3.310556943749999981, 15.58864905735836537, -54.34743913623282907 ) ) ;
#4111=CARTESIAN_POINT ( 'NONE',  ( 3.310556943749999981, 15.58864905735837247, -111.4349391362327850 ) ) ;
#4112=CARTESIAN_POINT ( 'NONE',  ( 4.648177544792955347E-16, 21.00000000000001776, -94.21098080242150274 ) ) ;
#4113=CARTESIAN_POINT ( 'NONE',  ( 1.750000000000001110, 20.53108891324554719, -28.98806413671076143 ) ) ;
#4114=CARTESIAN_POINT ( 'NONE',  ( 0.000000000000000000, 21.00000000000002487, -149.5231586289125687 ) ) ;
#4116=CARTESIAN_POINT ( 'NONE',  ( -1.655278471875002211, 14.63297358603755249, -126.6849391362327992 ) ) ;
#4119=CARTESIAN_POINT ( 'NONE',  ( -7.460324959392693302E-14, 21.00000000000001776, -85.90473080337741862 ) ) ;
#4120=CARTESIAN_POINT ( 'NONE',  ( -3.310556943750000425, 19.41135094264166128, -63.93493913623280633 ) ) ;
#4124=CARTESIAN_POINT ( 'NONE',  ( 1.655278471874998436, 14.63297358603754361, -78.51827246956614204 ) ) ;
#4125=CARTESIAN_POINT ( 'NONE',  ( 3.500000000000000000, 15.47927405783632082, -26.23806413671075433 ) ) ;
#4130=CARTESIAN_POINT ( 'NONE',  ( -1.655278471874999990, 20.36702641396248481, -42.93077246956614346 ) ) ;
#4132=CARTESIAN_POINT ( 'NONE',  ( -3.310556943750002645, 15.58864905735837425, -101.6807724695661364 ) ) ;
#4133=CARTESIAN_POINT ( 'NONE',  ( 0.9378221735089281585, 14.00000000000001066, -42.36007260463891555 ) ) ;
#4134=VECTOR ( 'NONE', #26916, 1000.000000000000000 ) ;
#4139=EDGE_CURVE ( 'NONE', #38180, #16644, #35913, .T. ) ;
#4140=CARTESIAN_POINT ( 'NONE',  ( -3.310556943750001313, 17.50000000000001421, -54.76410580289947916 ) ) ;
#4141=VERTEX_POINT ( 'NONE', #13373 ) ;
#4142=ORIENTED_EDGE ( 'NONE', *, *, #5077, .F. ) ;
#4143=CARTESIAN_POINT ( 'NONE',  ( 0.9378221735089300459, 21.00000000000001776, -93.25563900116002003 ) ) ;
#4144=CARTESIAN_POINT ( 'NONE',  ( 1.749999999999998224, 14.46891108675448656, -125.3213974700440900 ) ) ;
#4149=CARTESIAN_POINT ( 'NONE',  ( 3.500000000000001332, 17.50000000000001066, -45.46098080242151696 ) ) ;
#4150=CARTESIAN_POINT ( 'NONE',  ( 3.500000000000001332, 19.52072594216371826, -108.3776474690881599 ) ) ;
#4151=CARTESIAN_POINT ( 'NONE',  ( 1.750000000000001110, 20.53108891324555429, -96.98806413671076143 ) ) ;
#4153=DIRECTION ( 'NONE',  ( -0.000000000000000000, 1.259100132267607459E-16, -1.000000000000000000 ) ) ;
#4155=CARTESIAN_POINT ( 'NONE',  ( 3.310556943750001313, 17.50000000000001066, -27.35160580289947063 ) ) ;
#4156=CARTESIAN_POINT ( 'NONE',  ( -1.655278471874999990, 20.36702641396248481, -24.01827246956612782 ) ) ;
#4157=CARTESIAN_POINT ( 'NONE',  ( 2.340729813953370519E-16, 21.32270188528331190, -83.10160580289947063 ) ) ;
#4158=CARTESIAN_POINT ( 'NONE',  ( 2.340729813953370519E-16, 21.32270188528332255, -133.0141058028994792 ) ) ;
#4162=( BOUNDED_CURVE ( )  B_SPLINE_CURVE ( 2, ( #1063, #27833, #5076, #37209, #10633, #8064, #36789, #23611, #14038 ),
 .UNSPECIFIED., .F., .T. ) 
 B_SPLINE_CURVE_WITH_KNOTS ( ( 3, 2, 2, 2, 3 ),
 ( 0.07708333333333333703, 0.07777777777777777901, 0.07916666666666666297, 0.08055555555555556080, 0.08125000000000000278 ),
 .UNSPECIFIED. ) 
 CURVE ( )  GEOMETRIC_REPRESENTATION_ITEM ( )  RATIONAL_B_SPLINE_CURVE ( ( 0.9330127018922194093, 0.9330127018922194093, 1.000000000000000000, 0.8660254037844387076, 1.000000000000000000, 0.8660254037844387076, 1.000000000000000000, 0.9330127018922194093, 0.9330127018922194093 ) ) 
 REPRESENTATION_ITEM ( '' )  );
#4164=CARTESIAN_POINT ( 'NONE',  ( -3.310556943750000425, 19.41135094264166838, -125.9349391362327992 ) ) ;
#4166=CARTESIAN_POINT ( 'NONE',  ( 3.310556943750001313, 19.41135094264166483, -87.18077246956613635 ) ) ;
#4167=LINE ( 'NONE', #26513, #19243 ) ;
#4168=CARTESIAN_POINT ( 'NONE',  ( 1.749999999999998224, 14.46891108675447946, -75.62764746908817415 ) ) ;
#4169=CARTESIAN_POINT ( 'NONE',  ( -7.022189441860112050E-16, 13.67729811471673074, -142.6016058028994564 ) ) ;
#4170=CARTESIAN_POINT ( 'NONE',  ( -3.500000000000001332, 17.50000000000001776, -76.65473080337741862 ) ) ;
#4171=CARTESIAN_POINT ( 'NONE',  ( 1.655278471875001101, 20.36702641396248836, -53.18493913623280633 ) ) ;
#4174=CARTESIAN_POINT ( 'NONE',  ( -1.750000000000002220, 14.46891108675448478, -98.79431413575484555 ) ) ;
#4176=CARTESIAN_POINT ( 'NONE',  ( -1.655278471874999990, 20.36702641396249192, -81.01827246956614204 ) ) ;
#4177=CARTESIAN_POINT ( 'NONE',  ( -3.310556943750001313, 17.50000000000002487, -139.8516058028994564 ) ) ;
#4180=CARTESIAN_POINT ( 'NONE',  ( -7.022189441860112050E-16, 13.67729811471672896, -109.5141058028994649 ) ) ;
#4181=CARTESIAN_POINT ( 'NONE',  ( 3.310556943750001313, 17.50000000000001421, -73.26410580289947916 ) ) ;
#4184=CARTESIAN_POINT ( 'NONE',  ( 2.340729813953370519E-16, 21.32270188528331900, -102.1016058028994564 ) ) ;
#4185=CARTESIAN_POINT ( 'NONE',  ( 1.749999999999998224, 14.46891108675448301, -101.3213974700440900 ) ) ;
#4188=CARTESIAN_POINT ( 'NONE',  ( 0.9378221735089300459, 21.00000000000001066, -43.94938900211594301 ) ) ;
#4189=CARTESIAN_POINT ( 'NONE',  ( 1.749999999999998224, 14.46891108675447768, -58.32139747004409713 ) ) ;
#4191=CARTESIAN_POINT ( 'NONE',  ( -7.022189441860112050E-16, 13.67729811471672186, -60.51410580289945784 ) ) ;
#4193=CARTESIAN_POINT ( 'NONE',  ( 1.655278471874998436, 14.63297358603754894, -115.4307724695661364 ) ) ;
#4194=CARTESIAN_POINT ( 'NONE',  ( -0.9378221735089291577, 21.00000000000002132, -118.1663226036829997 ) ) ;
#4196=ORIENTED_EDGE ( 'NONE', *, *, #14263, .T. ) ;
#4202=CARTESIAN_POINT ( 'NONE',  ( -3.310556943750000425, 19.41135094264166128, -70.84743913623279354 ) ) ;
#4203=VERTEX_POINT ( 'NONE', #9983 ) ;
#4204=EDGE_LOOP ( 'NONE', ( #18313, #3307, #32089, #32756 ) ) ;
#4207=FACE_OUTER_BOUND ( 'NONE', #32755, .T. ) ;
#4210=VERTEX_POINT ( 'NONE', #6993 ) ;
#4211=CARTESIAN_POINT ( 'NONE',  ( -3.310556943750002201, 15.58864905735837780, -134.6807724695661364 ) ) ;
#4212=CARTESIAN_POINT ( 'NONE',  ( -0.9378221735089310451, 14.00000000000001599, -74.44938900211596433 ) ) ;
#4213=CARTESIAN_POINT ( 'NONE',  ( 1.655278471875001101, 20.36702641396248481, -43.18493913623279212 ) ) ;
#4214=CARTESIAN_POINT ( 'NONE',  ( -1.749999999999999778, 20.53108891324555785, -111.1276474690881741 ) ) ;
#4215=CARTESIAN_POINT ( 'NONE',  ( 2.340729813953370519E-16, 21.32270188528330479, -38.10160580289946353 ) ) ;
#4216=CARTESIAN_POINT ( 'NONE',  ( 2.340729813953370519E-16, 21.32270188528331190, -101.1016058028994706 ) ) ;
#4219=CARTESIAN_POINT ( 'NONE',  ( 3.310556943750001313, 17.50000000000002487, -143.3516058028994564 ) ) ;
#4220=DIRECTION ( 'NONE',  ( -0.000000000000000000, 1.259100132267607459E-16, -1.000000000000000000 ) ) ;
#4221=CARTESIAN_POINT ( 'NONE',  ( -3.500000000000002220, 15.47927405783632970, -101.8776474690881741 ) ) ;
#4223=CARTESIAN_POINT ( 'NONE',  ( -1.394453263437886604E-15, 14.00000000000002132, -126.4047308033774186 ) ) ;
#4224=CARTESIAN_POINT ( 'NONE',  ( -1.750000000000002220, 14.46891108675448301, -93.48806413671076143 ) ) ;
#4229=DIRECTION ( 'NONE',  ( 0.000000000000000000, 1.000000000000000000, 0.000000000000000000 ) ) ;
#4230=CARTESIAN_POINT ( 'NONE',  ( -3.500000000000001332, 17.50000000000001421, -53.96098080242150985 ) ) ;
#4231=CARTESIAN_POINT ( 'NONE',  ( -3.500000000000002220, 15.47927405783632793, -73.87764746908817415 ) ) ;
#4233=CARTESIAN_POINT ( 'NONE',  ( -1.394453263437886604E-15, 14.00000000000001066, -34.71098080242151696 ) ) ;
#4235=EDGE_LOOP ( 'NONE', ( #419, #3404, #38925, #29433 ) ) ;
#4236=CARTESIAN_POINT ( 'NONE',  ( 1.749999999999998224, 14.46891108675447590, -42.32139747004409713 ) ) ;
#4237=LINE ( 'NONE', #7641, #28043 ) ;
#4238=CARTESIAN_POINT ( 'NONE',  ( -3.310556943750000425, 19.41135094264166128, -25.93493913623279212 ) ) ;
#4239=CARTESIAN_POINT ( 'NONE',  ( -1.749999999999999778, 20.53108891324555429, -80.82139747004410424 ) ) ;
#4241=CARTESIAN_POINT ( 'NONE',  ( 4.648177544792955347E-16, 21.00000000000001066, -33.90473080337743284 ) ) ;
#4243=CARTESIAN_POINT ( 'NONE',  ( 1.655278471874998436, 14.63297358603754361, -74.43077246956613635 ) ) ;
#4246=CARTESIAN_POINT ( 'NONE',  ( 4.286263797015737581E-16, 14.00000000000002487, -149.5231586289125687 ) ) ;
#4248=ORIENTED_EDGE ( 'NONE', *, *, #33469, .T. ) ;
#4251=CARTESIAN_POINT ( 'NONE',  ( 1.655278471875001101, 20.36702641396249192, -82.09743913623279354 ) ) ;
#4253=ORIENTED_EDGE ( 'NONE', *, *, #10625, .T. ) ;
#4256=CARTESIAN_POINT ( 'NONE',  ( 4.648177544792955347E-16, 21.00000000000002132, -115.2109808024215027 ) ) ;
#4258=CARTESIAN_POINT ( 'NONE',  ( -3.310556943750000425, 19.41135094264166838, -126.8474391362328078 ) ) ;
#4260=CARTESIAN_POINT ( 'NONE',  ( -3.310556943750001313, 17.50000000000001421, -55.85160580289947063 ) ) ;
#4261=CARTESIAN_POINT ( 'NONE',  ( -3.310556943750001313, 17.50000000000002132, -116.8516058028994706 ) ) ;
#4264=CARTESIAN_POINT ( 'NONE',  ( -7.424026671074350129E-16, 13.45854811567264164, -125.4047308033774328 ) ) ;
#4265=CARTESIAN_POINT ( 'NONE',  ( -1.655278471874999990, 20.36702641396248481, -38.93077246956613635 ) ) ;
#4266=CARTESIAN_POINT ( 'NONE',  ( 2.340729813953370519E-16, 21.32270188528330834, -68.10160580289945642 ) ) ;
#4267=CARTESIAN_POINT ( 'NONE',  ( 3.500000000000000000, 15.47927405783632970, -118.5443141357548313 ) ) ;
#4268=CARTESIAN_POINT ( 'NONE',  ( -1.655278471875002211, 14.63297358603754894, -104.5974391362328078 ) ) ;
#4271=FACE_OUTER_BOUND ( 'NONE', #23116, .T. ) ;
#4272=DIRECTION ( 'NONE',  ( -0.000000000000000000, 1.259100132267607459E-16, -1.000000000000000000 ) ) ;
#4273=VECTOR ( 'NONE', #28051, 1000.000000000000000 ) ;
#4275=CARTESIAN_POINT ( 'NONE',  ( -1.749999999999999778, 20.53108891324555074, -68.12764746908817415 ) ) ;
#4276=FACE_OUTER_BOUND ( 'NONE', #13870, .T. ) ;
#4277=CARTESIAN_POINT ( 'NONE',  ( 2.340729813953370519E-16, 21.32270188528330479, -35.01410580289947205 ) ) ;
#4278=CARTESIAN_POINT ( 'NONE',  ( -1.655278471874999990, 20.36702641396249192, -91.01827246956612782 ) ) ;
#4279=CARTESIAN_POINT ( 'NONE',  ( 3.500000000000001332, 17.50000000000001421, -61.15473080337742573 ) ) ;
#4281=CARTESIAN_POINT ( 'NONE',  ( 1.655278471874998436, 14.63297358603754894, -111.5182724695661420 ) ) ;
#4282=CARTESIAN_POINT ( 'NONE',  ( 1.655278471874998436, 14.63297358603754006, -45.51827246956613493 ) ) ;
#4288=CARTESIAN_POINT ( 'NONE',  ( 3.500000000000001332, 17.50000000000001421, -61.46098080242150274 ) ) ;
#4289=EDGE_CURVE ( 'NONE', #32893, #39031, #24550, .T. ) ;
#4290=CARTESIAN_POINT ( 'NONE',  ( -1.655278471875002211, 14.63297358603754894, -95.59743913623280775 ) ) ;
#4291=CARTESIAN_POINT ( 'NONE',  ( -1.750000000000002220, 14.46891108675447590, -36.48806413671076854 ) ) ;
#4296=( BOUNDED_CURVE ( )  B_SPLINE_CURVE ( 2, ( #27049, #26410, #36831, #39157, #33419, #16839, #7692, #33644, #33201 ),
 .UNSPECIFIED., .F., .T. ) 
 B_SPLINE_CURVE_WITH_KNOTS ( ( 3, 2, 2, 2, 3 ),
 ( 0.6687499999999999556, 0.6694444444444443976, 0.6708333333333332815, 0.6722222222222222765, 0.6729166666666667185 ),
 .UNSPECIFIED. ) 
 CURVE ( )  GEOMETRIC_REPRESENTATION_ITEM ( )  RATIONAL_B_SPLINE_CURVE ( ( 0.9330127018922194093, 0.9330127018922194093, 1.000000000000000000, 0.8660254037844387076, 1.000000000000000000, 0.8660254037844387076, 1.000000000000000000, 0.9330127018922194093, 0.9330127018922194093 ) ) 
 REPRESENTATION_ITEM ( '' )  );
#4297=VERTEX_POINT ( 'NONE', #16370 ) ;
#4300=CARTESIAN_POINT ( 'NONE',  ( -1.655278471875002211, 14.63297358603754006, -27.59743913623280420 ) ) ;
#4301=ORIENTED_EDGE ( 'NONE', *, *, #27257, .T. ) ;
#4307=VECTOR ( 'NONE', #28662, 1000.000000000000000 ) ;
#4309=CARTESIAN_POINT ( 'NONE',  ( -1.394453263437886604E-15, 14.00000000000001066, -45.71098080242150274 ) ) ;
#4312=CARTESIAN_POINT ( 'NONE',  ( 3.310556943750001313, 19.41135094264167549, -142.1807724695661364 ) ) ;
#4314=CARTESIAN_POINT ( 'NONE',  ( -0.9378221735089291577, 21.00000000000001776, -75.16632260368299967 ) ) ;
#4315=CARTESIAN_POINT ( 'NONE',  ( -3.310556943750002645, 15.58864905735837780, -132.7682724695661136 ) ) ;
#4316=CARTESIAN_POINT ( 'NONE',  ( 3.500000000000000000, 15.47927405783632082, -28.54431413575483845 ) ) ;
#4318=CARTESIAN_POINT ( 'NONE',  ( 3.500000000000001776, 19.52072594216372181, -143.0713974700441042 ) ) ;
#4321=CARTESIAN_POINT ( 'NONE',  ( 1.749999999999998224, 14.46891108675448656, -134.6276474690881741 ) ) ;
#4322=CARTESIAN_POINT ( 'NONE',  ( 2.340729813953370519E-16, 21.32270188528331900, -116.0141058028994649 ) ) ;
#4325=CARTESIAN_POINT ( 'NONE',  ( -3.500000000000001332, 17.50000000000001776, -83.96098080242150274 ) ) ;
#4327=CARTESIAN_POINT ( 'NONE',  ( -7.022189441860112050E-16, 13.67729811471671830, -54.51410580289947205 ) ) ;
#4328=CARTESIAN_POINT ( 'NONE',  ( -3.310556943750002645, 15.58864905735837780, -113.7682724695661278 ) ) ;
#4330=CARTESIAN_POINT ( 'NONE',  ( 3.602337597214540226E-14, 14.00000000000002132, -116.7109808024215170 ) ) ;
#4332=CARTESIAN_POINT ( 'NONE',  ( 1.655278471875001101, 20.36702641396249902, -131.1849391362327992 ) ) ;
#4335=CARTESIAN_POINT ( 'NONE',  ( -3.695301148110399846E-14, 21.00000000000002132, -123.9047308033774044 ) ) ;
#4338=CARTESIAN_POINT ( 'NONE',  ( -3.310556943750000425, 19.41135094264166128, -64.93493913623279923 ) ) ;
#4341=CARTESIAN_POINT ( 'NONE',  ( 3.310556943749999981, 15.58864905735836714, -80.43493913623281344 ) ) ;
#4342=ADVANCED_FACE ( 'NONE', ( #30095 ), #39672, .T. ) ;
#4347=FACE_OUTER_BOUND ( 'NONE', #23779, .T. ) ;
#4349=CARTESIAN_POINT ( 'NONE',  ( -7.022189441860112050E-16, 13.67729811471671830, -46.51410580289947205 ) ) ;
#4350=CARTESIAN_POINT ( 'NONE',  ( -3.310556943750002645, 15.58864905735837425, -100.6807724695661364 ) ) ;
#4351=CARTESIAN_POINT ( 'NONE',  ( -0.9378221735089291577, 21.00000000000001776, -93.86007260463891555 ) ) ;
#4356=CARTESIAN_POINT ( 'NONE',  ( -3.310556943750001313, 17.50000000000001421, -52.76410580289947205 ) ) ;
#4357=ORIENTED_EDGE ( 'NONE', *, *, #18698, .T. ) ;
#4360=CARTESIAN_POINT ( 'NONE',  ( 0.9378221735089630196, 14.00000000000003553, -93.66632260368298546 ) ) ;
#4364=EDGE_LOOP ( 'NONE', ( #10423, #13027, #12894, #21986 ) ) ;
#4366=CARTESIAN_POINT ( 'NONE',  ( 3.500000000000001332, 17.50000000000001066, -42.46098080242151696 ) ) ;
#4367=( BOUNDED_CURVE ( )  B_SPLINE_CURVE ( 2, ( #2553, #9144, #7644, #20618, #13813, #20407, #33371, #29756, #23391 ),
 .UNSPECIFIED., .F., .T. ) 
 B_SPLINE_CURVE_WITH_KNOTS ( ( 3, 2, 2, 2, 3 ),
 ( 0.7187500000000000000, 0.7194444444444444420, 0.7208333333333333259, 0.7222222222222222099, 0.7229166666666666519 ),
 .UNSPECIFIED. ) 
 CURVE ( )  GEOMETRIC_REPRESENTATION_ITEM ( )  RATIONAL_B_SPLINE_CURVE ( ( 0.9330127018922194093, 0.9330127018922194093, 1.000000000000000000, 0.8660254037844387076, 1.000000000000000000, 0.8660254037844387076, 1.000000000000000000, 0.9330127018922194093, 0.9330127018922194093 ) ) 
 REPRESENTATION_ITEM ( '' )  );
#4369=FACE_OUTER_BOUND ( 'NONE', #29872, .T. ) ;
#4371=VECTOR ( 'NONE', #30765, 1000.000000000000000 ) ;
#4373=CARTESIAN_POINT ( 'NONE',  ( -7.022189441860112050E-16, 13.67729811471671475, -27.60160580289947063 ) ) ;
#4375=CARTESIAN_POINT ( 'NONE',  ( -1.750000000000002220, 14.46891108675448478, -97.48806413671076143 ) ) ;
#4376=CARTESIAN_POINT ( 'NONE',  ( -3.310556943750002645, 15.58864905735837070, -80.76827246956612782 ) ) ;
#4377=CARTESIAN_POINT ( 'NONE',  ( -3.310556943750001313, 17.50000000000002487, -133.7641058028994507 ) ) ;
#4380=CARTESIAN_POINT ( 'NONE',  ( -3.500000000000002220, 15.47927405783632793, -75.57139747004410424 ) ) ;
#4382=CARTESIAN_POINT ( 'NONE',  ( 1.655278471874998436, 14.63297358603755072, -130.5182724695661136 ) ) ;
#4384=CARTESIAN_POINT ( 'NONE',  ( -1.655278471874999990, 20.36702641396249192, -87.93077246956613635 ) ) ;
#4385=DIRECTION ( 'NONE',  ( -0.000000000000000000, 1.259100132267607459E-16, -1.000000000000000000 ) ) ;
#4386=CARTESIAN_POINT ( 'NONE',  ( 0.000000000000000000, 17.50000000000002487, -149.5231586289125687 ) ) ;
#4387=CARTESIAN_POINT ( 'NONE',  ( 3.310556943750001313, 19.41135094264167549, -143.2682724695661420 ) ) ;
#4388=CARTESIAN_POINT ( 'NONE',  ( -1.749999999999999778, 20.53108891324555074, -69.82139747004409003 ) ) ;
#4389=EDGE_CURVE ( 'NONE', #14931, #16704, #1389, .T. ) ;
#4390=CARTESIAN_POINT ( 'NONE',  ( -7.022189441860112050E-16, 13.67729811471672186, -56.60160580289947063 ) ) ;
#4392=DIRECTION ( 'NONE',  ( 0.000000000000000000, 1.000000000000000000, 0.000000000000000000 ) ) ;
#4393=CARTESIAN_POINT ( 'NONE',  ( 4.648177544792955347E-16, 21.00000000000001421, -49.21098080242150274 ) ) ;
#4394=CARTESIAN_POINT ( 'NONE',  ( 2.340729813953370519E-16, 21.32270188528331190, -79.10160580289945642 ) ) ;
#4395=CARTESIAN_POINT ( 'NONE',  ( -1.655278471874999990, 20.36702641396249902, -142.0182724695661420 ) ) ;
#4397=CARTESIAN_POINT ( 'NONE',  ( -3.310556943750002201, 15.58864905735837780, -111.6807724695661506 ) ) ;
#4398=CARTESIAN_POINT ( 'NONE',  ( 3.310556943749999981, 15.58864905735836714, -77.34743913623279354 ) ) ;
#4400=CARTESIAN_POINT ( 'NONE',  ( 2.340729813953370519E-16, 21.32270188528331190, -99.10160580289948484 ) ) ;
#4401=CARTESIAN_POINT ( 'NONE',  ( -3.500000000000000888, 19.52072594216371115, -99.73806413671076143 ) ) ;
#4402=AXIS2_PLACEMENT_3D ( 'NONE', #33355, #3580, #13799 ) ;
#4404=CARTESIAN_POINT ( 'NONE',  ( -1.394453263437886604E-15, 14.00000000000001066, -48.40473080337742573 ) ) ;
#4405=CARTESIAN_POINT ( 'NONE',  ( 1.750000000000001110, 20.53108891324554719, -26.29431413575483845 ) ) ;
#4406=CARTESIAN_POINT ( 'NONE',  ( -1.394453263437886604E-15, 14.00000000000002132, -131.7109808024214885 ) ) ;
#4407=CARTESIAN_POINT ( 'NONE',  ( 1.655278471874998436, 14.63297358603754184, -62.43077246956614346 ) ) ;
#4408=CARTESIAN_POINT ( 'NONE',  ( -0.9378221735089465882, 21.00000000000001066, -125.1663226036829855 ) ) ;
#4409=CARTESIAN_POINT ( 'NONE',  ( 1.655278471874998436, 14.63297358603754894, -114.4307724695661364 ) ) ;
#4410=VECTOR ( 'NONE', #1242, 1000.000000000000000 ) ;
#4412=ORIENTED_EDGE ( 'NONE', *, *, #5156, .F. ) ;
#4414=AXIS2_PLACEMENT_3D ( 'NONE', #11994, #13254, #272 ) ;
#4418=CARTESIAN_POINT ( 'NONE',  ( 1.655278471874998436, 14.63297358603754184, -67.43077246956613635 ) ) ;
#4420=ORIENTED_EDGE ( 'NONE', *, *, #18858, .F. ) ;
#4421=CARTESIAN_POINT ( 'NONE',  ( -3.500000000000002220, 15.47927405783632970, -86.87764746908817415 ) ) ;
#4426=CARTESIAN_POINT ( 'NONE',  ( -3.310556943750000425, 19.41135094264167549, -134.8474391362328220 ) ) ;
#4428=( BOUNDED_CURVE ( )  B_SPLINE_CURVE ( 2, ( #26614, #14274, #39798, #10450, #10663, #13848, #30005, #23644, #4490 ),
 .UNSPECIFIED., .F., .T. ) 
 B_SPLINE_CURVE_WITH_KNOTS ( ( 3, 2, 2, 2, 3 ),
 ( 0.1729166666666666630, 0.1736111111111111049, 0.1749999999999999889, 0.1763888888888889006, 0.1770833333333333426 ),
 .UNSPECIFIED. ) 
 CURVE ( )  GEOMETRIC_REPRESENTATION_ITEM ( )  RATIONAL_B_SPLINE_CURVE ( ( 0.9330127018922194093, 0.9330127018922194093, 1.000000000000000000, 0.8660254037844387076, 1.000000000000000000, 0.8660254037844387076, 1.000000000000000000, 0.9330127018922194093, 0.9330127018922194093 ) ) 
 REPRESENTATION_ITEM ( '' )  );
#4430=CARTESIAN_POINT ( 'NONE',  ( -7.022189441860112050E-16, 13.67729811471671653, -44.60160580289947063 ) ) ;
#4432=CARTESIAN_POINT ( 'NONE',  ( -1.655278471874999990, 20.36702641396248481, -39.01827246956612782 ) ) ;
#4433=CARTESIAN_POINT ( 'NONE',  ( 1.655278471874998436, 14.63297358603754716, -100.5182724695661278 ) ) ;
#4436=CARTESIAN_POINT ( 'NONE',  ( 3.310556943749999981, 15.58864905735837780, -142.4349391362327708 ) ) ;
#4438=CYLINDRICAL_SURFACE ( 'NONE', #28442, 3.499999999999999556 ) ;
#4439=CARTESIAN_POINT ( 'NONE',  ( 1.750000000000001110, 20.53108891324555429, -94.29431413575484555 ) ) ;
#4440=CARTESIAN_POINT ( 'NONE',  ( 0.9378221735089300459, 21.00000000000002487, -132.2556390011600342 ) ) ;
#4441=CARTESIAN_POINT ( 'NONE',  ( 1.749999999999998224, 14.46891108675447768, -64.62764746908818836 ) ) ;
#4442=CARTESIAN_POINT ( 'NONE',  ( 2.474675557024783212E-16, 21.54145188432739744, -84.90473080337741862 ) ) ;
#4443=EDGE_CURVE ( 'NONE', #10652, #34168, #27338, .T. ) ;
#4444=CARTESIAN_POINT ( 'NONE',  ( -7.022189441860112050E-16, 13.67729811471672186, -67.60160580289947063 ) ) ;
#4448=CYLINDRICAL_SURFACE ( 'NONE', #6501, 3.499999999999999556 ) ;
#4449=CARTESIAN_POINT ( 'NONE',  ( -3.500000000000000888, 19.52072594216370760, -54.04431413575484555 ) ) ;
#4452=ORIENTED_EDGE ( 'NONE', *, *, #34938, .T. ) ;
#4453=CARTESIAN_POINT ( 'NONE',  ( -3.500000000000001332, 17.50000000000001066, -41.65473080337743284 ) ) ;
#4455=CARTESIAN_POINT ( 'NONE',  ( -1.655278471874999990, 20.36702641396248481, -24.01827246956612782 ) ) ;
#4456=CARTESIAN_POINT ( 'NONE',  ( -1.394453263437886604E-15, 14.00000000000001421, -76.40473080337740441 ) ) ;
#4457=CARTESIAN_POINT ( 'NONE',  ( -1.750000000000002220, 14.46891108675448301, -90.48806413671076143 ) ) ;
#4459=CARTESIAN_POINT ( 'NONE',  ( -1.394453263437886604E-15, 14.00000000000001421, -78.71098080242148853 ) ) ;
#4461=CARTESIAN_POINT ( 'NONE',  ( -7.022189441860112050E-16, 13.67729811471672186, -77.51410580289945074 ) ) ;
#4462=CARTESIAN_POINT ( 'NONE',  ( 0.9378221735089455890, 14.00000000000003197, -116.3600726046389155 ) ) ;
#4464=DIRECTION ( 'NONE',  ( 0.000000000000000000, 1.000000000000000000, 0.000000000000000000 ) ) ;
#4466=ORIENTED_EDGE ( 'NONE', *, *, #30308, .T. ) ;
#4467=CARTESIAN_POINT ( 'NONE',  ( -1.750000000000002220, 14.46891108675448656, -120.4880641367107614 ) ) ;
#4468=CARTESIAN_POINT ( 'NONE',  ( 3.310556943750001313, 17.50000000000001776, -86.26410580289947916 ) ) ;
#4469=ORIENTED_EDGE ( 'NONE', *, *, #2117, .T. ) ;
#4474=CYLINDRICAL_SURFACE ( 'NONE', #5645, 3.499999999999999556 ) ;
#4475=CARTESIAN_POINT ( 'NONE',  ( -3.310556943750001313, 17.50000000000002132, -126.7641058028994792 ) ) ;
#4476=CARTESIAN_POINT ( 'NONE',  ( -3.500000000000000000, 19.52072594216371115, -95.04431413575484555 ) ) ;
#4477=CARTESIAN_POINT ( 'NONE',  ( -7.022189441860112050E-16, 13.67729811471671653, -52.60160580289947063 ) ) ;
#4478=CARTESIAN_POINT ( 'NONE',  ( -1.655278471874999990, 20.36702641396249547, -117.0182724695661278 ) ) ;
#4480=CARTESIAN_POINT ( 'NONE',  ( 1.749999999999998224, 14.46891108675448656, -126.3213974700440900 ) ) ;
#4481=CARTESIAN_POINT ( 'NONE',  ( 1.655278471874998436, 14.63297358603754006, -42.43077246956614346 ) ) ;
#4482=CARTESIAN_POINT ( 'NONE',  ( -1.655278471874999990, 20.36702641396248836, -67.01827246956612782 ) ) ;
#4483=CARTESIAN_POINT ( 'NONE',  ( -1.750000000000002220, 14.46891108675448656, -119.7943141357548313 ) ) ;
#4484=CARTESIAN_POINT ( 'NONE',  ( 2.340729813953370519E-16, 21.32270188528331190, -96.01410580289946495 ) ) ;
#4486=CARTESIAN_POINT ( 'NONE',  ( 4.648177544792955347E-16, 21.00000000000001066, -27.90473080337742928 ) ) ;
#4489=CARTESIAN_POINT ( 'NONE',  ( -1.750000000000002220, 14.46891108675448123, -69.79431413575484555 ) ) ;
#4490=CARTESIAN_POINT ( 'NONE',  ( 4.648177544792955347E-16, 21.00000000000002132, -122.2109808024215170 ) ) ;
#4491=CARTESIAN_POINT ( 'NONE',  ( 1.655278471875001101, 20.36702641396248481, -31.09743913623280775 ) ) ;
#4492=CARTESIAN_POINT ( 'NONE',  ( 1.655278471875001101, 20.36702641396249192, -93.18493913623279923 ) ) ;
#4493=CARTESIAN_POINT ( 'NONE',  ( 1.750000000000001110, 20.53108891324555074, -56.98806413671076143 ) ) ;
#4494=DIRECTION ( 'NONE',  ( -0.000000000000000000, 1.259100132267607459E-16, -1.000000000000000000 ) ) ;
#4495=CARTESIAN_POINT ( 'NONE',  ( -3.310556943750001313, 17.50000000000002132, -110.8516058028994564 ) ) ;
#4496=CARTESIAN_POINT ( 'NONE',  ( -7.022189441860112050E-16, 13.67729811471671830, -42.60160580289946353 ) ) ;
#4503=CARTESIAN_POINT ( 'NONE',  ( -1.655278471875002211, 14.63297358603754716, -91.59743913623280775 ) ) ;
#4509=DIRECTION ( 'NONE',  ( -0.000000000000000000, 1.259100132267607459E-16, -1.000000000000000000 ) ) ;
#4514=CYLINDRICAL_SURFACE ( 'NONE', #15710, 3.499999999999999556 ) ;
#4518=VERTEX_POINT ( 'NONE', #40308 ) ;
#4519=CARTESIAN_POINT ( 'NONE',  ( -1.750000000000002220, 14.46891108675447590, -27.48806413671076143 ) ) ;
#4521=CARTESIAN_POINT ( 'NONE',  ( -3.310556943750000425, 19.41135094264167549, -140.8474391362327935 ) ) ;
#4523=CARTESIAN_POINT ( 'NONE',  ( 0.000000000000000000, 21.00000000000002487, -149.5231586289125687 ) ) ;
#4525=CARTESIAN_POINT ( 'NONE',  ( 1.655278471875001101, 20.36702641396249902, -130.1849391362327992 ) ) ;
#4526=CARTESIAN_POINT ( 'NONE',  ( -3.500000000000002220, 15.47927405783632082, -27.87764746908817770 ) ) ;
#4527=EDGE_CURVE ( 'NONE', #5302, #524, #32118, .T. ) ;
#4529=CARTESIAN_POINT ( 'NONE',  ( 2.474675557024783212E-16, 21.54145188432740810, -140.9047308033774186 ) ) ;
#4531=CARTESIAN_POINT ( 'NONE',  ( -3.500000000000001332, 17.50000000000002487, -134.9609808024214885 ) ) ;
#4532=CARTESIAN_POINT ( 'NONE',  ( 1.655278471874998436, 14.63297358603754894, -115.4307724695661364 ) ) ;
#4535=CARTESIAN_POINT ( 'NONE',  ( 2.474675557024783212E-16, 21.54145188432739744, -85.21098080242150274 ) ) ;
#4536=( BOUNDED_CURVE ( )  B_SPLINE_CURVE ( 2, ( #40662, #21725, #25138, #31507, #34909, #38103, #8335, #40873, #34284 ),
 .UNSPECIFIED., .F., .T. ) 
 B_SPLINE_CURVE_WITH_KNOTS ( ( 3, 2, 2, 2, 3 ),
 ( 0.08125000000000000278, 0.08194444444444444475, 0.08333333333333332871, 0.08472222222222222654, 0.08541666666666666852 ),
 .UNSPECIFIED. ) 
 CURVE ( )  GEOMETRIC_REPRESENTATION_ITEM ( )  RATIONAL_B_SPLINE_CURVE ( ( 0.9330127018922194093, 0.9330127018922194093, 1.000000000000000000, 0.8660254037844387076, 1.000000000000000000, 0.8660254037844387076, 1.000000000000000000, 0.9330127018922194093, 0.9330127018922194093 ) ) 
 REPRESENTATION_ITEM ( '' )  );
#4538=CARTESIAN_POINT ( 'NONE',  ( -7.022189441860112050E-16, 13.67729811471671653, -47.51410580289947205 ) ) ;
#4539=CARTESIAN_POINT ( 'NONE',  ( 3.310556943750001313, 17.50000000000002132, -107.3516058028994564 ) ) ;
#4540=( BOUNDED_CURVE ( )  B_SPLINE_CURVE ( 2, ( #22559, #29136, #14, #28520, #12994, #9814, #41511, #15774, #29346 ),
 .UNSPECIFIED., .F., .T. ) 
 B_SPLINE_CURVE_WITH_KNOTS ( ( 3, 2, 2, 2, 3 ),
 ( 0.1145833333333333426, 0.1152777777777777846, 0.1166666666666666685, 0.1180555555555555525, 0.1187500000000000083 ),
 .UNSPECIFIED. ) 
 CURVE ( )  GEOMETRIC_REPRESENTATION_ITEM ( )  RATIONAL_B_SPLINE_CURVE ( ( 0.9330127018922194093, 0.9330127018922200755, 1.000000000000000000, 0.8660254037844387076, 1.000000000000000000, 0.8660254037844387076, 1.000000000000000000, 0.9330127018922187432, 0.9330127018922194093 ) ) 
 REPRESENTATION_ITEM ( '' )  );
#4541=CARTESIAN_POINT ( 'NONE',  ( -1.394453263437886604E-15, 14.00000000000002132, -111.4047308033774186 ) ) ;
#4542=CARTESIAN_POINT ( 'NONE',  ( -7.460324959392693302E-14, 21.00000000000001776, -87.90473080337741862 ) ) ;
#4544=CARTESIAN_POINT ( 'NONE',  ( -3.310556943750001313, 17.50000000000002487, -129.8516058028994564 ) ) ;
#4547=LINE ( 'NONE', #17526, #23489 ) ;
#4549=CARTESIAN_POINT ( 'NONE',  ( -3.310556943750000425, 19.41135094264166128, -56.93493913623279212 ) ) ;
#4550=EDGE_CURVE ( 'NONE', #13090, #17014, #8759, .T. ) ;
#4551=VERTEX_POINT ( 'NONE', #36913 ) ;
#4552=CARTESIAN_POINT ( 'NONE',  ( -3.310556943750001313, 17.50000000000001776, -80.85160580289945642 ) ) ;
#4554=DIRECTION ( 'NONE',  ( -0.000000000000000000, 1.259100132267607459E-16, -1.000000000000000000 ) ) ;
#4559=CARTESIAN_POINT ( 'NONE',  ( -3.310556943750002201, 15.58864905735836537, -39.68077246956613635 ) ) ;
#4560=CARTESIAN_POINT ( 'NONE',  ( -3.310556943750000425, 19.41135094264166483, -101.8474391362328078 ) ) ;
#4563=ORIENTED_EDGE ( 'NONE', *, *, #16552, .F. ) ;
#4565=CARTESIAN_POINT ( 'NONE',  ( 2.340729813953370519E-16, 21.32270188528330834, -51.01410580289947205 ) ) ;
#4566=ORIENTED_EDGE ( 'NONE', *, *, #27344, .T. ) ;
#4567=VERTEX_POINT ( 'NONE', #20112 ) ;
#4568=CARTESIAN_POINT ( 'NONE',  ( 4.648177544792955347E-16, 21.00000000000001066, -43.90473080337743284 ) ) ;
#4569=CARTESIAN_POINT ( 'NONE',  ( 7.367361408496833051E-14, 14.00000000000001776, -95.71098080242150274 ) ) ;
#4571=DIRECTION ( 'NONE',  ( -0.000000000000000000, 1.259100132267607459E-16, -1.000000000000000000 ) ) ;
#4572=ORIENTED_EDGE ( 'NONE', *, *, #182, .T. ) ;
#4574=CARTESIAN_POINT ( 'NONE',  ( 1.749999999999998224, 14.46891108675447590, -42.62764746908817415 ) ) ;
#4578=EDGE_CURVE ( 'NONE', #21522, #22611, #35100, .T. ) ;
#4580=CARTESIAN_POINT ( 'NONE',  ( -1.655278471875002211, 14.63297358603754006, -29.68493913623279568 ) ) ;
#4581=CARTESIAN_POINT ( 'NONE',  ( 3.500000000000001332, 17.50000000000002132, -122.1547308033774328 ) ) ;
#4582=CARTESIAN_POINT ( 'NONE',  ( 3.310556943749999981, 15.58864905735836714, -80.43493913623281344 ) ) ;
#4583=CARTESIAN_POINT ( 'NONE',  ( 1.655278471875001101, 20.36702641396249902, -132.0974391362328220 ) ) ;
#4587=CARTESIAN_POINT ( 'NONE',  ( -1.750000000000002220, 14.46891108675448123, -75.48806413671076143 ) ) ;
#4588=CARTESIAN_POINT ( 'NONE',  ( -3.310556943750001313, 17.50000000000002132, -120.8516058028994706 ) ) ;
#4589=CARTESIAN_POINT ( 'NONE',  ( 0.000000000000000000, 17.50000000000002487, -149.5231586289125687 ) ) ;
#4590=CARTESIAN_POINT ( 'NONE',  ( -7.022189441860112050E-16, 13.67729811471672363, -84.51410580289947916 ) ) ;
#4592=CARTESIAN_POINT ( 'NONE',  ( -1.394453263437886604E-15, 14.00000000000001421, -65.40473080337743284 ) ) ;
#4593=CARTESIAN_POINT ( 'NONE',  ( 0.000000000000000000, 17.50000000000002487, -149.5231586289125687 ) ) ;
#4594=CARTESIAN_POINT ( 'NONE',  ( -3.500000000000002220, 15.47927405783632615, -72.57139747004409003 ) ) ;
#4595=CARTESIAN_POINT ( 'NONE',  ( -1.655278471874999990, 20.36702641396248836, -53.01827246956612782 ) ) ;
#4598=CARTESIAN_POINT ( 'NONE',  ( -3.500000000000000000, 19.52072594216371115, -99.04431413575484555 ) ) ;
#4599=CARTESIAN_POINT ( 'NONE',  ( -1.655278471875002211, 14.63297358603754539, -78.68493913623279923 ) ) ;
#4600=CARTESIAN_POINT ( 'NONE',  ( -1.655278471874999990, 20.36702641396249902, -141.0182724695661420 ) ) ;
#4602=CARTESIAN_POINT ( 'NONE',  ( 1.655278471875001101, 20.36702641396249547, -103.0974391362328220 ) ) ;
#4603=CARTESIAN_POINT ( 'NONE',  ( -3.310556943750002645, 15.58864905735837070, -74.68077246956613635 ) ) ;
#4604=FACE_OUTER_BOUND ( 'NONE', #30391, .T. ) ;
#4606=CARTESIAN_POINT ( 'NONE',  ( -3.310556943750000425, 19.41135094264166838, -98.93493913623279923 ) ) ;
#4608=CARTESIAN_POINT ( 'NONE',  ( -3.500000000000002220, 15.47927405783632970, -86.57139747004409003 ) ) ;
#4609=CARTESIAN_POINT ( 'NONE',  ( -1.394453263437886604E-15, 14.00000000000001776, -81.40473080337743284 ) ) ;
#4610=LINE ( 'NONE', #17589, #12361 ) ;
#4611=CARTESIAN_POINT ( 'NONE',  ( -3.310556943750001313, 17.50000000000001421, -60.76410580289946495 ) ) ;
#4613=CARTESIAN_POINT ( 'NONE',  ( 1.655278471875001101, 20.36702641396249547, -115.0974391362327935 ) ) ;
#4614=ADVANCED_FACE ( 'NONE', ( #24780 ), #11996, .T. ) ;
#4618=ADVANCED_FACE ( 'NONE', ( #8386 ), #11784, .T. ) ;
#4620=ORIENTED_EDGE ( 'NONE', *, *, #1194, .T. ) ;
#4622=CARTESIAN_POINT ( 'NONE',  ( -3.310556943750002645, 15.58864905735837070, -67.68077246956613635 ) ) ;
#4623=( BOUNDED_CURVE ( )  B_SPLINE_CURVE ( 2, ( #30305, #26701, #27335, #37125, #7978, #36910, #7772, #4778, #10537 ),
 .UNSPECIFIED., .F., .T. ) 
 B_SPLINE_CURVE_WITH_KNOTS ( ( 3, 2, 2, 2, 3 ),
 ( 0.2479166666666666741, 0.2486111111111111160, 0.2500000000000000000, 0.2513888888888888840, 0.2520833333333333259 ),
 .UNSPECIFIED. ) 
 CURVE ( )  GEOMETRIC_REPRESENTATION_ITEM ( )  RATIONAL_B_SPLINE_CURVE ( ( 0.9330127018922194093, 0.9330127018922194093, 1.000000000000000000, 0.8660254037844387076, 1.000000000000000000, 0.8660254037844387076, 1.000000000000000000, 0.9330127018922194093, 0.9330127018922194093 ) ) 
 REPRESENTATION_ITEM ( '' )  );
#4625=ORIENTED_EDGE ( 'NONE', *, *, #38722, .T. ) ;
#4631=ORIENTED_EDGE ( 'NONE', *, *, #12438, .T. ) ;
#4633=CARTESIAN_POINT ( 'NONE',  ( -7.022189441860112050E-16, 13.67729811471672896, -134.5141058028994507 ) ) ;
#4637=CARTESIAN_POINT ( 'NONE',  ( -3.310556943750001313, 17.50000000000001066, -42.85160580289947063 ) ) ;
#4639=CARTESIAN_POINT ( 'NONE',  ( 1.655278471874998436, 14.63297358603753828, -31.51827246956613493 ) ) ;
#4640=CARTESIAN_POINT ( 'NONE',  ( -3.310556943750002645, 15.58864905735837425, -98.76827246956612782 ) ) ;
#4642=CARTESIAN_POINT ( 'NONE',  ( -7.022189441860112050E-16, 13.67729811471672896, -141.6016058028994564 ) ) ;
#4643=FACE_OUTER_BOUND ( 'NONE', #11272, .T. ) ;
#4644=CARTESIAN_POINT ( 'NONE',  ( -7.424026671074350129E-16, 13.45854811567263809, -97.71098080242148853 ) ) ;
#4646=CARTESIAN_POINT ( 'NONE',  ( -3.500000000000002220, 15.47927405783632793, -88.57139747004410424 ) ) ;
#4647=CARTESIAN_POINT ( 'NONE',  ( -1.655278471874999990, 20.36702641396248836, -71.01827246956612782 ) ) ;
#4652=CARTESIAN_POINT ( 'NONE',  ( 2.474675557024783212E-16, 21.54145188432739388, -47.21098080242150274 ) ) ;
#4653=AXIS2_PLACEMENT_3D ( 'NONE', #29130, #19363, #16190 ) ;
#4654=CARTESIAN_POINT ( 'NONE',  ( 3.310556943750001313, 17.50000000000002132, -119.2641058028994792 ) ) ;
#4655=CARTESIAN_POINT ( 'NONE',  ( -3.500000000000000000, 19.52072594216371115, -79.73806413671076143 ) ) ;
#4658=CARTESIAN_POINT ( 'NONE',  ( -3.500000000000000888, 19.52072594216371826, -115.7380641367107614 ) ) ;
#4660=CARTESIAN_POINT ( 'NONE',  ( 4.286263797015755330E-16, 13.99999999999998401, 153.5815388724490163 ) ) ;
#4663=CARTESIAN_POINT ( 'NONE',  ( 1.655278471875001101, 20.36702641396249192, -76.09743913623280775 ) ) ;
#4665=FACE_OUTER_BOUND ( 'NONE', #166, .T. ) ;
#4666=CARTESIAN_POINT ( 'NONE',  ( 1.750000000000001110, 20.53108891324554719, -26.98806413671076143 ) ) ;
#4667=ORIENTED_EDGE ( 'NONE', *, *, #35828, .F. ) ;
#4668=EDGE_CURVE ( 'NONE', #29443, #15700, #11375, .T. ) ;
#4669=CARTESIAN_POINT ( 'NONE',  ( 3.500000000000000000, 15.47927405783632793, -88.54431413575483134 ) ) ;
#4670=CARTESIAN_POINT ( 'NONE',  ( 3.310556943750001313, 19.41135094264166483, -83.18077246956613635 ) ) ;
#4672=VERTEX_POINT ( 'NONE', #15198 ) ;
#4673=( BOUNDED_CURVE ( )  B_SPLINE_CURVE ( 2, ( #36875, #21121, #13684, #30272, #40269, #16882, #33244, #29845, #10923 ),
 .UNSPECIFIED., .F., .T. ) 
 B_SPLINE_CURVE_WITH_KNOTS ( ( 3, 2, 2, 2, 3 ),
 ( 0.6104166666666667185, 0.6111111111111111605, 0.6125000000000000444, 0.6138888888888889284, 0.6145833333333333703 ),
 .UNSPECIFIED. ) 
 CURVE ( )  GEOMETRIC_REPRESENTATION_ITEM ( )  RATIONAL_B_SPLINE_CURVE ( ( 0.9330127018922194093, 0.9330127018922194093, 1.000000000000000000, 0.8660254037844387076, 1.000000000000000000, 0.8660254037844387076, 1.000000000000000000, 0.9330127018922194093, 0.9330127018922194093 ) ) 
 REPRESENTATION_ITEM ( '' )  );
#4677=CARTESIAN_POINT ( 'NONE',  ( -0.9378221735089291577, 21.00000000000001421, -59.16632260368298546 ) ) ;
#4681=CARTESIAN_POINT ( 'NONE',  ( -7.022189441860112050E-16, 13.67729811471671653, -53.60160580289946353 ) ) ;
#4682=CARTESIAN_POINT ( 'NONE',  ( -1.655278471875002211, 14.63297358603755072, -116.6849391362327850 ) ) ;
#4684=CARTESIAN_POINT ( 'NONE',  ( 2.474675557024783212E-16, 21.54145188432740099, -122.9047308033774044 ) ) ;
#4685=CARTESIAN_POINT ( 'NONE',  ( -7.022189441860112050E-16, 13.67729811471671475, -39.51410580289947916 ) ) ;
#4686=CARTESIAN_POINT ( 'NONE',  ( 1.655278471875001101, 20.36702641396248836, -68.18493913623279923 ) ) ;
#4687=CARTESIAN_POINT ( 'NONE',  ( -1.749999999999999778, 20.53108891324555785, -114.1276474690881741 ) ) ;
#4689=CARTESIAN_POINT ( 'NONE',  ( 2.340729813953370519E-16, 21.32270188528331190, -99.01410580289946495 ) ) ;
#4690=CARTESIAN_POINT ( 'NONE',  ( 0.9378221735089281585, 14.00000000000001243, -60.36007260463890134 ) ) ;
#4694=CARTESIAN_POINT ( 'NONE',  ( 3.500000000000001776, 19.52072594216370760, -63.37764746908817415 ) ) ;
#4695=LINE ( 'NONE', #33411, #8784 ) ;
#4696=CARTESIAN_POINT ( 'NONE',  ( -7.022189441860112050E-16, 13.67729811471671475, -32.51410580289946495 ) ) ;
#4697=CARTESIAN_POINT ( 'NONE',  ( 3.310556943750001313, 19.41135094264166483, -89.26827246956612782 ) ) ;
#4698=CARTESIAN_POINT ( 'NONE',  ( -3.500000000000000888, 19.52072594216370760, -54.73806413671076854 ) ) ;
#4699=CARTESIAN_POINT ( 'NONE',  ( 0.000000000000000000, 21.00000000000002487, -149.5231586289125687 ) ) ;
#4700=CARTESIAN_POINT ( 'NONE',  ( -1.655278471874999990, 20.36702641396249547, -110.0182724695661420 ) ) ;
#4701=CARTESIAN_POINT ( 'NONE',  ( 3.310556943750001313, 19.41135094264166128, -36.26827246956612782 ) ) ;
#4707=FACE_OUTER_BOUND ( 'NONE', #27170, .T. ) ;
#4708=CARTESIAN_POINT ( 'NONE',  ( 2.340729813953370519E-16, 21.32270188528331190, -94.01410580289947916 ) ) ;
#4709=CARTESIAN_POINT ( 'NONE',  ( -1.836030130193217234E-14, 21.00000000000002132, -129.2109808024214601 ) ) ;
#4711=AXIS2_PLACEMENT_3D ( 'NONE', #6165, #15965, #28914 ) ;
#4712=ORIENTED_EDGE ( 'NONE', *, *, #41031, .T. ) ;
#4715=CARTESIAN_POINT ( 'NONE',  ( 4.286263797015737581E-16, 14.00000000000002487, -149.5231586289125687 ) ) ;
#4716=ORIENTED_EDGE ( 'NONE', *, *, #21766, .T. ) ;
#4729=CARTESIAN_POINT ( 'NONE',  ( -7.022189441860112050E-16, 13.67729811471672896, -142.5141058028994507 ) ) ;
#4730=CARTESIAN_POINT ( 'NONE',  ( 1.749999999999998224, 14.46891108675448478, -110.3213974700441042 ) ) ;
#4731=CARTESIAN_POINT ( 'NONE',  ( 1.750000000000001110, 20.53108891324555074, -54.29431413575484555 ) ) ;
#4732=CARTESIAN_POINT ( 'NONE',  ( -7.022189441860112050E-16, 13.67729811471672718, -129.6016058028994564 ) ) ;
#4733=CARTESIAN_POINT ( 'NONE',  ( -3.310556943750001313, 17.50000000000001421, -55.85160580289947063 ) ) ;
#4734=ORIENTED_EDGE ( 'NONE', *, *, #23272, .F. ) ;
#4736=CARTESIAN_POINT ( 'NONE',  ( 3.500000000000001332, 17.50000000000002487, -143.1547308033774186 ) ) ;
#4738=CARTESIAN_POINT ( 'NONE',  ( 3.500000000000001332, 17.50000000000001066, -43.15473080337743284 ) ) ;
#4740=CARTESIAN_POINT ( 'NONE',  ( 2.474675557024783212E-16, 21.54145188432740099, -129.2109808024214885 ) ) ;
#4741=CARTESIAN_POINT ( 'NONE',  ( 3.310556943750001313, 19.41135094264166838, -111.1807724695661506 ) ) ;
#4744=CARTESIAN_POINT ( 'NONE',  ( -1.750000000000002220, 14.46891108675448301, -85.79431413575483134 ) ) ;
#4745=LINE ( 'NONE', #37090, #2903 ) ;
#4746=CARTESIAN_POINT ( 'NONE',  ( -3.310556943750002645, 15.58864905735836714, -50.68077246956613635 ) ) ;
#4747=VECTOR ( 'NONE', #29622, 1000.000000000000000 ) ;
#4748=CARTESIAN_POINT ( 'NONE',  ( 3.310556943750001313, 19.41135094264166838, -106.2682724695661278 ) ) ;
#4749=DIRECTION ( 'NONE',  ( -0.000000000000000000, 1.259100132267607459E-16, -1.000000000000000000 ) ) ;
#4751=CARTESIAN_POINT ( 'NONE',  ( -1.394453263437886604E-15, 14.00000000000001421, -72.40473080337743284 ) ) ;
#4752=CARTESIAN_POINT ( 'NONE',  ( -7.022189441860112050E-16, 13.67729811471672896, -128.6016058028994848 ) ) ;
#4755=CARTESIAN_POINT ( 'NONE',  ( 3.500000000000001332, 19.52072594216371115, -83.07139747004410424 ) ) ;
#4756=CARTESIAN_POINT ( 'NONE',  ( 1.749999999999998224, 14.46891108675448123, -86.32139747004409003 ) ) ;
#4757=CARTESIAN_POINT ( 'NONE',  ( 1.655278471874998436, 14.63297358603754184, -59.51827246956613493 ) ) ;
#4759=CARTESIAN_POINT ( 'NONE',  ( 3.310556943749999981, 15.58864905735836714, -78.43493913623278502 ) ) ;
#4760=CARTESIAN_POINT ( 'NONE',  ( 3.500000000000001332, 19.52072594216370405, -30.07139747004410069 ) ) ;
#4761=CARTESIAN_POINT ( 'NONE',  ( 4.648177544792955347E-16, 21.00000000000001066, -44.21098080242150985 ) ) ;
#4764=CARTESIAN_POINT ( 'NONE',  ( 3.310556943750001313, 19.41135094264166128, -40.18077246956613635 ) ) ;
#4765=EDGE_CURVE ( 'NONE', #1224, #1017, #38080, .T. ) ;
#4766=CARTESIAN_POINT ( 'NONE',  ( -3.310556943750000425, 19.41135094264166483, -93.84743913623279354 ) ) ;
#4769=ORIENTED_EDGE ( 'NONE', *, *, #15523, .F. ) ;
#4771=CARTESIAN_POINT ( 'NONE',  ( -1.655278471875002211, 14.63297358603754184, -50.59743913623280775 ) ) ;
#4773=VERTEX_POINT ( 'NONE', #34753 ) ;
#4774=FACE_OUTER_BOUND ( 'NONE', #15283, .T. ) ;
#4778=CARTESIAN_POINT ( 'NONE',  ( 0.9378221735089300459, 21.00000000000002132, -113.2556390011600200 ) ) ;
#4781=CARTESIAN_POINT ( 'NONE',  ( -3.500000000000002220, 15.47927405783632082, -38.87764746908817415 ) ) ;
#4784=CARTESIAN_POINT ( 'NONE',  ( -3.695301148110399846E-14, 21.00000000000002132, -125.2109808024214885 ) ) ;
#4785=( BOUNDED_CURVE ( )  B_SPLINE_CURVE ( 2, ( #17776, #34357, #27352, #2233, #27564, #21798, #37545, #14796, #2019 ),
 .UNSPECIFIED., .F., .F. ) 
 B_SPLINE_CURVE_WITH_KNOTS ( ( 3, 2, 2, 2, 3 ),
 ( 0.7770833333333333481, 0.7777777777777777901, 0.7791666666666666741, 0.7805555555555555580, 0.7812500000000000000 ),
 .UNSPECIFIED. ) 
 CURVE ( )  GEOMETRIC_REPRESENTATION_ITEM ( )  RATIONAL_B_SPLINE_CURVE ( ( 0.9330127018922194093, 0.9330127018922194093, 1.000000000000000000, 0.8660254037844387076, 1.000000000000000000, 0.8660254037844387076, 1.000000000000000000, 0.9330127018922194093, 0.9330127018922194093 ) ) 
 REPRESENTATION_ITEM ( '' )  );
#4786=EDGE_CURVE ( 'NONE', #31496, #21662, #31147, .T. ) ;
#4788=CARTESIAN_POINT ( 'NONE',  ( -3.310556943750000425, 19.41135094264165772, -30.93493913623279923 ) ) ;
#4789=CARTESIAN_POINT ( 'NONE',  ( 1.750000000000001110, 20.53108891324555785, -121.9880641367107614 ) ) ;
#4790=CARTESIAN_POINT ( 'NONE',  ( -3.310556943750001313, 17.50000000000002487, -129.7641058028994507 ) ) ;
#4795=CARTESIAN_POINT ( 'NONE',  ( 3.310556943750001313, 19.41135094264166838, -122.2682724695661278 ) ) ;
#4796=FACE_OUTER_BOUND ( 'NONE', #41078, .T. ) ;
#4797=CARTESIAN_POINT ( 'NONE',  ( 1.655278471875001101, 20.36702641396249192, -88.09743913623280775 ) ) ;
#4799=CARTESIAN_POINT ( 'NONE',  ( 4.648177544792955347E-16, 21.00000000000001421, -64.90473080337743284 ) ) ;
#4800=CARTESIAN_POINT ( 'NONE',  ( 3.310556943750001313, 17.50000000000002487, -143.3516058028994564 ) ) ;
#4801=CARTESIAN_POINT ( 'NONE',  ( -1.750000000000002220, 14.46891108675448123, -72.48806413671076143 ) ) ;
#4802=CARTESIAN_POINT ( 'NONE',  ( 3.310556943750001313, 19.41135094264166483, -54.26827246956612782 ) ) ;
#4805=CARTESIAN_POINT ( 'NONE',  ( -3.310556943750000425, 19.41135094264166483, -76.93493913623278502 ) ) ;
#4806=CARTESIAN_POINT ( 'NONE',  ( -1.655278471875002211, 14.63297358603755427, -138.6849391362327992 ) ) ;
#4808=CARTESIAN_POINT ( 'NONE',  ( -7.022189441860112050E-16, 13.67729811471672541, -102.5141058028994649 ) ) ;
#4809=CARTESIAN_POINT ( 'NONE',  ( -3.310556943750001313, 17.50000000000001776, -77.76410580289946495 ) ) ;
#4810=ORIENTED_EDGE ( 'NONE', *, *, #17303, .T. ) ;
#4812=CARTESIAN_POINT ( 'NONE',  ( -1.655278471874999990, 20.36702641396249192, -95.01827246956612782 ) ) ;
#4815=CYLINDRICAL_SURFACE ( 'NONE', #38306, 3.499999999999999556 ) ;
#4817=CARTESIAN_POINT ( 'NONE',  ( 1.655278471875001101, 20.36702641396248836, -53.09743913623281486 ) ) ;
#4820=CARTESIAN_POINT ( 'NONE',  ( 2.340729813953370519E-16, 21.32270188528331900, -115.0141058028994934 ) ) ;
#4823=VERTEX_POINT ( 'NONE', #29191 ) ;
#4825=ORIENTED_EDGE ( 'NONE', *, *, #17100, .F. ) ;
#4827=CARTESIAN_POINT ( 'NONE',  ( 2.340729813953370519E-16, 21.32270188528330834, -69.01410580289947916 ) ) ;
#4828=ORIENTED_EDGE ( 'NONE', *, *, #8193, .T. ) ;
#4831=CARTESIAN_POINT ( 'NONE',  ( 1.743066579297357930E-14, 14.00000000000002132, -128.7109808024214885 ) ) ;
#4837=CARTESIAN_POINT ( 'NONE',  ( -3.310556943750001313, 17.50000000000002487, -131.7641058028994507 ) ) ;
#4838=CARTESIAN_POINT ( 'NONE',  ( -3.500000000000000000, 19.52072594216371826, -131.7380641367107614 ) ) ;
#4840=CARTESIAN_POINT ( 'NONE',  ( -3.310556943750001313, 17.50000000000001066, -44.85160580289947063 ) ) ;
#4841=CARTESIAN_POINT ( 'NONE',  ( 3.310556943749999981, 15.58864905735836182, -31.43493913623279923 ) ) ;
#4842=CARTESIAN_POINT ( 'NONE',  ( -1.655278471875002211, 14.63297358603754894, -99.68493913623279923 ) ) ;
#4844=CARTESIAN_POINT ( 'NONE',  ( -7.022189441860112050E-16, 13.67729811471672896, -137.6016058028994564 ) ) ;
#4846=CARTESIAN_POINT ( 'NONE',  ( -3.500000000000000888, 19.52072594216371115, -98.04431413575484555 ) ) ;
#4849=CARTESIAN_POINT ( 'NONE',  ( -1.749999999999999778, 20.53108891324555429, -86.82139747004409003 ) ) ;
#4850=CARTESIAN_POINT ( 'NONE',  ( -3.310556943750001313, 17.50000000000001421, -71.85160580289947063 ) ) ;
#4855=CARTESIAN_POINT ( 'NONE',  ( -7.424026671074350129E-16, 13.45854811567263276, -50.71098080242151696 ) ) ;
#4856=CARTESIAN_POINT ( 'NONE',  ( -3.310556943750002201, 15.58864905735837780, -117.6807724695661364 ) ) ;
#4857=CYLINDRICAL_SURFACE ( 'NONE', #39375, 3.499999999999999556 ) ;
#4858=CARTESIAN_POINT ( 'NONE',  ( -1.750000000000002220, 14.46891108675447590, -34.79431413575484555 ) ) ;
#4860=CARTESIAN_POINT ( 'NONE',  ( -3.500000000000001332, 17.50000000000002132, -113.6547308033774328 ) ) ;
#4863=CARTESIAN_POINT ( 'NONE',  ( 0.9378221735089281585, 14.00000000000000888, -37.66632260368299256 ) ) ;
#4866=CARTESIAN_POINT ( 'NONE',  ( 1.655278471875001101, 20.36702641396248836, -70.09743913623280775 ) ) ;
#4867=EDGE_CURVE ( 'NONE', #27019, #24771, #29123, .T. ) ;
#4868=( BOUNDED_CURVE ( )  B_SPLINE_CURVE ( 2, ( #7575, #14164, #20335, #7158, #23963, #20127, #33302, #26938, #27140 ),
 .UNSPECIFIED., .F., .T. ) 
 B_SPLINE_CURVE_WITH_KNOTS ( ( 3, 2, 2, 2, 3 ),
 ( 0.3479166666666666519, 0.3486111111111110938, 0.3499999999999999778, 0.3513888888888888618, 0.3520833333333333592 ),
 .UNSPECIFIED. ) 
 CURVE ( )  GEOMETRIC_REPRESENTATION_ITEM ( )  RATIONAL_B_SPLINE_CURVE ( ( 0.9330127018922194093, 0.9330127018922194093, 1.000000000000000000, 0.8660254037844387076, 1.000000000000000000, 0.8660254037844387076, 1.000000000000000000, 0.9330127018922167448, 0.9330127018922194093 ) ) 
 REPRESENTATION_ITEM ( '' )  );
#4871=EDGE_CURVE ( 'NONE', #4672, #11828, #27537, .T. ) ;
#4872=CARTESIAN_POINT ( 'NONE',  ( -1.394453263437886604E-15, 14.00000000000001421, -65.71098080242150274 ) ) ;
#4875=CARTESIAN_POINT ( 'NONE',  ( 1.655278471874998436, 14.63297358603754539, -84.43077246956613635 ) ) ;
#4877=ORIENTED_EDGE ( 'NONE', *, *, #38855, .F. ) ;
#4880=FACE_OUTER_BOUND ( 'NONE', #34474, .T. ) ;
#4881=VERTEX_POINT ( 'NONE', #2848 ) ;
#4882=CARTESIAN_POINT ( 'NONE',  ( 4.286263797015737581E-16, 14.00000000000002487, -149.5231586289125687 ) ) ;
#4883=CARTESIAN_POINT ( 'NONE',  ( -3.310556943750002645, 15.58864905735836714, -50.76827246956612072 ) ) ;
#4884=CARTESIAN_POINT ( 'NONE',  ( 3.310556943750001313, 19.41135094264166838, -116.2682724695661420 ) ) ;
#4885=ORIENTED_EDGE ( 'NONE', *, *, #10155, .T. ) ;
#4886=CARTESIAN_POINT ( 'NONE',  ( -1.750000000000002220, 14.46891108675448656, -122.4880641367107614 ) ) ;
#4889=CARTESIAN_POINT ( 'NONE',  ( 3.310556943750001313, 19.41135094264165772, -35.18077246956615056 ) ) ;
#4890=CARTESIAN_POINT ( 'NONE',  ( 3.310556943749999981, 15.58864905735836537, -66.43493913623279923 ) ) ;
#4891=CARTESIAN_POINT ( 'NONE',  ( 1.750000000000001110, 20.53108891324555785, -113.2943141357548456 ) ) ;
#4892=EDGE_CURVE ( 'NONE', #11460, #1684, #12633, .T. ) ;
#4894=CARTESIAN_POINT ( 'NONE',  ( -7.022189441860112050E-16, 13.67729811471672541, -97.51410580289947916 ) ) ;
#4896=CARTESIAN_POINT ( 'NONE',  ( 1.750000000000001110, 20.53108891324555074, -51.98806413671076854 ) ) ;
#4897=CARTESIAN_POINT ( 'NONE',  ( -1.394453263437886604E-15, 14.00000000000001776, -85.40473080337743284 ) ) ;
#4899=CARTESIAN_POINT ( 'NONE',  ( 3.500000000000001332, 17.50000000000001421, -64.46098080242150274 ) ) ;
#4900=CARTESIAN_POINT ( 'NONE',  ( -1.655278471875002211, 14.63297358603754006, -30.59743913623280775 ) ) ;
#4901=CARTESIAN_POINT ( 'NONE',  ( 3.310556943749999981, 15.58864905735836892, -91.43493913623279923 ) ) ;
#4902=CARTESIAN_POINT ( 'NONE',  ( -3.500000000000000888, 19.52072594216370760, -51.73806413671076854 ) ) ;
#4903=CARTESIAN_POINT ( 'NONE',  ( 3.500000000000000000, 15.47927405783632793, -92.54431413575484555 ) ) ;
#4904=CARTESIAN_POINT ( 'NONE',  ( 3.310556943749999981, 15.58864905735837070, -108.4349391362327992 ) ) ;
#4905=CARTESIAN_POINT ( 'NONE',  ( 1.655278471874998436, 14.63297358603753828, -38.51827246956612782 ) ) ;
#4907=CARTESIAN_POINT ( 'NONE',  ( 3.500000000000001332, 19.52072594216371826, -135.3776474690881741 ) ) ;
#4908=ADVANCED_FACE ( 'NONE', ( #35384 ), #6460, .T. ) ;
#4912=CARTESIAN_POINT ( 'NONE',  ( -0.9378221735089291577, 21.00000000000001421, -50.16632260368299256 ) ) ;
#4913=CARTESIAN_POINT ( 'NONE',  ( -3.310556943750002201, 15.58864905735837247, -90.68077246956613635 ) ) ;
#4914=CARTESIAN_POINT ( 'NONE',  ( 3.500000000000000000, 15.47927405783633326, -117.2380641367107614 ) ) ;
#4916=ORIENTED_EDGE ( 'NONE', *, *, #30708, .T. ) ;
#4917=CARTESIAN_POINT ( 'NONE',  ( 0.9378221735089281585, 14.00000000000001243, -57.66632260368298546 ) ) ;
#4918=CARTESIAN_POINT ( 'NONE',  ( -1.750000000000002220, 14.46891108675447946, -64.79431413575484555 ) ) ;
#4919=ORIENTED_EDGE ( 'NONE', *, *, #39997, .F. ) ;
#4923=VERTEX_POINT ( 'NONE', #3059 ) ;
#4924=CARTESIAN_POINT ( 'NONE',  ( 4.648177544792955347E-16, 21.00000000000002132, -117.9047308033774328 ) ) ;
#4929=ORIENTED_EDGE ( 'NONE', *, *, #27344, .F. ) ;
#4931=CARTESIAN_POINT ( 'NONE',  ( 3.369928719974892676E-15, 14.00000000000002309, -140.4047308033774186 ) ) ;
#4932=CARTESIAN_POINT ( 'NONE',  ( -7.022189441860112050E-16, 13.67729811471672718, -134.5141058028994507 ) ) ;
#4934=CARTESIAN_POINT ( 'NONE',  ( -0.9378221735089310451, 14.00000000000002309, -132.4493890021159359 ) ) ;
#4937=CYLINDRICAL_SURFACE ( 'NONE', #24817, 3.499999999999999556 ) ;
#4938=CARTESIAN_POINT ( 'NONE',  ( -3.310556943750000425, 19.41135094264166838, -128.9349391362327992 ) ) ;
#4939=CARTESIAN_POINT ( 'NONE',  ( 3.310556943749999981, 15.58864905735836537, -58.43493913623279212 ) ) ;
#4943=CARTESIAN_POINT ( 'NONE',  ( 3.500000000000000000, 15.47927405783633503, -137.2380641367107899 ) ) ;
#4945=CARTESIAN_POINT ( 'NONE',  ( 3.500000000000001332, 17.50000000000002132, -126.4609808024215170 ) ) ;
#4946=CARTESIAN_POINT ( 'NONE',  ( -3.310556943750000425, 19.41135094264166838, -113.8474391362328078 ) ) ;
#4949=CARTESIAN_POINT ( 'NONE',  ( 1.750000000000001110, 20.53108891324555429, -80.29431413575484555 ) ) ;
#4950=CARTESIAN_POINT ( 'NONE',  ( 3.500000000000001332, 19.52072594216370760, -51.37764746908816704 ) ) ;
#4951=CARTESIAN_POINT ( 'NONE',  ( 2.340729813953370519E-16, 21.32270188528330834, -47.01410580289947205 ) ) ;
#4952=CARTESIAN_POINT ( 'NONE',  ( -3.310556943750002645, 15.58864905735837425, -104.7682724695661420 ) ) ;
#4953=CARTESIAN_POINT ( 'NONE',  ( -1.749999999999999778, 20.53108891324556140, -130.8213974700441042 ) ) ;
#4956=CARTESIAN_POINT ( 'NONE',  ( 3.310556943749999981, 15.58864905735837425, -128.4349391362327992 ) ) ;
#4960=CARTESIAN_POINT ( 'NONE',  ( 1.749999999999998224, 14.46891108675448656, -124.3213974700440900 ) ) ;
#4962=CARTESIAN_POINT ( 'NONE',  ( -3.310556943750001313, 17.50000000000001421, -60.85160580289945642 ) ) ;
#4963=EDGE_LOOP ( 'NONE', ( #31946, #22444, #32378, #28566 ) ) ;
#4964=CARTESIAN_POINT ( 'NONE',  ( -7.022189441860112050E-16, 13.67729811471672186, -79.60160580289945642 ) ) ;
#4965=CARTESIAN_POINT ( 'NONE',  ( 0.9378221735089281585, 14.00000000000001243, -58.36007260463891555 ) ) ;
#4967=DIRECTION ( 'NONE',  ( -0.000000000000000000, 1.259100132267607459E-16, -1.000000000000000000 ) ) ;
#4970=AXIS2_PLACEMENT_3D ( 'NONE', #20126, #36283, #29903 ) ;
#4972=CARTESIAN_POINT ( 'NONE',  ( 1.655278471874998436, 14.63297358603754006, -40.43077246956613635 ) ) ;
#4974=CARTESIAN_POINT ( 'NONE',  ( 4.648177544792955347E-16, 21.00000000000001776, -83.90473080337743284 ) ) ;
#4976=ORIENTED_EDGE ( 'NONE', *, *, #38428, .F. ) ;
#4978=CARTESIAN_POINT ( 'NONE',  ( 3.310556943750001313, 19.41135094264165772, -46.18077246956615056 ) ) ;
#4979=( BOUNDED_CURVE ( )  B_SPLINE_CURVE ( 2, ( #23128, #4194, #29717, #39923, #36309, #30348, #36523, #17178, #30138 ),
 .UNSPECIFIED., .F., .F. ) 
 B_SPLINE_CURVE_WITH_KNOTS ( ( 3, 2, 2, 2, 3 ),
 ( 0.2104166666666666685, 0.2111111111111111105, 0.2124999999999999944, 0.2138888888888888784, 0.2145833333333333481 ),
 .UNSPECIFIED. ) 
 CURVE ( )  GEOMETRIC_REPRESENTATION_ITEM ( )  RATIONAL_B_SPLINE_CURVE ( ( 0.9330127018922194093, 0.9330127018922194093, 1.000000000000000000, 0.8660254037844387076, 1.000000000000000000, 0.8660254037844387076, 1.000000000000000000, 0.9330127018922180770, 0.9330127018922194093 ) ) 
 REPRESENTATION_ITEM ( '' )  );
#4980=ORIENTED_EDGE ( 'NONE', *, *, #1977, .F. ) ;
#4981=ORIENTED_EDGE ( 'NONE', *, *, #37568, .T. ) ;
#4982=CARTESIAN_POINT ( 'NONE',  ( -3.500000000000002220, 15.47927405783632437, -43.57139747004409713 ) ) ;
#4983=CARTESIAN_POINT ( 'NONE',  ( -1.750000000000002220, 14.46891108675447413, -23.79431413575484910 ) ) ;
#4986=ORIENTED_EDGE ( 'NONE', *, *, #1036, .F. ) ;
#4987=CARTESIAN_POINT ( 'NONE',  ( 1.750000000000001110, 20.53108891324554719, -43.29431413575483845 ) ) ;
#4988=CARTESIAN_POINT ( 'NONE',  ( 2.474675557024783212E-16, 21.54145188432739033, -36.21098080242150274 ) ) ;
#4989=CARTESIAN_POINT ( 'NONE',  ( -7.460324959392693302E-14, 21.00000000000001776, -86.21098080242150274 ) ) ;
#4990=CYLINDRICAL_SURFACE ( 'NONE', #2684, 3.499999999999999556 ) ;
#4993=CARTESIAN_POINT ( 'NONE',  ( -1.655278471875002211, 14.63297358603753828, -25.68493913623279212 ) ) ;
#4994=CARTESIAN_POINT ( 'NONE',  ( 4.648177544792955347E-16, 21.00000000000002132, -106.9047308033774328 ) ) ;
#4995=CARTESIAN_POINT ( 'NONE',  ( 1.655278471874998436, 14.63297358603755072, -130.4307724695661364 ) ) ;
#4998=CARTESIAN_POINT ( 'NONE',  ( 1.749999999999998224, 14.46891108675447413, -29.32139747004410069 ) ) ;
#4999=CARTESIAN_POINT ( 'NONE',  ( -1.655278471874999990, 20.36702641396249547, -122.0182724695661278 ) ) ;
#5000=CARTESIAN_POINT ( 'NONE',  ( 3.500000000000001776, 19.52072594216370405, -36.07139747004409003 ) ) ;
#5001=CARTESIAN_POINT ( 'NONE',  ( -1.394453263437886604E-15, 14.00000000000001421, -56.40473080337742573 ) ) ;
#5003=DIRECTION ( 'NONE',  ( 0.000000000000000000, 1.000000000000000000, 0.000000000000000000 ) ) ;
#5004=CARTESIAN_POINT ( 'NONE',  ( 0.9378221735089300459, 21.00000000000001066, -24.94938900211595723 ) ) ;
#5005=CARTESIAN_POINT ( 'NONE',  ( 3.500000000000000000, 15.47927405783632437, -70.23806413671077564 ) ) ;
#5007=CARTESIAN_POINT ( 'NONE',  ( -3.310556943750000425, 19.41135094264166483, -54.93493913623280633 ) ) ;
#5010=CARTESIAN_POINT ( 'NONE',  ( -1.655278471874999990, 20.36702641396249192, -76.01827246956612782 ) ) ;
#5012=CARTESIAN_POINT ( 'NONE',  ( 3.310556943750001313, 19.41135094264166838, -106.1807724695661364 ) ) ;
#5013=CARTESIAN_POINT ( 'NONE',  ( -7.022189441860112050E-16, 13.67729811471672186, -74.51410580289947916 ) ) ;
#5015=CARTESIAN_POINT ( 'NONE',  ( 3.310556943749999981, 15.58864905735837070, -96.43493913623281344 ) ) ;
#5017=CARTESIAN_POINT ( 'NONE',  ( -1.749999999999999778, 20.53108891324555429, -86.82139747004409003 ) ) ;
#5018=CARTESIAN_POINT ( 'NONE',  ( 0.9378221735089281585, 14.00000000000001066, -51.36007260463890134 ) ) ;
#5020=CARTESIAN_POINT ( 'NONE',  ( 3.310556943750001313, 17.50000000000001421, -58.26410580289947916 ) ) ;
#5022=CARTESIAN_POINT ( 'NONE',  ( 1.655278471874998436, 14.63297358603754894, -111.4307724695661506 ) ) ;
#5023=CARTESIAN_POINT ( 'NONE',  ( 0.9378221735089300459, 21.00000000000001776, -84.25563900116002003 ) ) ;
#5029=CARTESIAN_POINT ( 'NONE',  ( -1.750000000000002220, 14.46891108675448656, -109.7943141357548456 ) ) ;
#5030=CARTESIAN_POINT ( 'NONE',  ( -7.022189441860112050E-16, 13.67729811471671830, -64.51410580289946495 ) ) ;
#5031=ORIENTED_EDGE ( 'NONE', *, *, #41512, .F. ) ;
#5040=CARTESIAN_POINT ( 'NONE',  ( -3.500000000000000000, 19.52072594216371826, -143.0443141357548313 ) ) ;
#5041=CARTESIAN_POINT ( 'NONE',  ( 1.655278471875001101, 20.36702641396249902, -130.0974391362328220 ) ) ;
#5042=CARTESIAN_POINT ( 'NONE',  ( -0.9378221735089291577, 21.00000000000001776, -74.86007260463890134 ) ) ;
#5043=CARTESIAN_POINT ( 'NONE',  ( 2.340729813953370519E-16, 21.32270188528330479, -40.10160580289946353 ) ) ;
#5044=CARTESIAN_POINT ( 'NONE',  ( 2.340729813953370519E-16, 21.32270188528330479, -32.10160580289945642 ) ) ;
#5045=CARTESIAN_POINT ( 'NONE',  ( 3.310556943750001313, 19.41135094264166483, -91.26827246956614204 ) ) ;
#5046=CARTESIAN_POINT ( 'NONE',  ( 2.474675557024783212E-16, 21.54145188432739033, -26.90473080337743639 ) ) ;
#5048=EDGE_CURVE ( 'NONE', #39830, #35892, #40570, .T. ) ;
#5051=CARTESIAN_POINT ( 'NONE',  ( -7.022189441860112050E-16, 13.67729811471672896, -138.6016058028994564 ) ) ;
#5053=CARTESIAN_POINT ( 'NONE',  ( 4.648177544792955347E-16, 21.00000000000001776, -78.21098080242148853 ) ) ;
#5054=CARTESIAN_POINT ( 'NONE',  ( -7.424026671074350129E-16, 13.45854811567263631, -94.71098080242150274 ) ) ;
#5055=CARTESIAN_POINT ( 'NONE',  ( 0.9378221735089300459, 21.00000000000002487, -135.9493890021159359 ) ) ;
#5056=CARTESIAN_POINT ( 'NONE',  ( -0.9378221735089310451, 14.00000000000001599, -61.44938900211595012 ) ) ;
#5057=CARTESIAN_POINT ( 'NONE',  ( -3.500000000000002220, 15.47927405783632793, -87.57139747004409003 ) ) ;
#5058=CARTESIAN_POINT ( 'NONE',  ( -1.655278471875002211, 14.63297358603754539, -67.68493913623279923 ) ) ;
#5062=DIRECTION ( 'NONE',  ( 0.000000000000000000, 1.000000000000000000, 0.000000000000000000 ) ) ;
#5063=CARTESIAN_POINT ( 'NONE',  ( 3.500000000000000000, 15.47927405783632082, -47.54431413575483845 ) ) ;
#5064=CARTESIAN_POINT ( 'NONE',  ( -3.310556943750000425, 19.41135094264166838, -121.8474391362328078 ) ) ;
#5065=DIRECTION ( 'NONE',  ( 0.000000000000000000, 1.000000000000000000, 0.000000000000000000 ) ) ;
#5067=ORIENTED_EDGE ( 'NONE', *, *, #9863, .F. ) ;
#5068=CARTESIAN_POINT ( 'NONE',  ( 3.500000000000001776, 19.52072594216371826, -112.0713974700440900 ) ) ;
#5071=CARTESIAN_POINT ( 'NONE',  ( 0.9378221735089281585, 14.00000000000001599, -76.36007260463890134 ) ) ;
#5075=CARTESIAN_POINT ( 'NONE',  ( 2.340729813953370519E-16, 21.32270188528331190, -74.01410580289947916 ) ) ;
#5076=CARTESIAN_POINT ( 'NONE',  ( -1.749999999999999778, 20.53108891324556140, -134.1276474690881741 ) ) ;
#5077=EDGE_CURVE ( 'NONE', #5926, #15124, #10131, .T. ) ;
#5079=EDGE_CURVE ( 'NONE', #23270, #27029, #37417, .T. ) ;
#5081=CARTESIAN_POINT ( 'NONE',  ( -0.9378221735089291577, 21.00000000000002132, -104.1663226036829855 ) ) ;
#5082=CARTESIAN_POINT ( 'NONE',  ( -3.310556943750001313, 17.50000000000001776, -86.76410580289947916 ) ) ;
#5083=VERTEX_POINT ( 'NONE', #37623 ) ;
#5085=VECTOR ( 'NONE', #25775, 1000.000000000000000 ) ;
#5088=CARTESIAN_POINT ( 'NONE',  ( 4.286263797015737581E-16, 14.00000000000002487, -149.5231586289125687 ) ) ;
#5090=VERTEX_POINT ( 'NONE', #35061 ) ;
#5091=CARTESIAN_POINT ( 'NONE',  ( 3.310556943749999981, 15.58864905735836182, -49.43493913623279212 ) ) ;
#5092=CARTESIAN_POINT ( 'NONE',  ( -3.310556943750001313, 17.50000000000002132, -110.8516058028994564 ) ) ;
#5093=ORIENTED_EDGE ( 'NONE', *, *, #32081, .F. ) ;
#5094=EDGE_CURVE ( 'NONE', #19458, #1263, #41238, .T. ) ;
#5095=EDGE_CURVE ( 'NONE', #26058, #21358, #1689, .T. ) ;
#5096=EDGE_CURVE ( 'NONE', #4567, #3726, #7152, .T. ) ;
#5097=CARTESIAN_POINT ( 'NONE',  ( 3.310556943750001313, 19.41135094264165772, -33.18077246956615056 ) ) ;
#5098=CARTESIAN_POINT ( 'NONE',  ( 3.310556943750001313, 17.50000000000001421, -64.35160580289945642 ) ) ;
#5099=CARTESIAN_POINT ( 'NONE',  ( -3.500000000000002220, 15.47927405783633503, -114.8776474690881741 ) ) ;
#5101=CARTESIAN_POINT ( 'NONE',  ( 3.310556943750001313, 17.50000000000001776, -94.26410580289947916 ) ) ;
#5102=DIRECTION ( 'NONE',  ( 0.000000000000000000, 1.000000000000000000, 0.000000000000000000 ) ) ;
#5103=CARTESIAN_POINT ( 'NONE',  ( -0.9378221735089310451, 14.00000000000002309, -124.4493890021159359 ) ) ;
#5106=CARTESIAN_POINT ( 'NONE',  ( 3.500000000000001776, 19.52072594216370760, -65.37764746908818836 ) ) ;
#5107=DIRECTION ( 'NONE',  ( -0.000000000000000000, 1.259100132267607459E-16, -1.000000000000000000 ) ) ;
#5108=CARTESIAN_POINT ( 'NONE',  ( -3.310556943750002645, 15.58864905735836537, -34.68077246956615056 ) ) ;
#5109=CARTESIAN_POINT ( 'NONE',  ( -7.022189441860112050E-16, 13.67729811471672363, -88.60160580289947063 ) ) ;
#5111=CARTESIAN_POINT ( 'NONE',  ( 1.749999999999998224, 14.46891108675447768, -56.32139747004409713 ) ) ;
#5113=CARTESIAN_POINT ( 'NONE',  ( -3.310556943750002201, 15.58864905735837425, -104.7682724695661420 ) ) ;
#5114=CARTESIAN_POINT ( 'NONE',  ( 3.310556943750001313, 17.50000000000001066, -39.35160580289946353 ) ) ;
#5123=CARTESIAN_POINT ( 'NONE',  ( -7.022189441860112050E-16, 13.67729811471672363, -89.51410580289949337 ) ) ;
#5126=ORIENTED_EDGE ( 'NONE', *, *, #18089, .F. ) ;
#5128=CARTESIAN_POINT ( 'NONE',  ( -0.9378221735089310451, 14.00000000000002132, -101.7556390011600200 ) ) ;
#5135=DIRECTION ( 'NONE',  ( -0.000000000000000000, 1.259100132267607459E-16, -1.000000000000000000 ) ) ;
#5137=EDGE_CURVE ( 'NONE', #14839, #25969, #16148, .T. ) ;
#5144=VERTEX_POINT ( 'NONE', #32495 ) ;
#5145=CARTESIAN_POINT ( 'NONE',  ( -1.394453263437886604E-15, 14.00000000000002132, -109.4047308033774186 ) ) ;
#5146=CARTESIAN_POINT ( 'NONE',  ( 0.9378221735089279365, 21.00000000000002842, -139.9493890021159643 ) ) ;
#5147=CARTESIAN_POINT ( 'NONE',  ( 3.310556943750001313, 19.41135094264167549, -134.1807724695661364 ) ) ;
#5148=CARTESIAN_POINT ( 'NONE',  ( 1.749999999999998224, 14.46891108675447413, -38.32139747004409713 ) ) ;
#5149=VERTEX_POINT ( 'NONE', #10164 ) ;
#5152=CARTESIAN_POINT ( 'NONE',  ( 3.310556943749999981, 15.58864905735836182, -53.43493913623279923 ) ) ;
#5155=CARTESIAN_POINT ( 'NONE',  ( 1.749999999999998224, 14.46891108675448834, -136.3213974700441042 ) ) ;
#5156=EDGE_CURVE ( 'NONE', #31496, #38091, #36468, .T. ) ;
#5157=( BOUNDED_CURVE ( )  B_SPLINE_CURVE ( 2, ( #28439, #18244, #35040, #22069, #28026, #12709, #25687, #41642, #5901 ),
 .UNSPECIFIED., .F., .T. ) 
 B_SPLINE_CURVE_WITH_KNOTS ( ( 3, 2, 2, 2, 3 ),
 ( 0.7020833333333332815, 0.7027777777777777235, 0.7041666666666667185, 0.7055555555555556024, 0.7062500000000000444 ),
 .UNSPECIFIED. ) 
 CURVE ( )  GEOMETRIC_REPRESENTATION_ITEM ( )  RATIONAL_B_SPLINE_CURVE ( ( 0.9330127018922194093, 0.9330127018922194093, 1.000000000000000000, 0.8660254037844387076, 1.000000000000000000, 0.8660254037844387076, 1.000000000000000000, 0.9330127018922194093, 0.9330127018922194093 ) ) 
 REPRESENTATION_ITEM ( '' )  );
#5158=VECTOR ( 'NONE', #34488, 1000.000000000000000 ) ;
#5160=CARTESIAN_POINT ( 'NONE',  ( 3.500000000000001776, 19.52072594216371826, -128.3776474690881741 ) ) ;
#5161=CARTESIAN_POINT ( 'NONE',  ( -1.655278471874999990, 20.36702641396249547, -112.9307724695661364 ) ) ;
#5165=CARTESIAN_POINT ( 'NONE',  ( 3.500000000000000000, 15.47927405783632437, -78.54431413575484555 ) ) ;
#5167=CARTESIAN_POINT ( 'NONE',  ( 3.310556943750001313, 17.50000000000001421, -50.26410580289947205 ) ) ;
#5168=( BOUNDED_CURVE ( )  B_SPLINE_CURVE ( 2, ( #20348, #5596, #14177, #11756, #24753, #40899, #20562, #5378, #27154 ),
 .UNSPECIFIED., .F., .T. ) 
 B_SPLINE_CURVE_WITH_KNOTS ( ( 3, 2, 2, 2, 3 ),
 ( 0.3520833333333333592, 0.3527777777777778012, 0.3541666666666666852, 0.3555555555555555691, 0.3562500000000000111 ),
 .UNSPECIFIED. ) 
 CURVE ( )  GEOMETRIC_REPRESENTATION_ITEM ( )  RATIONAL_B_SPLINE_CURVE ( ( 0.9330127018922194093, 0.9330127018922220739, 1.000000000000000000, 0.8660254037844387076, 1.000000000000000000, 0.8660254037844387076, 1.000000000000000000, 0.9330127018922194093, 0.9330127018922194093 ) ) 
 REPRESENTATION_ITEM ( '' )  );
#5169=CARTESIAN_POINT ( 'NONE',  ( -1.655278471874999990, 20.36702641396249547, -105.0182724695661278 ) ) ;
#5171=CARTESIAN_POINT ( 'NONE',  ( -1.750000000000002220, 14.46891108675447768, -42.48806413671076143 ) ) ;
#5172=LINE ( 'NONE', #1969, #9394 ) ;
#5174=CARTESIAN_POINT ( 'NONE',  ( 3.310556943750001313, 17.50000000000002132, -122.3516058028994706 ) ) ;
#5177=CARTESIAN_POINT ( 'NONE',  ( -1.394453263437886604E-15, 14.00000000000001066, -27.71098080242150985 ) ) ;
#5178=CARTESIAN_POINT ( 'NONE',  ( -1.749999999999999778, 20.53108891324555074, -57.82139747004409713 ) ) ;
#5179=CARTESIAN_POINT ( 'NONE',  ( -1.655278471874999990, 20.36702641396248836, -57.01827246956612782 ) ) ;
#5180=VERTEX_POINT ( 'NONE', #26131 ) ;
#5181=CARTESIAN_POINT ( 'NONE',  ( -1.655278471874999990, 20.36702641396248836, -74.01827246956612782 ) ) ;
#5182=CARTESIAN_POINT ( 'NONE',  ( 0.000000000000000000, 17.50000000000002487, -149.5231586289125687 ) ) ;
#5185=LINE ( 'NONE', #11355, #19412 ) ;
#5187=CARTESIAN_POINT ( 'NONE',  ( 1.655278471875001101, 20.36702641396248481, -42.09743913623280065 ) ) ;
#5189=VERTEX_POINT ( 'NONE', #6971 ) ;
#5191=VERTEX_POINT ( 'NONE', #9966 ) ;
#5193=CARTESIAN_POINT ( 'NONE',  ( -3.310556943750002645, 15.58864905735836714, -46.68077246956614346 ) ) ;
#5195=ORIENTED_EDGE ( 'NONE', *, *, #2162, .F. ) ;
#5196=CARTESIAN_POINT ( 'NONE',  ( 4.648177544792955347E-16, 21.00000000000001421, -55.90473080337743284 ) ) ;
#5197=CARTESIAN_POINT ( 'NONE',  ( 1.750000000000001110, 20.53108891324554719, -25.29431413575484910 ) ) ;
#5202=CARTESIAN_POINT ( 'NONE',  ( 2.474675557024783212E-16, 21.54145188432739033, -41.21098080242151696 ) ) ;
#5204=CARTESIAN_POINT ( 'NONE',  ( 3.500000000000001332, 19.52072594216370760, -70.37764746908817415 ) ) ;
#5206=CARTESIAN_POINT ( 'NONE',  ( -1.655278471875002211, 14.63297358603753828, -24.68493913623280633 ) ) ;
#5207=CARTESIAN_POINT ( 'NONE',  ( 4.648177544792955347E-16, 21.00000000000002487, -132.2109808024214885 ) ) ;
#5208=CARTESIAN_POINT ( 'NONE',  ( -3.310556943750001313, 17.50000000000002132, -128.7641058028994792 ) ) ;
#5211=DIRECTION ( 'NONE',  ( -0.000000000000000000, 1.259100132267607459E-16, -1.000000000000000000 ) ) ;
#5212=CARTESIAN_POINT ( 'NONE',  ( -1.655278471874999990, 20.36702641396249547, -121.0182724695661278 ) ) ;
#5213=DIRECTION ( 'NONE',  ( -0.000000000000000000, 1.259100132267607459E-16, -1.000000000000000000 ) ) ;
#5214=CARTESIAN_POINT ( 'NONE',  ( -1.750000000000002220, 14.46891108675447590, -37.48806413671076854 ) ) ;
#5216=CARTESIAN_POINT ( 'NONE',  ( 1.743066579297357930E-14, 14.00000000000002132, -129.7109808024214885 ) ) ;
#5217=CARTESIAN_POINT ( 'NONE',  ( 2.340729813953370519E-16, 21.32270188528332255, -138.1016058028994564 ) ) ;
#5218=CARTESIAN_POINT ( 'NONE',  ( 3.500000000000001776, 19.52072594216370760, -69.07139747004409003 ) ) ;
#5219=CARTESIAN_POINT ( 'NONE',  ( 0.9378221735089300459, 21.00000000000001066, -29.25563900116003069 ) ) ;
#5220=CARTESIAN_POINT ( 'NONE',  ( 1.655278471875001101, 20.36702641396248836, -51.18493913623279923 ) ) ;
#5223=CARTESIAN_POINT ( 'NONE',  ( -3.310556943750002645, 15.58864905735837070, -73.76827246956612782 ) ) ;
#5225=CARTESIAN_POINT ( 'NONE',  ( -3.310556943750001313, 17.50000000000002132, -103.7641058028994649 ) ) ;
#5226=CARTESIAN_POINT ( 'NONE',  ( 1.655278471875001101, 20.36702641396248836, -69.09743913623280775 ) ) ;
#5228=CARTESIAN_POINT ( 'NONE',  ( -1.655278471875002211, 14.63297358603754894, -95.68493913623279923 ) ) ;
#5231=CARTESIAN_POINT ( 'NONE',  ( 0.9378221735089300459, 21.00000000000001066, -26.25563900116002714 ) ) ;
#5233=CARTESIAN_POINT ( 'NONE',  ( 1.655278471874998436, 14.63297358603754184, -56.43077246956614346 ) ) ;
#5234=( BOUNDED_CURVE ( )  B_SPLINE_CURVE ( 2, ( #18355, #27926, #31329, #8989, #21962, #18779, #12393, #25379, #38339 ),
 .UNSPECIFIED., .F., .F. ) 
 B_SPLINE_CURVE_WITH_KNOTS ( ( 3, 2, 2, 2, 3 ),
 ( 0.6895833333333333259, 0.6902777777777777679, 0.6916666666666666519, 0.6930555555555555358, 0.6937499999999999778 ),
 .UNSPECIFIED. ) 
 CURVE ( )  GEOMETRIC_REPRESENTATION_ITEM ( )  RATIONAL_B_SPLINE_CURVE ( ( 0.9330127018922194093, 0.9330127018922194093, 1.000000000000000000, 0.8660254037844387076, 1.000000000000000000, 0.8660254037844387076, 1.000000000000000000, 0.9330127018922194093, 0.9330127018922194093 ) ) 
 REPRESENTATION_ITEM ( '' )  );
#5236=CARTESIAN_POINT ( 'NONE',  ( 3.310556943750001313, 17.50000000000002132, -111.2641058028994649 ) ) ;
#5237=CARTESIAN_POINT ( 'NONE',  ( -1.394453263437886604E-15, 14.00000000000001776, -84.71098080242150274 ) ) ;
#5238=ORIENTED_EDGE ( 'NONE', *, *, #31612, .F. ) ;
#5239=VERTEX_POINT ( 'NONE', #2730 ) ;
#5243=CARTESIAN_POINT ( 'NONE',  ( -3.310556943750001313, 17.50000000000001421, -60.76410580289946495 ) ) ;
#5245=EDGE_LOOP ( 'NONE', ( #10789, #34582, #5662, #15126 ) ) ;
#5246=CARTESIAN_POINT ( 'NONE',  ( 0.000000000000000000, 17.50000000000002487, -149.5231586289125687 ) ) ;
#5249=LINE ( 'NONE', #6709, #27229 ) ;
#5253=CARTESIAN_POINT ( 'NONE',  ( 3.310556943750001313, 19.41135094264167549, -130.1807724695661364 ) ) ;
#5255=CARTESIAN_POINT ( 'NONE',  ( 1.655278471875001101, 20.36702641396248481, -39.18493913623280633 ) ) ;
#5256=CARTESIAN_POINT ( 'NONE',  ( -3.310556943750002645, 15.58864905735836537, -30.76827246956613848 ) ) ;
#5257=CARTESIAN_POINT ( 'NONE',  ( -3.310556943750000425, 19.41135094264166483, -94.93493913623278502 ) ) ;
#5258=CARTESIAN_POINT ( 'NONE',  ( 3.500000000000001332, 17.50000000000001066, -26.15473080337743639 ) ) ;
#5261=CARTESIAN_POINT ( 'NONE',  ( 2.340729813953370519E-16, 21.32270188528332255, -141.1016058028994564 ) ) ;
#5263=CARTESIAN_POINT ( 'NONE',  ( 3.500000000000001776, 19.52072594216371115, -94.37764746908817415 ) ) ;
#5264=CARTESIAN_POINT ( 'NONE',  ( 0.9378221735089324884, 14.00000000000002665, -136.3600726046389298 ) ) ;
#5265=CARTESIAN_POINT ( 'NONE',  ( 3.310556943750001313, 17.50000000000001421, -57.26410580289947916 ) ) ;
#5267=CARTESIAN_POINT ( 'NONE',  ( 1.749999999999998224, 14.46891108675448123, -86.32139747004409003 ) ) ;
#5268=CARTESIAN_POINT ( 'NONE',  ( 1.655278471874998436, 14.63297358603754361, -69.51827246956612782 ) ) ;
#5271=CARTESIAN_POINT ( 'NONE',  ( -0.9378221735089291577, 21.00000000000001776, -91.16632260368298546 ) ) ;
#5273=CARTESIAN_POINT ( 'NONE',  ( 1.750000000000001110, 20.53108891324555074, -47.29431413575483845 ) ) ;
#5274=CARTESIAN_POINT ( 'NONE',  ( 2.340729813953370519E-16, 21.32270188528331900, -122.0141058028994792 ) ) ;
#5275=CARTESIAN_POINT ( 'NONE',  ( 0.000000000000000000, 17.50000000000002487, -149.5231586289125687 ) ) ;
#5278=CARTESIAN_POINT ( 'NONE',  ( -3.500000000000001332, 17.50000000000002132, -111.6547308033774328 ) ) ;
#5284=CARTESIAN_POINT ( 'NONE',  ( 1.655278471875001101, 20.36702641396248836, -74.09743913623280775 ) ) ;
#5286=( BOUNDED_CURVE ( )  B_SPLINE_CURVE ( 2, ( #3986, #39284, #16968, #586, #29292, #9760, #3561, #9967, #6559 ),
 .UNSPECIFIED., .F., .F. ) 
 B_SPLINE_CURVE_WITH_KNOTS ( ( 3, 2, 2, 2, 3 ),
 ( 0.1229166666666666741, 0.1236111111111111160, 0.1250000000000000000, 0.1263888888888888840, 0.1270833333333333259 ),
 .UNSPECIFIED. ) 
 CURVE ( )  GEOMETRIC_REPRESENTATION_ITEM ( )  RATIONAL_B_SPLINE_CURVE ( ( 0.9330127018922194093, 0.9330127018922200755, 1.000000000000000000, 0.8660254037844387076, 1.000000000000000000, 0.8660254037844387076, 1.000000000000000000, 0.9330127018922194093, 0.9330127018922194093 ) ) 
 REPRESENTATION_ITEM ( '' )  );
#5287=CARTESIAN_POINT ( 'NONE',  ( -0.9378221735089310451, 14.00000000000001066, -44.75563900116002003 ) ) ;
#5288=ORIENTED_EDGE ( 'NONE', *, *, #16489, .F. ) ;
#5289=CARTESIAN_POINT ( 'NONE',  ( 2.340729813953370519E-16, 21.32270188528330834, -25.01410580289947916 ) ) ;
#5291=CARTESIAN_POINT ( 'NONE',  ( 3.310556943749999981, 15.58864905735836714, -80.34743913623279354 ) ) ;
#5292=EDGE_CURVE ( 'NONE', #9419, #18937, #36528, .T. ) ;
#5297=CARTESIAN_POINT ( 'NONE',  ( -1.836030130193217234E-14, 21.00000000000002132, -128.9047308033774470 ) ) ;
#5299=FACE_OUTER_BOUND ( 'NONE', #35109, .T. ) ;
#5300=CARTESIAN_POINT ( 'NONE',  ( 1.655278471875001101, 20.36702641396248836, -48.18493913623279923 ) ) ;
#5301=CARTESIAN_POINT ( 'NONE',  ( -3.310556943750002645, 15.58864905735837425, -106.7682724695661278 ) ) ;
#5302=VERTEX_POINT ( 'NONE', #11005 ) ;
#5303=EDGE_CURVE ( 'NONE', #38292, #31753, #17183, .T. ) ;
#5304=EDGE_CURVE ( 'NONE', #34399, #39141, #26405, .T. ) ;
#5305=CARTESIAN_POINT ( 'NONE',  ( 3.310556943750001313, 17.50000000000001066, -35.26410580289947205 ) ) ;
#5306=CARTESIAN_POINT ( 'NONE',  ( -3.310556943750002645, 15.58864905735836892, -59.76827246956613493 ) ) ;
#5307=CARTESIAN_POINT ( 'NONE',  ( 2.474675557024783212E-16, 21.54145188432740099, -111.2109808024215027 ) ) ;
#5309=CARTESIAN_POINT ( 'NONE',  ( 3.310556943749999981, 15.58864905735837070, -99.34743913623280775 ) ) ;
#5310=CYLINDRICAL_SURFACE ( 'NONE', #2356, 3.499999999999999556 ) ;
#5313=CARTESIAN_POINT ( 'NONE',  ( -3.500000000000002220, 15.47927405783632437, -64.87764746908818836 ) ) ;
#5314=CARTESIAN_POINT ( 'NONE',  ( 4.286263797015737581E-16, 14.00000000000002487, -149.5231586289125687 ) ) ;
#5315=CARTESIAN_POINT ( 'NONE',  ( -7.022189441860112050E-16, 13.67729811471671475, -33.51410580289947205 ) ) ;
#5316=CARTESIAN_POINT ( 'NONE',  ( -3.500000000000002220, 15.47927405783632437, -54.57139747004409003 ) ) ;
#5317=FACE_OUTER_BOUND ( 'NONE', #16277, .T. ) ;
#5318=CARTESIAN_POINT ( 'NONE',  ( 2.340729813953370519E-16, 21.32270188528331900, -109.1016058028994564 ) ) ;
#5319=CARTESIAN_POINT ( 'NONE',  ( 1.655278471874998436, 14.63297358603753828, -36.51827246956612782 ) ) ;
#5321=CARTESIAN_POINT ( 'NONE',  ( 0.9378221735089281585, 14.00000000000001066, -53.66632260368298546 ) ) ;
#5327=CARTESIAN_POINT ( 'NONE',  ( 3.310556943750001313, 19.41135094264166838, -88.18077246956613635 ) ) ;
#5328=DIRECTION ( 'NONE',  ( 0.000000000000000000, 1.000000000000000000, 0.000000000000000000 ) ) ;
#5329=ORIENTED_EDGE ( 'NONE', *, *, #35988, .F. ) ;
#5330=CARTESIAN_POINT ( 'NONE',  ( -1.749999999999999778, 20.53108891324555429, -102.1276474690881741 ) ) ;
#5331=CARTESIAN_POINT ( 'NONE',  ( 4.648177544792955347E-16, 21.00000000000001421, -54.21098080242150985 ) ) ;
#5332=ORIENTED_EDGE ( 'NONE', *, *, #33823, .T. ) ;
#5337=CARTESIAN_POINT ( 'NONE',  ( -7.460324959392693302E-14, 21.00000000000001776, -101.2109808024215170 ) ) ;
#5342=CARTESIAN_POINT ( 'NONE',  ( 4.286263797015737581E-16, 14.00000000000002487, -149.5231586289125687 ) ) ;
#5345=VERTEX_POINT ( 'NONE', #23255 ) ;
#5346=CARTESIAN_POINT ( 'NONE',  ( 1.749999999999998224, 14.46891108675448123, -91.32139747004410424 ) ) ;
#5348=CARTESIAN_POINT ( 'NONE',  ( -1.655278471874999990, 20.36702641396249902, -136.9307724695661364 ) ) ;
#5349=CARTESIAN_POINT ( 'NONE',  ( 4.648177544792955347E-16, 21.00000000000002132, -103.9047308033774186 ) ) ;
#5350=ORIENTED_EDGE ( 'NONE', *, *, #30406, .F. ) ;
#5351=CARTESIAN_POINT ( 'NONE',  ( -1.750000000000002220, 14.46891108675447590, -26.48806413671075788 ) ) ;
#5352=CARTESIAN_POINT ( 'NONE',  ( -3.310556943750002645, 15.58864905735837780, -123.7682724695661420 ) ) ;
#5353=CARTESIAN_POINT ( 'NONE',  ( -3.310556943750001313, 17.50000000000001421, -57.85160580289947063 ) ) ;
#5356=CARTESIAN_POINT ( 'NONE',  ( -3.500000000000000888, 19.52072594216372181, -136.7380641367107614 ) ) ;
#5358=CARTESIAN_POINT ( 'NONE',  ( -7.022189441860112050E-16, 13.67729811471672186, -78.60160580289944221 ) ) ;
#5359=CARTESIAN_POINT ( 'NONE',  ( -3.500000000000001332, 17.50000000000002132, -125.9609808024215170 ) ) ;
#5360=CARTESIAN_POINT ( 'NONE',  ( -1.655278471875002211, 14.63297358603755072, -111.5974391362328078 ) ) ;
#5364=CARTESIAN_POINT ( 'NONE',  ( 3.500000000000001332, 17.50000000000001776, -82.46098080242150274 ) ) ;
#5365=CARTESIAN_POINT ( 'NONE',  ( -1.394453263437886604E-15, 14.00000000000001776, -92.40473080337741862 ) ) ;
#5366=CARTESIAN_POINT ( 'NONE',  ( -3.310556943750002645, 15.58864905735836714, -45.68077246956614346 ) ) ;
#5367=CARTESIAN_POINT ( 'NONE',  ( 3.310556943750001313, 19.41135094264166838, -104.2682724695661420 ) ) ;
#5371=ADVANCED_FACE ( 'NONE', ( #9671 ), #39409, .T. ) ;
#5372=CARTESIAN_POINT ( 'NONE',  ( 3.310556943750001313, 17.50000000000002132, -121.3516058028994706 ) ) ;
#5377=CARTESIAN_POINT ( 'NONE',  ( -0.9378221735089291577, 21.00000000000001421, -57.86007260463890844 ) ) ;
#5378=CARTESIAN_POINT ( 'NONE',  ( -0.9378221735089310451, 14.00000000000002132, -100.7556390011600342 ) ) ;
#5379=CARTESIAN_POINT ( 'NONE',  ( -3.310556943750000425, 19.41135094264166128, -59.93493913623279212 ) ) ;
#5381=CARTESIAN_POINT ( 'NONE',  ( 1.655278471875001101, 20.36702641396249192, -75.18493913623279923 ) ) ;
#5383=DIRECTION ( 'NONE',  ( -0.000000000000000000, 1.259100132267607459E-16, -1.000000000000000000 ) ) ;
#5384=CARTESIAN_POINT ( 'NONE',  ( 3.500000000000001332, 17.50000000000001776, -80.15473080337743284 ) ) ;
#5387=CYLINDRICAL_SURFACE ( 'NONE', #36774, 3.499999999999999556 ) ;
#5389=CARTESIAN_POINT ( 'NONE',  ( -7.022189441860112050E-16, 13.67729811471671653, -38.51410580289947916 ) ) ;
#5390=EDGE_CURVE ( 'NONE', #21956, #38468, #11485, .T. ) ;
#5392=EDGE_CURVE ( 'NONE', #16027, #18829, #40815, .T. ) ;
#5394=ORIENTED_EDGE ( 'NONE', *, *, #24842, .T. ) ;
#5396=CARTESIAN_POINT ( 'NONE',  ( 1.655278471874998436, 14.63297358603754006, -45.43077246956614346 ) ) ;
#5397=ORIENTED_EDGE ( 'NONE', *, *, #29565, .F. ) ;
#5401=CARTESIAN_POINT ( 'NONE',  ( 1.749999999999998224, 14.46891108675447235, -23.62764746908817415 ) ) ;
#5403=( BOUNDED_CURVE ( )  B_SPLINE_CURVE ( 2, ( #10276, #33678, #23247, #20488, #4738, #4101, #36435, #923, #27296 ),
 .UNSPECIFIED., .F., .T. ) 
 B_SPLINE_CURVE_WITH_KNOTS ( ( 3, 2, 2, 2, 3 ),
 ( 0.8312500000000000444, 0.8319444444444444864, 0.8333333333333333703, 0.8347222222222222543, 0.8354166666666666963 ),
 .UNSPECIFIED. ) 
 CURVE ( )  GEOMETRIC_REPRESENTATION_ITEM ( )  RATIONAL_B_SPLINE_CURVE ( ( 0.9330127018922194093, 0.9330127018922194093, 1.000000000000000000, 0.8660254037844387076, 1.000000000000000000, 0.8660254037844387076, 1.000000000000000000, 0.9330127018922194093, 0.9330127018922194093 ) ) 
 REPRESENTATION_ITEM ( '' )  );
#5404=CARTESIAN_POINT ( 'NONE',  ( -1.394453263437886604E-15, 14.00000000000001421, -63.40473080337742573 ) ) ;
#5405=CARTESIAN_POINT ( 'NONE',  ( -1.394453263437886604E-15, 14.00000000000001066, -27.71098080242150630 ) ) ;
#5406=CARTESIAN_POINT ( 'NONE',  ( 3.500000000000001776, 19.52072594216370405, -38.37764746908817415 ) ) ;
#5408=DIRECTION ( 'NONE',  ( 0.000000000000000000, -0.000000000000000000, 1.000000000000000000 ) ) ;
#5410=CARTESIAN_POINT ( 'NONE',  ( 3.500000000000001332, 17.50000000000001776, -96.46098080242150274 ) ) ;
#5412=CARTESIAN_POINT ( 'NONE',  ( -3.310556943750000425, 19.41135094264165772, -25.93493913623279212 ) ) ;
#5413=CYLINDRICAL_SURFACE ( 'NONE', #27255, 3.499999999999999556 ) ;
#5414=CARTESIAN_POINT ( 'NONE',  ( 1.655278471875001101, 20.36702641396249902, -130.0974391362328220 ) ) ;
#5417=CARTESIAN_POINT ( 'NONE',  ( -1.394453263437886604E-15, 14.00000000000001776, -94.40473080337744705 ) ) ;
#5418=CARTESIAN_POINT ( 'NONE',  ( -3.310556943750000425, 19.41135094264166838, -124.9349391362327850 ) ) ;
#5420=CARTESIAN_POINT ( 'NONE',  ( 3.500000000000000000, 15.47927405783632082, -36.23806413671076854 ) ) ;
#5423=EDGE_CURVE ( 'NONE', #25189, #27672, #15867, .T. ) ;
#5424=CARTESIAN_POINT ( 'NONE',  ( -1.655278471875002211, 14.63297358603755427, -139.6849391362327708 ) ) ;
#5426=CARTESIAN_POINT ( 'NONE',  ( 3.310556943750001313, 19.41135094264166483, -50.26827246956614204 ) ) ;
#5429=CARTESIAN_POINT ( 'NONE',  ( 3.310556943750001313, 19.41135094264166128, -73.26827246956614204 ) ) ;
#5432=CARTESIAN_POINT ( 'NONE',  ( 3.310556943750001313, 17.50000000000002132, -106.2641058028994649 ) ) ;
#5433=CARTESIAN_POINT ( 'NONE',  ( 1.655278471875001101, 20.36702641396248836, -72.09743913623280775 ) ) ;
#5434=ORIENTED_EDGE ( 'NONE', *, *, #30885, .T. ) ;
#5435=CARTESIAN_POINT ( 'NONE',  ( -3.310556943750000425, 19.41135094264166838, -90.93493913623279923 ) ) ;
#5439=EDGE_CURVE ( 'NONE', #39717, #23270, #3052, .T. ) ;
#5441=CARTESIAN_POINT ( 'NONE',  ( 1.655278471875001101, 20.36702641396248836, -54.09743913623281486 ) ) ;
#5443=CARTESIAN_POINT ( 'NONE',  ( -3.310556943750002645, 15.58864905735837425, -108.6807724695661364 ) ) ;
#5450=CARTESIAN_POINT ( 'NONE',  ( -1.655278471874999990, 20.36702641396248836, -65.93077246956613635 ) ) ;
#5452=ORIENTED_EDGE ( 'NONE', *, *, #21945, .F. ) ;
#5453=DIRECTION ( 'NONE',  ( 0.000000000000000000, 1.000000000000000000, 0.000000000000000000 ) ) ;
#5454=DIRECTION ( 'NONE',  ( -0.000000000000000000, 1.259100132267607459E-16, -1.000000000000000000 ) ) ;
#5456=DIRECTION ( 'NONE',  ( 0.000000000000000000, 1.000000000000000000, 0.000000000000000000 ) ) ;
#5457=ORIENTED_EDGE ( 'NONE', *, *, #38296, .T. ) ;
#5459=CARTESIAN_POINT ( 'NONE',  ( -1.655278471874999990, 20.36702641396249547, -127.9307724695661364 ) ) ;
#5461=CARTESIAN_POINT ( 'NONE',  ( -3.500000000000001332, 17.50000000000002132, -102.9609808024215027 ) ) ;
#5462=CARTESIAN_POINT ( 'NONE',  ( 3.310556943750001313, 17.50000000000001066, -41.35160580289947063 ) ) ;
#5464=CARTESIAN_POINT ( 'NONE',  ( -3.310556943750000425, 19.41135094264165772, -31.93493913623279568 ) ) ;
#5465=CARTESIAN_POINT ( 'NONE',  ( 1.655278471875001101, 20.36702641396249192, -92.18493913623279923 ) ) ;
#5466=CARTESIAN_POINT ( 'NONE',  ( -1.749999999999999778, 20.53108891324554719, -25.82139747004409713 ) ) ;
#5469=VECTOR ( 'NONE', #10965, 1000.000000000000000 ) ;
#5471=CARTESIAN_POINT ( 'NONE',  ( 1.655278471875001101, 20.36702641396249902, -141.1849391362327708 ) ) ;
#5473=CARTESIAN_POINT ( 'NONE',  ( -1.749999999999999778, 20.53108891324555785, -123.1276474690881741 ) ) ;
#5474=CARTESIAN_POINT ( 'NONE',  ( -3.310556943750002645, 15.58864905735836892, -60.68077246956614346 ) ) ;
#5476=CARTESIAN_POINT ( 'NONE',  ( -1.749999999999999778, 20.53108891324555429, -82.82139747004410424 ) ) ;
#5477=CARTESIAN_POINT ( 'NONE',  ( 1.655278471874998436, 14.63297358603754184, -62.51827246956613493 ) ) ;
#5478=( BOUNDED_CURVE ( )  B_SPLINE_CURVE ( 2, ( #37794, #8650, #21622, #34598, #5461, #2275, #6923, #32250, #6713 ),
 .UNSPECIFIED., .F., .T. ) 
 B_SPLINE_CURVE_WITH_KNOTS ( ( 3, 2, 2, 2, 3 ),
 ( 0.3354166666666666963, 0.3361111111111111382, 0.3375000000000000222, 0.3388888888888889062, 0.3395833333333333481 ),
 .UNSPECIFIED. ) 
 CURVE ( )  GEOMETRIC_REPRESENTATION_ITEM ( )  RATIONAL_B_SPLINE_CURVE ( ( 0.9330127018922194093, 0.9330127018922220739, 1.000000000000000000, 0.8660254037844387076, 1.000000000000000000, 0.8660254037844387076, 1.000000000000000000, 0.9330127018922194093, 0.9330127018922194093 ) ) 
 REPRESENTATION_ITEM ( '' )  );
#5483=ORIENTED_EDGE ( 'NONE', *, *, #34811, .T. ) ;
#5484=CARTESIAN_POINT ( 'NONE',  ( 3.310556943750001313, 19.41135094264166838, -122.1807724695661364 ) ) ;
#5485=CARTESIAN_POINT ( 'NONE',  ( -1.394453263437886604E-15, 14.00000000000001066, -34.71098080242151696 ) ) ;
#5488=CARTESIAN_POINT ( 'NONE',  ( 3.500000000000000000, 15.47927405783632970, -111.2380641367107756 ) ) ;
#5491=EDGE_CURVE ( 'NONE', #14873, #35536, #11334, .T. ) ;
#5494=CARTESIAN_POINT ( 'NONE',  ( -3.310556943750001313, 17.50000000000001421, -72.76410580289947916 ) ) ;
#5496=VECTOR ( 'NONE', #40016, 1000.000000000000000 ) ;
#5497=LINE ( 'NONE', #5711, #18247 ) ;
#5499=EDGE_LOOP ( 'NONE', ( #26903, #23996, #4452, #12997 ) ) ;
#5500=CARTESIAN_POINT ( 'NONE',  ( -3.310556943750000425, 19.41135094264166128, -25.84743913623280420 ) ) ;
#5502=CARTESIAN_POINT ( 'NONE',  ( 3.310556943750001313, 17.50000000000001776, -79.26410580289946495 ) ) ;
#5503=ORIENTED_EDGE ( 'NONE', *, *, #29515, .T. ) ;
#5506=CARTESIAN_POINT ( 'NONE',  ( -3.500000000000002220, 15.47927405783633503, -127.8776474690881884 ) ) ;
#5511=CARTESIAN_POINT ( 'NONE',  ( -8.715332896486792803E-15, 21.00000000000002842, -137.2109808024214885 ) ) ;
#5512=CARTESIAN_POINT ( 'NONE',  ( 3.310556943750001313, 17.50000000000001421, -47.35160580289946353 ) ) ;
#5513=CARTESIAN_POINT ( 'NONE',  ( -7.022189441860112050E-16, 13.67729811471672718, -110.6016058028994706 ) ) ;
#5517=CARTESIAN_POINT ( 'NONE',  ( 2.340729813953370519E-16, 21.32270188528330479, -33.01410580289947205 ) ) ;
#5518=CARTESIAN_POINT ( 'NONE',  ( -1.655278471875002211, 14.63297358603754361, -63.68493913623279923 ) ) ;
#5519=CARTESIAN_POINT ( 'NONE',  ( -1.749999999999999778, 20.53108891324555785, -110.1276474690881741 ) ) ;
#5521=CARTESIAN_POINT ( 'NONE',  ( 3.310556943749999981, 15.58864905735836892, -89.34743913623279354 ) ) ;
#5522=CARTESIAN_POINT ( 'NONE',  ( 3.500000000000001332, 19.52072594216370760, -63.37764746908818125 ) ) ;
#5525=CARTESIAN_POINT ( 'NONE',  ( -1.749999999999999778, 20.53108891324555074, -63.12764746908818125 ) ) ;
#5526=CARTESIAN_POINT ( 'NONE',  ( -3.500000000000000000, 19.52072594216370760, -72.04431413575483134 ) ) ;
#5527=CARTESIAN_POINT ( 'NONE',  ( -1.655278471874999990, 20.36702641396248481, -25.93077246956613990 ) ) ;
#5528=( BOUNDED_CURVE ( )  B_SPLINE_CURVE ( 2, ( #2944, #31234, #28461, #22501, #9543, #12298, #35486, #18263, #15506 ),
 .UNSPECIFIED., .F., .T. ) 
 B_SPLINE_CURVE_WITH_KNOTS ( ( 3, 2, 2, 2, 3 ),
 ( 0.9270833333333333703, 0.9277777777777778123, 0.9291666666666666963, 0.9305555555555555802, 0.9312500000000000222 ),
 .UNSPECIFIED. ) 
 CURVE ( )  GEOMETRIC_REPRESENTATION_ITEM ( )  RATIONAL_B_SPLINE_CURVE ( ( 0.9330127018922194093, 0.9330127018922194093, 1.000000000000000000, 0.8660254037844387076, 1.000000000000000000, 0.8660254037844387076, 1.000000000000000000, 0.9330127018922194093, 0.9330127018922194093 ) ) 
 REPRESENTATION_ITEM ( '' )  );
#5530=CARTESIAN_POINT ( 'NONE',  ( -3.500000000000001332, 17.50000000000001421, -54.65473080337743284 ) ) ;
#5532=CARTESIAN_POINT ( 'NONE',  ( 2.340729813953370519E-16, 21.32270188528331900, -108.1016058028994706 ) ) ;
#5533=CARTESIAN_POINT ( 'NONE',  ( 3.310556943750001313, 17.50000000000001066, -38.35160580289946353 ) ) ;
#5538=DIRECTION ( 'NONE',  ( 0.000000000000000000, 1.000000000000000000, 0.000000000000000000 ) ) ;
#5540=CARTESIAN_POINT ( 'NONE',  ( -3.310556943750001313, 17.50000000000001776, -86.76410580289947916 ) ) ;
#5543=ORIENTED_EDGE ( 'NONE', *, *, #8488, .T. ) ;
#5546=ORIENTED_EDGE ( 'NONE', *, *, #15248, .F. ) ;
#5550=CARTESIAN_POINT ( 'NONE',  ( 3.310556943750001313, 19.41135094264166483, -95.18077246956613635 ) ) ;
#5553=CYLINDRICAL_SURFACE ( 'NONE', #31992, 3.499999999999999556 ) ;
#5560=EDGE_LOOP ( 'NONE', ( #111, #30563, #40560, #1639 ) ) ;
#5562=VECTOR ( 'NONE', #33870, 1000.000000000000000 ) ;
#5564=CARTESIAN_POINT ( 'NONE',  ( -3.310556943750001313, 17.50000000000002487, -136.7641058028994792 ) ) ;
#5565=ORIENTED_EDGE ( 'NONE', *, *, #40868, .T. ) ;
#5566=DIRECTION ( 'NONE',  ( 0.000000000000000000, 1.000000000000000000, 0.000000000000000000 ) ) ;
#5567=CARTESIAN_POINT ( 'NONE',  ( -3.310556943750001313, 17.50000000000002132, -125.8516058028994706 ) ) ;
#5568=CARTESIAN_POINT ( 'NONE',  ( -3.310556943750000425, 19.41135094264166128, -47.93493913623279212 ) ) ;
#5571=CARTESIAN_POINT ( 'NONE',  ( -3.500000000000001332, 17.50000000000002487, -134.6547308033774186 ) ) ;
#5572=( NAMED_UNIT ( * ) PLANE_ANGLE_UNIT ( ) SI_UNIT ( $, .RADIAN. ) );
#5574=CARTESIAN_POINT ( 'NONE',  ( -1.655278471875002211, 14.63297358603754539, -74.68493913623279923 ) ) ;
#5575=CARTESIAN_POINT ( 'NONE',  ( -3.500000000000000888, 19.52072594216371826, -127.0443141357548456 ) ) ;
#5576=CARTESIAN_POINT ( 'NONE',  ( 2.340729813953370519E-16, 21.32270188528331900, -111.0141058028994792 ) ) ;
#5582=CARTESIAN_POINT ( 'NONE',  ( -1.750000000000002220, 14.46891108675448301, -82.79431413575483134 ) ) ;
#5584=CARTESIAN_POINT ( 'NONE',  ( -3.310556943750001313, 17.50000000000001066, -40.76410580289947916 ) ) ;
#5585=EDGE_CURVE ( 'NONE', #1017, #37668, #4745, .T. ) ;
#5586=CARTESIAN_POINT ( 'NONE',  ( 3.310556943749999981, 15.58864905735837070, -99.43493913623281344 ) ) ;
#5587=CARTESIAN_POINT ( 'NONE',  ( 1.743066579297357930E-14, 14.00000000000002132, -129.7109808024214885 ) ) ;
#5588=CARTESIAN_POINT ( 'NONE',  ( 3.500000000000001332, 17.50000000000001066, -39.46098080242150985 ) ) ;
#5590=CARTESIAN_POINT ( 'NONE',  ( -3.310556943750001313, 17.50000000000002132, -124.8516058028994564 ) ) ;
#5595=CARTESIAN_POINT ( 'NONE',  ( -3.500000000000000000, 19.52072594216370760, -71.73806413671076143 ) ) ;
#5596=CARTESIAN_POINT ( 'NONE',  ( -0.9378221735089640188, 20.99999999999999645, -101.1663226036829855 ) ) ;
#5598=VERTEX_POINT ( 'NONE', #1561 ) ;
#5599=CARTESIAN_POINT ( 'NONE',  ( -7.022189441860112050E-16, 13.67729811471672186, -77.60160580289945642 ) ) ;
#5600=CARTESIAN_POINT ( 'NONE',  ( 1.749999999999998224, 14.46891108675447590, -40.62764746908817415 ) ) ;
#5601=CARTESIAN_POINT ( 'NONE',  ( 3.500000000000001332, 17.50000000000001066, -40.15473080337743284 ) ) ;
#5604=CARTESIAN_POINT ( 'NONE',  ( -1.655278471874999990, 20.36702641396248481, -35.93077246956613635 ) ) ;
#5607=CARTESIAN_POINT ( 'NONE',  ( 0.9378221735089281585, 14.00000000000001599, -72.36007260463891555 ) ) ;
#5608=EDGE_CURVE ( 'NONE', #35046, #21198, #37291, .T. ) ;
#5613=CARTESIAN_POINT ( 'NONE',  ( -3.310556943750000425, 19.41135094264166128, -48.84743913623280775 ) ) ;
#5616=ORIENTED_EDGE ( 'NONE', *, *, #38716, .F. ) ;
#5617=CARTESIAN_POINT ( 'NONE',  ( 1.750000000000001110, 20.53108891324555074, -55.98806413671076143 ) ) ;
#5618=FACE_OUTER_BOUND ( 'NONE', #11106, .T. ) ;
#5620=LINE ( 'NONE', #18175, #16359 ) ;
#5621=CARTESIAN_POINT ( 'NONE',  ( 3.500000000000001332, 17.50000000000001066, -39.46098080242150985 ) ) ;
#5623=CARTESIAN_POINT ( 'NONE',  ( -0.9378221735089310451, 14.00000000000001599, -64.44938900211595012 ) ) ;
#5624=DIRECTION ( 'NONE',  ( -0.000000000000000000, 1.259100132267607459E-16, -1.000000000000000000 ) ) ;
#5626=CARTESIAN_POINT ( 'NONE',  ( -3.310556943750001313, 17.50000000000001066, -26.85160580289947063 ) ) ;
#5627=CARTESIAN_POINT ( 'NONE',  ( -3.500000000000002220, 15.47927405783632437, -52.87764746908817415 ) ) ;
#5628=CARTESIAN_POINT ( 'NONE',  ( 2.340729813953370519E-16, 21.32270188528331900, -127.0141058028994507 ) ) ;
#5631=EDGE_CURVE ( 'NONE', #12942, #1684, #4673, .T. ) ;
#5632=CARTESIAN_POINT ( 'NONE',  ( -1.394453263437886604E-15, 14.00000000000001421, -76.40473080337740441 ) ) ;
#5634=CARTESIAN_POINT ( 'NONE',  ( 3.310556943749999981, 15.58864905735837247, -118.4349391362327992 ) ) ;
#5636=CARTESIAN_POINT ( 'NONE',  ( -1.749999999999999778, 20.53108891324554719, -35.82139747004409003 ) ) ;
#5637=CARTESIAN_POINT ( 'NONE',  ( -0.9378221735089310451, 14.00000000000002309, -121.4493890021159643 ) ) ;
#5639=CARTESIAN_POINT ( 'NONE',  ( 3.310556943749999981, 15.58864905735837780, -138.4349391362327708 ) ) ;
#5640=AXIS2_PLACEMENT_3D ( 'NONE', #23853, #36818, #28432 ) ;
#5642=CARTESIAN_POINT ( 'NONE',  ( 1.655278471874998436, 14.63297358603754006, -49.51827246956613493 ) ) ;
#5644=DIRECTION ( 'NONE',  ( -0.000000000000000000, 1.259100132267607459E-16, -1.000000000000000000 ) ) ;
#5645=AXIS2_PLACEMENT_3D ( 'NONE', #30414, #7242, #33820 ) ;
#5646=CARTESIAN_POINT ( 'NONE',  ( 2.340729813953370519E-16, 21.32270188528330834, -74.10160580289947063 ) ) ;
#5648=CARTESIAN_POINT ( 'NONE',  ( 2.340729813953370519E-16, 21.32270188528331190, -97.01410580289947916 ) ) ;
#5649=CARTESIAN_POINT ( 'NONE',  ( -3.310556943750001313, 17.50000000000001421, -71.76410580289947916 ) ) ;
#5651=CARTESIAN_POINT ( 'NONE',  ( 3.310556943750001313, 17.50000000000001776, -93.35160580289947063 ) ) ;
#5653=CARTESIAN_POINT ( 'NONE',  ( 1.750000000000001110, 20.53108891324555074, -49.29431413575484555 ) ) ;
#5654=CARTESIAN_POINT ( 'NONE',  ( -1.750000000000002220, 14.46891108675448301, -84.79431413575483134 ) ) ;
#5655=CARTESIAN_POINT ( 'NONE',  ( 3.310556943750001313, 17.50000000000001421, -56.26410580289947916 ) ) ;
#5657=CARTESIAN_POINT ( 'NONE',  ( 3.310556943750001313, 19.41135094264166838, -111.1807724695661506 ) ) ;
#5658=ORIENTED_EDGE ( 'NONE', *, *, #5137, .T. ) ;
#5660=ORIENTED_EDGE ( 'NONE', *, *, #35023, .F. ) ;
#5662=ORIENTED_EDGE ( 'NONE', *, *, #27991, .T. ) ;
#5664=CARTESIAN_POINT ( 'NONE',  ( -3.310556943750000425, 19.41135094264166128, -62.84743913623280775 ) ) ;
#5665=ORIENTED_EDGE ( 'NONE', *, *, #22507, .F. ) ;
#5667=DIRECTION ( 'NONE',  ( 0.000000000000000000, 1.000000000000000000, 0.000000000000000000 ) ) ;
#5668=EDGE_CURVE ( 'NONE', #31249, #5717, #11989, .T. ) ;
#5672=CARTESIAN_POINT ( 'NONE',  ( -1.394453263437886604E-15, 14.00000000000002132, -133.4047308033774186 ) ) ;
#5673=EDGE_CURVE ( 'NONE', #29038, #15095, #5784, .T. ) ;
#5677=CARTESIAN_POINT ( 'NONE',  ( -3.310556943750000425, 19.41135094264167549, -129.8474391362328220 ) ) ;
#5679=AXIS2_PLACEMENT_3D ( 'NONE', #8720, #33843, #17683 ) ;
#5680=CARTESIAN_POINT ( 'NONE',  ( -7.022189441860112050E-16, 13.67729811471671475, -38.60160580289946353 ) ) ;
#5681=CARTESIAN_POINT ( 'NONE',  ( 3.310556943750001313, 19.41135094264165772, -27.26827246956613138 ) ) ;
#5683=CARTESIAN_POINT ( 'NONE',  ( 1.655278471874998436, 14.63297358603754539, -93.51827246956612782 ) ) ;
#5684=CARTESIAN_POINT ( 'NONE',  ( 1.750000000000001110, 20.53108891324554719, -25.98806413671075788 ) ) ;
#5687=CARTESIAN_POINT ( 'NONE',  ( -3.310556943750001313, 17.50000000000002487, -137.8516058028994564 ) ) ;
#5688=CARTESIAN_POINT ( 'NONE',  ( -1.750000000000002220, 14.46891108675448301, -83.79431413575483134 ) ) ;
#5689=CARTESIAN_POINT ( 'NONE',  ( 3.500000000000001332, 19.52072594216371115, -87.07139747004409003 ) ) ;
#5691=CARTESIAN_POINT ( 'NONE',  ( 2.474675557024783212E-16, 21.54145188432739744, -79.90473080337741862 ) ) ;
#5692=CARTESIAN_POINT ( 'NONE',  ( -1.655278471875002211, 14.63297358603754361, -64.68493913623279923 ) ) ;
#5695=CARTESIAN_POINT ( 'NONE',  ( 3.500000000000001332, 19.52072594216370760, -47.37764746908818125 ) ) ;
#5698=CARTESIAN_POINT ( 'NONE',  ( -3.310556943750000425, 19.41135094264166838, -111.8474391362328220 ) ) ;
#5702=CARTESIAN_POINT ( 'NONE',  ( -7.424026671074350129E-16, 13.45854811567263987, -109.4047308033774044 ) ) ;
#5706=FACE_OUTER_BOUND ( 'NONE', #38885, .T. ) ;
#5707=CARTESIAN_POINT ( 'NONE',  ( 1.749999999999998224, 14.46891108675447768, -59.32139747004409713 ) ) ;
#5709=CARTESIAN_POINT ( 'NONE',  ( 1.655278471874998436, 14.63297358603754361, -72.43077246956613635 ) ) ;
#5711=CARTESIAN_POINT ( 'NONE',  ( 0.000000000000000000, 21.00000000000002487, -149.5231586289125687 ) ) ;
#5712=CYLINDRICAL_SURFACE ( 'NONE', #8768, 3.499999999999999556 ) ;
#5714=CARTESIAN_POINT ( 'NONE',  ( -1.655278471875002211, 14.63297358603753828, -23.59743913623281486 ) ) ;
#5715=CARTESIAN_POINT ( 'NONE',  ( -1.749999999999999778, 20.53108891324555785, -105.1276474690881741 ) ) ;
#5716=CARTESIAN_POINT ( 'NONE',  ( 3.310556943749999981, 15.58864905735836714, -77.34743913623279354 ) ) ;
#5717=VERTEX_POINT ( 'NONE', #5365 ) ;
#5723=VECTOR ( 'NONE', #33379, 1000.000000000000000 ) ;
#5725=CARTESIAN_POINT ( 'NONE',  ( 3.310556943750001313, 17.50000000000001421, -50.35160580289946353 ) ) ;
#5726=EDGE_CURVE ( 'NONE', #18793, #36671, #22056, .T. ) ;
#5727=CARTESIAN_POINT ( 'NONE',  ( -3.310556943750002645, 15.58864905735837780, -111.7682724695661420 ) ) ;
#5729=( BOUNDED_CURVE ( )  B_SPLINE_CURVE ( 2, ( #974, #24359, #7983, #30948, #26922, #20953, #40520, #1390, #40309 ),
 .UNSPECIFIED., .F., .F. ) 
 B_SPLINE_CURVE_WITH_KNOTS ( ( 3, 2, 2, 2, 3 ),
 ( 0.1979166666666666574, 0.1986111111111110994, 0.2000000000000000111, 0.2013888888888888951, 0.2020833333333333370 ),
 .UNSPECIFIED. ) 
 CURVE ( )  GEOMETRIC_REPRESENTATION_ITEM ( )  RATIONAL_B_SPLINE_CURVE ( ( 0.9330127018922194093, 0.9330127018922194093, 1.000000000000000000, 0.8660254037844387076, 1.000000000000000000, 0.8660254037844387076, 1.000000000000000000, 0.9330127018922194093, 0.9330127018922194093 ) ) 
 REPRESENTATION_ITEM ( '' )  );
#5730=CARTESIAN_POINT ( 'NONE',  ( -7.022189441860112050E-16, 13.67729811471671475, -34.51410580289947205 ) ) ;
#5732=CARTESIAN_POINT ( 'NONE',  ( 3.310556943750001313, 19.41135094264166128, -60.26827246956613493 ) ) ;
#5733=CARTESIAN_POINT ( 'NONE',  ( -7.424026671074350129E-16, 13.45854811567263809, -105.7109808024215170 ) ) ;
#5735=CARTESIAN_POINT ( 'NONE',  ( -3.310556943750002645, 15.58864905735837247, -89.68077246956615056 ) ) ;
#5736=CARTESIAN_POINT ( 'NONE',  ( -3.500000000000001332, 17.50000000000001776, -95.65473080337743284 ) ) ;
#5740=CARTESIAN_POINT ( 'NONE',  ( -3.500000000000000888, 19.52072594216370760, -58.04431413575483845 ) ) ;
#5742=CARTESIAN_POINT ( 'NONE',  ( 1.655278471874998436, 14.63297358603753651, -24.43077246956613990 ) ) ;
#5743=CARTESIAN_POINT ( 'NONE',  ( 3.500000000000000000, 15.47927405783632082, -48.23806413671076854 ) ) ;
#5745=CARTESIAN_POINT ( 'NONE',  ( 3.310556943750001313, 19.41135094264166838, -107.2682724695661278 ) ) ;
#5746=CARTESIAN_POINT ( 'NONE',  ( 1.655278471875001101, 20.36702641396248481, -30.18493913623279568 ) ) ;
#5752=CARTESIAN_POINT ( 'NONE',  ( -3.310556943750000425, 19.41135094264166838, -86.84743913623280775 ) ) ;
#5754=VERTEX_POINT ( 'NONE', #21539 ) ;
#5756=CARTESIAN_POINT ( 'NONE',  ( 3.500000000000000000, 15.47927405783633326, -109.5443141357548456 ) ) ;
#5761=CARTESIAN_POINT ( 'NONE',  ( -3.310556943750002645, 15.58864905735837425, -95.68077246956615056 ) ) ;
#5763=VERTEX_POINT ( 'NONE', #37911 ) ;
#5765=EDGE_LOOP ( 'NONE', ( #14046, #10106, #22180, #7654 ) ) ;
#5769=DIRECTION ( 'NONE',  ( -0.000000000000000000, 1.259100132267607459E-16, -1.000000000000000000 ) ) ;
#5772=ORIENTED_EDGE ( 'NONE', *, *, #20988, .F. ) ;
#5773=CARTESIAN_POINT ( 'NONE',  ( 3.500000000000001332, 17.50000000000002487, -135.1547308033774186 ) ) ;
#5775=CARTESIAN_POINT ( 'NONE',  ( -3.310556943750000425, 19.41135094264167549, -135.8474391362328220 ) ) ;
#5776=FACE_OUTER_BOUND ( 'NONE', #11072, .T. ) ;
#5780=CARTESIAN_POINT ( 'NONE',  ( -3.310556943750002645, 15.58864905735837780, -124.7682724695661136 ) ) ;
#5781=CARTESIAN_POINT ( 'NONE',  ( -7.022189441860112050E-16, 13.67729811471671653, -51.60160580289946353 ) ) ;
#5783=CARTESIAN_POINT ( 'NONE',  ( 1.749999999999998224, 14.46891108675448656, -134.3213974700441042 ) ) ;
#5784=( BOUNDED_CURVE ( )  B_SPLINE_CURVE ( 2, ( #21329, #8563, #8769, #5796, #15383, #11957, #21741, #15159, #38324 ),
 .UNSPECIFIED., .F., .T. ) 
 B_SPLINE_CURVE_WITH_KNOTS ( ( 3, 2, 2, 2, 3 ),
 ( 0.6770833333333333703, 0.6777777777777778123, 0.6791666666666666963, 0.6805555555555555802, 0.6812500000000000222 ),
 .UNSPECIFIED. ) 
 CURVE ( )  GEOMETRIC_REPRESENTATION_ITEM ( )  RATIONAL_B_SPLINE_CURVE ( ( 0.9330127018922194093, 0.9330127018922194093, 1.000000000000000000, 0.8660254037844387076, 1.000000000000000000, 0.8660254037844387076, 1.000000000000000000, 0.9330127018922194093, 0.9330127018922194093 ) ) 
 REPRESENTATION_ITEM ( '' )  );
#5786=( NAMED_UNIT ( * ) SI_UNIT ( $, .STERADIAN. ) SOLID_ANGLE_UNIT ( ) );
#5788=CARTESIAN_POINT ( 'NONE',  ( -3.310556943750001313, 17.50000000000001776, -79.85160580289945642 ) ) ;
#5789=CARTESIAN_POINT ( 'NONE',  ( 1.749999999999998224, 14.46891108675448656, -123.6276474690881741 ) ) ;
#5790=CARTESIAN_POINT ( 'NONE',  ( 3.310556943750001313, 19.41135094264166838, -107.1807724695661364 ) ) ;
#5791=CARTESIAN_POINT ( 'NONE',  ( 3.500000000000000000, 15.47927405783632793, -81.23806413671076143 ) ) ;
#5794=CARTESIAN_POINT ( 'NONE',  ( 3.500000000000000000, 15.47927405783632615, -82.54431413575483134 ) ) ;
#5796=CARTESIAN_POINT ( 'NONE',  ( -3.500000000000000000, 19.52072594216370760, -62.04431413575484555 ) ) ;
#5797=CARTESIAN_POINT ( 'NONE',  ( -1.655278471875002211, 14.63297358603754184, -42.59743913623280065 ) ) ;
#5798=CARTESIAN_POINT ( 'NONE',  ( 1.655278471874998436, 14.63297358603754716, -103.5182724695661278 ) ) ;
#5799=CARTESIAN_POINT ( 'NONE',  ( 1.750000000000001110, 20.53108891324555074, -67.98806413671076143 ) ) ;
#5800=CYLINDRICAL_SURFACE ( 'NONE', #40254, 3.499999999999999556 ) ;
#5802=CARTESIAN_POINT ( 'NONE',  ( 3.310556943750001313, 19.41135094264166838, -122.2682724695661278 ) ) ;
#5803=DIRECTION ( 'NONE',  ( 0.000000000000000000, 1.000000000000000000, 0.000000000000000000 ) ) ;
#5806=CARTESIAN_POINT ( 'NONE',  ( -3.500000000000002220, 15.47927405783632793, -71.57139747004409003 ) ) ;
#5809=ORIENTED_EDGE ( 'NONE', *, *, #118, .F. ) ;
#5810=CARTESIAN_POINT ( 'NONE',  ( 3.310556943750001313, 17.50000000000001776, -75.35160580289947063 ) ) ;
#5812=CARTESIAN_POINT ( 'NONE',  ( 1.749999999999998224, 14.46891108675447590, -45.32139747004409713 ) ) ;
#5817=CARTESIAN_POINT ( 'NONE',  ( 3.310556943750001313, 19.41135094264166128, -35.18077246956615056 ) ) ;
#5820=ORIENTED_EDGE ( 'NONE', *, *, #25915, .F. ) ;
#5822=CARTESIAN_POINT ( 'NONE',  ( -3.310556943750000425, 19.41135094264166128, -49.84743913623281486 ) ) ;
#5825=VERTEX_POINT ( 'NONE', #31727 ) ;
#5829=CARTESIAN_POINT ( 'NONE',  ( 4.648177544792955347E-16, 21.00000000000001776, -97.21098080242148853 ) ) ;
#5830=AXIS2_PLACEMENT_3D ( 'NONE', #1539, #11937, #24930 ) ;
#5832=CARTESIAN_POINT ( 'NONE',  ( -3.500000000000002220, 15.47927405783632082, -31.87764746908818125 ) ) ;
#5834=CARTESIAN_POINT ( 'NONE',  ( 1.749999999999998224, 14.46891108675448123, -82.62764746908818836 ) ) ;
#5837=CARTESIAN_POINT ( 'NONE',  ( -3.500000000000002220, 15.47927405783633503, -141.8776474690881741 ) ) ;
#5838=CARTESIAN_POINT ( 'NONE',  ( -7.460324959392693302E-14, 21.00000000000001776, -100.9047308033774186 ) ) ;
#5839=CARTESIAN_POINT ( 'NONE',  ( 3.310556943750001313, 19.41135094264166838, -122.1807724695661364 ) ) ;
#5842=EDGE_CURVE ( 'NONE', #24201, #1595, #31317, .T. ) ;
#5844=CARTESIAN_POINT ( 'NONE',  ( 1.655278471875001101, 20.36702641396249547, -116.1849391362327850 ) ) ;
#5845=EDGE_CURVE ( 'NONE', #19887, #14042, #20203, .T. ) ;
#5847=CARTESIAN_POINT ( 'NONE',  ( -1.750000000000002220, 14.46891108675447590, -39.48806413671076854 ) ) ;
#5848=CARTESIAN_POINT ( 'NONE',  ( 3.500000000000001332, 17.50000000000001776, -92.15473080337743284 ) ) ;
#5850=CARTESIAN_POINT ( 'NONE',  ( -7.022189441860112050E-16, 13.67729811471673074, -141.6016058028994564 ) ) ;
#5853=CARTESIAN_POINT ( 'NONE',  ( -3.310556943750000425, 19.41135094264166483, -46.93493913623279923 ) ) ;
#5855=CARTESIAN_POINT ( 'NONE',  ( -1.750000000000002220, 14.46891108675448656, -114.4880641367107614 ) ) ;
#5856=CARTESIAN_POINT ( 'NONE',  ( -1.655278471874999990, 20.36702641396248836, -70.01827246956612782 ) ) ;
#5859=CARTESIAN_POINT ( 'NONE',  ( -3.310556943750002201, 15.58864905735837247, -91.76827246956615625 ) ) ;
#5860=AXIS2_PLACEMENT_3D ( 'NONE', #40986, #22252, #12044 ) ;
#5862=CARTESIAN_POINT ( 'NONE',  ( -0.9378221735089310451, 14.00000000000002132, -107.7556390011600342 ) ) ;
#5864=CARTESIAN_POINT ( 'NONE',  ( 1.750000000000001110, 20.53108891324556140, -131.2943141357548598 ) ) ;
#5865=CARTESIAN_POINT ( 'NONE',  ( 1.655278471874998436, 14.63297358603754006, -51.43077246956613635 ) ) ;
#5867=CARTESIAN_POINT ( 'NONE',  ( 2.340729813953370519E-16, 21.32270188528331900, -110.0141058028994649 ) ) ;
#5874=CARTESIAN_POINT ( 'NONE',  ( 2.340729813953370519E-16, 21.32270188528330834, -65.01410580289947916 ) ) ;
#5877=CARTESIAN_POINT ( 'NONE',  ( -1.394453263437886604E-15, 14.00000000000002132, -126.7109808024214885 ) ) ;
#5882=VERTEX_POINT ( 'NONE', #34304 ) ;
#5884=CARTESIAN_POINT ( 'NONE',  ( 2.340729813953370519E-16, 21.32270188528331900, -123.0141058028994649 ) ) ;
#5886=CARTESIAN_POINT ( 'NONE',  ( 1.655278471874998436, 14.63297358603753828, -38.51827246956612782 ) ) ;
#5887=CARTESIAN_POINT ( 'NONE',  ( -3.310556943750002645, 15.58864905735836537, -27.76827246956613138 ) ) ;
#5888=CARTESIAN_POINT ( 'NONE',  ( 3.310556943750001313, 19.41135094264166483, -86.26827246956614204 ) ) ;
#5889=CARTESIAN_POINT ( 'NONE',  ( 3.310556943750001313, 17.50000000000002487, -138.2641058028994792 ) ) ;
#5893=CARTESIAN_POINT ( 'NONE',  ( 1.655278471875001101, 20.36702641396249902, -133.1849391362327992 ) ) ;
#5896=CARTESIAN_POINT ( 'NONE',  ( 3.500000000000001332, 19.52072594216371115, -95.07139747004409003 ) ) ;
#5897=CARTESIAN_POINT ( 'NONE',  ( -1.749999999999999778, 20.53108891324555429, -79.82139747004410424 ) ) ;
#5898=CARTESIAN_POINT ( 'NONE',  ( 3.310556943750001313, 17.50000000000001421, -63.35160580289946353 ) ) ;
#5900=LINE ( 'NONE', #31215, #23787 ) ;
#5901=CARTESIAN_POINT ( 'NONE',  ( -1.394453263437886604E-15, 14.00000000000001421, -58.40473080337741862 ) ) ;
#5902=CARTESIAN_POINT ( 'NONE',  ( 3.310556943750001313, 19.41135094264166483, -86.26827246956614204 ) ) ;
#5903=FACE_OUTER_BOUND ( 'NONE', #39138, .T. ) ;
#5904=CARTESIAN_POINT ( 'NONE',  ( 3.310556943749999981, 15.58864905735837247, -116.3474391362327935 ) ) ;
#5906=( BOUNDED_CURVE ( )  B_SPLINE_CURVE ( 2, ( #30525, #8391, #2011, #1808, #11578, #8605, #21370, #11381, #31151 ),
 .UNSPECIFIED., .F., .T. ) 
 B_SPLINE_CURVE_WITH_KNOTS ( ( 3, 2, 2, 2, 3 ),
 ( 0.6937499999999999778, 0.6944444444444444198, 0.6958333333333333037, 0.6972222222222221877, 0.6979166666666666297 ),
 .UNSPECIFIED. ) 
 CURVE ( )  GEOMETRIC_REPRESENTATION_ITEM ( )  RATIONAL_B_SPLINE_CURVE ( ( 0.9330127018922194093, 0.9330127018922194093, 1.000000000000000000, 0.8660254037844387076, 1.000000000000000000, 0.8660254037844387076, 1.000000000000000000, 0.9330127018922194093, 0.9330127018922194093 ) ) 
 REPRESENTATION_ITEM ( '' )  );
#5907=CARTESIAN_POINT ( 'NONE',  ( 4.648177544792955347E-16, 21.00000000000001421, -72.21098080242151696 ) ) ;
#5910=CARTESIAN_POINT ( 'NONE',  ( 3.500000000000000000, 15.47927405783632970, -110.2380641367107614 ) ) ;
#5911=CARTESIAN_POINT ( 'NONE',  ( -3.500000000000001332, 17.50000000000001066, -28.65473080337743639 ) ) ;
#5912=( BOUNDED_CURVE ( )  B_SPLINE_CURVE ( 2, ( #25206, #9029, #18816, #2231, #24371, #15427, #34558, #37341, #8194 ),
 .UNSPECIFIED., .F., .F. ) 
 B_SPLINE_CURVE_WITH_KNOTS ( ( 3, 2, 2, 2, 3 ),
 ( 0.7270833333333333037, 0.7277777777777777457, 0.7291666666666666297, 0.7305555555555555136, 0.7312499999999999556 ),
 .UNSPECIFIED. ) 
 CURVE ( )  GEOMETRIC_REPRESENTATION_ITEM ( )  RATIONAL_B_SPLINE_CURVE ( ( 0.9330127018922194093, 0.9330127018922194093, 1.000000000000000000, 0.8660254037844387076, 1.000000000000000000, 0.8660254037844387076, 1.000000000000000000, 0.9330127018922194093, 0.9330127018922194093 ) ) 
 REPRESENTATION_ITEM ( '' )  );
#5914=CARTESIAN_POINT ( 'NONE',  ( -1.750000000000002220, 14.46891108675448123, -67.79431413575484555 ) ) ;
#5915=CARTESIAN_POINT ( 'NONE',  ( -1.750000000000002220, 14.46891108675447590, -26.79431413575483845 ) ) ;
#5918=CARTESIAN_POINT ( 'NONE',  ( 3.310556943750001313, 17.50000000000001421, -65.26410580289946495 ) ) ;
#5919=CARTESIAN_POINT ( 'NONE',  ( 4.286263797015737581E-16, 14.00000000000002487, -149.5231586289125687 ) ) ;
#5922=CARTESIAN_POINT ( 'NONE',  ( -7.022189441860112050E-16, 13.67729811471671297, -25.51410580289947205 ) ) ;
#5924=CARTESIAN_POINT ( 'NONE',  ( 2.340729813953370519E-16, 21.32270188528331190, -78.01410580289946495 ) ) ;
#5926=VERTEX_POINT ( 'NONE', #22791 ) ;
#5927=CARTESIAN_POINT ( 'NONE',  ( 4.648177544792955347E-16, 21.00000000000001421, -48.90473080337742573 ) ) ;
#5932=CARTESIAN_POINT ( 'NONE',  ( 2.340729813953370519E-16, 21.32270188528330479, -41.10160580289946353 ) ) ;
#5933=CARTESIAN_POINT ( 'NONE',  ( 1.655278471874998436, 14.63297358603754716, -107.5182724695661278 ) ) ;
#5934=EDGE_LOOP ( 'NONE', ( #28555, #24447, #28056, #11886 ) ) ;
#5935=CARTESIAN_POINT ( 'NONE',  ( -7.022189441860112050E-16, 13.67729811471671475, -28.51410580289948271 ) ) ;
#5936=CARTESIAN_POINT ( 'NONE',  ( 1.655278471875001101, 20.36702641396248836, -63.18493913623279923 ) ) ;
#5937=CARTESIAN_POINT ( 'NONE',  ( 1.750000000000001110, 20.53108891324555785, -109.2943141357548456 ) ) ;
#5939=CARTESIAN_POINT ( 'NONE',  ( 1.750000000000001110, 20.53108891324555429, -94.98806413671076143 ) ) ;
#5943=CARTESIAN_POINT ( 'NONE',  ( 1.750000000000001110, 20.53108891324555074, -57.29431413575483845 ) ) ;
#5945=CARTESIAN_POINT ( 'NONE',  ( 3.310556943750001313, 17.50000000000001066, -29.26410580289948271 ) ) ;
#5946=CARTESIAN_POINT ( 'NONE',  ( 1.749999999999998224, 14.46891108675447590, -47.32139747004410424 ) ) ;
#5948=CARTESIAN_POINT ( 'NONE',  ( -3.310556943750000425, 19.41135094264166838, -100.9349391362328134 ) ) ;
#5950=CARTESIAN_POINT ( 'NONE',  ( 1.655278471875001101, 20.36702641396248481, -32.18493913623279923 ) ) ;
#5953=CARTESIAN_POINT ( 'NONE',  ( -3.500000000000002220, 15.47927405783633503, -141.8776474690881741 ) ) ;
#5957=CARTESIAN_POINT ( 'NONE',  ( -7.022189441860112050E-16, 13.67729811471672363, -83.51410580289947916 ) ) ;
#5958=VERTEX_POINT ( 'NONE', #28741 ) ;
#5960=VERTEX_POINT ( 'NONE', #41949 ) ;
#5966=CARTESIAN_POINT ( 'NONE',  ( 3.310556943750001313, 17.50000000000001776, -93.26410580289947916 ) ) ;
#5969=CARTESIAN_POINT ( 'NONE',  ( 1.749999999999998224, 14.46891108675448478, -121.3213974700441042 ) ) ;
#5971=CARTESIAN_POINT ( 'NONE',  ( 4.648177544792955347E-16, 21.00000000000001066, -29.90473080337743639 ) ) ;
#5974=CARTESIAN_POINT ( 'NONE',  ( -3.500000000000001332, 17.50000000000001776, -84.65473080337743284 ) ) ;
#5978=( BOUNDED_CURVE ( )  B_SPLINE_CURVE ( 2, ( #32196, #3060, #12839, #38787, #33876, #39616, #27295, #29836, #36434 ),
 .UNSPECIFIED., .F., .F. ) 
 B_SPLINE_CURVE_WITH_KNOTS ( ( 3, 2, 2, 2, 3 ),
 ( 0.8187499999999999778, 0.8194444444444444198, 0.8208333333333333037, 0.8222222222222221877, 0.8229166666666666297 ),
 .UNSPECIFIED. ) 
 CURVE ( )  GEOMETRIC_REPRESENTATION_ITEM ( )  RATIONAL_B_SPLINE_CURVE ( ( 0.9330127018922194093, 0.9330127018922194093, 1.000000000000000000, 0.8660254037844387076, 1.000000000000000000, 0.8660254037844387076, 1.000000000000000000, 0.9330127018922194093, 0.9330127018922194093 ) ) 
 REPRESENTATION_ITEM ( '' )  );
#5980=CARTESIAN_POINT ( 'NONE',  ( 4.286263797015737581E-16, 14.00000000000002487, -149.5231586289125687 ) ) ;
#5981=CARTESIAN_POINT ( 'NONE',  ( 0.000000000000000000, 17.50000000000002487, -149.5231586289125687 ) ) ;
#5982=CARTESIAN_POINT ( 'NONE',  ( -3.310556943750000425, 19.41135094264166838, -128.8474391362327935 ) ) ;
#5983=DIRECTION ( 'NONE',  ( -0.000000000000000000, 1.259100132267607459E-16, -1.000000000000000000 ) ) ;
#5985=CARTESIAN_POINT ( 'NONE',  ( 4.648177544792955347E-16, 21.00000000000001066, -28.21098080242150985 ) ) ;
#5986=CARTESIAN_POINT ( 'NONE',  ( -3.310556943750001313, 17.50000000000002132, -126.8516058028994422 ) ) ;
#5987=CARTESIAN_POINT ( 'NONE',  ( -3.310556943750001313, 17.50000000000001421, -52.85160580289946353 ) ) ;
#5988=ORIENTED_EDGE ( 'NONE', *, *, #25876, .T. ) ;
#5989=CARTESIAN_POINT ( 'NONE',  ( 3.500000000000000000, 15.47927405783633503, -132.2380641367107614 ) ) ;
#5991=CARTESIAN_POINT ( 'NONE',  ( 3.310556943750001313, 17.50000000000001776, -76.35160580289945642 ) ) ;
#5992=CARTESIAN_POINT ( 'NONE',  ( 1.750000000000001110, 20.53108891324555785, -124.2943141357548456 ) ) ;
#5993=CARTESIAN_POINT ( 'NONE',  ( -3.310556943750002645, 15.58864905735837425, -105.6807724695661364 ) ) ;
#5994=CARTESIAN_POINT ( 'NONE',  ( 3.310556943749999981, 15.58864905735836004, -23.43493913623280633 ) ) ;
#5997=CARTESIAN_POINT ( 'NONE',  ( -3.500000000000002220, 15.47927405783632615, -76.87764746908817415 ) ) ;
#5998=CARTESIAN_POINT ( 'NONE',  ( -7.022189441860112050E-16, 13.67729811471671653, -41.51410580289947916 ) ) ;
#5999=CARTESIAN_POINT ( 'NONE',  ( 3.310556943749999981, 15.58864905735837070, -102.4349391362328134 ) ) ;
#6001=CARTESIAN_POINT ( 'NONE',  ( 1.749999999999998224, 14.46891108675447768, -65.32139747004410424 ) ) ;
#6003=ORIENTED_EDGE ( 'NONE', *, *, #34811, .F. ) ;
#6004=CARTESIAN_POINT ( 'NONE',  ( 2.340729813953370519E-16, 21.32270188528331900, -122.1016058028994564 ) ) ;
#6008=CARTESIAN_POINT ( 'NONE',  ( -1.394453263437886604E-15, 14.00000000000001421, -79.71098080242148853 ) ) ;
#6014=CARTESIAN_POINT ( 'NONE',  ( 1.655278471875001101, 20.36702641396248836, -73.18493913623279923 ) ) ;
#6015=LINE ( 'NONE', #28557, #25115 ) ;
#6019=EDGE_CURVE ( 'NONE', #14042, #34385, #33489, .T. ) ;
#6021=CARTESIAN_POINT ( 'NONE',  ( 3.310556943750001313, 17.50000000000001066, -34.26410580289947205 ) ) ;
#6022=CARTESIAN_POINT ( 'NONE',  ( -1.394453263437886604E-15, 14.00000000000001421, -72.40473080337743284 ) ) ;
#6024=ORIENTED_EDGE ( 'NONE', *, *, #4578, .F. ) ;
#6026=DIRECTION ( 'NONE',  ( 0.000000000000000000, 1.000000000000000000, 0.000000000000000000 ) ) ;
#6027=ORIENTED_EDGE ( 'NONE', *, *, #17543, .F. ) ;
#6029=( BOUNDED_CURVE ( )  B_SPLINE_CURVE ( 2, ( #33090, #6728, #26309, #29263, #38853, #26100, #9942, #20128, #16937 ),
 .UNSPECIFIED., .F., .T. ) 
 B_SPLINE_CURVE_WITH_KNOTS ( ( 3, 2, 2, 2, 3 ),
 ( 0.2645833333333333370, 0.2652777777777777790, 0.2666666666666666630, 0.2680555555555555469, 0.2687499999999999889 ),
 .UNSPECIFIED. ) 
 CURVE ( )  GEOMETRIC_REPRESENTATION_ITEM ( )  RATIONAL_B_SPLINE_CURVE ( ( 0.9330127018922194093, 0.9330127018922194093, 1.000000000000000000, 0.8660254037844387076, 1.000000000000000000, 0.8660254037844387076, 1.000000000000000000, 0.9330127018922194093, 0.9330127018922194093 ) ) 
 REPRESENTATION_ITEM ( '' )  );
#6033=CARTESIAN_POINT ( 'NONE',  ( -3.500000000000001332, 17.50000000000002132, -117.6547308033774328 ) ) ;
#6034=CARTESIAN_POINT ( 'NONE',  ( -1.749999999999999778, 20.53108891324554719, -34.12764746908818125 ) ) ;
#6035=CARTESIAN_POINT ( 'NONE',  ( -7.424026671074350129E-16, 13.45854811567263098, -31.71098080242150274 ) ) ;
#6036=CARTESIAN_POINT ( 'NONE',  ( -3.500000000000002220, 15.47927405783632615, -65.87764746908817415 ) ) ;
#6037=FACE_OUTER_BOUND ( 'NONE', #40911, .T. ) ;
#6039=CARTESIAN_POINT ( 'NONE',  ( 3.500000000000001332, 19.52072594216370405, -37.07139747004409003 ) ) ;
#6041=CARTESIAN_POINT ( 'NONE',  ( -3.500000000000002220, 15.47927405783633503, -136.8776474690881741 ) ) ;
#6043=CARTESIAN_POINT ( 'NONE',  ( 3.310556943749999981, 15.58864905735837425, -124.3474391362328078 ) ) ;
#6047=CARTESIAN_POINT ( 'NONE',  ( 3.500000000000000000, 15.47927405783632615, -92.54431413575483134 ) ) ;
#6048=CARTESIAN_POINT ( 'NONE',  ( -1.655278471874999990, 20.36702641396249547, -120.0182724695661278 ) ) ;
#6050=CARTESIAN_POINT ( 'NONE',  ( -1.749999999999999778, 20.53108891324554719, -34.82139747004410424 ) ) ;
#6051=DIRECTION ( 'NONE',  ( 0.000000000000000000, 1.000000000000000000, 0.000000000000000000 ) ) ;
#6053=CARTESIAN_POINT ( 'NONE',  ( 2.340729813953370519E-16, 21.32270188528332255, -141.1016058028994564 ) ) ;
#6055=CARTESIAN_POINT ( 'NONE',  ( 1.749999999999998224, 14.46891108675448834, -138.3213974700441042 ) ) ;
#6056=CARTESIAN_POINT ( 'NONE',  ( -3.310556943750000425, 19.41135094264166483, -47.93493913623279212 ) ) ;
#6058=CARTESIAN_POINT ( 'NONE',  ( -3.500000000000000000, 19.52072594216370760, -73.04431413575483134 ) ) ;
#6059=CARTESIAN_POINT ( 'NONE',  ( 3.310556943750001313, 19.41135094264166128, -69.26827246956612782 ) ) ;
#6061=CARTESIAN_POINT ( 'NONE',  ( -3.310556943750001313, 17.50000000000001421, -67.76410580289947916 ) ) ;
#6062=ORIENTED_EDGE ( 'NONE', *, *, #24315, .F. ) ;
#6063=CARTESIAN_POINT ( 'NONE',  ( -3.310556943750000425, 19.41135094264166838, -91.93493913623281344 ) ) ;
#6065=CARTESIAN_POINT ( 'NONE',  ( 4.648177544792955347E-16, 21.00000000000001421, -49.21098080242150274 ) ) ;
#6066=LINE ( 'NONE', #25438, #13876 ) ;
#6067=DIRECTION ( 'NONE',  ( -0.000000000000000000, 1.259100132267607459E-16, -1.000000000000000000 ) ) ;
#6068=CARTESIAN_POINT ( 'NONE',  ( -3.310556943750002201, 15.58864905735836714, -51.68077246956612925 ) ) ;
#6070=CARTESIAN_POINT ( 'NONE',  ( -3.310556943750000425, 19.41135094264166838, -106.8474391362327935 ) ) ;
#6071=CARTESIAN_POINT ( 'NONE',  ( -0.9378221735089310451, 14.00000000000001066, -35.75563900116002714 ) ) ;
#6072=ORIENTED_EDGE ( 'NONE', *, *, #1510, .F. ) ;
#6076=CARTESIAN_POINT ( 'NONE',  ( -3.310556943750000425, 19.41135094264166128, -57.84743913623280065 ) ) ;
#6077=ORIENTED_EDGE ( 'NONE', *, *, #36386, .T. ) ;
#6080=CARTESIAN_POINT ( 'NONE',  ( 0.9378221735089300459, 21.00000000000001066, -30.25563900116003069 ) ) ;
#6081=DIRECTION ( 'NONE',  ( -0.000000000000000000, 1.259100132267607459E-16, -1.000000000000000000 ) ) ;
#6084=LINE ( 'NONE', #15038, #37387 ) ;
#6086=CARTESIAN_POINT ( 'NONE',  ( 4.648177544792955347E-16, 21.00000000000001776, -99.90473080337743284 ) ) ;
#6087=CARTESIAN_POINT ( 'NONE',  ( -1.655278471874999990, 20.36702641396249547, -126.9307724695661364 ) ) ;
#6090=CARTESIAN_POINT ( 'NONE',  ( 1.655278471874998436, 14.63297358603753828, -34.51827246956614204 ) ) ;
#6091=CARTESIAN_POINT ( 'NONE',  ( 1.655278471874998436, 14.63297358603753828, -29.51827246956613493 ) ) ;
#6092=CARTESIAN_POINT ( 'NONE',  ( 1.655278471874998436, 14.63297358603754539, -86.51827246956612782 ) ) ;
#6093=CARTESIAN_POINT ( 'NONE',  ( -1.655278471875002211, 14.63297358603755427, -140.5974391362327935 ) ) ;
#6096=CARTESIAN_POINT ( 'NONE',  ( -7.022189441860112050E-16, 13.67729811471672718, -131.6016058028994564 ) ) ;
#6100=DIRECTION ( 'NONE',  ( 0.000000000000000000, 1.000000000000000000, 0.000000000000000000 ) ) ;
#6101=CARTESIAN_POINT ( 'NONE',  ( -1.750000000000002220, 14.46891108675448301, -82.48806413671074722 ) ) ;
#6103=CARTESIAN_POINT ( 'NONE',  ( -7.022189441860112050E-16, 13.67729811471672186, -64.60160580289945642 ) ) ;
#6106=CARTESIAN_POINT ( 'NONE',  ( 0.9378221735089300459, 21.00000000000001421, -47.25563900116002714 ) ) ;
#6107=CARTESIAN_POINT ( 'NONE',  ( -7.022189441860112050E-16, 13.67729811471672363, -87.60160580289947063 ) ) ;
#6109=CARTESIAN_POINT ( 'NONE',  ( -7.022189441860112050E-16, 13.67729811471672896, -112.5141058028994792 ) ) ;
#6110=DIRECTION ( 'NONE',  ( -0.000000000000000000, 1.259100132267607459E-16, -1.000000000000000000 ) ) ;
#6112=ORIENTED_EDGE ( 'NONE', *, *, #31825, .F. ) ;
#6113=AXIS2_PLACEMENT_3D ( 'NONE', #10190, #3588, #32519 ) ;
#6115=CARTESIAN_POINT ( 'NONE',  ( 3.500000000000001332, 17.50000000000002132, -107.1547308033774186 ) ) ;
#6122=CARTESIAN_POINT ( 'NONE',  ( -3.310556943750000425, 19.41135094264166483, -64.84743913623280775 ) ) ;
#6124=CARTESIAN_POINT ( 'NONE',  ( -1.655278471875002211, 14.63297358603755072, -119.5974391362328078 ) ) ;
#6130=CARTESIAN_POINT ( 'NONE',  ( -3.310556943750000425, 19.41135094264166483, -76.84743913623280775 ) ) ;
#6135=CARTESIAN_POINT ( 'NONE',  ( -0.9378221735089310451, 14.00000000000001066, -48.44938900211594301 ) ) ;
#6136=EDGE_CURVE ( 'NONE', #2470, #18307, #37834, .T. ) ;
#6137=CARTESIAN_POINT ( 'NONE',  ( 3.310556943750001313, 17.50000000000002487, -142.2641058028994792 ) ) ;
#6141=CARTESIAN_POINT ( 'NONE',  ( -1.655278471875002211, 14.63297358603754184, -41.68493913623279212 ) ) ;
#6142=CARTESIAN_POINT ( 'NONE',  ( 3.310556943749999981, 15.58864905735837070, -104.4349391362328134 ) ) ;
#6144=( BOUNDED_CURVE ( )  B_SPLINE_CURVE ( 2, ( #34747, #27948, #15191, #2422, #9223, #34956, #5617, #15410, #5196 ),
 .UNSPECIFIED., .F., .F. ) 
 B_SPLINE_CURVE_WITH_KNOTS ( ( 3, 2, 2, 2, 3 ),
 ( 0.7229166666666666519, 0.7236111111111110938, 0.7249999999999999778, 0.7263888888888888618, 0.7270833333333333037 ),
 .UNSPECIFIED. ) 
 CURVE ( )  GEOMETRIC_REPRESENTATION_ITEM ( )  RATIONAL_B_SPLINE_CURVE ( ( 0.9330127018922194093, 0.9330127018922194093, 1.000000000000000000, 0.8660254037844387076, 1.000000000000000000, 0.8660254037844387076, 1.000000000000000000, 0.9330127018922194093, 0.9330127018922194093 ) ) 
 REPRESENTATION_ITEM ( '' )  );
#6145=CARTESIAN_POINT ( 'NONE',  ( -1.655278471875002211, 14.63297358603754006, -30.59743913623280775 ) ) ;
#6146=CARTESIAN_POINT ( 'NONE',  ( 2.340729813953370519E-16, 21.32270188528330834, -62.10160580289945642 ) ) ;
#6147=CARTESIAN_POINT ( 'NONE',  ( 3.500000000000000000, 15.47927405783632793, -104.5443141357548456 ) ) ;
#6150=CARTESIAN_POINT ( 'NONE',  ( -3.500000000000001332, 17.50000000000001776, -97.65473080337743284 ) ) ;
#6151=ADVANCED_FACE ( 'NONE', ( #22993 ), #38957, .T. ) ;
#6152=CARTESIAN_POINT ( 'NONE',  ( 0.9378221735089281585, 14.00000000000001243, -63.66632260368299256 ) ) ;
#6155=CARTESIAN_POINT ( 'NONE',  ( -3.500000000000000888, 19.52072594216370760, -60.04431413575484555 ) ) ;
#6157=CARTESIAN_POINT ( 'NONE',  ( -0.9378221735089291577, 21.00000000000001421, -47.16632260368299967 ) ) ;
#6158=CARTESIAN_POINT ( 'NONE',  ( -3.310556943750002645, 15.58864905735836182, -25.68077246956613990 ) ) ;
#6160=CARTESIAN_POINT ( 'NONE',  ( -3.500000000000002220, 15.47927405783632260, -48.57139747004411134 ) ) ;
#6162=CARTESIAN_POINT ( 'NONE',  ( 3.310556943750001313, 19.41135094264166128, -33.26827246956613493 ) ) ;
#6165=CARTESIAN_POINT ( 'NONE',  ( 0.000000000000000000, 17.50000000000002487, -149.5231586289125687 ) ) ;
#6169=CARTESIAN_POINT ( 'NONE',  ( -1.655278471875002211, 14.63297358603754716, -83.59743913623279354 ) ) ;
#6172=CARTESIAN_POINT ( 'NONE',  ( -1.394453263437886604E-15, 14.00000000000001066, -35.40473080337743284 ) ) ;
#6178=CARTESIAN_POINT ( 'NONE',  ( 3.310556943750001313, 19.41135094264166483, -96.18077246956612214 ) ) ;
#6181=CARTESIAN_POINT ( 'NONE',  ( 4.648177544792955347E-16, 21.00000000000002132, -120.9047308033774328 ) ) ;
#6182=ORIENTED_EDGE ( 'NONE', *, *, #30841, .F. ) ;
#6184=CARTESIAN_POINT ( 'NONE',  ( -1.750000000000002220, 14.46891108675448301, -84.48806413671076143 ) ) ;
#6188=DIRECTION ( 'NONE',  ( 0.000000000000000000, 1.000000000000000000, 0.000000000000000000 ) ) ;
#6189=CARTESIAN_POINT ( 'NONE',  ( 0.000000000000000000, 17.50000000000002487, -149.5231586289125687 ) ) ;
#6190=EDGE_CURVE ( 'NONE', #33770, #11167, #4428, .T. ) ;
#6191=CARTESIAN_POINT ( 'NONE',  ( -1.655278471874999990, 20.36702641396249902, -131.9307724695661364 ) ) ;
#6192=LINE ( 'NONE', #32920, #29137 ) ;
#6194=ORIENTED_EDGE ( 'NONE', *, *, #20044, .F. ) ;
#6195=CARTESIAN_POINT ( 'NONE',  ( 2.340729813953370519E-16, 21.32270188528331900, -120.1016058028994706 ) ) ;
#6196=CARTESIAN_POINT ( 'NONE',  ( -1.655278471874999990, 20.36702641396248836, -50.01827246956614204 ) ) ;
#6197=ORIENTED_EDGE ( 'NONE', *, *, #7143, .T. ) ;
#6198=CARTESIAN_POINT ( 'NONE',  ( 1.750000000000001110, 20.53108891324555785, -128.9880641367107614 ) ) ;
#6201=CARTESIAN_POINT ( 'NONE',  ( -1.655278471874999990, 20.36702641396249192, -78.01827246956614204 ) ) ;
#6202=CARTESIAN_POINT ( 'NONE',  ( 1.749999999999998224, 14.46891108675448478, -122.6276474690881741 ) ) ;
#6203=CARTESIAN_POINT ( 'NONE',  ( 3.310556943750001313, 17.50000000000002132, -105.2641058028994649 ) ) ;
#6204=EDGE_CURVE ( 'NONE', #24826, #13587, #24070, .T. ) ;
#6208=CARTESIAN_POINT ( 'NONE',  ( -3.500000000000000888, 19.52072594216371115, -76.04431413575483134 ) ) ;
#6210=CARTESIAN_POINT ( 'NONE',  ( 3.310556943750001313, 19.41135094264165772, -41.18077246956613635 ) ) ;
#6211=CARTESIAN_POINT ( 'NONE',  ( -3.310556943750001313, 17.50000000000002132, -102.8516058028994564 ) ) ;
#6212=CARTESIAN_POINT ( 'NONE',  ( -1.394453263437886604E-15, 14.00000000000001776, -82.71098080242150274 ) ) ;
#6213=CARTESIAN_POINT ( 'NONE',  ( -1.749999999999999778, 20.53108891324555074, -63.82139747004410424 ) ) ;
#6215=ORIENTED_EDGE ( 'NONE', *, *, #20376, .F. ) ;
#6216=CARTESIAN_POINT ( 'NONE',  ( 3.310556943750001313, 17.50000000000002132, -117.3516058028994706 ) ) ;
#6217=CARTESIAN_POINT ( 'NONE',  ( -1.749999999999999778, 20.53108891324556140, -136.8213974700441042 ) ) ;
#6222=CARTESIAN_POINT ( 'NONE',  ( -1.394453263437886604E-15, 14.00000000000002132, -120.4047308033774328 ) ) ;
#6224=ORIENTED_EDGE ( 'NONE', *, *, #22812, .T. ) ;
#6226=CARTESIAN_POINT ( 'NONE',  ( -1.394453263437886604E-15, 14.00000000000001066, -45.40473080337742573 ) ) ;
#6230=CARTESIAN_POINT ( 'NONE',  ( -7.022189441860112050E-16, 13.67729811471671653, -34.51410580289947205 ) ) ;
#6231=( BOUNDED_CURVE ( )  B_SPLINE_CURVE ( 2, ( #10908, #23894, #4730, #36862, #7506, #7722, #20694, #27288, #11123 ),
 .UNSPECIFIED., .F., .F. ) 
 B_SPLINE_CURVE_WITH_KNOTS ( ( 3, 2, 2, 2, 3 ),
 ( 0.2729166666666666963, 0.2736111111111111382, 0.2750000000000000222, 0.2763888888888889062, 0.2770833333333333481 ),
 .UNSPECIFIED. ) 
 CURVE ( )  GEOMETRIC_REPRESENTATION_ITEM ( )  RATIONAL_B_SPLINE_CURVE ( ( 0.9330127018922194093, 0.9330127018922220739, 1.000000000000000000, 0.8660254037844387076, 1.000000000000000000, 0.8660254037844387076, 1.000000000000000000, 0.9330127018922194093, 0.9330127018922194093 ) ) 
 REPRESENTATION_ITEM ( '' )  );
#6232=CARTESIAN_POINT ( 'NONE',  ( 3.500000000000001332, 17.50000000000001421, -72.15473080337743284 ) ) ;
#6233=AXIS2_PLACEMENT_3D ( 'NONE', #29061, #12910, #32047 ) ;
#6235=ORIENTED_EDGE ( 'NONE', *, *, #2258, .F. ) ;
#6238=CARTESIAN_POINT ( 'NONE',  ( 0.000000000000000000, 17.50000000000002487, -149.5231586289125687 ) ) ;
#6239=ORIENTED_EDGE ( 'NONE', *, *, #36981, .F. ) ;
#6241=CARTESIAN_POINT ( 'NONE',  ( -3.500000000000002220, 15.47927405783633503, -114.8776474690881741 ) ) ;
#6243=DIRECTION ( 'NONE',  ( -0.000000000000000000, 1.259100132267607459E-16, -1.000000000000000000 ) ) ;
#6244=CARTESIAN_POINT ( 'NONE',  ( -1.749999999999999778, 20.53108891324555785, -119.8213974700440900 ) ) ;
#6246=CARTESIAN_POINT ( 'NONE',  ( 1.749999999999998224, 14.46891108675447413, -34.62764746908818125 ) ) ;
#6248=CARTESIAN_POINT ( 'NONE',  ( 3.500000000000000000, 15.47927405783632082, -35.54431413575484555 ) ) ;
#6252=CARTESIAN_POINT ( 'NONE',  ( -3.500000000000001332, 17.50000000000002487, -140.9609808024215170 ) ) ;
#6253=CARTESIAN_POINT ( 'NONE',  ( 4.648177544792955347E-16, 21.00000000000002132, -120.2109808024215170 ) ) ;
#6254=CARTESIAN_POINT ( 'NONE',  ( 3.310556943750001313, 17.50000000000002132, -123.2641058028994649 ) ) ;
#6255=ADVANCED_FACE ( 'NONE', ( #17042 ), #7259, .T. ) ;
#6259=CARTESIAN_POINT ( 'NONE',  ( 1.749999999999998224, 14.46891108675448123, -89.62764746908817415 ) ) ;
#6262=CARTESIAN_POINT ( 'NONE',  ( -3.310556943750002645, 15.58864905735836892, -56.68077246956614346 ) ) ;
#6263=CARTESIAN_POINT ( 'NONE',  ( 3.310556943750001313, 19.41135094264166838, -118.2682724695661278 ) ) ;
#6265=CARTESIAN_POINT ( 'NONE',  ( -1.749999999999999778, 20.53108891324554719, -31.82139747004410069 ) ) ;
#6266=CARTESIAN_POINT ( 'NONE',  ( -3.500000000000000000, 19.52072594216371826, -109.0443141357548456 ) ) ;
#6268=CARTESIAN_POINT ( 'NONE',  ( 3.310556943750001313, 17.50000000000002487, -135.3516058028994564 ) ) ;
#6271=CARTESIAN_POINT ( 'NONE',  ( 3.310556943750001313, 17.50000000000001066, -42.35160580289947063 ) ) ;
#6272=DIRECTION ( 'NONE',  ( 0.000000000000000000, 1.000000000000000000, 0.000000000000000000 ) ) ;
#6273=CARTESIAN_POINT ( 'NONE',  ( 3.310556943749999981, 15.58864905735836537, -67.43493913623279923 ) ) ;
#6274=CARTESIAN_POINT ( 'NONE',  ( 3.310556943749999981, 15.58864905735836537, -64.34743913623280775 ) ) ;
#6275=VERTEX_POINT ( 'NONE', #39575 ) ;
#6276=CARTESIAN_POINT ( 'NONE',  ( -1.655278471875002211, 14.63297358603754716, -92.68493913623279923 ) ) ;
#6278=LINE ( 'NONE', #25852, #15676 ) ;
#6281=CARTESIAN_POINT ( 'NONE',  ( -1.750000000000002220, 14.46891108675448123, -69.79431413575484555 ) ) ;
#6282=CARTESIAN_POINT ( 'NONE',  ( 1.655278471874998436, 14.63297358603754006, -52.43077246956613635 ) ) ;
#6284=CARTESIAN_POINT ( 'NONE',  ( -3.310556943750001313, 17.50000000000002132, -106.7641058028994649 ) ) ;
#6285=( BOUNDED_CURVE ( )  B_SPLINE_CURVE ( 2, ( #36139, #32954, #3400, #15755, #12978, #25958, #9367, #19771, #38924 ),
 .UNSPECIFIED., .F., .T. ) 
 B_SPLINE_CURVE_WITH_KNOTS ( ( 3, 2, 2, 2, 3 ),
 ( 0.1604166666666666796, 0.1611111111111111216, 0.1625000000000000056, 0.1638888888888888895, 0.1645833333333333315 ),
 .UNSPECIFIED. ) 
 CURVE ( )  GEOMETRIC_REPRESENTATION_ITEM ( )  RATIONAL_B_SPLINE_CURVE ( ( 0.9330127018922194093, 0.9330127018922207416, 1.000000000000000000, 0.8660254037844387076, 1.000000000000000000, 0.8660254037844387076, 1.000000000000000000, 0.9330127018922194093, 0.9330127018922194093 ) ) 
 REPRESENTATION_ITEM ( '' )  );
#6290=CARTESIAN_POINT ( 'NONE',  ( -7.022189441860112050E-16, 13.67729811471671830, -57.51410580289947916 ) ) ;
#6294=CARTESIAN_POINT ( 'NONE',  ( 3.500000000000000000, 15.47927405783632437, -55.54431413575484555 ) ) ;
#6296=VERTEX_POINT ( 'NONE', #36392 ) ;
#6297=CARTESIAN_POINT ( 'NONE',  ( 3.500000000000001332, 17.50000000000001066, -35.15473080337742573 ) ) ;
#6298=CARTESIAN_POINT ( 'NONE',  ( 3.310556943750001313, 19.41135094264166838, -123.1807724695661506 ) ) ;
#6299=CARTESIAN_POINT ( 'NONE',  ( 3.500000000000001332, 19.52072594216371115, -94.37764746908817415 ) ) ;
#6300=VECTOR ( 'NONE', #17932, 1000.000000000000000 ) ;
#6302=CARTESIAN_POINT ( 'NONE',  ( -3.310556943750001313, 17.50000000000001066, -36.85160580289946353 ) ) ;
#6303=CARTESIAN_POINT ( 'NONE',  ( 3.310556943750001313, 17.50000000000001066, -29.35160580289947063 ) ) ;
#6304=CARTESIAN_POINT ( 'NONE',  ( -3.310556943750000425, 19.41135094264166483, -87.93493913623279923 ) ) ;
#6305=CARTESIAN_POINT ( 'NONE',  ( 3.310556943750001313, 17.50000000000002487, -139.2641058028994792 ) ) ;
#6307=CARTESIAN_POINT ( 'NONE',  ( 1.750000000000001110, 20.53108891324555074, -48.98806413671076854 ) ) ;
#6309=CARTESIAN_POINT ( 'NONE',  ( 1.750000000000001110, 20.53108891324555785, -113.9880641367107472 ) ) ;
#6311=CARTESIAN_POINT ( 'NONE',  ( -3.310556943750002645, 15.58864905735837780, -135.7682724695661136 ) ) ;
#6312=CYLINDRICAL_SURFACE ( 'NONE', #34971, 3.499999999999999556 ) ;
#6316=CARTESIAN_POINT ( 'NONE',  ( 2.474675557024783212E-16, 21.54145188432739744, -82.90473080337743284 ) ) ;
#6317=CARTESIAN_POINT ( 'NONE',  ( 1.655278471875001101, 20.36702641396248836, -65.18493913623279923 ) ) ;
#6321=CARTESIAN_POINT ( 'NONE',  ( -3.310556943750001313, 17.50000000000001776, -82.85160580289947063 ) ) ;
#6322=CARTESIAN_POINT ( 'NONE',  ( -1.394453263437886604E-15, 14.00000000000001421, -59.71098080242150274 ) ) ;
#6323=CARTESIAN_POINT ( 'NONE',  ( -1.655278471875002211, 14.63297358603755072, -116.5974391362327935 ) ) ;
#6324=CARTESIAN_POINT ( 'NONE',  ( -1.655278471875002211, 14.63297358603754716, -82.59743913623279354 ) ) ;
#6325=CARTESIAN_POINT ( 'NONE',  ( -3.500000000000000000, 19.52072594216371115, -96.73806413671076143 ) ) ;
#6327=CARTESIAN_POINT ( 'NONE',  ( 2.474675557024783212E-16, 21.54145188432740099, -107.9047308033774328 ) ) ;
#6330=CARTESIAN_POINT ( 'NONE',  ( -3.500000000000000000, 19.52072594216370760, -50.04431413575484555 ) ) ;
#6331=DIRECTION ( 'NONE',  ( -0.000000000000000000, 1.259100132267607459E-16, -1.000000000000000000 ) ) ;
#6332=CARTESIAN_POINT ( 'NONE',  ( -1.394453263437886604E-15, 14.00000000000001066, -26.71098080242150985 ) ) ;
#6333=CARTESIAN_POINT ( 'NONE',  ( 4.648177544792955347E-16, 21.00000000000001421, -58.90473080337742573 ) ) ;
#6335=CARTESIAN_POINT ( 'NONE',  ( -3.310556943750001313, 17.50000000000001421, -65.76410580289947916 ) ) ;
#6337=CARTESIAN_POINT ( 'NONE',  ( 1.655278471875001101, 20.36702641396249547, -124.0974391362328078 ) ) ;
#6340=EDGE_LOOP ( 'NONE', ( #4667, #12146, #40079, #23718 ) ) ;
#6344=CARTESIAN_POINT ( 'NONE',  ( -3.310556943750001313, 17.50000000000001421, -71.76410580289947916 ) ) ;
#6347=ORIENTED_EDGE ( 'NONE', *, *, #1440, .F. ) ;
#6349=ADVANCED_FACE ( 'NONE', ( #4276 ), #20231, .T. ) ;
#6350=( BOUNDED_CURVE ( )  B_SPLINE_CURVE ( 2, ( #6022, #5607, #11980, #35369, #6232, #2415, #15820, #22189, #12618 ),
 .UNSPECIFIED., .F., .F. ) 
 B_SPLINE_CURVE_WITH_KNOTS ( ( 3, 2, 2, 2, 3 ),
 ( 0.5895833333333333481, 0.5902777777777777901, 0.5916666666666666741, 0.5930555555555555580, 0.5937500000000000000 ),
 .UNSPECIFIED. ) 
 CURVE ( )  GEOMETRIC_REPRESENTATION_ITEM ( )  RATIONAL_B_SPLINE_CURVE ( ( 0.9330127018922194093, 0.9330127018922194093, 1.000000000000000000, 0.8660254037844387076, 1.000000000000000000, 0.8660254037844387076, 1.000000000000000000, 0.9330127018922194093, 0.9330127018922194093 ) ) 
 REPRESENTATION_ITEM ( '' )  );
#6351=CARTESIAN_POINT ( 'NONE',  ( -3.310556943750000425, 19.41135094264167549, -142.8474391362327935 ) ) ;
#6353=LINE ( 'NONE', #21880, #14613 ) ;
#6354=CARTESIAN_POINT ( 'NONE',  ( 3.310556943750001313, 19.41135094264165772, -41.26827246956613493 ) ) ;
#6355=CARTESIAN_POINT ( 'NONE',  ( -3.310556943750002645, 15.58864905735837425, -105.7682724695661278 ) ) ;
#6356=CARTESIAN_POINT ( 'NONE',  ( -3.310556943750001313, 17.50000000000001066, -31.76410580289946850 ) ) ;
#6358=CARTESIAN_POINT ( 'NONE',  ( -1.749999999999999778, 20.53108891324555785, -107.1276474690881741 ) ) ;
#6361=CARTESIAN_POINT ( 'NONE',  ( 3.500000000000000000, 15.47927405783632793, -97.23806413671077564 ) ) ;
#6362=CARTESIAN_POINT ( 'NONE',  ( 4.648177544792955347E-16, 21.00000000000002132, -104.9047308033774186 ) ) ;
#6364=ADVANCED_FACE ( 'NONE', ( #33193 ), #36170, .T. ) ;
#6366=CARTESIAN_POINT ( 'NONE',  ( -1.749999999999999778, 20.53108891324555074, -61.12764746908818125 ) ) ;
#6368=CARTESIAN_POINT ( 'NONE',  ( -3.310556943750001313, 17.50000000000001066, -25.76410580289947916 ) ) ;
#6369=EDGE_CURVE ( 'NONE', #1891, #6975, #1507, .T. ) ;
#6370=CARTESIAN_POINT ( 'NONE',  ( 3.500000000000001332, 17.50000000000001066, -46.15473080337742573 ) ) ;
#6372=AXIS2_PLACEMENT_3D ( 'NONE', #35923, #19982, #23390 ) ;
#6373=CARTESIAN_POINT ( 'NONE',  ( -1.655278471875002211, 14.63297358603754006, -32.68493913623279923 ) ) ;
#6375=CARTESIAN_POINT ( 'NONE',  ( 1.750000000000001110, 20.53108891324555074, -65.98806413671076143 ) ) ;
#6376=CARTESIAN_POINT ( 'NONE',  ( -3.500000000000001332, 17.50000000000002487, -141.9609808024215170 ) ) ;
#6380=CARTESIAN_POINT ( 'NONE',  ( -7.022189441860112050E-16, 13.67729811471672186, -80.51410580289945074 ) ) ;
#6382=VERTEX_POINT ( 'NONE', #26829 ) ;
#6383=DIRECTION ( 'NONE',  ( 0.000000000000000000, 1.000000000000000000, 0.000000000000000000 ) ) ;
#6384=ORIENTED_EDGE ( 'NONE', *, *, #35483, .F. ) ;
#6387=CARTESIAN_POINT ( 'NONE',  ( 1.655278471874998436, 14.63297358603754539, -91.43077246956613635 ) ) ;
#6389=CARTESIAN_POINT ( 'NONE',  ( -1.394453263437886604E-15, 14.00000000000001066, -30.40473080337742928 ) ) ;
#6390=ORIENTED_EDGE ( 'NONE', *, *, #21839, .F. ) ;
#6392=FACE_OUTER_BOUND ( 'NONE', #39373, .T. ) ;
#6395=EDGE_CURVE ( 'NONE', #21358, #22548, #4695, .T. ) ;
#6396=EDGE_CURVE ( 'NONE', #39728, #11063, #28886, .T. ) ;
#6398=CARTESIAN_POINT ( 'NONE',  ( -0.9378221735089310451, 14.00000000000002132, -88.44938900211595012 ) ) ;
#6401=EDGE_CURVE ( 'NONE', #25342, #37569, #61, .T. ) ;
#6402=CARTESIAN_POINT ( 'NONE',  ( -3.310556943750001313, 17.50000000000002487, -131.7641058028994507 ) ) ;
#6403=AXIS2_PLACEMENT_3D ( 'NONE', #32014, #9050, #9264 ) ;
#6406=CARTESIAN_POINT ( 'NONE',  ( 3.310556943750001313, 17.50000000000002132, -121.3516058028994706 ) ) ;
#6407=CARTESIAN_POINT ( 'NONE',  ( -3.310556943750000425, 19.41135094264166128, -49.93493913623279923 ) ) ;
#6409=CARTESIAN_POINT ( 'NONE',  ( -3.500000000000002220, 15.47927405783633503, -132.5713974700440758 ) ) ;
#6411=CARTESIAN_POINT ( 'NONE',  ( -3.310556943750002645, 15.58864905735837070, -71.76827246956612782 ) ) ;
#6412=CARTESIAN_POINT ( 'NONE',  ( -3.500000000000001332, 17.50000000000002132, -123.9609808024215027 ) ) ;
#6413=CARTESIAN_POINT ( 'NONE',  ( 3.310556943749999981, 15.58864905735837070, -108.3474391362328078 ) ) ;
#6414=CYLINDRICAL_SURFACE ( 'NONE', #41772, 3.499999999999999556 ) ;
#6415=FACE_OUTER_BOUND ( 'NONE', #21517, .T. ) ;
#6417=CARTESIAN_POINT ( 'NONE',  ( 1.749999999999998224, 14.46891108675447946, -77.62764746908817415 ) ) ;
#6419=CARTESIAN_POINT ( 'NONE',  ( 1.655278471874998436, 14.63297358603754006, -43.43077246956614346 ) ) ;
#6420=CARTESIAN_POINT ( 'NONE',  ( -7.022189441860112050E-16, 13.67729811471672541, -100.6016058028994564 ) ) ;
#6421=CARTESIAN_POINT ( 'NONE',  ( -3.500000000000000000, 19.52072594216371826, -114.0443141357548313 ) ) ;
#6423=CARTESIAN_POINT ( 'NONE',  ( 1.750000000000001110, 20.53108891324555074, -62.98806413671076143 ) ) ;
#6426=CARTESIAN_POINT ( 'NONE',  ( 3.310556943750001313, 17.50000000000002132, -116.3516058028994706 ) ) ;
#6432=CARTESIAN_POINT ( 'NONE',  ( 1.655278471874998436, 14.63297358603754716, -98.43077246956613635 ) ) ;
#6435=VERTEX_POINT ( 'NONE', #12107 ) ;
#6436=CARTESIAN_POINT ( 'NONE',  ( -1.750000000000002220, 14.46891108675447590, -28.79431413575483845 ) ) ;
#6440=CARTESIAN_POINT ( 'NONE',  ( 1.750000000000001110, 20.53108891324554719, -44.98806413671076143 ) ) ;
#6444=CARTESIAN_POINT ( 'NONE',  ( -3.310556943750000425, 19.41135094264166128, -35.84743913623281486 ) ) ;
#6445=CARTESIAN_POINT ( 'NONE',  ( 4.648177544792955347E-16, 21.00000000000002132, -106.9047308033774328 ) ) ;
#6449=EDGE_CURVE ( 'NONE', #1125, #22806, #17474, .T. ) ;
#6450=FACE_OUTER_BOUND ( 'NONE', #21144, .T. ) ;
#6451=ORIENTED_EDGE ( 'NONE', *, *, #7947, .F. ) ;
#6452=CARTESIAN_POINT ( 'NONE',  ( 0.000000000000000000, 21.00000000000002487, -149.5231586289125687 ) ) ;
#6454=EDGE_CURVE ( 'NONE', #39933, #25787, #24268, .T. ) ;
#6455=CARTESIAN_POINT ( 'NONE',  ( -1.394453263437886604E-15, 14.00000000000002132, -119.4047308033774328 ) ) ;
#6456=CARTESIAN_POINT ( 'NONE',  ( 3.500000000000000000, 15.47927405783632970, -119.2380641367107614 ) ) ;
#6457=CARTESIAN_POINT ( 'NONE',  ( -1.394453263437886604E-15, 14.00000000000001066, -33.71098080242150985 ) ) ;
#6458=CARTESIAN_POINT ( 'NONE',  ( 3.310556943750001313, 17.50000000000002487, -134.3516058028994564 ) ) ;
#6459=CARTESIAN_POINT ( 'NONE',  ( -3.500000000000001332, 17.50000000000001066, -34.96098080242150985 ) ) ;
#6460=CYLINDRICAL_SURFACE ( 'NONE', #7653, 3.499999999999999556 ) ;
#6462=CIRCLE ( 'NONE', #2364, 3.499999999999999556 ) ;
#6463=AXIS2_PLACEMENT_3D ( 'NONE', #19287, #16525, #35236 ) ;
#6464=CARTESIAN_POINT ( 'NONE',  ( 3.500000000000001332, 19.52072594216370405, -41.37764746908818125 ) ) ;
#6466=CARTESIAN_POINT ( 'NONE',  ( 2.474675557024783212E-16, 21.54145188432740810, -138.2109808024215170 ) ) ;
#6468=CARTESIAN_POINT ( 'NONE',  ( -3.310556943750000425, 19.41135094264166838, -122.8474391362328220 ) ) ;
#6471=CARTESIAN_POINT ( 'NONE',  ( -0.9378221735089310451, 14.00000000000002132, -81.75563900116002003 ) ) ;
#6472=CARTESIAN_POINT ( 'NONE',  ( 3.500000000000001332, 17.50000000000001776, -89.46098080242151696 ) ) ;
#6473=CARTESIAN_POINT ( 'NONE',  ( 0.9378221735089281585, 14.00000000000000888, -33.36007260463891555 ) ) ;
#6474=CARTESIAN_POINT ( 'NONE',  ( 2.340729813953370519E-16, 21.32270188528330834, -59.01410580289947916 ) ) ;
#6475=CARTESIAN_POINT ( 'NONE',  ( 3.310556943750001313, 17.50000000000002132, -118.3516058028994706 ) ) ;
#6477=CARTESIAN_POINT ( 'NONE',  ( 2.474675557024783212E-16, 21.54145188432739033, -30.90473080337742573 ) ) ;
#6478=CARTESIAN_POINT ( 'NONE',  ( -1.749999999999999778, 20.53108891324555785, -109.1276474690881741 ) ) ;
#6480=CARTESIAN_POINT ( 'NONE',  ( -7.022189441860112050E-16, 13.67729811471672896, -135.6016058028994564 ) ) ;
#6482=CARTESIAN_POINT ( 'NONE',  ( 3.500000000000001332, 17.50000000000002487, -138.1547308033774186 ) ) ;
#6483=CARTESIAN_POINT ( 'NONE',  ( -7.022189441860112050E-16, 13.67729811471671830, -45.60160580289945642 ) ) ;
#6485=CARTESIAN_POINT ( 'NONE',  ( -1.655278471875002211, 14.63297358603754539, -69.68493913623279923 ) ) ;
#6487=CARTESIAN_POINT ( 'NONE',  ( -3.310556943750002645, 15.58864905735836892, -65.68077246956613635 ) ) ;
#6489=CARTESIAN_POINT ( 'NONE',  ( 3.310556943750001313, 19.41135094264166838, -83.26827246956612782 ) ) ;
#6494=CARTESIAN_POINT ( 'NONE',  ( -1.655278471875002211, 14.63297358603754184, -52.59743913623281486 ) ) ;
#6496=CARTESIAN_POINT ( 'NONE',  ( -3.310556943750002645, 15.58864905735837425, -106.6807724695661506 ) ) ;
#6497=CARTESIAN_POINT ( 'NONE',  ( 3.500000000000001332, 19.52072594216371115, -96.07139747004409003 ) ) ;
#6498=PRODUCT_DEFINITION ( 'UNKNOWN', '', #14641, #13521 ) ;
#6501=AXIS2_PLACEMENT_3D ( 'NONE', #36557, #8255, #5062 ) ;
#6503=VERTEX_POINT ( 'NONE', #2544 ) ;
#6505=ADVANCED_FACE ( 'NONE', ( #17880 ), #15528, .T. ) ;
#6506=CARTESIAN_POINT ( 'NONE',  ( 3.310556943749999981, 15.58864905735836537, -57.34743913623279354 ) ) ;
#6507=ORIENTED_EDGE ( 'NONE', *, *, #6454, .F. ) ;
#6508=ORIENTED_EDGE ( 'NONE', *, *, #24409, .F. ) ;
#6509=CYLINDRICAL_SURFACE ( 'NONE', #26688, 3.499999999999999556 ) ;
#6510=DIRECTION ( 'NONE',  ( -0.000000000000000000, 1.259100132267607459E-16, -1.000000000000000000 ) ) ;
#6514=CARTESIAN_POINT ( 'NONE',  ( 0.000000000000000000, 17.50000000000002487, -149.5231586289125687 ) ) ;
#6515=CARTESIAN_POINT ( 'NONE',  ( -7.022189441860112050E-16, 13.67729811471672896, -122.5141058028994792 ) ) ;
#6516=CARTESIAN_POINT ( 'NONE',  ( -1.394453263437886604E-15, 14.00000000000001776, -94.71098080242150274 ) ) ;
#6518=CARTESIAN_POINT ( 'NONE',  ( -7.022189441860112050E-16, 13.67729811471671475, -36.60160580289946353 ) ) ;
#6519=CARTESIAN_POINT ( 'NONE',  ( 3.310556943750001313, 19.41135094264165772, -28.26827246956613493 ) ) ;
#6520=CARTESIAN_POINT ( 'NONE',  ( 1.655278471874998436, 14.63297358603754539, -89.51827246956612782 ) ) ;
#6521=CARTESIAN_POINT ( 'NONE',  ( 3.310556943750001313, 17.50000000000002487, -140.2641058028994792 ) ) ;
#6524=( BOUNDED_CURVE ( )  B_SPLINE_CURVE ( 2, ( #28815, #41815, #12668, #41180, #25018, #37979, #5654, #9692, #33052 ),
 .UNSPECIFIED., .F., .T. ) 
 B_SPLINE_CURVE_WITH_KNOTS ( ( 3, 2, 2, 2, 3 ),
 ( 0.4854166666666666630, 0.4861111111111111049, 0.4874999999999999889, 0.4888888888888888729, 0.4895833333333333148 ),
 .UNSPECIFIED. ) 
 CURVE ( )  GEOMETRIC_REPRESENTATION_ITEM ( )  RATIONAL_B_SPLINE_CURVE ( ( 0.9330127018922194093, 0.9330127018922194093, 1.000000000000000000, 0.8660254037844387076, 1.000000000000000000, 0.8660254037844387076, 1.000000000000000000, 0.9330127018922194093, 0.9330127018922194093 ) ) 
 REPRESENTATION_ITEM ( '' )  );
#6525=CARTESIAN_POINT ( 'NONE',  ( 1.655278471874998436, 14.63297358603755072, -132.5182724695661420 ) ) ;
#6528=CARTESIAN_POINT ( 'NONE',  ( 3.310556943750001313, 19.41135094264166483, -93.18077246956613635 ) ) ;
#6529=CARTESIAN_POINT ( 'NONE',  ( 0.9378221735089281585, 14.00000000000000888, -28.36007260463891200 ) ) ;
#6531=CARTESIAN_POINT ( 'NONE',  ( 4.648177544792955347E-16, 21.00000000000001066, -32.21098080242150274 ) ) ;
#6533=CARTESIAN_POINT ( 'NONE',  ( 1.750000000000001110, 20.53108891324555074, -72.98806413671076143 ) ) ;
#6534=CARTESIAN_POINT ( 'NONE',  ( 3.310556943750001313, 17.50000000000001421, -60.35160580289947063 ) ) ;
#6537=CARTESIAN_POINT ( 'NONE',  ( -3.500000000000000000, 19.52072594216371826, -129.7380641367107614 ) ) ;
#6538=CARTESIAN_POINT ( 'NONE',  ( -3.310556943750000425, 19.41135094264166483, -83.93493913623278502 ) ) ;
#6539=CARTESIAN_POINT ( 'NONE',  ( -3.310556943750000425, 19.41135094264167549, -142.9349391362327992 ) ) ;
#6541=CARTESIAN_POINT ( 'NONE',  ( 3.310556943750001313, 19.41135094264166838, -115.1807724695661364 ) ) ;
#6542=CARTESIAN_POINT ( 'NONE',  ( -3.310556943750000425, 19.41135094264166483, -81.84743913623279354 ) ) ;
#6543=CYLINDRICAL_SURFACE ( 'NONE', #30832, 3.499999999999999556 ) ;
#6545=( BOUNDED_CURVE ( )  B_SPLINE_CURVE ( 2, ( #40643, #34678, #5330, #28087, #22127, #41491, #28499, #5128, #12340 ),
 .UNSPECIFIED., .F., .T. ) 
 B_SPLINE_CURVE_WITH_KNOTS ( ( 3, 2, 2, 2, 3 ),
 ( 0.3437500000000000000, 0.3444444444444444420, 0.3458333333333333259, 0.3472222222222222099, 0.3479166666666666519 ),
 .UNSPECIFIED. ) 
 CURVE ( )  GEOMETRIC_REPRESENTATION_ITEM ( )  RATIONAL_B_SPLINE_CURVE ( ( 0.9330127018922194093, 0.9330127018922194093, 1.000000000000000000, 0.8660254037844387076, 1.000000000000000000, 0.8660254037844387076, 1.000000000000000000, 0.9330127018922194093, 0.9330127018922194093 ) ) 
 REPRESENTATION_ITEM ( '' )  );
#6546=CARTESIAN_POINT ( 'NONE',  ( -3.500000000000002220, 15.47927405783632970, -107.5713974700440900 ) ) ;
#6548=CARTESIAN_POINT ( 'NONE',  ( 3.500000000000001332, 19.52072594216370760, -71.37764746908817415 ) ) ;
#6549=CARTESIAN_POINT ( 'NONE',  ( 3.500000000000001332, 17.50000000000001066, -44.15473080337743994 ) ) ;
#6551=CARTESIAN_POINT ( 'NONE',  ( 3.500000000000000000, 15.47927405783632437, -65.54431413575484555 ) ) ;
#6552=CARTESIAN_POINT ( 'NONE',  ( -3.310556943750001313, 17.50000000000001421, -68.76410580289947916 ) ) ;
#6554=CARTESIAN_POINT ( 'NONE',  ( 1.655278471875001101, 20.36702641396249547, -123.0974391362328078 ) ) ;
#6555=CARTESIAN_POINT ( 'NONE',  ( 1.750000000000001110, 20.53108891324555074, -70.98806413671076143 ) ) ;
#6556=CARTESIAN_POINT ( 'NONE',  ( -3.500000000000000000, 19.52072594216371826, -125.7380641367107756 ) ) ;
#6557=VERTEX_POINT ( 'NONE', #19758 ) ;
#6558=CARTESIAN_POINT ( 'NONE',  ( -0.9378221735089291577, 21.00000000000001066, -43.16632260368298546 ) ) ;
#6559=CARTESIAN_POINT ( 'NONE',  ( 4.648177544792955347E-16, 21.00000000000002132, -127.9047308033774186 ) ) ;
#6561=CARTESIAN_POINT ( 'NONE',  ( -7.022189441860112050E-16, 13.67729811471672186, -76.51410580289947916 ) ) ;
#6562=EDGE_LOOP ( 'NONE', ( #17760, #21645, #26226, #33335 ) ) ;
#6566=CARTESIAN_POINT ( 'NONE',  ( -3.310556943750000425, 19.41135094264167549, -139.8474391362327935 ) ) ;
#6568=CARTESIAN_POINT ( 'NONE',  ( 3.500000000000001332, 17.50000000000002487, -134.4609808024214885 ) ) ;
#6569=CARTESIAN_POINT ( 'NONE',  ( -1.655278471875002211, 14.63297358603754184, -43.68493913623279212 ) ) ;
#6570=CARTESIAN_POINT ( 'NONE',  ( -1.655278471874999990, 20.36702641396249547, -105.0182724695661278 ) ) ;
#6571=CARTESIAN_POINT ( 'NONE',  ( -1.655278471875002211, 14.63297358603754006, -31.59743913623280775 ) ) ;
#6572=CARTESIAN_POINT ( 'NONE',  ( 1.750000000000001110, 20.53108891324555074, -68.98806413671077564 ) ) ;
#6573=CARTESIAN_POINT ( 'NONE',  ( 3.500000000000001332, 17.50000000000002132, -108.4609808024215027 ) ) ;
#6575=CARTESIAN_POINT ( 'NONE',  ( -1.394453263437886604E-15, 14.00000000000002132, -118.7109808024215170 ) ) ;
#6576=CARTESIAN_POINT ( 'NONE',  ( -3.500000000000000888, 19.52072594216371115, -88.73806413671076143 ) ) ;
#6580=CARTESIAN_POINT ( 'NONE',  ( 3.500000000000001776, 19.52072594216370760, -58.37764746908818125 ) ) ;
#6582=CARTESIAN_POINT ( 'NONE',  ( -1.750000000000002220, 14.46891108675447413, -24.79431413575484910 ) ) ;
#6583=CARTESIAN_POINT ( 'NONE',  ( -3.500000000000000888, 19.52072594216370760, -48.73806413671076143 ) ) ;
#6584=CARTESIAN_POINT ( 'NONE',  ( -0.9378221735089291577, 21.00000000000002487, -132.1663226036829712 ) ) ;
#6585=CARTESIAN_POINT ( 'NONE',  ( -3.310556943750000425, 19.41135094264166128, -31.93493913623279568 ) ) ;
#6590=EDGE_CURVE ( 'NONE', #23833, #9218, #18918, .T. ) ;
#6592=CARTESIAN_POINT ( 'NONE',  ( 2.340729813953370519E-16, 21.32270188528331190, -84.01410580289947916 ) ) ;
#6599=CARTESIAN_POINT ( 'NONE',  ( -7.022189441860112050E-16, 13.67729811471672363, -88.51410580289947916 ) ) ;
#6600=( BOUNDED_CURVE ( )  B_SPLINE_CURVE ( 2, ( #40860, #11715, #37674, #17285, #28094, #34687, #12773, #12563, #38510 ),
 .UNSPECIFIED., .F., .F. ) 
 B_SPLINE_CURVE_WITH_KNOTS ( ( 3, 2, 2, 2, 3 ),
 ( 0.5354166666666666519, 0.5361111111111110938, 0.5374999999999999778, 0.5388888888888888618, 0.5395833333333333037 ),
 .UNSPECIFIED. ) 
 CURVE ( )  GEOMETRIC_REPRESENTATION_ITEM ( )  RATIONAL_B_SPLINE_CURVE ( ( 0.9330127018922194093, 0.9330127018922194093, 1.000000000000000000, 0.8660254037844387076, 1.000000000000000000, 0.8660254037844387076, 1.000000000000000000, 0.9330127018922194093, 0.9330127018922194093 ) ) 
 REPRESENTATION_ITEM ( '' )  );
#6602=ORIENTED_EDGE ( 'NONE', *, *, #15523, .T. ) ;
#6604=CARTESIAN_POINT ( 'NONE',  ( 3.500000000000001332, 19.52072594216370760, -66.37764746908817415 ) ) ;
#6607=CARTESIAN_POINT ( 'NONE',  ( 4.648177544792955347E-16, 21.00000000000002132, -127.9047308033774186 ) ) ;
#6610=CARTESIAN_POINT ( 'NONE',  ( -3.310556943750002645, 15.58864905735837780, -132.6807724695661364 ) ) ;
#6613=CARTESIAN_POINT ( 'NONE',  ( 0.9378221735089281585, 14.00000000000001599, -73.36007260463891555 ) ) ;
#6614=CARTESIAN_POINT ( 'NONE',  ( -7.022189441860112050E-16, 13.67729811471672718, -119.6016058028994706 ) ) ;
#6616=CARTESIAN_POINT ( 'NONE',  ( -1.750000000000002220, 14.46891108675448834, -128.4880641367107614 ) ) ;
#6617=CARTESIAN_POINT ( 'NONE',  ( -1.655278471875002211, 14.63297358603754539, -73.68493913623279923 ) ) ;
#6618=CARTESIAN_POINT ( 'NONE',  ( 3.500000000000001776, 19.52072594216371826, -121.3776474690881741 ) ) ;
#6619=CARTESIAN_POINT ( 'NONE',  ( 3.310556943750001313, 17.50000000000001776, -101.2641058028994792 ) ) ;
#6620=CARTESIAN_POINT ( 'NONE',  ( -1.749999999999999778, 20.53108891324555785, -107.8213974700441042 ) ) ;
#6621=EDGE_CURVE ( 'NONE', #3780, #41828, #7662, .T. ) ;
#6624=CARTESIAN_POINT ( 'NONE',  ( -3.500000000000001332, 17.50000000000001421, -73.96098080242151696 ) ) ;
#6625=DIRECTION ( 'NONE',  ( 0.000000000000000000, 1.000000000000000000, 0.000000000000000000 ) ) ;
#6626=CARTESIAN_POINT ( 'NONE',  ( 1.655278471875001101, 20.36702641396248481, -40.09743913623281486 ) ) ;
#6627=CARTESIAN_POINT ( 'NONE',  ( -7.022189441860112050E-16, 13.67729811471672541, -96.60160580289947063 ) ) ;
#6628=CARTESIAN_POINT ( 'NONE',  ( 3.500000000000001332, 17.50000000000001421, -65.15473080337743284 ) ) ;
#6629=CARTESIAN_POINT ( 'NONE',  ( 1.655278471875001101, 20.36702641396249547, -118.1849391362327850 ) ) ;
#6630=EDGE_CURVE ( 'NONE', #12051, #20737, #30504, .T. ) ;
#6631=LINE ( 'NONE', #9840, #293 ) ;
#6636=CARTESIAN_POINT ( 'NONE',  ( -3.310556943750000425, 19.41135094264166838, -98.84743913623280775 ) ) ;
#6639=CARTESIAN_POINT ( 'NONE',  ( 1.750000000000001110, 20.53108891324556140, -136.2943141357548598 ) ) ;
#6640=EDGE_CURVE ( 'NONE', #2211, #14503, #39184, .T. ) ;
#6641=CARTESIAN_POINT ( 'NONE',  ( 1.749999999999998224, 14.46891108675448123, -81.62764746908818836 ) ) ;
#6642=CARTESIAN_POINT ( 'NONE',  ( 4.648177544792955347E-16, 21.00000000000001421, -71.21098080242150274 ) ) ;
#6647=CARTESIAN_POINT ( 'NONE',  ( 2.340729813953370519E-16, 21.32270188528330834, -27.01410580289947916 ) ) ;
#6648=ORIENTED_EDGE ( 'NONE', *, *, #18687, .F. ) ;
#6655=LINE ( 'NONE', #19620, #11704 ) ;
#6657=DIRECTION ( 'NONE',  ( -0.000000000000000000, 1.259100132267607459E-16, -1.000000000000000000 ) ) ;
#6658=CARTESIAN_POINT ( 'NONE',  ( -1.749999999999999778, 20.53108891324555785, -118.8213974700440900 ) ) ;
#6660=CARTESIAN_POINT ( 'NONE',  ( -3.310556943750000425, 19.41135094264167549, -136.9349391362327992 ) ) ;
#6661=CARTESIAN_POINT ( 'NONE',  ( -3.500000000000000888, 19.52072594216370405, -35.04431413575484555 ) ) ;
#6665=CARTESIAN_POINT ( 'NONE',  ( 3.500000000000000000, 15.47927405783633503, -139.5443141357548313 ) ) ;
#6666=ADVANCED_FACE ( 'NONE', ( #23809 ), #36775, .T. ) ;
#6667=CARTESIAN_POINT ( 'NONE',  ( -7.022189441860112050E-16, 13.67729811471672718, -121.5141058028994792 ) ) ;
#6670=DIRECTION ( 'NONE',  ( -0.000000000000000000, 1.259100132267607459E-16, -1.000000000000000000 ) ) ;
#6671=CARTESIAN_POINT ( 'NONE',  ( -3.500000000000000888, 19.52072594216371115, -90.04431413575483134 ) ) ;
#6673=CARTESIAN_POINT ( 'NONE',  ( -3.310556943750000425, 19.41135094264166128, -57.84743913623280065 ) ) ;
#6674=CARTESIAN_POINT ( 'NONE',  ( -7.022189441860112050E-16, 13.67729811471672718, -109.6016058028994564 ) ) ;
#6675=CYLINDRICAL_SURFACE ( 'NONE', #23448, 3.499999999999999556 ) ;
#6676=CARTESIAN_POINT ( 'NONE',  ( -7.424026671074350129E-16, 13.45854811567263098, -32.40473080337742573 ) ) ;
#6677=LINE ( 'NONE', #4114, #14457 ) ;
#6679=CARTESIAN_POINT ( 'NONE',  ( 3.310556943750001313, 19.41135094264167549, -134.2682724695661420 ) ) ;
#6684=CARTESIAN_POINT ( 'NONE',  ( 3.310556943749999981, 15.58864905735836714, -68.43493913623279923 ) ) ;
#6686=CARTESIAN_POINT ( 'NONE',  ( 3.310556943749999981, 15.58864905735836537, -65.34743913623282197 ) ) ;
#6687=ORIENTED_EDGE ( 'NONE', *, *, #18356, .T. ) ;
#6688=CARTESIAN_POINT ( 'NONE',  ( 1.655278471874998436, 14.63297358603754539, -88.51827246956612782 ) ) ;
#6689=EDGE_CURVE ( 'NONE', #11167, #39978, #29960, .T. ) ;
#6693=CARTESIAN_POINT ( 'NONE',  ( -3.310556943750000425, 19.41135094264166128, -42.84743913623280065 ) ) ;
#6695=CARTESIAN_POINT ( 'NONE',  ( -3.310556943750001313, 17.50000000000002132, -107.7641058028994649 ) ) ;
#6700=ORIENTED_EDGE ( 'NONE', *, *, #40594, .F. ) ;
#6702=CARTESIAN_POINT ( 'NONE',  ( -3.310556943750000425, 19.41135094264166128, -55.84743913623280065 ) ) ;
#6703=ORIENTED_EDGE ( 'NONE', *, *, #27816, .T. ) ;
#6704=ORIENTED_EDGE ( 'NONE', *, *, #37617, .T. ) ;
#6707=CARTESIAN_POINT ( 'NONE',  ( -1.750000000000002220, 14.46891108675447768, -40.48806413671076143 ) ) ;
#6709=CARTESIAN_POINT ( 'NONE',  ( 4.286263797015737581E-16, 14.00000000000002487, -149.5231586289125687 ) ) ;
#6711=CARTESIAN_POINT ( 'NONE',  ( 3.500000000000001332, 19.52072594216371826, -143.3776474690881741 ) ) ;
#6712=CARTESIAN_POINT ( 'NONE',  ( -3.310556943750001313, 17.50000000000002132, -125.7641058028994792 ) ) ;
#6713=CARTESIAN_POINT ( 'NONE',  ( -1.394453263437886604E-15, 14.00000000000001776, -102.7109808024215027 ) ) ;
#6716=EDGE_CURVE ( 'NONE', #8532, #19157, #1448, .T. ) ;
#6717=CARTESIAN_POINT ( 'NONE',  ( -1.655278471875002211, 14.63297358603753828, -24.68493913623280633 ) ) ;
#6718=CARTESIAN_POINT ( 'NONE',  ( -1.655278471874999990, 20.36702641396249192, -90.01827246956612782 ) ) ;
#6719=CARTESIAN_POINT ( 'NONE',  ( 1.655278471874998436, 14.63297358603755249, -140.4307724695661364 ) ) ;
#6721=CARTESIAN_POINT ( 'NONE',  ( -3.500000000000002220, 15.47927405783632082, -34.57139747004410424 ) ) ;
#6723=CARTESIAN_POINT ( 'NONE',  ( -3.310556943750001313, 17.50000000000002487, -130.8516058028994564 ) ) ;
#6725=CARTESIAN_POINT ( 'NONE',  ( -3.310556943750001313, 17.50000000000001776, -89.76410580289947916 ) ) ;
#6727=DIRECTION ( 'NONE',  ( -0.000000000000000000, 1.259100132267607459E-16, -1.000000000000000000 ) ) ;
#6728=CARTESIAN_POINT ( 'NONE',  ( 0.9378221735089281585, 14.00000000000002132, -111.6663226036829712 ) ) ;
#6729=CARTESIAN_POINT ( 'NONE',  ( -3.500000000000001332, 17.50000000000001776, -77.65473080337741862 ) ) ;
#6731=CARTESIAN_POINT ( 'NONE',  ( 3.310556943750001313, 17.50000000000001421, -59.35160580289947063 ) ) ;
#6735=CARTESIAN_POINT ( 'NONE',  ( -3.310556943750001313, 17.50000000000001776, -86.85160580289947063 ) ) ;
#6739=CARTESIAN_POINT ( 'NONE',  ( 2.340729813953370519E-16, 21.32270188528331900, -108.0141058028994649 ) ) ;
#6740=CARTESIAN_POINT ( 'NONE',  ( 3.310556943750001313, 19.41135094264166483, -82.18077246956616477 ) ) ;
#6741=CARTESIAN_POINT ( 'NONE',  ( 1.749999999999998224, 14.46891108675448834, -138.6276474690881741 ) ) ;
#6742=ORIENTED_EDGE ( 'NONE', *, *, #27748, .F. ) ;
#6743=CARTESIAN_POINT ( 'NONE',  ( 1.655278471875001101, 20.36702641396249547, -104.1849391362328134 ) ) ;
#6744=CARTESIAN_POINT ( 'NONE',  ( 3.500000000000000000, 15.47927405783632793, -101.2380641367107614 ) ) ;
#6747=DIRECTION ( 'NONE',  ( 0.000000000000000000, 1.000000000000000000, 0.000000000000000000 ) ) ;
#6748=CARTESIAN_POINT ( 'NONE',  ( 1.749999999999998224, 14.46891108675447768, -54.32139747004409713 ) ) ;
#6750=CARTESIAN_POINT ( 'NONE',  ( 3.310556943750001313, 19.41135094264166483, -65.18077246956615056 ) ) ;
#6752=CARTESIAN_POINT ( 'NONE',  ( -1.655278471874999990, 20.36702641396249547, -119.9307724695661364 ) ) ;
#6753=DIRECTION ( 'NONE',  ( -0.000000000000000000, 1.259100132267607459E-16, -1.000000000000000000 ) ) ;
#6756=EDGE_LOOP ( 'NONE', ( #13786, #8647, #23495, #27791 ) ) ;
#6757=CARTESIAN_POINT ( 'NONE',  ( -3.500000000000002220, 15.47927405783632437, -42.87764746908817415 ) ) ;
#6758=CARTESIAN_POINT ( 'NONE',  ( 4.648177544792955347E-16, 21.00000000000002132, -115.2109808024214885 ) ) ;
#6759=CARTESIAN_POINT ( 'NONE',  ( -1.655278471874999990, 20.36702641396248836, -71.93077246956613635 ) ) ;
#6760=VERTEX_POINT ( 'NONE', #36125 ) ;
#6765=CARTESIAN_POINT ( 'NONE',  ( 1.655278471874998436, 14.63297358603755249, -141.4307724695661364 ) ) ;
#6768=( BOUNDED_CURVE ( )  B_SPLINE_CURVE ( 2, ( #21446, #34421, #17842, #24440, #37407, #17640, #11252, #21239, #36783 ),
 .UNSPECIFIED., .F., .F. ) 
 B_SPLINE_CURVE_WITH_KNOTS ( ( 3, 2, 2, 2, 3 ),
 ( 0.4937500000000000222, 0.4944444444444444642, 0.4958333333333333481, 0.4972222222222222321, 0.4979166666666666741 ),
 .UNSPECIFIED. ) 
 CURVE ( )  GEOMETRIC_REPRESENTATION_ITEM ( )  RATIONAL_B_SPLINE_CURVE ( ( 0.9330127018922194093, 0.9330127018922194093, 1.000000000000000000, 0.8660254037844387076, 1.000000000000000000, 0.8660254037844387076, 1.000000000000000000, 0.9330127018922194093, 0.9330127018922194093 ) ) 
 REPRESENTATION_ITEM ( '' )  );
#6770=CARTESIAN_POINT ( 'NONE',  ( 3.310556943750001313, 17.50000000000001066, -37.35160580289946353 ) ) ;
#6771=CARTESIAN_POINT ( 'NONE',  ( 1.655278471874998436, 14.63297358603754716, -105.5182724695661278 ) ) ;
#6773=CARTESIAN_POINT ( 'NONE',  ( 2.340729813953370519E-16, 21.32270188528330479, -30.01410580289948271 ) ) ;
#6774=CARTESIAN_POINT ( 'NONE',  ( 0.9378221735089281585, 14.00000000000001599, -69.36007260463891555 ) ) ;
#6775=CARTESIAN_POINT ( 'NONE',  ( 3.500000000000000000, 15.47927405783632793, -101.5443141357548456 ) ) ;
#6777=DIRECTION ( 'NONE',  ( 0.000000000000000000, 1.000000000000000000, 0.000000000000000000 ) ) ;
#6778=CARTESIAN_POINT ( 'NONE',  ( 3.500000000000001332, 17.50000000000001776, -92.15473080337743284 ) ) ;
#6780=CARTESIAN_POINT ( 'NONE',  ( -0.9378221735089291577, 21.00000000000001776, -78.16632260368297125 ) ) ;
#6783=CARTESIAN_POINT ( 'NONE',  ( 3.500000000000000000, 15.47927405783632082, -51.54431413575484555 ) ) ;
#6784=DIRECTION ( 'NONE',  ( -0.000000000000000000, 1.259100132267607459E-16, -1.000000000000000000 ) ) ;
#6785=CARTESIAN_POINT ( 'NONE',  ( 1.655278471875001101, 20.36702641396248481, -24.09743913623281486 ) ) ;
#6786=CARTESIAN_POINT ( 'NONE',  ( 3.500000000000001332, 17.50000000000001066, -41.15473080337743284 ) ) ;
#6787=CARTESIAN_POINT ( 'NONE',  ( -3.310556943750001313, 17.50000000000001066, -25.85160580289947063 ) ) ;
#6789=CARTESIAN_POINT ( 'NONE',  ( -3.500000000000000000, 19.52072594216371115, -80.73806413671076143 ) ) ;
#6790=CARTESIAN_POINT ( 'NONE',  ( 4.648177544792955347E-16, 21.00000000000001066, -42.21098080242150274 ) ) ;
#6792=CARTESIAN_POINT ( 'NONE',  ( 0.000000000000000000, 17.50000000000002487, -149.5231586289125687 ) ) ;
#6794=CARTESIAN_POINT ( 'NONE',  ( 2.340729813953370519E-16, 21.32270188528331190, -81.01410580289947916 ) ) ;
#6798=LINE ( 'NONE', #42116, #967 ) ;
#6799=CARTESIAN_POINT ( 'NONE',  ( 1.749999999999998224, 14.46891108675447946, -80.62764746908818836 ) ) ;
#6800=VERTEX_POINT ( 'NONE', #13585 ) ;
#6802=CARTESIAN_POINT ( 'NONE',  ( -3.310556943750002645, 15.58864905735837247, -87.68077246956613635 ) ) ;
#6803=EDGE_CURVE ( 'NONE', #28459, #24957, #18830, .T. ) ;
#6805=ORIENTED_EDGE ( 'NONE', *, *, #26192, .F. ) ;
#6808=DIRECTION ( 'NONE',  ( -0.000000000000000000, 1.259100132267607459E-16, -1.000000000000000000 ) ) ;
#6809=CARTESIAN_POINT ( 'NONE',  ( -1.749999999999999778, 20.53108891324556140, -143.1276474690881741 ) ) ;
#6810=CARTESIAN_POINT ( 'NONE',  ( 1.655278471875001101, 20.36702641396249547, -129.0974391362328220 ) ) ;
#6814=CARTESIAN_POINT ( 'NONE',  ( 3.310556943749999981, 15.58864905735837247, -117.4349391362327850 ) ) ;
#6816=ORIENTED_EDGE ( 'NONE', *, *, #37130, .T. ) ;
#6817=CARTESIAN_POINT ( 'NONE',  ( -1.749999999999999778, 20.53108891324556140, -129.8213974700441042 ) ) ;
#6818=AXIS2_PLACEMENT_3D ( 'NONE', #27266, #890, #26840 ) ;
#6819=CARTESIAN_POINT ( 'NONE',  ( -7.022189441860112050E-16, 13.67729811471672186, -71.60160580289947063 ) ) ;
#6820=CARTESIAN_POINT ( 'NONE',  ( -1.749999999999999778, 20.53108891324555785, -117.1276474690881741 ) ) ;
#6821=CARTESIAN_POINT ( 'NONE',  ( 1.655278471874998436, 14.63297358603754716, -102.4307724695661364 ) ) ;
#6823=CARTESIAN_POINT ( 'NONE',  ( 3.500000000000000000, 15.47927405783632970, -105.5443141357548171 ) ) ;
#6825=CARTESIAN_POINT ( 'NONE',  ( -7.424026671074350129E-16, 13.45854811567263454, -72.71098080242150274 ) ) ;
#6826=CARTESIAN_POINT ( 'NONE',  ( 4.648177544792955347E-16, 21.00000000000002132, -125.9047308033774186 ) ) ;
#6827=CARTESIAN_POINT ( 'NONE',  ( -3.310556943750001313, 17.50000000000001066, -37.76410580289947205 ) ) ;
#6829=CARTESIAN_POINT ( 'NONE',  ( -1.655278471874999990, 20.36702641396249192, -98.01827246956612782 ) ) ;
#6830=CARTESIAN_POINT ( 'NONE',  ( -1.750000000000002220, 14.46891108675447946, -64.48806413671076143 ) ) ;
#6832=CARTESIAN_POINT ( 'NONE',  ( -1.655278471874999990, 20.36702641396249547, -118.0182724695661278 ) ) ;
#6839=CARTESIAN_POINT ( 'NONE',  ( 3.310556943749999981, 15.58864905735837070, -96.34743913623280775 ) ) ;
#6840=( BOUNDED_CURVE ( )  B_SPLINE_CURVE ( 2, ( #737, #10523, #23505, #39652, #36467, #7331, #22865, #20301, #3501 ),
 .UNSPECIFIED., .F., .T. ) 
 B_SPLINE_CURVE_WITH_KNOTS ( ( 3, 2, 2, 2, 3 ),
 ( 0.7479166666666666741, 0.7486111111111111160, 0.7500000000000000000, 0.7513888888888888840, 0.7520833333333333259 ),
 .UNSPECIFIED. ) 
 CURVE ( )  GEOMETRIC_REPRESENTATION_ITEM ( )  RATIONAL_B_SPLINE_CURVE ( ( 0.9330127018922194093, 0.9330127018922194093, 1.000000000000000000, 0.8660254037844387076, 1.000000000000000000, 0.8660254037844387076, 1.000000000000000000, 0.9330127018922194093, 0.9330127018922194093 ) ) 
 REPRESENTATION_ITEM ( '' )  );
#6843=ORIENTED_EDGE ( 'NONE', *, *, #31572, .T. ) ;
#6847=CARTESIAN_POINT ( 'NONE',  ( -3.500000000000001332, 17.50000000000001421, -70.96098080242151696 ) ) ;
#6848=ORIENTED_EDGE ( 'NONE', *, *, #2433, .T. ) ;
#6852=CARTESIAN_POINT ( 'NONE',  ( 3.310556943750001313, 17.50000000000001066, -31.26410580289946850 ) ) ;
#6853=VERTEX_POINT ( 'NONE', #40485 ) ;
#6854=AXIS2_PLACEMENT_3D ( 'NONE', #27279, #40454, #8118 ) ;
#6857=CARTESIAN_POINT ( 'NONE',  ( -3.500000000000002220, 15.47927405783632615, -57.87764746908817415 ) ) ;
#6858=ORIENTED_EDGE ( 'NONE', *, *, #2162, .T. ) ;
#6859=DIRECTION ( 'NONE',  ( -0.000000000000000000, 1.259100132267607459E-16, -1.000000000000000000 ) ) ;
#6861=CARTESIAN_POINT ( 'NONE',  ( 1.749999999999998224, 14.46891108675448123, -90.62764746908817415 ) ) ;
#6862=CARTESIAN_POINT ( 'NONE',  ( 3.500000000000001332, 19.52072594216370405, -31.07139747004410069 ) ) ;
#6863=CARTESIAN_POINT ( 'NONE',  ( 3.500000000000001776, 19.52072594216371826, -119.0713974700441042 ) ) ;
#6865=CARTESIAN_POINT ( 'NONE',  ( 2.340729813953370519E-16, 21.32270188528332255, -134.1016058028994564 ) ) ;
#6866=CARTESIAN_POINT ( 'NONE',  ( -1.750000000000002220, 14.46891108675447590, -28.79431413575483845 ) ) ;
#6867=EDGE_CURVE ( 'NONE', #15124, #17014, #27921, .T. ) ;
#6871=CARTESIAN_POINT ( 'NONE',  ( 1.750000000000001110, 20.53108891324555785, -118.2943141357548313 ) ) ;
#6873=CARTESIAN_POINT ( 'NONE',  ( -3.500000000000000888, 19.52072594216372181, -135.0443141357548598 ) ) ;
#6874=CARTESIAN_POINT ( 'NONE',  ( -3.310556943750002645, 15.58864905735837780, -118.6807724695661364 ) ) ;
#6877=CARTESIAN_POINT ( 'NONE',  ( 3.500000000000001776, 19.52072594216371115, -93.37764746908817415 ) ) ;
#6878=CARTESIAN_POINT ( 'NONE',  ( 2.340729813953370519E-16, 21.32270188528330834, -55.01410580289947205 ) ) ;
#6879=CARTESIAN_POINT ( 'NONE',  ( 2.340729813953370519E-16, 21.32270188528331900, -112.1016058028994706 ) ) ;
#6880=CARTESIAN_POINT ( 'NONE',  ( -3.500000000000001332, 17.50000000000002132, -121.9609808024215170 ) ) ;
#6881=CARTESIAN_POINT ( 'NONE',  ( 1.750000000000001110, 20.53108891324554719, -33.98806413671076854 ) ) ;
#6884=CARTESIAN_POINT ( 'NONE',  ( 1.655278471874998436, 14.63297358603755072, -132.5182724695661420 ) ) ;
#6886=DIRECTION ( 'NONE',  ( 0.000000000000000000, 1.000000000000000000, 0.000000000000000000 ) ) ;
#6888=CARTESIAN_POINT ( 'NONE',  ( 1.655278471874998436, 14.63297358603754184, -63.51827246956613493 ) ) ;
#6889=EDGE_CURVE ( 'NONE', #1116, #19567, #2800, .T. ) ;
#6891=CARTESIAN_POINT ( 'NONE',  ( 1.655278471874998436, 14.63297358603754184, -66.43077246956613635 ) ) ;
#6892=EDGE_LOOP ( 'NONE', ( #1173, #16846, #6235, #34621 ) ) ;
#6893=( BOUNDED_CURVE ( )  B_SPLINE_CURVE ( 2, ( #25021, #27987, #31597, #40966, #9267, #8841, #37566, #2464, #28403 ),
 .UNSPECIFIED., .F., .T. ) 
 B_SPLINE_CURVE_WITH_KNOTS ( ( 3, 2, 2, 2, 3 ),
 ( 0.9854166666666667185, 0.9861111111111111605, 0.9875000000000000444, 0.9888888888888889284, 0.9895833333333333703 ),
 .UNSPECIFIED. ) 
 CURVE ( )  GEOMETRIC_REPRESENTATION_ITEM ( )  RATIONAL_B_SPLINE_CURVE ( ( 0.9330127018922194093, 0.9330127018922194093, 1.000000000000000000, 0.8660254037844387076, 1.000000000000000000, 0.8660254037844387076, 1.000000000000000000, 0.9330127018922194093, 0.9330127018922194093 ) ) 
 REPRESENTATION_ITEM ( '' )  );
#6894=AXIS2_PLACEMENT_3D ( 'NONE', #40001, #13627, #13845 ) ;
#6895=CARTESIAN_POINT ( 'NONE',  ( 3.310556943750001313, 19.41135094264166838, -84.26827246956615625 ) ) ;
#6898=CARTESIAN_POINT ( 'NONE',  ( -3.500000000000002220, 15.47927405783633326, -103.5713974700440900 ) ) ;
#6900=CARTESIAN_POINT ( 'NONE',  ( 2.340729813953370519E-16, 21.32270188528330834, -45.01410580289947916 ) ) ;
#6902=CARTESIAN_POINT ( 'NONE',  ( 1.655278471875001101, 20.36702641396249547, -105.0974391362328078 ) ) ;
#6903=CYLINDRICAL_SURFACE ( 'NONE', #31181, 3.499999999999999556 ) ;
#6904=ORIENTED_EDGE ( 'NONE', *, *, #9654, .T. ) ;
#6905=PRODUCT_CONTEXT ( 'NONE', #2994, 'mechanical' ) ;
#6907=ORIENTED_EDGE ( 'NONE', *, *, #12642, .F. ) ;
#6909=CARTESIAN_POINT ( 'NONE',  ( 3.310556943749999981, 15.58864905735836537, -60.34743913623280065 ) ) ;
#6910=EDGE_LOOP ( 'NONE', ( #12196, #30784, #3930, #25664 ) ) ;
#6912=LINE ( 'NONE', #19889, #3570 ) ;
#6913=CARTESIAN_POINT ( 'NONE',  ( 1.750000000000001110, 20.53108891324555074, -55.29431413575484555 ) ) ;
#6916=CARTESIAN_POINT ( 'NONE',  ( -1.394453263437886604E-15, 14.00000000000002132, -114.7109808024214885 ) ) ;
#6917=ORIENTED_EDGE ( 'NONE', *, *, #17860, .F. ) ;
#6918=CARTESIAN_POINT ( 'NONE',  ( -3.500000000000002220, 15.47927405783632260, -41.87764746908817415 ) ) ;
#6919=CARTESIAN_POINT ( 'NONE',  ( -3.310556943750001313, 17.50000000000001066, -43.76410580289947916 ) ) ;
#6921=EDGE_CURVE ( 'NONE', #21133, #15247, #5172, .T. ) ;
#6922=CARTESIAN_POINT ( 'NONE',  ( -3.500000000000000000, 19.52072594216371826, -133.7380641367107614 ) ) ;
#6923=CARTESIAN_POINT ( 'NONE',  ( -1.750000000000002220, 14.46891108675448478, -102.7943141357548456 ) ) ;
#6927=CARTESIAN_POINT ( 'NONE',  ( 1.655278471875001101, 20.36702641396248481, -36.18493913623279923 ) ) ;
#6928=CARTESIAN_POINT ( 'NONE',  ( -3.310556943750002645, 15.58864905735836182, -24.76827246956612782 ) ) ;
#6929=CARTESIAN_POINT ( 'NONE',  ( -1.655278471874999990, 20.36702641396249192, -85.01827246956612782 ) ) ;
#6930=CARTESIAN_POINT ( 'NONE',  ( 1.655278471874998436, 14.63297358603755072, -133.4307724695661364 ) ) ;
#6932=CARTESIAN_POINT ( 'NONE',  ( -1.394453263437886604E-15, 14.00000000000001066, -49.40473080337742573 ) ) ;
#6934=CARTESIAN_POINT ( 'NONE',  ( -7.022189441860112050E-16, 13.67729811471672718, -129.6016058028994564 ) ) ;
#6936=CARTESIAN_POINT ( 'NONE',  ( 1.655278471874998436, 14.63297358603754539, -89.43077246956613635 ) ) ;
#6938=CARTESIAN_POINT ( 'NONE',  ( -1.394453263437886604E-15, 14.00000000000002132, -125.7109808024214885 ) ) ;
#6940=CARTESIAN_POINT ( 'NONE',  ( 3.500000000000001332, 17.50000000000001776, -76.15473080337741862 ) ) ;
#6942=CARTESIAN_POINT ( 'NONE',  ( 1.655278471875001101, 20.36702641396248836, -61.18493913623279923 ) ) ;
#6947=CARTESIAN_POINT ( 'NONE',  ( -3.310556943750002645, 15.58864905735837070, -78.76827246956614204 ) ) ;
#6948=DIRECTION ( 'NONE',  ( -0.000000000000000000, 1.259100132267607459E-16, -1.000000000000000000 ) ) ;
#6950=CARTESIAN_POINT ( 'NONE',  ( 1.655278471874998436, 14.63297358603754894, -109.4307724695661506 ) ) ;
#6951=CARTESIAN_POINT ( 'NONE',  ( 1.655278471874998436, 14.63297358603754361, -78.43077246956615056 ) ) ;
#6954=CARTESIAN_POINT ( 'NONE',  ( -1.655278471875002211, 14.63297358603754894, -100.6849391362327992 ) ) ;
#6955=CARTESIAN_POINT ( 'NONE',  ( -3.500000000000001332, 17.50000000000002132, -102.6547308033774186 ) ) ;
#6957=CARTESIAN_POINT ( 'NONE',  ( -1.394453263437886604E-15, 14.00000000000001421, -71.71098080242150274 ) ) ;
#6958=CARTESIAN_POINT ( 'NONE',  ( -1.394453263437886604E-15, 14.00000000000001776, -88.40473080337740441 ) ) ;
#6961=CARTESIAN_POINT ( 'NONE',  ( -1.655278471874999990, 20.36702641396248836, -59.93077246956614346 ) ) ;
#6963=CARTESIAN_POINT ( 'NONE',  ( 3.310556943750001313, 17.50000000000002132, -124.2641058028994649 ) ) ;
#6964=CARTESIAN_POINT ( 'NONE',  ( 1.750000000000001110, 20.53108891324554719, -36.29431413575484555 ) ) ;
#6971=CARTESIAN_POINT ( 'NONE',  ( 4.648177544792955347E-16, 21.00000000000001421, -58.90473080337742573 ) ) ;
#6972=CARTESIAN_POINT ( 'NONE',  ( 1.749999999999998224, 14.46891108675447946, -79.32139747004410424 ) ) ;
#6973=CARTESIAN_POINT ( 'NONE',  ( -3.310556943750000425, 19.41135094264166483, -75.84743913623279354 ) ) ;
#6974=ORIENTED_EDGE ( 'NONE', *, *, #29744, .F. ) ;
#6975=VERTEX_POINT ( 'NONE', #30109 ) ;
#6978=VECTOR ( 'NONE', #26878, 1000.000000000000000 ) ;
#6979=EDGE_CURVE ( 'NONE', #33859, #19669, #31865, .T. ) ;
#6982=CARTESIAN_POINT ( 'NONE',  ( 3.310556943750001313, 19.41135094264167549, -141.1807724695661364 ) ) ;
#6983=CARTESIAN_POINT ( 'NONE',  ( -1.749999999999999778, 20.53108891324555785, -129.1276474690881741 ) ) ;
#6985=CARTESIAN_POINT ( 'NONE',  ( 3.310556943750001313, 19.41135094264165772, -38.26827246956612782 ) ) ;
#6986=CARTESIAN_POINT ( 'NONE',  ( 3.310556943750001313, 19.41135094264166838, -104.2682724695661420 ) ) ;
#6987=CARTESIAN_POINT ( 'NONE',  ( -3.310556943750001313, 17.50000000000002487, -142.8516058028994564 ) ) ;
#6989=CARTESIAN_POINT ( 'NONE',  ( -1.750000000000002220, 14.46891108675448478, -102.7943141357548456 ) ) ;
#6991=CARTESIAN_POINT ( 'NONE',  ( -1.749999999999999778, 20.53108891324555785, -119.1276474690881741 ) ) ;
#6992=CARTESIAN_POINT ( 'NONE',  ( 3.500000000000001776, 19.52072594216371115, -93.07139747004409003 ) ) ;
#6993=CARTESIAN_POINT ( 'NONE',  ( 7.785697387528201340E-15, 14.00000000000002487, -136.7109808024214885 ) ) ;
#6996=CARTESIAN_POINT ( 'NONE',  ( -1.749999999999999778, 20.53108891324555074, -53.12764746908817415 ) ) ;
#6998=CARTESIAN_POINT ( 'NONE',  ( -3.500000000000002220, 15.47927405783632082, -24.87764746908817415 ) ) ;
#6999=CARTESIAN_POINT ( 'NONE',  ( -3.500000000000000888, 19.52072594216370405, -40.73806413671075433 ) ) ;
#7001=CARTESIAN_POINT ( 'NONE',  ( 3.310556943750001313, 19.41135094264166128, -29.26827246956613138 ) ) ;
#7007=CARTESIAN_POINT ( 'NONE',  ( 1.749999999999998224, 14.46891108675448478, -120.3213974700441042 ) ) ;
#7010=CARTESIAN_POINT ( 'NONE',  ( 2.340729813953370519E-16, 21.32270188528331190, -75.01410580289947916 ) ) ;
#7012=ORIENTED_EDGE ( 'NONE', *, *, #32428, .F. ) ;
#7014=VERTEX_POINT ( 'NONE', #8155 ) ;
#7016=CARTESIAN_POINT ( 'NONE',  ( 3.310556943750001313, 17.50000000000001776, -91.26410580289947916 ) ) ;
#7019=( BOUNDED_CURVE ( )  B_SPLINE_CURVE ( 2, ( #38789, #32401, #3267, #31984, #38370, #19631, #16459, #28784, #71 ),
 .UNSPECIFIED., .F., .F. ) 
 B_SPLINE_CURVE_WITH_KNOTS ( ( 3, 2, 2, 2, 3 ),
 ( 0.6437500000000000444, 0.6444444444444444864, 0.6458333333333333703, 0.6472222222222222543, 0.6479166666666666963 ),
 .UNSPECIFIED. ) 
 CURVE ( )  GEOMETRIC_REPRESENTATION_ITEM ( )  RATIONAL_B_SPLINE_CURVE ( ( 0.9330127018922194093, 0.9330127018922194093, 1.000000000000000000, 0.8660254037844387076, 1.000000000000000000, 0.8660254037844387076, 1.000000000000000000, 0.9330127018922194093, 0.9330127018922194093 ) ) 
 REPRESENTATION_ITEM ( '' )  );
#7021=ADVANCED_FACE ( 'NONE', ( #30281 ), #33896, .T. ) ;
#7025=CARTESIAN_POINT ( 'NONE',  ( 2.340729813953370519E-16, 21.32270188528331900, -128.0141058028994792 ) ) ;
#7028=CARTESIAN_POINT ( 'NONE',  ( 1.655278471875001101, 20.36702641396248836, -54.18493913623280633 ) ) ;
#7029=CARTESIAN_POINT ( 'NONE',  ( -7.022189441860112050E-16, 13.67729811471672718, -118.6016058028994706 ) ) ;
#7031=VERTEX_POINT ( 'NONE', #34101 ) ;
#7032=CARTESIAN_POINT ( 'NONE',  ( -1.750000000000002220, 14.46891108675448834, -126.4880641367107614 ) ) ;
#7034=CARTESIAN_POINT ( 'NONE',  ( 3.310556943750001313, 19.41135094264166128, -69.26827246956612782 ) ) ;
#7035=CARTESIAN_POINT ( 'NONE',  ( 1.749999999999998224, 14.46891108675448478, -115.6276474690881741 ) ) ;
#7036=CARTESIAN_POINT ( 'NONE',  ( 1.655278471875001101, 20.36702641396249192, -101.0974391362328078 ) ) ;
#7040=CARTESIAN_POINT ( 'NONE',  ( 1.749999999999998224, 14.46891108675447946, -68.62764746908817415 ) ) ;
#7041=CARTESIAN_POINT ( 'NONE',  ( -3.500000000000002220, 15.47927405783632437, -43.87764746908817415 ) ) ;
#7042=CARTESIAN_POINT ( 'NONE',  ( -3.310556943750000425, 19.41135094264165772, -39.84743913623280775 ) ) ;
#7043=CARTESIAN_POINT ( 'NONE',  ( 3.310556943749999981, 15.58864905735837070, -96.43493913623281344 ) ) ;
#7044=CARTESIAN_POINT ( 'NONE',  ( -1.750000000000002220, 14.46891108675447946, -60.48806413671076143 ) ) ;
#7046=CARTESIAN_POINT ( 'NONE',  ( 3.310556943749999981, 15.58864905735837247, -117.4349391362327850 ) ) ;
#7048=CARTESIAN_POINT ( 'NONE',  ( -3.500000000000000000, 19.52072594216370760, -61.04431413575483845 ) ) ;
#7052=CARTESIAN_POINT ( 'NONE',  ( 3.500000000000001332, 19.52072594216370760, -61.37764746908818125 ) ) ;
#7053=CARTESIAN_POINT ( 'NONE',  ( -3.310556943750001313, 17.50000000000001776, -99.76410580289947916 ) ) ;
#7054=CARTESIAN_POINT ( 'NONE',  ( -3.500000000000001332, 17.50000000000001066, -36.65473080337743284 ) ) ;
#7056=ORIENTED_EDGE ( 'NONE', *, *, #12080, .F. ) ;
#7057=CARTESIAN_POINT ( 'NONE',  ( -3.500000000000000000, 19.52072594216371115, -87.73806413671076143 ) ) ;
#7058=CARTESIAN_POINT ( 'NONE',  ( 4.648177544792955347E-16, 21.00000000000001776, -81.21098080242150274 ) ) ;
#7061=ORIENTED_EDGE ( 'NONE', *, *, #21454, .F. ) ;
#7064=CARTESIAN_POINT ( 'NONE',  ( 4.648177544792955347E-16, 21.00000000000001421, -73.90473080337743284 ) ) ;
#7066=CARTESIAN_POINT ( 'NONE',  ( 3.310556943749999981, 15.58864905735836182, -30.34743913623280775 ) ) ;
#7068=DIRECTION ( 'NONE',  ( -0.000000000000000000, 1.259100132267607459E-16, -1.000000000000000000 ) ) ;
#7069=AXIS2_PLACEMENT_3D ( 'NONE', #32226, #10518, #19660 ) ;
#7073=EDGE_CURVE ( 'NONE', #18164, #21610, #36203, .T. ) ;
#7074=ORIENTED_EDGE ( 'NONE', *, *, #41992, .F. ) ;
#7077=CARTESIAN_POINT ( 'NONE',  ( -7.022189441860112050E-16, 13.67729811471672896, -140.5141058028994792 ) ) ;
#7079=CARTESIAN_POINT ( 'NONE',  ( 4.286263797015737581E-16, 14.00000000000002487, -149.5231586289125687 ) ) ;
#7080=CARTESIAN_POINT ( 'NONE',  ( -1.655278471875002211, 14.63297358603755427, -137.6849391362327992 ) ) ;
#7081=CARTESIAN_POINT ( 'NONE',  ( 1.749999999999998224, 14.46891108675447413, -29.62764746908817770 ) ) ;
#7083=EDGE_CURVE ( 'NONE', #40297, #24209, #16358, .T. ) ;
#7088=CARTESIAN_POINT ( 'NONE',  ( -7.424026671074350129E-16, 13.45854811567264164, -131.7109808024214885 ) ) ;
#7089=CARTESIAN_POINT ( 'NONE',  ( 1.655278471875001101, 20.36702641396249547, -120.0974391362328078 ) ) ;
#7094=CARTESIAN_POINT ( 'NONE',  ( 3.500000000000001776, 19.52072594216371115, -88.37764746908817415 ) ) ;
#7095=CARTESIAN_POINT ( 'NONE',  ( -1.750000000000002220, 14.46891108675447768, -40.79431413575483845 ) ) ;
#7096=CARTESIAN_POINT ( 'NONE',  ( 3.310556943750001313, 17.50000000000001421, -51.26410580289947205 ) ) ;
#7097=CARTESIAN_POINT ( 'NONE',  ( 2.340729813953370519E-16, 21.32270188528331900, -111.1016058028994564 ) ) ;
#7099=CARTESIAN_POINT ( 'NONE',  ( -1.749999999999999778, 20.53108891324554719, -29.82139747004410069 ) ) ;
#7103=CARTESIAN_POINT ( 'NONE',  ( -3.310556943750002201, 15.58864905735837780, -134.7682724695661420 ) ) ;
#7105=LINE ( 'NONE', #10931, #220 ) ;
#7107=CARTESIAN_POINT ( 'NONE',  ( -3.310556943750002645, 15.58864905735836892, -65.76827246956611361 ) ) ;
#7109=CARTESIAN_POINT ( 'NONE',  ( 3.310556943750001313, 19.41135094264166128, -66.18077246956613635 ) ) ;
#7111=CARTESIAN_POINT ( 'NONE',  ( 3.310556943749999981, 15.58864905735836892, -83.43493913623278502 ) ) ;
#7116=CARTESIAN_POINT ( 'NONE',  ( -1.655278471874999990, 20.36702641396248836, -46.93077246956614346 ) ) ;
#7117=EDGE_CURVE ( 'NONE', #18625, #17551, #9010, .T. ) ;
#7119=CARTESIAN_POINT ( 'NONE',  ( 3.310556943749999981, 15.58864905735837070, -102.3474391362328078 ) ) ;
#7121=AXIS2_PLACEMENT_3D ( 'NONE', #32151, #3015, #38320 ) ;
#7124=ORIENTED_EDGE ( 'NONE', *, *, #11662, .T. ) ;
#7126=CARTESIAN_POINT ( 'NONE',  ( 3.310556943749999981, 15.58864905735836182, -53.34743913623280775 ) ) ;
#7130=VECTOR ( 'NONE', #30624, 1000.000000000000000 ) ;
#7136=ORIENTED_EDGE ( 'NONE', *, *, #39638, .F. ) ;
#7138=CARTESIAN_POINT ( 'NONE',  ( 3.500000000000000000, 15.47927405783632082, -41.54431413575483134 ) ) ;
#7139=CARTESIAN_POINT ( 'NONE',  ( -3.500000000000000000, 19.52072594216371826, -139.0443141357548313 ) ) ;
#7140=CARTESIAN_POINT ( 'NONE',  ( -1.750000000000002220, 14.46891108675448834, -133.4880641367107614 ) ) ;
#7142=CARTESIAN_POINT ( 'NONE',  ( -3.500000000000000000, 19.52072594216371826, -117.7380641367107614 ) ) ;
#7143=EDGE_CURVE ( 'NONE', #12093, #16494, #18322, .T. ) ;
#7145=CARTESIAN_POINT ( 'NONE',  ( -3.310556943750002645, 15.58864905735836537, -28.76827246956613848 ) ) ;
#7146=CARTESIAN_POINT ( 'NONE',  ( -3.310556943750000425, 19.41135094264165772, -24.93493913623280278 ) ) ;
#7147=CARTESIAN_POINT ( 'NONE',  ( 1.655278471875001101, 20.36702641396249192, -80.18493913623279923 ) ) ;
#7148=CARTESIAN_POINT ( 'NONE',  ( 1.655278471875001101, 20.36702641396249902, -133.0974391362328220 ) ) ;
#7152=( BOUNDED_CURVE ( )  B_SPLINE_CURVE ( 2, ( #9758, #6558, #12938, #22500, #163, #6757, #19730, #25918, #19525 ),
 .UNSPECIFIED., .F., .F. ) 
 B_SPLINE_CURVE_WITH_KNOTS ( ( 3, 2, 2, 2, 3 ),
 ( 0.8354166666666666963, 0.8361111111111111382, 0.8375000000000000222, 0.8388888888888889062, 0.8395833333333333481 ),
 .UNSPECIFIED. ) 
 CURVE ( )  GEOMETRIC_REPRESENTATION_ITEM ( )  RATIONAL_B_SPLINE_CURVE ( ( 0.9330127018922194093, 0.9330127018922194093, 1.000000000000000000, 0.8660254037844387076, 1.000000000000000000, 0.8660254037844387076, 1.000000000000000000, 0.9330127018922194093, 0.9330127018922194093 ) ) 
 REPRESENTATION_ITEM ( '' )  );
#7153=CARTESIAN_POINT ( 'NONE',  ( 2.340729813953370519E-16, 21.32270188528331900, -127.1016058028994706 ) ) ;
#7155=DIRECTION ( 'NONE',  ( 0.000000000000000000, 1.000000000000000000, 0.000000000000000000 ) ) ;
#7156=CARTESIAN_POINT ( 'NONE',  ( -3.310556943750001313, 17.50000000000001776, -83.76410580289947916 ) ) ;
#7157=CARTESIAN_POINT ( 'NONE',  ( 4.648177544792955347E-16, 21.00000000000001066, -24.21098080242150985 ) ) ;
#7158=CARTESIAN_POINT ( 'NONE',  ( 3.500000000000000000, 15.47927405783632970, -101.2380641367107756 ) ) ;
#7160=CARTESIAN_POINT ( 'NONE',  ( -7.424026671074350129E-16, 13.45854811567263454, -77.40473080337741862 ) ) ;
#7161=CARTESIAN_POINT ( 'NONE',  ( -1.655278471874999990, 20.36702641396248836, -61.01827246956613493 ) ) ;
#7165=CARTESIAN_POINT ( 'NONE',  ( -3.310556943750002645, 15.58864905735837070, -77.76827246956614204 ) ) ;
#7168=CARTESIAN_POINT ( 'NONE',  ( 2.340729813953370519E-16, 21.32270188528331900, -110.0141058028994649 ) ) ;
#7169=CARTESIAN_POINT ( 'NONE',  ( -1.655278471874999990, 20.36702641396249192, -81.93077246956615056 ) ) ;
#7170=CARTESIAN_POINT ( 'NONE',  ( 3.500000000000001332, 19.52072594216370760, -57.07139747004409713 ) ) ;
#7172=EDGE_LOOP ( 'NONE', ( #6347, #3303, #17904, #32133 ) ) ;
#7173=CARTESIAN_POINT ( 'NONE',  ( -1.655278471874999990, 20.36702641396249547, -103.0182724695661278 ) ) ;
#7174=CARTESIAN_POINT ( 'NONE',  ( 2.474675557024783212E-16, 21.54145188432740099, -101.9047308033774044 ) ) ;
#7179=CARTESIAN_POINT ( 'NONE',  ( 3.310556943750001313, 17.50000000000001421, -61.26410580289946495 ) ) ;
#7181=CARTESIAN_POINT ( 'NONE',  ( -1.655278471874999990, 20.36702641396249547, -113.9307724695661364 ) ) ;
#7182=LINE ( 'NONE', #20791, #1258 ) ;
#7183=EDGE_CURVE ( 'NONE', #34390, #3345, #16972, .T. ) ;
#7188=DIRECTION ( 'NONE',  ( -0.000000000000000000, 1.259100132267607459E-16, -1.000000000000000000 ) ) ;
#7189=DIRECTION ( 'NONE',  ( 0.000000000000000000, 1.000000000000000000, 0.000000000000000000 ) ) ;
#7190=CARTESIAN_POINT ( 'NONE',  ( -3.310556943750002645, 15.58864905735837070, -74.68077246956613635 ) ) ;
#7196=CARTESIAN_POINT ( 'NONE',  ( 3.310556943750001313, 19.41135094264167549, -133.1807724695661364 ) ) ;
#7197=CARTESIAN_POINT ( 'NONE',  ( 4.648177544792955347E-16, 21.00000000000002487, -141.2109808024214601 ) ) ;
#7199=CARTESIAN_POINT ( 'NONE',  ( 2.340729813953370519E-16, 21.32270188528330479, -44.10160580289946353 ) ) ;
#7200=CARTESIAN_POINT ( 'NONE',  ( 1.743066579297357930E-14, 14.00000000000002132, -134.7109808024214885 ) ) ;
#7201=CARTESIAN_POINT ( 'NONE',  ( 1.655278471875001101, 20.36702641396248481, -38.18493913623280633 ) ) ;
#7202=CARTESIAN_POINT ( 'NONE',  ( 3.310556943750001313, 17.50000000000001776, -98.35160580289947063 ) ) ;
#7204=EDGE_CURVE ( 'NONE', #2381, #14819, #10932, .T. ) ;
#7205=CARTESIAN_POINT ( 'NONE',  ( 1.655278471875001101, 20.36702641396248481, -26.09743913623280420 ) ) ;
#7206=CARTESIAN_POINT ( 'NONE',  ( 3.500000000000001332, 19.52072594216371826, -121.3776474690881741 ) ) ;
#7207=CARTESIAN_POINT ( 'NONE',  ( -1.749999999999999778, 20.53108891324555429, -102.1276474690881741 ) ) ;
#7209=EDGE_CURVE ( 'NONE', #30038, #5598, #4547, .T. ) ;
#7210=CARTESIAN_POINT ( 'NONE',  ( -0.9378221735089291577, 21.00000000000002132, -119.1663226036829855 ) ) ;
#7211=CARTESIAN_POINT ( 'NONE',  ( 3.500000000000001332, 17.50000000000001776, -90.15473080337743284 ) ) ;
#7215=CARTESIAN_POINT ( 'NONE',  ( -3.500000000000002220, 15.47927405783632970, -82.87764746908818836 ) ) ;
#7216=CARTESIAN_POINT ( 'NONE',  ( 1.749999999999998224, 14.46891108675447768, -54.62764746908817415 ) ) ;
#7217=CARTESIAN_POINT ( 'NONE',  ( -0.9378221735089310451, 14.00000000000001599, -73.75563900116003424 ) ) ;
#7218=CARTESIAN_POINT ( 'NONE',  ( 2.340729813953370519E-16, 21.32270188528330479, -24.01410580289947916 ) ) ;
#7219=VERTEX_POINT ( 'NONE', #12175 ) ;
#7220=CARTESIAN_POINT ( 'NONE',  ( -3.500000000000001332, 17.50000000000001066, -43.65473080337743994 ) ) ;
#7222=CARTESIAN_POINT ( 'NONE',  ( 3.310556943750001313, 19.41135094264166128, -25.26827246956613138 ) ) ;
#7223=CARTESIAN_POINT ( 'NONE',  ( -0.9378221735089310451, 14.00000000000001599, -80.44938900211593591 ) ) ;
#7226=CARTESIAN_POINT ( 'NONE',  ( -1.750000000000002220, 14.46891108675448478, -106.7943141357548456 ) ) ;
#7228=CARTESIAN_POINT ( 'NONE',  ( 3.310556943750001313, 17.50000000000001776, -76.26410580289946495 ) ) ;
#7230=ORIENTED_EDGE ( 'NONE', *, *, #19381, .F. ) ;
#7231=CARTESIAN_POINT ( 'NONE',  ( 3.500000000000000000, 15.47927405783633503, -127.2380641367107756 ) ) ;
#7233=CARTESIAN_POINT ( 'NONE',  ( 3.500000000000001332, 19.52072594216371115, -90.07139747004410424 ) ) ;
#7237=CARTESIAN_POINT ( 'NONE',  ( 3.310556943749999981, 15.58864905735836892, -91.34743913623280775 ) ) ;
#7242=DIRECTION ( 'NONE',  ( -0.000000000000000000, 1.259100132267607459E-16, -1.000000000000000000 ) ) ;
#7243=CARTESIAN_POINT ( 'NONE',  ( 3.310556943750001313, 17.50000000000002132, -127.2641058028994792 ) ) ;
#7244=CARTESIAN_POINT ( 'NONE',  ( -1.749999999999999778, 20.53108891324555429, -95.12764746908815994 ) ) ;
#7245=CARTESIAN_POINT ( 'NONE',  ( -1.655278471875002211, 14.63297358603754361, -54.68493913623280633 ) ) ;
#7246=CARTESIAN_POINT ( 'NONE',  ( -3.310556943750002645, 15.58864905735837780, -114.7682724695661278 ) ) ;
#7247=ORIENTED_EDGE ( 'NONE', *, *, #19415, .F. ) ;
#7248=ORIENTED_EDGE ( 'NONE', *, *, #21188, .F. ) ;
#7249=CARTESIAN_POINT ( 'NONE',  ( -7.424026671074350129E-16, 13.45854811567264164, -127.4047308033774470 ) ) ;
#7250=CARTESIAN_POINT ( 'NONE',  ( 1.655278471875001101, 20.36702641396248481, -39.09743913623281486 ) ) ;
#7251=CARTESIAN_POINT ( 'NONE',  ( 1.655278471875001101, 20.36702641396248836, -71.18493913623278502 ) ) ;
#7252=CARTESIAN_POINT ( 'NONE',  ( -3.500000000000002220, 15.47927405783633503, -117.8776474690881741 ) ) ;
#7253=ADVANCED_FACE ( 'NONE', ( #28753 ), #31951, .T. ) ;
#7254=CARTESIAN_POINT ( 'NONE',  ( -3.310556943750002645, 15.58864905735837425, -104.6807724695661364 ) ) ;
#7256=LINE ( 'NONE', #33190, #8924 ) ;
#7258=CARTESIAN_POINT ( 'NONE',  ( 3.500000000000001776, 19.52072594216370760, -71.37764746908817415 ) ) ;
#7259=CYLINDRICAL_SURFACE ( 'NONE', #37544, 3.499999999999999556 ) ;
#7260=CARTESIAN_POINT ( 'NONE',  ( 2.340729813953370519E-16, 21.32270188528330479, -37.01410580289946495 ) ) ;
#7261=CARTESIAN_POINT ( 'NONE',  ( 3.310556943750001313, 19.41135094264166483, -98.26827246956612782 ) ) ;
#7262=CARTESIAN_POINT ( 'NONE',  ( -1.749999999999999778, 20.53108891324555074, -61.82139747004410424 ) ) ;
#7264=CARTESIAN_POINT ( 'NONE',  ( -7.022189441860112050E-16, 13.67729811471672896, -114.6016058028994564 ) ) ;
#7265=CARTESIAN_POINT ( 'NONE',  ( 1.655278471875001101, 20.36702641396248481, -43.18493913623279212 ) ) ;
#7267=CARTESIAN_POINT ( 'NONE',  ( 4.648177544792955347E-16, 21.00000000000002132, -107.9047308033774328 ) ) ;
#7272=CARTESIAN_POINT ( 'NONE',  ( 1.750000000000001110, 20.53108891324555785, -107.2943141357548456 ) ) ;
#7273=CARTESIAN_POINT ( 'NONE',  ( 3.310556943750001313, 17.50000000000001776, -93.26410580289947916 ) ) ;
#7275=ORIENTED_EDGE ( 'NONE', *, *, #36903, .F. ) ;
#7276=( BOUNDED_CURVE ( )  B_SPLINE_CURVE ( 2, ( #347, #3130, #36071, #3744, #13325, #16320, #38642, #19289, #6938 ),
 .UNSPECIFIED., .F., .F. ) 
 B_SPLINE_CURVE_WITH_KNOTS ( ( 3, 2, 2, 2, 3 ),
 ( 0.1437499999999999889, 0.1444444444444444309, 0.1458333333333333426, 0.1472222222222222265, 0.1479166666666666685 ),
 .UNSPECIFIED. ) 
 CURVE ( )  GEOMETRIC_REPRESENTATION_ITEM ( )  RATIONAL_B_SPLINE_CURVE ( ( 0.9330127018922194093, 0.9330127018922194093, 1.000000000000000000, 0.8660254037844387076, 1.000000000000000000, 0.8660254037844387076, 1.000000000000000000, 0.9330127018922194093, 0.9330127018922194093 ) ) 
 REPRESENTATION_ITEM ( '' )  );
#7280=CARTESIAN_POINT ( 'NONE',  ( 3.500000000000001332, 19.52072594216371826, -123.0713974700441042 ) ) ;
#7281=ORIENTED_EDGE ( 'NONE', *, *, #14337, .F. ) ;
#7284=CARTESIAN_POINT ( 'NONE',  ( -1.655278471874999990, 20.36702641396248481, -29.93077246956614346 ) ) ;
#7285=EDGE_LOOP ( 'NONE', ( #40706, #27155, #22567, #15649 ) ) ;
#7291=CARTESIAN_POINT ( 'NONE',  ( -3.500000000000000000, 19.52072594216370760, -54.04431413575484555 ) ) ;
#7293=CARTESIAN_POINT ( 'NONE',  ( -3.310556943750001313, 17.50000000000002487, -142.7641058028994792 ) ) ;
#7295=CARTESIAN_POINT ( 'NONE',  ( -1.749999999999999778, 20.53108891324556140, -136.1276474690881741 ) ) ;
#7296=CARTESIAN_POINT ( 'NONE',  ( -7.022189441860112050E-16, 13.67729811471672718, -134.6016058028994564 ) ) ;
#7297=CARTESIAN_POINT ( 'NONE',  ( 3.500000000000001332, 17.50000000000001066, -29.46098080242151696 ) ) ;
#7299=CARTESIAN_POINT ( 'NONE',  ( -1.750000000000002220, 14.46891108675449011, -141.4880641367107614 ) ) ;
#7301=CARTESIAN_POINT ( 'NONE',  ( -1.750000000000002220, 14.46891108675448834, -134.7943141357548598 ) ) ;
#7302=CARTESIAN_POINT ( 'NONE',  ( 1.655278471874998436, 14.63297358603754894, -116.4307724695661364 ) ) ;
#7306=CARTESIAN_POINT ( 'NONE',  ( 3.500000000000001332, 17.50000000000001776, -86.46098080242151696 ) ) ;
#7307=CARTESIAN_POINT ( 'NONE',  ( -3.500000000000000000, 19.52072594216371115, -92.73806413671076143 ) ) ;
#7308=CARTESIAN_POINT ( 'NONE',  ( 1.655278471874998436, 14.63297358603754184, -54.43077246956613635 ) ) ;
#7309=CARTESIAN_POINT ( 'NONE',  ( -3.310556943750000425, 19.41135094264166838, -109.9349391362327992 ) ) ;
#7311=CARTESIAN_POINT ( 'NONE',  ( -1.750000000000002220, 14.46891108675447590, -29.48806413671076143 ) ) ;
#7314=CARTESIAN_POINT ( 'NONE',  ( 1.655278471874998436, 14.63297358603755072, -127.5182724695661278 ) ) ;
#7319=CARTESIAN_POINT ( 'NONE',  ( 1.655278471874998436, 14.63297358603754184, -66.51827246956612782 ) ) ;
#7321=CARTESIAN_POINT ( 'NONE',  ( -3.310556943750002645, 15.58864905735836892, -61.68077246956614346 ) ) ;
#7322=ORIENTED_EDGE ( 'NONE', *, *, #19854, .T. ) ;
#7323=CARTESIAN_POINT ( 'NONE',  ( 1.655278471874998436, 14.63297358603754539, -87.51827246956612782 ) ) ;
#7324=CARTESIAN_POINT ( 'NONE',  ( -1.394453263437886604E-15, 14.00000000000001066, -26.40473080337743284 ) ) ;
#7326=CARTESIAN_POINT ( 'NONE',  ( -1.394453263437886604E-15, 14.00000000000001776, -103.4047308033774186 ) ) ;
#7328=CARTESIAN_POINT ( 'NONE',  ( 3.310556943750001313, 19.41135094264166128, -44.18077246956614346 ) ) ;
#7330=CARTESIAN_POINT ( 'NONE',  ( 3.310556943749999981, 15.58864905735837070, -100.3474391362328220 ) ) ;
#7331=CARTESIAN_POINT ( 'NONE',  ( 3.500000000000001332, 19.52072594216370760, -53.07139747004409003 ) ) ;
#7332=EDGE_LOOP ( 'NONE', ( #24205, #39769, #38023, #32908 ) ) ;
#7334=ORIENTED_EDGE ( 'NONE', *, *, #13375, .F. ) ;
#7336=CARTESIAN_POINT ( 'NONE',  ( -3.310556943750002645, 15.58864905735836714, -52.68077246956613635 ) ) ;
#7340=CARTESIAN_POINT ( 'NONE',  ( -1.394453263437886604E-15, 14.00000000000001776, -91.40473080337741862 ) ) ;
#7342=CARTESIAN_POINT ( 'NONE',  ( 0.000000000000000000, 21.00000000000002487, -149.5231586289125687 ) ) ;
#7345=CARTESIAN_POINT ( 'NONE',  ( 1.749999999999998224, 14.46891108675447590, -43.62764746908817415 ) ) ;
#7346=( BOUNDED_CURVE ( )  B_SPLINE_CURVE ( 2, ( #21006, #33981, #30788, #1649, #18020, #30998, #14833, #27802, #9287 ),
 .UNSPECIFIED., .F., .T. ) 
 B_SPLINE_CURVE_WITH_KNOTS ( ( 3, 2, 2, 2, 3 ),
 ( 0.1979166666666666574, 0.1986111111111110994, 0.2000000000000000111, 0.2013888888888888951, 0.2020833333333333370 ),
 .UNSPECIFIED. ) 
 CURVE ( )  GEOMETRIC_REPRESENTATION_ITEM ( )  RATIONAL_B_SPLINE_CURVE ( ( 0.9330127018922194093, 0.9330127018922194093, 1.000000000000000000, 0.8660254037844387076, 1.000000000000000000, 0.8660254037844387076, 1.000000000000000000, 0.9330127018922194093, 0.9330127018922194093 ) ) 
 REPRESENTATION_ITEM ( '' )  );
#7347=CARTESIAN_POINT ( 'NONE',  ( 0.000000000000000000, 21.00000000000002487, -149.5231586289125687 ) ) ;
#7348=CARTESIAN_POINT ( 'NONE',  ( 1.750000000000001110, 20.53108891324555429, -77.98806413671076143 ) ) ;
#7350=CARTESIAN_POINT ( 'NONE',  ( 1.655278471875001101, 20.36702641396248481, -30.18493913623279568 ) ) ;
#7352=CARTESIAN_POINT ( 'NONE',  ( 1.655278471875001101, 20.36702641396249192, -83.18493913623278502 ) ) ;
#7353=CARTESIAN_POINT ( 'NONE',  ( -1.655278471874999990, 20.36702641396249902, -132.9307724695661364 ) ) ;
#7358=CARTESIAN_POINT ( 'NONE',  ( 1.655278471875001101, 20.36702641396249547, -126.1849391362327992 ) ) ;
#7359=CARTESIAN_POINT ( 'NONE',  ( 0.9378221735089281585, 14.00000000000001066, -42.66632260368298546 ) ) ;
#7360=CARTESIAN_POINT ( 'NONE',  ( -3.310556943750000425, 19.41135094264166483, -84.84743913623279354 ) ) ;
#7362=CARTESIAN_POINT ( 'NONE',  ( 4.648177544792955347E-16, 21.00000000000001776, -75.21098080242150274 ) ) ;
#7364=CARTESIAN_POINT ( 'NONE',  ( 3.500000000000000000, 15.47927405783632437, -76.23806413671077564 ) ) ;
#7365=CARTESIAN_POINT ( 'NONE',  ( -3.310556943750000425, 19.41135094264166483, -57.93493913623279212 ) ) ;
#7367=CARTESIAN_POINT ( 'NONE',  ( -3.500000000000002220, 15.47927405783632793, -67.57139747004409003 ) ) ;
#7369=CARTESIAN_POINT ( 'NONE',  ( 3.310556943750001313, 17.50000000000001776, -80.35160580289945642 ) ) ;
#7370=CARTESIAN_POINT ( 'NONE',  ( 3.310556943750001313, 19.41135094264167549, -141.2682724695661420 ) ) ;
#7372=CARTESIAN_POINT ( 'NONE',  ( 3.310556943749999981, 15.58864905735837070, -108.3474391362328078 ) ) ;
#7373=CARTESIAN_POINT ( 'NONE',  ( -3.310556943750000425, 19.41135094264166128, -73.84743913623280775 ) ) ;
#7374=ORIENTED_EDGE ( 'NONE', *, *, #10392, .T. ) ;
#7375=CARTESIAN_POINT ( 'NONE',  ( 3.310556943749999981, 15.58864905735837070, -103.4349391362327992 ) ) ;
#7376=CARTESIAN_POINT ( 'NONE',  ( 1.750000000000001110, 20.53108891324555785, -104.9880641367107614 ) ) ;
#7378=CYLINDRICAL_SURFACE ( 'NONE', #40143, 3.499999999999999556 ) ;
#7379=CARTESIAN_POINT ( 'NONE',  ( 3.500000000000001332, 17.50000000000002132, -105.1547308033774186 ) ) ;
#7382=CARTESIAN_POINT ( 'NONE',  ( -1.655278471875002211, 14.63297358603754361, -61.59743913623280775 ) ) ;
#7385=CARTESIAN_POINT ( 'NONE',  ( -1.655278471875002211, 14.63297358603755072, -115.5974391362327935 ) ) ;
#7387=EDGE_CURVE ( 'NONE', #1263, #5149, #38947, .T. ) ;
#7389=VERTEX_POINT ( 'NONE', #38338 ) ;
#7390=EDGE_CURVE ( 'NONE', #21610, #26918, #15805, .T. ) ;
#7391=ORIENTED_EDGE ( 'NONE', *, *, #38676, .F. ) ;
#7395=CARTESIAN_POINT ( 'NONE',  ( 2.340729813953370519E-16, 21.32270188528330834, -71.01410580289947916 ) ) ;
#7398=CYLINDRICAL_SURFACE ( 'NONE', #36689, 3.499999999999999556 ) ;
#7399=DIRECTION ( 'NONE',  ( 0.000000000000000000, 1.000000000000000000, 0.000000000000000000 ) ) ;
#7402=VERTEX_POINT ( 'NONE', #8572 ) ;
#7403=CARTESIAN_POINT ( 'NONE',  ( -3.310556943750001313, 17.50000000000002487, -135.7641058028994792 ) ) ;
#7406=CARTESIAN_POINT ( 'NONE',  ( 1.655278471874998436, 14.63297358603754006, -43.51827246956613493 ) ) ;
#7407=CARTESIAN_POINT ( 'NONE',  ( -7.022189441860112050E-16, 13.67729811471671475, -38.60160580289946353 ) ) ;
#7408=CARTESIAN_POINT ( 'NONE',  ( 1.655278471875001101, 20.36702641396249192, -96.18493913623279923 ) ) ;
#7412=EDGE_CURVE ( 'NONE', #34385, #4923, #11010, .T. ) ;
#7413=CARTESIAN_POINT ( 'NONE',  ( -1.655278471875002211, 14.63297358603753828, -23.59743913623281486 ) ) ;
#7415=CARTESIAN_POINT ( 'NONE',  ( -3.500000000000000888, 19.52072594216371826, -104.0443141357548456 ) ) ;
#7416=CARTESIAN_POINT ( 'NONE',  ( 3.500000000000000000, 15.47927405783633503, -124.5443141357548456 ) ) ;
#7418=CARTESIAN_POINT ( 'NONE',  ( -1.750000000000002220, 14.46891108675448301, -89.48806413671076143 ) ) ;
#7422=CARTESIAN_POINT ( 'NONE',  ( -1.394453263437886604E-15, 14.00000000000002132, -124.4047308033774044 ) ) ;
#7423=CARTESIAN_POINT ( 'NONE',  ( 3.500000000000001776, 19.52072594216370760, -55.37764746908817415 ) ) ;
#7425=FACE_OUTER_BOUND ( 'NONE', #21770, .T. ) ;
#7426=ORIENTED_EDGE ( 'NONE', *, *, #33438, .T. ) ;
#7427=AXIS2_PLACEMENT_3D ( 'NONE', #34547, #11998, #5408 ) ;
#7428=CARTESIAN_POINT ( 'NONE',  ( 1.750000000000001110, 20.53108891324554719, -45.98806413671076143 ) ) ;
#7430=CARTESIAN_POINT ( 'NONE',  ( -1.655278471875002211, 14.63297358603753828, -24.68493913623280633 ) ) ;
#7434=CARTESIAN_POINT ( 'NONE',  ( -1.749999999999999778, 20.53108891324555785, -107.1276474690881741 ) ) ;
#7436=CARTESIAN_POINT ( 'NONE',  ( -1.655278471875002211, 14.63297358603754539, -74.59743913623280775 ) ) ;
#7437=CARTESIAN_POINT ( 'NONE',  ( 0.9378221735089300459, 21.00000000000001776, -98.25563900116003424 ) ) ;
#7438=VERTEX_POINT ( 'NONE', #18778 ) ;
#7440=LINE ( 'NONE', #17013, #14907 ) ;
#7441=EDGE_CURVE ( 'NONE', #35947, #24826, #27031, .T. ) ;
#7444=CARTESIAN_POINT ( 'NONE',  ( 3.310556943749999981, 15.58864905735836892, -82.34743913623280775 ) ) ;
#7450=FACE_OUTER_BOUND ( 'NONE', #38104, .T. ) ;
#7451=CARTESIAN_POINT ( 'NONE',  ( 1.655278471875001101, 20.36702641396249547, -128.0974391362328220 ) ) ;
#7454=CARTESIAN_POINT ( 'NONE',  ( -3.310556943750002645, 15.58864905735836714, -52.76827246956612782 ) ) ;
#7455=CARTESIAN_POINT ( 'NONE',  ( -3.310556943750002645, 15.58864905735837780, -112.7682724695661278 ) ) ;
#7459=CARTESIAN_POINT ( 'NONE',  ( 3.500000000000000000, 15.47927405783633503, -126.2380641367107614 ) ) ;
#7460=EDGE_CURVE ( 'NONE', #37215, #14314, #5185, .T. ) ;
#7461=CARTESIAN_POINT ( 'NONE',  ( 3.310556943750001313, 17.50000000000001066, -39.26410580289947916 ) ) ;
#7462=CARTESIAN_POINT ( 'NONE',  ( 3.310556943750001313, 19.41135094264166128, -68.26827246956612782 ) ) ;
#7463=CARTESIAN_POINT ( 'NONE',  ( -7.424026671074350129E-16, 13.45854811567263987, -118.7109808024215027 ) ) ;
#7464=CARTESIAN_POINT ( 'NONE',  ( 3.310556943750001313, 17.50000000000002132, -102.2641058028994649 ) ) ;
#7465=CARTESIAN_POINT ( 'NONE',  ( 4.648177544792955347E-16, 21.00000000000001776, -97.90473080337743284 ) ) ;
#7469=CARTESIAN_POINT ( 'NONE',  ( 3.500000000000001776, 19.52072594216370760, -67.37764746908817415 ) ) ;
#7471=DIRECTION ( 'NONE',  ( -0.000000000000000000, 1.259100132267607459E-16, -1.000000000000000000 ) ) ;
#7472=CARTESIAN_POINT ( 'NONE',  ( -3.310556943750002645, 15.58864905735836537, -36.68077246956612925 ) ) ;
#7473=CARTESIAN_POINT ( 'NONE',  ( -3.310556943750001313, 17.50000000000001776, -94.85160580289945642 ) ) ;
#7474=CARTESIAN_POINT ( 'NONE',  ( -1.750000000000002220, 14.46891108675447946, -61.48806413671076143 ) ) ;
#7476=CARTESIAN_POINT ( 'NONE',  ( -1.655278471875002211, 14.63297358603755072, -111.6849391362327992 ) ) ;
#7477=CARTESIAN_POINT ( 'NONE',  ( 3.310556943749999981, 15.58864905735836182, -44.43493913623279212 ) ) ;
#7479=CARTESIAN_POINT ( 'NONE',  ( -1.394453263437886604E-15, 14.00000000000002132, -127.7109808024214885 ) ) ;
#7483=CARTESIAN_POINT ( 'NONE',  ( 3.500000000000000000, 15.47927405783632437, -61.54431413575483845 ) ) ;
#7484=CARTESIAN_POINT ( 'NONE',  ( 3.310556943749999981, 15.58864905735836892, -94.34743913623280775 ) ) ;
#7485=CARTESIAN_POINT ( 'NONE',  ( 0.000000000000000000, 21.00000000000002487, -149.5231586289125687 ) ) ;
#7490=LINE ( 'NONE', #20883, #40652 ) ;
#7494=CARTESIAN_POINT ( 'NONE',  ( 3.310556943749999981, 15.58864905735836182, -29.34743913623280065 ) ) ;
#7495=VERTEX_POINT ( 'NONE', #18159 ) ;
#7497=ADVANCED_FACE ( 'NONE', ( #14967 ), #30927, .T. ) ;
#7503=CARTESIAN_POINT ( 'NONE',  ( -1.394453263437886604E-15, 14.00000000000001421, -75.71098080242151696 ) ) ;
#7505=CARTESIAN_POINT ( 'NONE',  ( 1.655278471874998436, 14.63297358603755249, -141.4307724695661364 ) ) ;
#7506=CARTESIAN_POINT ( 'NONE',  ( 3.500000000000001332, 17.50000000000002132, -110.1547308033774328 ) ) ;
#7509=CARTESIAN_POINT ( 'NONE',  ( -1.655278471874999990, 20.36702641396249547, -128.0182724695661136 ) ) ;
#7510=CARTESIAN_POINT ( 'NONE',  ( -3.500000000000000888, 19.52072594216370405, -27.04431413575483845 ) ) ;
#7512=CARTESIAN_POINT ( 'NONE',  ( -3.500000000000002220, 15.47927405783633503, -142.5713974700441042 ) ) ;
#7513=AXIS2_PLACEMENT_3D ( 'NONE', #34126, #10741, #24156 ) ;
#7514=CARTESIAN_POINT ( 'NONE',  ( 3.500000000000000000, 15.47927405783633503, -123.5443141357548456 ) ) ;
#7516=CARTESIAN_POINT ( 'NONE',  ( 3.500000000000000000, 15.47927405783633503, -135.5443141357548598 ) ) ;
#7517=CARTESIAN_POINT ( 'NONE',  ( 1.655278471875001101, 20.36702641396249547, -116.0974391362327935 ) ) ;
#7520=CARTESIAN_POINT ( 'NONE',  ( 1.749999999999998224, 14.46891108675448123, -86.62764746908817415 ) ) ;
#7521=( BOUNDED_CURVE ( )  B_SPLINE_CURVE ( 2, ( #38045, #27844, #21879, #40820, #11672, #24670, #34855, #2527, #5297 ),
 .UNSPECIFIED., .F., .F. ) 
 B_SPLINE_CURVE_WITH_KNOTS ( ( 3, 2, 2, 2, 3 ),
 ( 0.1145833333333333426, 0.1152777777777777846, 0.1166666666666666685, 0.1180555555555555525, 0.1187500000000000083 ),
 .UNSPECIFIED. ) 
 CURVE ( )  GEOMETRIC_REPRESENTATION_ITEM ( )  RATIONAL_B_SPLINE_CURVE ( ( 0.9330127018922194093, 0.9330127018922200755, 1.000000000000000000, 0.8660254037844387076, 1.000000000000000000, 0.8660254037844387076, 1.000000000000000000, 0.9330127018922187432, 0.9330127018922194093 ) ) 
 REPRESENTATION_ITEM ( '' )  );
#7522=CARTESIAN_POINT ( 'NONE',  ( -1.750000000000002220, 14.46891108675448301, -92.48806413671076143 ) ) ;
#7523=CARTESIAN_POINT ( 'NONE',  ( 3.310556943750001313, 19.41135094264166128, -51.18077246956613635 ) ) ;
#7524=CARTESIAN_POINT ( 'NONE',  ( 3.310556943750001313, 19.41135094264166838, -112.2682724695661420 ) ) ;
#7529=CARTESIAN_POINT ( 'NONE',  ( -3.310556943750001313, 17.50000000000002487, -130.8516058028994564 ) ) ;
#7533=CARTESIAN_POINT ( 'NONE',  ( -7.022189441860112050E-16, 13.67729811471671830, -65.60160580289945642 ) ) ;
#7536=CARTESIAN_POINT ( 'NONE',  ( -7.022189441860112050E-16, 13.67729811471672186, -78.60160580289944221 ) ) ;
#7540=CARTESIAN_POINT ( 'NONE',  ( -3.310556943750000425, 19.41135094264166128, -44.84743913623280775 ) ) ;
#7541=CARTESIAN_POINT ( 'NONE',  ( 2.340729813953370519E-16, 21.32270188528331190, -100.0141058028994792 ) ) ;
#7542=CARTESIAN_POINT ( 'NONE',  ( 3.500000000000000000, 15.47927405783632082, -42.23806413671075433 ) ) ;
#7543=AXIS2_PLACEMENT_3D ( 'NONE', #23479, #17514, #36656 ) ;
#7546=ORIENTED_EDGE ( 'NONE', *, *, #28164, .F. ) ;
#7548=CARTESIAN_POINT ( 'NONE',  ( -3.310556943750000425, 19.41135094264166128, -54.84743913623280775 ) ) ;
#7550=ORIENTED_EDGE ( 'NONE', *, *, #3149, .T. ) ;
#7551=CARTESIAN_POINT ( 'NONE',  ( 3.500000000000001332, 19.52072594216371115, -93.37764746908817415 ) ) ;
#7554=EDGE_CURVE ( 'NONE', #3199, #32425, #41940, .T. ) ;
#7555=ORIENTED_EDGE ( 'NONE', *, *, #28286, .F. ) ;
#7557=CARTESIAN_POINT ( 'NONE',  ( -3.500000000000000888, 19.52072594216370405, -45.04431413575484555 ) ) ;
#7560=CARTESIAN_POINT ( 'NONE',  ( 0.9378221735089281585, 14.00000000000001599, -78.36007260463891555 ) ) ;
#7562=CARTESIAN_POINT ( 'NONE',  ( 3.310556943750001313, 19.41135094264165772, -27.26827246956613138 ) ) ;
#7564=CARTESIAN_POINT ( 'NONE',  ( 2.340729813953370519E-16, 21.32270188528331190, -81.10160580289945642 ) ) ;
#7565=CARTESIAN_POINT ( 'NONE',  ( 3.310556943750001313, 19.41135094264167549, -136.1807724695661364 ) ) ;
#7568=CARTESIAN_POINT ( 'NONE',  ( -1.394453263437886604E-15, 14.00000000000001421, -75.40473080337740441 ) ) ;
#7569=VECTOR ( 'NONE', #285, 1000.000000000000000 ) ;
#7571=CARTESIAN_POINT ( 'NONE',  ( 3.310556943749999981, 15.58864905735837425, -127.4349391362327992 ) ) ;
#7573=CARTESIAN_POINT ( 'NONE',  ( -1.655278471875002211, 14.63297358603754716, -87.59743913623280775 ) ) ;
#7574=CARTESIAN_POINT ( 'NONE',  ( 0.000000000000000000, 17.50000000000002487, -149.5231586289125687 ) ) ;
#7575=CARTESIAN_POINT ( 'NONE',  ( -1.394453263437886604E-15, 14.00000000000001776, -101.4047308033774186 ) ) ;
#7576=DIRECTION ( 'NONE',  ( -0.000000000000000000, 1.259100132267607459E-16, -1.000000000000000000 ) ) ;
#7577=CARTESIAN_POINT ( 'NONE',  ( -1.750000000000002220, 14.46891108675448123, -71.48806413671076143 ) ) ;
#7578=CARTESIAN_POINT ( 'NONE',  ( -1.655278471875002211, 14.63297358603754361, -55.68493913623279212 ) ) ;
#7580=CARTESIAN_POINT ( 'NONE',  ( 3.500000000000001332, 19.52072594216371826, -137.3776474690881741 ) ) ;
#7582=CARTESIAN_POINT ( 'NONE',  ( 3.310556943750001313, 19.41135094264166483, -79.26827246956612782 ) ) ;
#7583=CARTESIAN_POINT ( 'NONE',  ( 3.310556943749999981, 15.58864905735837780, -142.4349391362327708 ) ) ;
#7585=CARTESIAN_POINT ( 'NONE',  ( 3.310556943750001313, 17.50000000000002132, -107.2641058028994649 ) ) ;
#7586=CARTESIAN_POINT ( 'NONE',  ( 2.340729813953370519E-16, 21.32270188528330834, -73.01410580289947916 ) ) ;
#7587=ORIENTED_EDGE ( 'NONE', *, *, #6395, .F. ) ;
#7588=CARTESIAN_POINT ( 'NONE',  ( -3.310556943750001313, 17.50000000000001776, -95.85160580289945642 ) ) ;
#7589=CARTESIAN_POINT ( 'NONE',  ( 3.500000000000001332, 17.50000000000001776, -101.1547308033774328 ) ) ;
#7592=CARTESIAN_POINT ( 'NONE',  ( -1.394453263437886604E-15, 14.00000000000001066, -51.40473080337743284 ) ) ;
#7594=CARTESIAN_POINT ( 'NONE',  ( 3.310556943750001313, 17.50000000000001421, -59.26410580289947916 ) ) ;
#7595=CARTESIAN_POINT ( 'NONE',  ( -3.500000000000001332, 17.50000000000002132, -112.9609808024215027 ) ) ;
#7596=CARTESIAN_POINT ( 'NONE',  ( -3.310556943750000425, 19.41135094264166838, -118.8474391362327935 ) ) ;
#7597=CARTESIAN_POINT ( 'NONE',  ( 0.000000000000000000, 21.00000000000002487, -149.5231586289125687 ) ) ;
#7599=ORIENTED_EDGE ( 'NONE', *, *, #35261, .F. ) ;
#7600=ORIENTED_EDGE ( 'NONE', *, *, #31450, .T. ) ;
#7604=CARTESIAN_POINT ( 'NONE',  ( 3.310556943750001313, 19.41135094264166128, -71.18077246956613635 ) ) ;
#7605=( BOUNDED_CURVE ( )  B_SPLINE_CURVE ( 2, ( #32461, #29897, #10971, #37138, #14159, #4380, #4587, #24368, #7568 ),
 .UNSPECIFIED., .F., .T. ) 
 B_SPLINE_CURVE_WITH_KNOTS ( ( 3, 2, 2, 2, 3 ),
 ( 0.5604166666666666741, 0.5611111111111111160, 0.5625000000000000000, 0.5638888888888888840, 0.5645833333333333259 ),
 .UNSPECIFIED. ) 
 CURVE ( )  GEOMETRIC_REPRESENTATION_ITEM ( )  RATIONAL_B_SPLINE_CURVE ( ( 0.9330127018922194093, 0.9330127018922194093, 1.000000000000000000, 0.8660254037844387076, 1.000000000000000000, 0.8660254037844387076, 1.000000000000000000, 0.9330127018922194093, 0.9330127018922194093 ) ) 
 REPRESENTATION_ITEM ( '' )  );
#7606=ORIENTED_EDGE ( 'NONE', *, *, #41106, .F. ) ;
#7608=LINE ( 'NONE', #40144, #35460 ) ;
#7613=ORIENTED_EDGE ( 'NONE', *, *, #16228, .F. ) ;
#7614=DIRECTION ( 'NONE',  ( 0.000000000000000000, 1.000000000000000000, 0.000000000000000000 ) ) ;
#7615=CARTESIAN_POINT ( 'NONE',  ( -7.022189441860112050E-16, 13.67729811471672896, -135.5141058028994507 ) ) ;
#7616=CARTESIAN_POINT ( 'NONE',  ( -3.500000000000001332, 17.50000000000002487, -131.6547308033774186 ) ) ;
#7617=CARTESIAN_POINT ( 'NONE',  ( -1.655278471875002211, 14.63297358603754184, -44.68493913623279923 ) ) ;
#7619=CARTESIAN_POINT ( 'NONE',  ( 1.655278471875001101, 20.36702641396248481, -40.18493913623280633 ) ) ;
#7621=CARTESIAN_POINT ( 'NONE',  ( -1.655278471874999990, 20.36702641396249192, -101.0182724695661278 ) ) ;
#7624=CARTESIAN_POINT ( 'NONE',  ( -3.310556943750001313, 17.50000000000001066, -25.76410580289947916 ) ) ;
#7626=CARTESIAN_POINT ( 'NONE',  ( 3.500000000000001332, 17.50000000000001776, -96.46098080242150274 ) ) ;
#7629=CARTESIAN_POINT ( 'NONE',  ( 1.749999999999998224, 14.46891108675448123, -83.32139747004410424 ) ) ;
#7630=CARTESIAN_POINT ( 'NONE',  ( -3.310556943750001313, 17.50000000000001421, -67.85160580289947063 ) ) ;
#7632=CARTESIAN_POINT ( 'NONE',  ( 0.9378221735089300459, 21.00000000000001776, -83.94938900211595012 ) ) ;
#7634=CARTESIAN_POINT ( 'NONE',  ( 4.648177544792955347E-16, 21.00000000000002132, -110.2109808024215170 ) ) ;
#7635=CARTESIAN_POINT ( 'NONE',  ( 3.500000000000001332, 17.50000000000001421, -52.46098080242150985 ) ) ;
#7636=DIRECTION ( 'NONE',  ( -0.000000000000000000, 1.259100132267607459E-16, -1.000000000000000000 ) ) ;
#7637=CARTESIAN_POINT ( 'NONE',  ( -1.394453263437886604E-15, 14.00000000000001421, -79.40473080337740441 ) ) ;
#7639=EDGE_LOOP ( 'NONE', ( #38407, #25077, #30306, #16201 ) ) ;
#7640=CARTESIAN_POINT ( 'NONE',  ( 1.749999999999998224, 14.46891108675447590, -45.32139747004409713 ) ) ;
#7641=CARTESIAN_POINT ( 'NONE',  ( 0.000000000000000000, 21.00000000000002487, -149.5231586289125687 ) ) ;
#7642=CARTESIAN_POINT ( 'NONE',  ( -7.022189441860112050E-16, 13.67729811471671653, -29.60160580289947418 ) ) ;
#7644=CARTESIAN_POINT ( 'NONE',  ( -1.749999999999999778, 20.53108891324555074, -57.12764746908817415 ) ) ;
#7648=CARTESIAN_POINT ( 'NONE',  ( 3.310556943750001313, 17.50000000000001776, -79.26410580289946495 ) ) ;
#7650=ORIENTED_EDGE ( 'NONE', *, *, #19032, .F. ) ;
#7651=CARTESIAN_POINT ( 'NONE',  ( -3.500000000000002220, 15.47927405783633326, -97.87764746908815994 ) ) ;
#7653=AXIS2_PLACEMENT_3D ( 'NONE', #32399, #25614, #13048 ) ;
#7654=ORIENTED_EDGE ( 'NONE', *, *, #28872, .T. ) ;
#7655=AXIS2_PLACEMENT_3D ( 'NONE', #28254, #41239, #38038 ) ;
#7657=CARTESIAN_POINT ( 'NONE',  ( 1.655278471875001101, 20.36702641396249192, -85.09743913623279354 ) ) ;
#7658=ADVANCED_FACE ( 'NONE', ( #19147 ), #34886, .T. ) ;
#7661=ORIENTED_EDGE ( 'NONE', *, *, #37903, .F. ) ;
#7662=( BOUNDED_CURVE ( )  B_SPLINE_CURVE ( 2, ( #41904, #6157, #3183, #22743, #16171, #22112, #42109, #19135, #15738 ),
 .UNSPECIFIED., .F., .T. ) 
 B_SPLINE_CURVE_WITH_KNOTS ( ( 3, 2, 2, 2, 3 ),
 ( 0.8020833333333333703, 0.8027777777777778123, 0.8041666666666666963, 0.8055555555555555802, 0.8062500000000000222 ),
 .UNSPECIFIED. ) 
 CURVE ( )  GEOMETRIC_REPRESENTATION_ITEM ( )  RATIONAL_B_SPLINE_CURVE ( ( 0.9330127018922194093, 0.9330127018922194093, 1.000000000000000000, 0.8660254037844387076, 1.000000000000000000, 0.8660254037844387076, 1.000000000000000000, 0.9330127018922194093, 0.9330127018922194093 ) ) 
 REPRESENTATION_ITEM ( '' )  );
#7666=CARTESIAN_POINT ( 'NONE',  ( -3.310556943750002645, 15.58864905735837780, -128.6807724695661364 ) ) ;
#7667=CARTESIAN_POINT ( 'NONE',  ( -0.9378221735089310451, 14.00000000000001066, -31.44938900211594657 ) ) ;
#7668=CARTESIAN_POINT ( 'NONE',  ( -3.310556943750001313, 17.50000000000001421, -56.85160580289947063 ) ) ;
#7669=CARTESIAN_POINT ( 'NONE',  ( 2.340729813953370519E-16, 21.32270188528331900, -115.1016058028994706 ) ) ;
#7671=EDGE_CURVE ( 'NONE', #19419, #18937, #24303, .T. ) ;
#7672=CARTESIAN_POINT ( 'NONE',  ( -1.750000000000002220, 14.46891108675448834, -123.4880641367107614 ) ) ;
#7674=CARTESIAN_POINT ( 'NONE',  ( -1.655278471874999990, 20.36702641396248481, -37.93077246956613635 ) ) ;
#7675=CARTESIAN_POINT ( 'NONE',  ( -3.310556943750002645, 15.58864905735837070, -68.76827246956612782 ) ) ;
#7676=CARTESIAN_POINT ( 'NONE',  ( 3.500000000000001332, 17.50000000000002132, -119.4609808024215170 ) ) ;
#7677=CARTESIAN_POINT ( 'NONE',  ( -3.310556943750000425, 19.41135094264166483, -94.84743913623280775 ) ) ;
#7679=CARTESIAN_POINT ( 'NONE',  ( -3.500000000000001332, 17.50000000000001421, -47.65473080337742573 ) ) ;
#7681=LINE ( 'NONE', #17672, #23195 ) ;
#7682=VECTOR ( 'NONE', #36374, 1000.000000000000000 ) ;
#7684=CARTESIAN_POINT ( 'NONE',  ( 3.500000000000001332, 17.50000000000001421, -71.46098080242151696 ) ) ;
#7685=CARTESIAN_POINT ( 'NONE',  ( 1.655278471874998436, 14.63297358603753828, -31.43077246956614701 ) ) ;
#7686=CARTESIAN_POINT ( 'NONE',  ( 2.340729813953370519E-16, 21.32270188528331190, -92.10160580289947063 ) ) ;
#7687=CARTESIAN_POINT ( 'NONE',  ( -3.500000000000001332, 17.50000000000001421, -61.65473080337742573 ) ) ;
#7688=CARTESIAN_POINT ( 'NONE',  ( -0.9378221735089268263, 14.00000000000002309, -137.7556390011600627 ) ) ;
#7689=CARTESIAN_POINT ( 'NONE',  ( -3.310556943750000425, 19.41135094264166838, -111.9349391362327992 ) ) ;
#7690=CARTESIAN_POINT ( 'NONE',  ( 2.340729813953370519E-16, 21.32270188528330834, -44.10160580289946353 ) ) ;
#7692=CARTESIAN_POINT ( 'NONE',  ( -1.750000000000002220, 14.46891108675447946, -62.48806413671076143 ) ) ;
#7696=CARTESIAN_POINT ( 'NONE',  ( 3.500000000000001332, 19.52072594216371826, -107.3776474690881741 ) ) ;
#7697=CARTESIAN_POINT ( 'NONE',  ( 3.310556943750001313, 19.41135094264166838, -91.18077246956613635 ) ) ;
#7698=CARTESIAN_POINT ( 'NONE',  ( 1.750000000000001110, 20.53108891324555074, -62.29431413575483845 ) ) ;
#7703=CYLINDRICAL_SURFACE ( 'NONE', #13467, 3.499999999999999556 ) ;
#7704=ORIENTED_EDGE ( 'NONE', *, *, #4080, .F. ) ;
#7707=EDGE_CURVE ( 'NONE', #14300, #21522, #9642, .T. ) ;
#7708=ORIENTED_EDGE ( 'NONE', *, *, #6630, .F. ) ;
#7709=CARTESIAN_POINT ( 'NONE',  ( -1.394453263437886604E-15, 14.00000000000001776, -82.40473080337743284 ) ) ;
#7718=CARTESIAN_POINT ( 'NONE',  ( -3.500000000000002220, 15.47927405783632082, -27.57139747004409713 ) ) ;
#7720=CARTESIAN_POINT ( 'NONE',  ( 1.655278471875001101, 20.36702641396249902, -142.0974391362327935 ) ) ;
#7722=CARTESIAN_POINT ( 'NONE',  ( 3.500000000000001332, 19.52072594216371826, -110.0713974700441184 ) ) ;
#7723=LINE ( 'NONE', #20484, #39718 ) ;
#7724=CARTESIAN_POINT ( 'NONE',  ( 3.310556943750001313, 19.41135094264166838, -128.2682724695661136 ) ) ;
#7725=CARTESIAN_POINT ( 'NONE',  ( -7.424026671074350129E-16, 13.45854811567263098, -26.71098080242150985 ) ) ;
#7726=( BOUNDED_CURVE ( )  B_SPLINE_CURVE ( 2, ( #22940, #6774, #28898, #13576, #16779, #393, #6572, #13159, #19126 ),
 .UNSPECIFIED., .F., .T. ) 
 B_SPLINE_CURVE_WITH_KNOTS ( ( 3, 2, 2, 2, 3 ),
 ( 0.6145833333333333703, 0.6152777777777778123, 0.6166666666666666963, 0.6180555555555555802, 0.6187500000000000222 ),
 .UNSPECIFIED. ) 
 CURVE ( )  GEOMETRIC_REPRESENTATION_ITEM ( )  RATIONAL_B_SPLINE_CURVE ( ( 0.9330127018922194093, 0.9330127018922194093, 1.000000000000000000, 0.8660254037844387076, 1.000000000000000000, 0.8660254037844387076, 1.000000000000000000, 0.9330127018922194093, 0.9330127018922194093 ) ) 
 REPRESENTATION_ITEM ( '' )  );
#7728=CARTESIAN_POINT ( 'NONE',  ( 2.474675557024783212E-16, 21.54145188432740810, -142.9047308033774186 ) ) ;
#7730=CARTESIAN_POINT ( 'NONE',  ( -3.500000000000000888, 19.52072594216372181, -136.0443141357548313 ) ) ;
#7731=CARTESIAN_POINT ( 'NONE',  ( 3.310556943749999981, 15.58864905735837247, -120.3474391362328078 ) ) ;
#7734=CARTESIAN_POINT ( 'NONE',  ( -3.500000000000002220, 15.47927405783632793, -87.87764746908817415 ) ) ;
#7737=CARTESIAN_POINT ( 'NONE',  ( 1.655278471875001101, 20.36702641396248836, -52.09743913623281486 ) ) ;
#7738=CARTESIAN_POINT ( 'NONE',  ( 1.655278471875001101, 20.36702641396249547, -104.1849391362328134 ) ) ;
#7743=CARTESIAN_POINT ( 'NONE',  ( 1.655278471874998436, 14.63297358603755072, -130.5182724695661136 ) ) ;
#7746=CARTESIAN_POINT ( 'NONE',  ( 1.750000000000001110, 20.53108891324555785, -123.9880641367107614 ) ) ;
#7748=CARTESIAN_POINT ( 'NONE',  ( -1.655278471875002211, 14.63297358603754361, -64.68493913623279923 ) ) ;
#7751=CARTESIAN_POINT ( 'NONE',  ( -1.655278471874999990, 20.36702641396249192, -83.01827246956614204 ) ) ;
#7753=CARTESIAN_POINT ( 'NONE',  ( -1.394453263437886604E-15, 14.00000000000001066, -44.71098080242150985 ) ) ;
#7755=CARTESIAN_POINT ( 'NONE',  ( 4.648177544792955347E-16, 21.00000000000001421, -71.21098080242150274 ) ) ;
#7758=CARTESIAN_POINT ( 'NONE',  ( -7.022189441860112050E-16, 13.67729811471671653, -37.51410580289947205 ) ) ;
#7759=CARTESIAN_POINT ( 'NONE',  ( -3.310556943750001313, 17.50000000000001776, -98.76410580289947916 ) ) ;
#7761=ADVANCED_FACE ( 'NONE', ( #19353 ), #9798, .T. ) ;
#7766=CARTESIAN_POINT ( 'NONE',  ( 3.310556943750001313, 17.50000000000001421, -52.26410580289947205 ) ) ;
#7769=CARTESIAN_POINT ( 'NONE',  ( -0.9378221735089310451, 14.00000000000002132, -98.44938900211596433 ) ) ;
#7772=CARTESIAN_POINT ( 'NONE',  ( 1.750000000000001110, 20.53108891324555785, -113.2943141357548456 ) ) ;
#7773=ORIENTED_EDGE ( 'NONE', *, *, #17017, .F. ) ;
#7775=CARTESIAN_POINT ( 'NONE',  ( -3.500000000000002220, 15.47927405783632260, -43.87764746908817415 ) ) ;
#7776=CARTESIAN_POINT ( 'NONE',  ( -1.394453263437886604E-15, 14.00000000000000711, -23.71098080242150985 ) ) ;
#7777=CARTESIAN_POINT ( 'NONE',  ( -1.394453263437886604E-15, 14.00000000000001421, -78.40473080337741862 ) ) ;
#7778=( BOUNDED_CURVE ( )  B_SPLINE_CURVE ( 2, ( #3456, #16446, #29396, #25396, #35991, #6857, #31969, #19829, #32796 ),
 .UNSPECIFIED., .F., .T. ) 
 B_SPLINE_CURVE_WITH_KNOTS ( ( 3, 2, 2, 2, 3 ),
 ( 0.7104166666666666963, 0.7111111111111111382, 0.7125000000000000222, 0.7138888888888889062, 0.7145833333333333481 ),
 .UNSPECIFIED. ) 
 CURVE ( )  GEOMETRIC_REPRESENTATION_ITEM ( )  RATIONAL_B_SPLINE_CURVE ( ( 0.9330127018922194093, 0.9330127018922194093, 1.000000000000000000, 0.8660254037844387076, 1.000000000000000000, 0.8660254037844387076, 1.000000000000000000, 0.9330127018922194093, 0.9330127018922194093 ) ) 
 REPRESENTATION_ITEM ( '' )  );
#7781=CARTESIAN_POINT ( 'NONE',  ( -3.310556943750002645, 15.58864905735836537, -29.76827246956613493 ) ) ;
#7783=CARTESIAN_POINT ( 'NONE',  ( -1.655278471874999990, 20.36702641396249192, -82.01827246956614204 ) ) ;
#7784=CARTESIAN_POINT ( 'NONE',  ( -1.655278471875002211, 14.63297358603755249, -131.5974391362328220 ) ) ;
#7788=CARTESIAN_POINT ( 'NONE',  ( -3.310556943750001313, 17.50000000000002132, -126.8516058028994422 ) ) ;
#7789=CARTESIAN_POINT ( 'NONE',  ( 3.500000000000001332, 19.52072594216370405, -42.37764746908817415 ) ) ;
#7790=CARTESIAN_POINT ( 'NONE',  ( 3.310556943750001313, 19.41135094264166483, -85.18077246956613635 ) ) ;
#7791=CARTESIAN_POINT ( 'NONE',  ( 3.500000000000001332, 17.50000000000001066, -24.46098080242150985 ) ) ;
#7795=CARTESIAN_POINT ( 'NONE',  ( 3.500000000000000000, 15.47927405783632437, -72.23806413671076143 ) ) ;
#7796=CARTESIAN_POINT ( 'NONE',  ( -3.310556943750002201, 15.58864905735836714, -53.76827246956612782 ) ) ;
#7798=CARTESIAN_POINT ( 'NONE',  ( 3.500000000000001332, 17.50000000000002487, -137.4609808024214885 ) ) ;
#7799=CARTESIAN_POINT ( 'NONE',  ( -0.9378221735089310451, 14.00000000000001066, -48.75563900116002714 ) ) ;
#7800=CARTESIAN_POINT ( 'NONE',  ( 1.655278471874998436, 14.63297358603754539, -82.51827246956614204 ) ) ;
#7801=CARTESIAN_POINT ( 'NONE',  ( 3.310556943750001313, 19.41135094264167549, -142.2682724695661420 ) ) ;
#7803=CARTESIAN_POINT ( 'NONE',  ( 1.655278471875001101, 20.36702641396249547, -104.0974391362328220 ) ) ;
#7804=CARTESIAN_POINT ( 'NONE',  ( 1.655278471874998436, 14.63297358603754361, -77.43077246956615056 ) ) ;
#7805=CARTESIAN_POINT ( 'NONE',  ( -3.500000000000002220, 15.47927405783633503, -115.5713974700440900 ) ) ;
#7807=CARTESIAN_POINT ( 'NONE',  ( 2.340729813953370519E-16, 21.32270188528331190, -98.10160580289947063 ) ) ;
#7808=AXIS2_PLACEMENT_3D ( 'NONE', #4593, #33941, #33526 ) ;
#7811=EDGE_CURVE ( 'NONE', #41237, #16907, #22676, .T. ) ;
#7813=CARTESIAN_POINT ( 'NONE',  ( -3.310556943750002201, 15.58864905735836892, -62.68077246956614346 ) ) ;
#7814=CARTESIAN_POINT ( 'NONE',  ( -1.750000000000002220, 14.46891108675448834, -124.7943141357548456 ) ) ;
#7815=CARTESIAN_POINT ( 'NONE',  ( -1.655278471874999990, 20.36702641396249547, -115.9307724695661364 ) ) ;
#7816=CARTESIAN_POINT ( 'NONE',  ( 3.500000000000001332, 19.52072594216370405, -36.37764746908816704 ) ) ;
#7820=ORIENTED_EDGE ( 'NONE', *, *, #14633, .T. ) ;
#7823=CARTESIAN_POINT ( 'NONE',  ( 1.749999999999998224, 14.46891108675448656, -131.3213974700441042 ) ) ;
#7825=CARTESIAN_POINT ( 'NONE',  ( -3.310556943750002645, 15.58864905735837070, -70.68077246956615056 ) ) ;
#7826=ORIENTED_EDGE ( 'NONE', *, *, #22451, .F. ) ;
#7828=CARTESIAN_POINT ( 'NONE',  ( -1.749999999999999778, 20.53108891324555429, -87.12764746908817415 ) ) ;
#7829=CARTESIAN_POINT ( 'NONE',  ( 0.9378221735089281585, 14.00000000000002132, -112.3600726046389013 ) ) ;
#7832=ORIENTED_EDGE ( 'NONE', *, *, #8589, .T. ) ;
#7834=CARTESIAN_POINT ( 'NONE',  ( 3.310556943749999981, 15.58864905735837780, -137.3474391362328220 ) ) ;
#7835=CARTESIAN_POINT ( 'NONE',  ( -1.750000000000002220, 14.46891108675448656, -115.7943141357548313 ) ) ;
#7837=CARTESIAN_POINT ( 'NONE',  ( 3.310556943750001313, 19.41135094264165772, -43.26827246956613493 ) ) ;
#7839=CARTESIAN_POINT ( 'NONE',  ( -7.022189441860112050E-16, 13.67729811471671475, -34.60160580289946353 ) ) ;
#7840=CARTESIAN_POINT ( 'NONE',  ( 1.655278471874998436, 14.63297358603754716, -99.51827246956612782 ) ) ;
#7842=CARTESIAN_POINT ( 'NONE',  ( -3.310556943750000425, 19.41135094264167549, -141.9349391362327708 ) ) ;
#7843=AXIS2_PLACEMENT_3D ( 'NONE', #3753, #29485, #38651 ) ;
#7844=CARTESIAN_POINT ( 'NONE',  ( 0.000000000000000000, 17.50000000000002487, -149.5231586289125687 ) ) ;
#7845=CARTESIAN_POINT ( 'NONE',  ( -7.424026671074350129E-16, 13.45854811567263809, -96.71098080242151696 ) ) ;
#7847=EDGE_CURVE ( 'NONE', #35947, #36360, #26583, .T. ) ;
#7849=CARTESIAN_POINT ( 'NONE',  ( 3.500000000000001332, 17.50000000000001776, -84.15473080337743284 ) ) ;
#7850=CARTESIAN_POINT ( 'NONE',  ( 3.310556943750001313, 17.50000000000001421, -72.35160580289947063 ) ) ;
#7854=CARTESIAN_POINT ( 'NONE',  ( 3.500000000000000000, 15.47927405783633326, -110.5443141357548456 ) ) ;
#7855=CARTESIAN_POINT ( 'NONE',  ( 3.500000000000001332, 17.50000000000001421, -49.46098080242150274 ) ) ;
#7856=CARTESIAN_POINT ( 'NONE',  ( -1.750000000000002220, 14.46891108675447590, -30.48806413671076143 ) ) ;
#7857=CARTESIAN_POINT ( 'NONE',  ( -1.749999999999999778, 20.53108891324555429, -79.82139747004410424 ) ) ;
#7858=CARTESIAN_POINT ( 'NONE',  ( 1.750000000000001110, 20.53108891324555429, -95.29431413575484555 ) ) ;
#7860=CARTESIAN_POINT ( 'NONE',  ( -3.500000000000002220, 15.47927405783633503, -112.5713974700440900 ) ) ;
#7862=CARTESIAN_POINT ( 'NONE',  ( -1.655278471875002211, 14.63297358603753828, -23.68493913623280633 ) ) ;
#7865=ADVANCED_FACE ( 'NONE', ( #13598 ), #16182, .T. ) ;
#7868=CARTESIAN_POINT ( 'NONE',  ( 1.655278471874998436, 14.63297358603754361, -77.43077246956615056 ) ) ;
#7871=CARTESIAN_POINT ( 'NONE',  ( 1.749999999999998224, 14.46891108675447413, -27.32139747004409713 ) ) ;
#7872=EDGE_LOOP ( 'NONE', ( #7334, #5988, #4466, #28002 ) ) ;
#7873=CARTESIAN_POINT ( 'NONE',  ( -1.394453263437886604E-15, 14.00000000000001776, -88.71098080242148853 ) ) ;
#7874=CARTESIAN_POINT ( 'NONE',  ( 1.655278471875001101, 20.36702641396249192, -84.09743913623279354 ) ) ;
#7876=ORIENTED_EDGE ( 'NONE', *, *, #19615, .T. ) ;
#7879=CARTESIAN_POINT ( 'NONE',  ( -3.500000000000002220, 15.47927405783632615, -58.87764746908817415 ) ) ;
#7880=CARTESIAN_POINT ( 'NONE',  ( -1.750000000000002220, 14.46891108675448834, -126.4880641367107614 ) ) ;
#7881=CARTESIAN_POINT ( 'NONE',  ( -1.655278471875002211, 14.63297358603754361, -55.68493913623279212 ) ) ;
#7882=CARTESIAN_POINT ( 'NONE',  ( -3.310556943750000425, 19.41135094264166838, -111.9349391362327992 ) ) ;
#7883=ORIENTED_EDGE ( 'NONE', *, *, #18982, .T. ) ;
#7884=CARTESIAN_POINT ( 'NONE',  ( 2.474675557024783212E-16, 21.54145188432740099, -126.9047308033774328 ) ) ;
#7885=CARTESIAN_POINT ( 'NONE',  ( -3.310556943750002645, 15.58864905735836714, -41.68077246956614346 ) ) ;
#7886=CARTESIAN_POINT ( 'NONE',  ( -7.022189441860112050E-16, 13.67729811471672186, -67.60160580289947063 ) ) ;
#7887=CARTESIAN_POINT ( 'NONE',  ( 3.500000000000001332, 17.50000000000002132, -114.4609808024215027 ) ) ;
#7888=CARTESIAN_POINT ( 'NONE',  ( -3.310556943750000425, 19.41135094264166483, -96.84743913623282197 ) ) ;
#7889=CARTESIAN_POINT ( 'NONE',  ( 1.749999999999998224, 14.46891108675447768, -60.32139747004409713 ) ) ;
#7894=CARTESIAN_POINT ( 'NONE',  ( 3.500000000000000000, 15.47927405783632437, -70.54431413575485976 ) ) ;
#7895=DIRECTION ( 'NONE',  ( 0.000000000000000000, 1.000000000000000000, 0.000000000000000000 ) ) ;
#7896=CARTESIAN_POINT ( 'NONE',  ( 3.310556943750001313, 19.41135094264165772, -32.18077246956615056 ) ) ;
#7897=CARTESIAN_POINT ( 'NONE',  ( -1.655278471875002211, 14.63297358603754716, -89.68493913623279923 ) ) ;
#7899=CARTESIAN_POINT ( 'NONE',  ( 3.500000000000001332, 17.50000000000001421, -52.15473080337743284 ) ) ;
#7900=CARTESIAN_POINT ( 'NONE',  ( 4.648177544792955347E-16, 21.00000000000001776, -77.90473080337741862 ) ) ;
#7901=CARTESIAN_POINT ( 'NONE',  ( 2.340729813953370519E-16, 21.32270188528331900, -111.1016058028994564 ) ) ;
#7902=CARTESIAN_POINT ( 'NONE',  ( 1.655278471875001101, 20.36702641396248481, -39.18493913623280633 ) ) ;
#7904=CYLINDRICAL_SURFACE ( 'NONE', #5679, 3.499999999999999556 ) ;
#7909=CARTESIAN_POINT ( 'NONE',  ( 3.310556943750001313, 19.41135094264166838, -95.18077246956613635 ) ) ;
#7914=CARTESIAN_POINT ( 'NONE',  ( -1.394453263437886604E-15, 14.00000000000001421, -60.40473080337743284 ) ) ;
#7920=ORIENTED_EDGE ( 'NONE', *, *, #3045, .T. ) ;
#7921=EDGE_CURVE ( 'NONE', #10439, #2948, #28634, .T. ) ;
#7928=CARTESIAN_POINT ( 'NONE',  ( 4.648177544792955347E-16, 21.00000000000001776, -93.21098080242150274 ) ) ;
#7930=CARTESIAN_POINT ( 'NONE',  ( -3.310556943750001313, 17.50000000000002487, -139.7641058028994792 ) ) ;
#7931=FACE_OUTER_BOUND ( 'NONE', #16654, .T. ) ;
#7933=CARTESIAN_POINT ( 'NONE',  ( 3.310556943750001313, 19.41135094264167549, -132.2682724695661420 ) ) ;
#7934=CARTESIAN_POINT ( 'NONE',  ( -7.022189441860112050E-16, 13.67729811471671830, -54.60160580289946353 ) ) ;
#7937=CARTESIAN_POINT ( 'NONE',  ( 1.750000000000001110, 20.53108891324556140, -138.9880641367107614 ) ) ;
#7939=CARTESIAN_POINT ( 'NONE',  ( 2.474675557024783212E-16, 21.54145188432740810, -130.2109808024214885 ) ) ;
#7941=CARTESIAN_POINT ( 'NONE',  ( -3.310556943750002645, 15.58864905735837780, -110.6807724695661506 ) ) ;
#7943=CARTESIAN_POINT ( 'NONE',  ( 4.648177544792955347E-16, 21.00000000000001066, -25.90473080337743284 ) ) ;
#7944=CARTESIAN_POINT ( 'NONE',  ( -3.500000000000002220, 15.47927405783632793, -85.87764746908817415 ) ) ;
#7946=CARTESIAN_POINT ( 'NONE',  ( 3.310556943749999981, 15.58864905735836182, -49.34743913623280775 ) ) ;
#7947=EDGE_CURVE ( 'NONE', #15014, #24979, #37105, .T. ) ;
#7948=CARTESIAN_POINT ( 'NONE',  ( 3.310556943749999981, 15.58864905735837070, -104.4349391362328134 ) ) ;
#7949=CARTESIAN_POINT ( 'NONE',  ( -0.9378221735089291577, 21.00000000000001776, -83.16632260368299967 ) ) ;
#7950=CARTESIAN_POINT ( 'NONE',  ( -3.500000000000000000, 19.52072594216371115, -80.04431413575484555 ) ) ;
#7953=CARTESIAN_POINT ( 'NONE',  ( 3.310556943749999981, 15.58864905735837425, -126.4349391362327992 ) ) ;
#7956=CARTESIAN_POINT ( 'NONE',  ( 3.500000000000001332, 17.50000000000001776, -83.15473080337743284 ) ) ;
#7957=CARTESIAN_POINT ( 'NONE',  ( 4.648177544792955347E-16, 21.00000000000001421, -61.21098080242150985 ) ) ;
#7958=CARTESIAN_POINT ( 'NONE',  ( -1.655278471874999990, 20.36702641396248836, -60.01827246956613493 ) ) ;
#7960=CARTESIAN_POINT ( 'NONE',  ( -3.310556943750001313, 17.50000000000001776, -82.85160580289947063 ) ) ;
#7961=LINE ( 'NONE', #34525, #28414 ) ;
#7962=CARTESIAN_POINT ( 'NONE',  ( 3.500000000000001332, 19.52072594216370405, -44.37764746908817415 ) ) ;
#7965=CARTESIAN_POINT ( 'NONE',  ( -7.022189441860112050E-16, 13.67729811471671830, -41.51410580289947916 ) ) ;
#7966=CARTESIAN_POINT ( 'NONE',  ( -1.655278471874999990, 20.36702641396249192, -98.93077246956613635 ) ) ;
#7969=ORIENTED_EDGE ( 'NONE', *, *, #29206, .T. ) ;
#7971=CARTESIAN_POINT ( 'NONE',  ( 1.655278471874998436, 14.63297358603754006, -52.43077246956613635 ) ) ;
#7972=( BOUNDED_CURVE ( )  B_SPLINE_CURVE ( 2, ( #1009, #17998, #5017, #40747, #30342, #4608, #17587, #11206, #13977 ),
 .UNSPECIFIED., .F., .T. ) 
 B_SPLINE_CURVE_WITH_KNOTS ( ( 3, 2, 2, 2, 3 ),
 ( 0.4687500000000000000, 0.4694444444444444420, 0.4708333333333333259, 0.4722222222222222099, 0.4729166666666666519 ),
 .UNSPECIFIED. ) 
 CURVE ( )  GEOMETRIC_REPRESENTATION_ITEM ( )  RATIONAL_B_SPLINE_CURVE ( ( 0.9330127018922194093, 0.9330127018922194093, 1.000000000000000000, 0.8660254037844387076, 1.000000000000000000, 0.8660254037844387076, 1.000000000000000000, 0.9330127018922194093, 0.9330127018922194093 ) ) 
 REPRESENTATION_ITEM ( '' )  );
#7973=ORIENTED_EDGE ( 'NONE', *, *, #14532, .T. ) ;
#7976=CARTESIAN_POINT ( 'NONE',  ( 3.500000000000001332, 17.50000000000002132, -125.1547308033774328 ) ) ;
#7978=CARTESIAN_POINT ( 'NONE',  ( 3.500000000000001332, 17.50000000000002132, -113.4609808024215027 ) ) ;
#7980=ORIENTED_EDGE ( 'NONE', *, *, #182, .F. ) ;
#7981=CARTESIAN_POINT ( 'NONE',  ( -1.750000000000002220, 14.46891108675447590, -37.79431413575484555 ) ) ;
#7983=CARTESIAN_POINT ( 'NONE',  ( 1.749999999999998224, 14.46891108675448478, -119.3213974700440900 ) ) ;
#7985=CARTESIAN_POINT ( 'NONE',  ( -3.310556943750002645, 15.58864905735836537, -31.76827246956613493 ) ) ;
#7986=CARTESIAN_POINT ( 'NONE',  ( -1.655278471874999990, 20.36702641396249547, -127.9307724695661364 ) ) ;
#7989=EDGE_CURVE ( 'NONE', #14972, #18659, #9900, .T. ) ;
#7992=CARTESIAN_POINT ( 'NONE',  ( -7.022189441860112050E-16, 13.67729811471672718, -122.6016058028994706 ) ) ;
#7994=CARTESIAN_POINT ( 'NONE',  ( -3.310556943750002645, 15.58864905735837247, -87.68077246956613635 ) ) ;
#7996=CARTESIAN_POINT ( 'NONE',  ( 1.750000000000001110, 20.53108891324555074, -64.98806413671076143 ) ) ;
#7997=CARTESIAN_POINT ( 'NONE',  ( -3.310556943750002201, 15.58864905735837958, -142.7682724695661420 ) ) ;
#7998=CARTESIAN_POINT ( 'NONE',  ( 1.749999999999998224, 14.46891108675447946, -71.32139747004409003 ) ) ;
#7999=CARTESIAN_POINT ( 'NONE',  ( 3.310556943749999981, 15.58864905735836537, -56.43493913623279212 ) ) ;
#8003=CARTESIAN_POINT ( 'NONE',  ( -3.310556943750000425, 19.41135094264166483, -75.93493913623279923 ) ) ;
#8004=CARTESIAN_POINT ( 'NONE',  ( 1.655278471875001101, 20.36702641396249902, -141.1849391362327708 ) ) ;
#8006=CARTESIAN_POINT ( 'NONE',  ( -1.655278471875002211, 14.63297358603754894, -101.5974391362328078 ) ) ;
#8007=CARTESIAN_POINT ( 'NONE',  ( -7.022189441860112050E-16, 13.67729811471672186, -73.51410580289947916 ) ) ;
#8008=CARTESIAN_POINT ( 'NONE',  ( 1.655278471875001101, 20.36702641396249192, -98.18493913623279923 ) ) ;
#8010=CARTESIAN_POINT ( 'NONE',  ( 1.749999999999998224, 14.46891108675448123, -91.62764746908817415 ) ) ;
#8012=CARTESIAN_POINT ( 'NONE',  ( 3.310556943749999981, 15.58864905735836182, -53.34743913623281486 ) ) ;
#8014=CARTESIAN_POINT ( 'NONE',  ( -3.310556943750002645, 15.58864905735837780, -115.6807724695661364 ) ) ;
#8015=CARTESIAN_POINT ( 'NONE',  ( 0.9378221735089300459, 21.00000000000001066, -36.25563900116004135 ) ) ;
#8016=CARTESIAN_POINT ( 'NONE',  ( -1.394453263437886604E-15, 14.00000000000001776, -88.71098080242148853 ) ) ;
#8017=ORIENTED_EDGE ( 'NONE', *, *, #29008, .F. ) ;
#8020=ORIENTED_EDGE ( 'NONE', *, *, #12478, .T. ) ;
#8022=CARTESIAN_POINT ( 'NONE',  ( -3.310556943750001313, 17.50000000000001421, -70.76410580289947916 ) ) ;
#8028=CARTESIAN_POINT ( 'NONE',  ( -1.394453263437886604E-15, 14.00000000000002132, -112.4047308033774186 ) ) ;
#8031=EDGE_CURVE ( 'NONE', #104, #16691, #12360, .T. ) ;
#8034=CARTESIAN_POINT ( 'NONE',  ( -1.655278471875002211, 14.63297358603755427, -136.5974391362328220 ) ) ;
#8035=CARTESIAN_POINT ( 'NONE',  ( 3.310556943750001313, 19.41135094264165772, -45.26827246956613493 ) ) ;
#8036=CARTESIAN_POINT ( 'NONE',  ( -1.655278471874999990, 20.36702641396248481, -34.01827246956613493 ) ) ;
#8038=CARTESIAN_POINT ( 'NONE',  ( -3.310556943750002645, 15.58864905735837425, -99.76827246956614204 ) ) ;
#8040=CARTESIAN_POINT ( 'NONE',  ( 2.340729813953370519E-16, 21.32270188528332255, -137.1016058028994564 ) ) ;
#8041=DIRECTION ( 'NONE',  ( -0.000000000000000000, 1.259100132267607459E-16, -1.000000000000000000 ) ) ;
#8042=CARTESIAN_POINT ( 'NONE',  ( 1.749999999999998224, 14.46891108675448301, -98.62764746908817415 ) ) ;
#8043=FACE_OUTER_BOUND ( 'NONE', #20316, .T. ) ;
#8044=CARTESIAN_POINT ( 'NONE',  ( 4.648177544792955347E-16, 21.00000000000001776, -77.21098080242148853 ) ) ;
#8045=CARTESIAN_POINT ( 'NONE',  ( -1.750000000000002220, 14.46891108675448301, -85.48806413671076143 ) ) ;
#8046=CARTESIAN_POINT ( 'NONE',  ( 1.655278471874998436, 14.63297358603754361, -68.51827246956612782 ) ) ;
#8050=CARTESIAN_POINT ( 'NONE',  ( -1.394453263437886604E-15, 14.00000000000001421, -55.40473080337743284 ) ) ;
#8051=CARTESIAN_POINT ( 'NONE',  ( -1.750000000000002220, 14.46891108675447768, -46.79431413575483845 ) ) ;
#8053=CARTESIAN_POINT ( 'NONE',  ( -1.655278471874999990, 20.36702641396249547, -117.9307724695661364 ) ) ;
#8054=FACE_OUTER_BOUND ( 'NONE', #3924, .T. ) ;
#8055=CARTESIAN_POINT ( 'NONE',  ( 3.500000000000001332, 19.52072594216371115, -95.37764746908817415 ) ) ;
#8057=CARTESIAN_POINT ( 'NONE',  ( 1.750000000000001110, 20.53108891324555785, -114.9880641367107614 ) ) ;
#8060=CARTESIAN_POINT ( 'NONE',  ( 0.9378221735089281585, 14.00000000000001243, -61.36007260463890134 ) ) ;
#8063=CARTESIAN_POINT ( 'NONE',  ( -3.310556943750001313, 17.50000000000001421, -70.76410580289947916 ) ) ;
#8064=CARTESIAN_POINT ( 'NONE',  ( -3.500000000000002220, 15.47927405783633503, -133.8776474690881741 ) ) ;
#8065=DIRECTION ( 'NONE',  ( -0.000000000000000000, 1.259100132267607459E-16, -1.000000000000000000 ) ) ;
#8067=EDGE_CURVE ( 'NONE', #36297, #5958, #4162, .T. ) ;
#8068=CARTESIAN_POINT ( 'NONE',  ( -3.500000000000000000, 19.52072594216370760, -64.04431413575484555 ) ) ;
#8069=CARTESIAN_POINT ( 'NONE',  ( -1.655278471874999990, 20.36702641396249192, -82.93077246956615056 ) ) ;
#8075=CARTESIAN_POINT ( 'NONE',  ( -0.9378221735089310451, 14.00000000000002309, -126.4493890021159359 ) ) ;
#8076=CARTESIAN_POINT ( 'NONE',  ( -7.022189441860112050E-16, 13.67729811471671653, -47.60160580289946353 ) ) ;
#8078=CARTESIAN_POINT ( 'NONE',  ( -3.310556943750000425, 19.41135094264166838, -114.9349391362327992 ) ) ;
#8079=ORIENTED_EDGE ( 'NONE', *, *, #7554, .F. ) ;
#8081=CARTESIAN_POINT ( 'NONE',  ( -3.500000000000002220, 15.47927405783633503, -122.5713974700441184 ) ) ;
#8082=CARTESIAN_POINT ( 'NONE',  ( 3.310556943750001313, 19.41135094264165772, -32.18077246956615056 ) ) ;
#8083=CARTESIAN_POINT ( 'NONE',  ( -1.655278471874999990, 20.36702641396248836, -65.01827246956614204 ) ) ;
#8084=CARTESIAN_POINT ( 'NONE',  ( -3.500000000000001332, 17.50000000000002132, -112.9609808024215027 ) ) ;
#8086=CARTESIAN_POINT ( 'NONE',  ( -1.655278471874999990, 20.36702641396249192, -94.93077246956613635 ) ) ;
#8088=FACE_OUTER_BOUND ( 'NONE', #40978, .T. ) ;
#8091=CARTESIAN_POINT ( 'NONE',  ( 1.749999999999998224, 14.46891108675447768, -64.62764746908818836 ) ) ;
#8093=CARTESIAN_POINT ( 'NONE',  ( 3.310556943749999981, 15.58864905735836182, -33.34743913623280775 ) ) ;
#8094=CARTESIAN_POINT ( 'NONE',  ( 2.340729813953370519E-16, 21.32270188528331190, -89.10160580289947063 ) ) ;
#8095=CARTESIAN_POINT ( 'NONE',  ( -3.500000000000000888, 19.52072594216370760, -55.73806413671075433 ) ) ;
#8096=LINE ( 'NONE', #11691, #20589 ) ;
#8097=CARTESIAN_POINT ( 'NONE',  ( 2.340729813953370519E-16, 21.32270188528331900, -106.1016058028994564 ) ) ;
#8098=CARTESIAN_POINT ( 'NONE',  ( 3.310556943750001313, 17.50000000000001066, -35.35160580289946353 ) ) ;
#8100=CARTESIAN_POINT ( 'NONE',  ( 1.743066579297357930E-14, 14.00000000000002132, -135.7109808024214885 ) ) ;
#8104=LINE ( 'NONE', #38661, #41474 ) ;
#8105=CARTESIAN_POINT ( 'NONE',  ( 1.655278471875001101, 20.36702641396249192, -91.09743913623280775 ) ) ;
#8106=CARTESIAN_POINT ( 'NONE',  ( 3.500000000000001332, 17.50000000000002132, -117.1547308033774328 ) ) ;
#8107=ADVANCED_FACE ( 'NONE', ( #24656 ), #41234, .T. ) ;
#8113=ORIENTED_EDGE ( 'NONE', *, *, #8031, .F. ) ;
#8118=DIRECTION ( 'NONE',  ( 0.000000000000000000, 1.000000000000000000, 0.000000000000000000 ) ) ;
#8124=ORIENTED_EDGE ( 'NONE', *, *, #32265, .T. ) ;
#8125=CARTESIAN_POINT ( 'NONE',  ( -3.500000000000000000, 19.52072594216370405, -27.73806413671076143 ) ) ;
#8127=CARTESIAN_POINT ( 'NONE',  ( -1.655278471875002211, 14.63297358603755427, -138.5974391362327935 ) ) ;
#8128=CARTESIAN_POINT ( 'NONE',  ( -1.749999999999999778, 20.53108891324556140, -132.8213974700441042 ) ) ;
#8129=CARTESIAN_POINT ( 'NONE',  ( 1.749999999999998224, 14.46891108675448301, -101.6276474690881741 ) ) ;
#8130=CARTESIAN_POINT ( 'NONE',  ( 1.655278471874998436, 14.63297358603755072, -129.5182724695661136 ) ) ;
#8131=CARTESIAN_POINT ( 'NONE',  ( -3.310556943750001313, 17.50000000000001421, -53.85160580289946353 ) ) ;
#8132=VERTEX_POINT ( 'NONE', #22288 ) ;
#8134=CARTESIAN_POINT ( 'NONE',  ( -3.500000000000000888, 19.52072594216372181, -138.7380641367107330 ) ) ;
#8136=( BOUNDED_CURVE ( )  B_SPLINE_CURVE ( 2, ( #39734, #23583, #22936, #23365, #32922, #33132, #35902, #16360, #33346 ),
 .UNSPECIFIED., .F., .F. ) 
 B_SPLINE_CURVE_WITH_KNOTS ( ( 3, 2, 2, 2, 3 ),
 ( 0.8479166666666666519, 0.8486111111111110938, 0.8499999999999999778, 0.8513888888888888618, 0.8520833333333333037 ),
 .UNSPECIFIED. ) 
 CURVE ( )  GEOMETRIC_REPRESENTATION_ITEM ( )  RATIONAL_B_SPLINE_CURVE ( ( 0.9330127018922194093, 0.9330127018922194093, 1.000000000000000000, 0.8660254037844387076, 1.000000000000000000, 0.8660254037844387076, 1.000000000000000000, 0.9330127018922194093, 0.9330127018922194093 ) ) 
 REPRESENTATION_ITEM ( '' )  );
#8138=VECTOR ( 'NONE', #4509, 1000.000000000000000 ) ;
#8139=CARTESIAN_POINT ( 'NONE',  ( 1.749999999999998224, 14.46891108675448656, -126.6276474690881741 ) ) ;
#8140=CARTESIAN_POINT ( 'NONE',  ( 3.310556943750001313, 17.50000000000002132, -110.2641058028994649 ) ) ;
#8144=CARTESIAN_POINT ( 'NONE',  ( -3.500000000000001332, 17.50000000000001776, -79.96098080242150274 ) ) ;
#8145=CARTESIAN_POINT ( 'NONE',  ( 0.000000000000000000, 21.00000000000002487, -149.5231586289125687 ) ) ;
#8146=CARTESIAN_POINT ( 'NONE',  ( 2.340729813953370519E-16, 21.32270188528330834, -48.01410580289946495 ) ) ;
#8147=VECTOR ( 'NONE', #16251, 1000.000000000000000 ) ;
#8148=CARTESIAN_POINT ( 'NONE',  ( 2.340729813953370519E-16, 21.32270188528331900, -109.1016058028994564 ) ) ;
#8149=CARTESIAN_POINT ( 'NONE',  ( -1.750000000000002220, 14.46891108675448478, -99.48806413671077564 ) ) ;
#8152=CARTESIAN_POINT ( 'NONE',  ( -1.655278471875002211, 14.63297358603755249, -130.6849391362327992 ) ) ;
#8155=CARTESIAN_POINT ( 'NONE',  ( -1.394453263437886604E-15, 14.00000000000002132, -125.7109808024214885 ) ) ;
#8156=CARTESIAN_POINT ( 'NONE',  ( 0.9378221735089281585, 14.00000000000001776, -86.36007260463890134 ) ) ;
#8157=CARTESIAN_POINT ( 'NONE',  ( -3.310556943750001313, 17.50000000000001421, -58.85160580289947063 ) ) ;
#8159=CARTESIAN_POINT ( 'NONE',  ( 3.310556943750001313, 19.41135094264166838, -81.26827246956615625 ) ) ;
#8161=CARTESIAN_POINT ( 'NONE',  ( -2.324088772396477673E-16, 14.00000000000002309, -142.4047308033774186 ) ) ;
#8165=CARTESIAN_POINT ( 'NONE',  ( -1.655278471875002211, 14.63297358603754184, -40.59743913623280065 ) ) ;
#8170=CARTESIAN_POINT ( 'NONE',  ( -1.655278471875002211, 14.63297358603754184, -45.59743913623280775 ) ) ;
#8171=EDGE_CURVE ( 'NONE', #1435, #26809, #8474, .T. ) ;
#8173=ORIENTED_EDGE ( 'NONE', *, *, #40242, .T. ) ;
#8174=CARTESIAN_POINT ( 'NONE',  ( 1.750000000000001110, 20.53108891324555429, -93.29431413575484555 ) ) ;
#8176=CARTESIAN_POINT ( 'NONE',  ( 2.474675557024783212E-16, 21.54145188432739033, -24.21098080242151340 ) ) ;
#8181=CARTESIAN_POINT ( 'NONE',  ( 3.500000000000001332, 19.52072594216371826, -112.3776474690881884 ) ) ;
#8182=CARTESIAN_POINT ( 'NONE',  ( -1.749999999999999778, 20.53108891324554719, -37.12764746908817415 ) ) ;
#8184=CARTESIAN_POINT ( 'NONE',  ( -3.500000000000002220, 15.47927405783633503, -110.5713974700440900 ) ) ;
#8186=CARTESIAN_POINT ( 'NONE',  ( -3.310556943750002645, 15.58864905735836182, -24.76827246956612782 ) ) ;
#8187=CARTESIAN_POINT ( 'NONE',  ( -1.655278471875002211, 14.63297358603755249, -130.5974391362328220 ) ) ;
#8192=CARTESIAN_POINT ( 'NONE',  ( -1.655278471875002211, 14.63297358603755072, -122.6849391362327992 ) ) ;
#8193=EDGE_CURVE ( 'NONE', #31901, #23995, #25070, .T. ) ;
#8194=CARTESIAN_POINT ( 'NONE',  ( -1.394453263437886604E-15, 14.00000000000001421, -55.40473080337743284 ) ) ;
#8195=CARTESIAN_POINT ( 'NONE',  ( 3.500000000000001776, 19.52072594216370405, -40.07139747004409713 ) ) ;
#8197=CARTESIAN_POINT ( 'NONE',  ( 1.750000000000001110, 20.53108891324556140, -130.2943141357548598 ) ) ;
#8199=CARTESIAN_POINT ( 'NONE',  ( -3.500000000000000888, 19.52072594216370760, -71.73806413671076143 ) ) ;
#8200=CARTESIAN_POINT ( 'NONE',  ( -3.310556943750001313, 17.50000000000001421, -51.85160580289946353 ) ) ;
#8202=CARTESIAN_POINT ( 'NONE',  ( -1.394453263437886604E-15, 14.00000000000001421, -67.40473080337741862 ) ) ;
#8203=CARTESIAN_POINT ( 'NONE',  ( 3.310556943750001313, 17.50000000000001776, -76.35160580289945642 ) ) ;
#8205=CARTESIAN_POINT ( 'NONE',  ( -7.022189441860112050E-16, 13.67729811471672541, -101.5141058028994792 ) ) ;
#8206=CARTESIAN_POINT ( 'NONE',  ( -3.310556943750000425, 19.41135094264166483, -74.84743913623280775 ) ) ;
#8209=CARTESIAN_POINT ( 'NONE',  ( 1.655278471874998436, 14.63297358603754716, -97.51827246956612782 ) ) ;
#8211=CARTESIAN_POINT ( 'NONE',  ( 4.648177544792955347E-16, 21.00000000000001066, -33.21098080242150274 ) ) ;
#8212=CARTESIAN_POINT ( 'NONE',  ( 3.500000000000001332, 19.52072594216371826, -117.3776474690881599 ) ) ;
#8213=CARTESIAN_POINT ( 'NONE',  ( 1.655278471875001101, 20.36702641396248836, -57.09743913623280065 ) ) ;
#8214=( BOUNDED_CURVE ( )  B_SPLINE_CURVE ( 2, ( #41385, #37978, #8838, #28610, #37772, #19044, #5653, #35200, #6065 ),
 .UNSPECIFIED., .F., .F. ) 
 B_SPLINE_CURVE_WITH_KNOTS ( ( 3, 2, 2, 2, 3 ),
 ( 0.7812500000000000000, 0.7819444444444444420, 0.7833333333333333259, 0.7847222222222222099, 0.7854166666666666519 ),
 .UNSPECIFIED. ) 
 CURVE ( )  GEOMETRIC_REPRESENTATION_ITEM ( )  RATIONAL_B_SPLINE_CURVE ( ( 0.9330127018922194093, 0.9330127018922194093, 1.000000000000000000, 0.8660254037844387076, 1.000000000000000000, 0.8660254037844387076, 1.000000000000000000, 0.9330127018922194093, 0.9330127018922194093 ) ) 
 REPRESENTATION_ITEM ( '' )  );
#8216=CARTESIAN_POINT ( 'NONE',  ( 3.310556943749999981, 15.58864905735837070, -108.3474391362328078 ) ) ;
#8217=CARTESIAN_POINT ( 'NONE',  ( 3.500000000000001332, 17.50000000000001776, -84.46098080242150274 ) ) ;
#8219=VERTEX_POINT ( 'NONE', #18259 ) ;
#8221=ORIENTED_EDGE ( 'NONE', *, *, #14974, .F. ) ;
#8222=CARTESIAN_POINT ( 'NONE',  ( 1.750000000000001110, 20.53108891324554719, -33.29431413575484555 ) ) ;
#8223=CARTESIAN_POINT ( 'NONE',  ( -1.655278471874999990, 20.36702641396248836, -67.93077246956613635 ) ) ;
#8225=EDGE_LOOP ( 'NONE', ( #29602, #22292, #31502, #36638 ) ) ;
#8226=EDGE_CURVE ( 'NONE', #29607, #11168, #12292, .T. ) ;
#8229=CYLINDRICAL_SURFACE ( 'NONE', #141, 3.499999999999999556 ) ;
#8230=CARTESIAN_POINT ( 'NONE',  ( 0.000000000000000000, 21.00000000000002487, -149.5231586289125687 ) ) ;
#8234=ORIENTED_EDGE ( 'NONE', *, *, #6190, .T. ) ;
#8236=CARTESIAN_POINT ( 'NONE',  ( 2.340729813953370519E-16, 21.32270188528331900, -128.0141058028994507 ) ) ;
#8237=CARTESIAN_POINT ( 'NONE',  ( -1.394453263437886604E-15, 14.00000000000001421, -74.40473080337743284 ) ) ;
#8239=CARTESIAN_POINT ( 'NONE',  ( -3.310556943750001313, 17.50000000000001066, -37.85160580289946353 ) ) ;
#8240=CARTESIAN_POINT ( 'NONE',  ( -3.310556943750001313, 17.50000000000001066, -33.85160580289946353 ) ) ;
#8241=CARTESIAN_POINT ( 'NONE',  ( -1.655278471875002211, 14.63297358603754716, -92.68493913623279923 ) ) ;
#8242=CARTESIAN_POINT ( 'NONE',  ( 3.500000000000001332, 17.50000000000001066, -24.15473080337743284 ) ) ;
#8245=CARTESIAN_POINT ( 'NONE',  ( -1.655278471875002211, 14.63297358603755427, -138.6849391362327992 ) ) ;
#8247=CARTESIAN_POINT ( 'NONE',  ( 3.500000000000001332, 17.50000000000001776, -95.46098080242150274 ) ) ;
#8248=LINE ( 'NONE', #35034, #8272 ) ;
#8249=FACE_OUTER_BOUND ( 'NONE', #22875, .T. ) ;
#8250=CARTESIAN_POINT ( 'NONE',  ( -3.500000000000002220, 15.47927405783632793, -86.57139747004409003 ) ) ;
#8251=CARTESIAN_POINT ( 'NONE',  ( 3.310556943750001313, 17.50000000000001421, -71.35160580289947063 ) ) ;
#8253=CARTESIAN_POINT ( 'NONE',  ( -0.9378221735089291577, 21.00000000000002132, -111.8600726046389013 ) ) ;
#8255=DIRECTION ( 'NONE',  ( -0.000000000000000000, 1.259100132267607459E-16, -1.000000000000000000 ) ) ;
#8256=CARTESIAN_POINT ( 'NONE',  ( 3.500000000000001776, 19.52072594216370760, -50.37764746908818125 ) ) ;
#8257=CARTESIAN_POINT ( 'NONE',  ( 1.655278471875001101, 20.36702641396249547, -120.0974391362328078 ) ) ;
#8258=CARTESIAN_POINT ( 'NONE',  ( -4.299564228933483745E-15, 21.00000000000002842, -140.2109808024215170 ) ) ;
#8260=ADVANCED_FACE ( 'NONE', ( #28038 ), #11872, .T. ) ;
#8262=CARTESIAN_POINT ( 'NONE',  ( 1.749999999999998224, 14.46891108675448478, -115.3213974700440900 ) ) ;
#8265=CARTESIAN_POINT ( 'NONE',  ( 1.750000000000001110, 20.53108891324555429, -75.98806413671076143 ) ) ;
#8266=DIRECTION ( 'NONE',  ( 0.000000000000000000, 1.000000000000000000, 0.000000000000000000 ) ) ;
#8269=CARTESIAN_POINT ( 'NONE',  ( -1.655278471875002211, 14.63297358603754539, -72.59743913623280775 ) ) ;
#8270=CARTESIAN_POINT ( 'NONE',  ( -1.750000000000002220, 14.46891108675448478, -96.79431413575484555 ) ) ;
#8272=VECTOR ( 'NONE', #41422, 1000.000000000000000 ) ;
#8273=CARTESIAN_POINT ( 'NONE',  ( -1.394453263437886604E-15, 14.00000000000001066, -44.71098080242150985 ) ) ;
#8275=CARTESIAN_POINT ( 'NONE',  ( 3.310556943749999981, 15.58864905735836182, -26.34743913623280065 ) ) ;
#8277=CARTESIAN_POINT ( 'NONE',  ( 3.310556943750001313, 17.50000000000001776, -85.26410580289947916 ) ) ;
#8280=EDGE_CURVE ( 'NONE', #31901, #10733, #24058, .T. ) ;
#8284=CARTESIAN_POINT ( 'NONE',  ( 0.000000000000000000, 17.50000000000002487, -149.5231586289125687 ) ) ;
#8285=CARTESIAN_POINT ( 'NONE',  ( 3.310556943750001313, 19.41135094264166128, -49.26827246956613493 ) ) ;
#8286=CARTESIAN_POINT ( 'NONE',  ( 1.655278471875001101, 20.36702641396249547, -111.1849391362327992 ) ) ;
#8289=CARTESIAN_POINT ( 'NONE',  ( -1.655278471875002211, 14.63297358603754006, -33.59743913623280775 ) ) ;
#8290=CARTESIAN_POINT ( 'NONE',  ( -3.310556943750000425, 19.41135094264166128, -64.93493913623279923 ) ) ;
#8291=CARTESIAN_POINT ( 'NONE',  ( 1.749999999999998224, 14.46891108675448478, -114.6276474690881741 ) ) ;
#8293=CARTESIAN_POINT ( 'NONE',  ( 3.310556943749999981, 15.58864905735837070, -97.34743913623280775 ) ) ;
#8294=CARTESIAN_POINT ( 'NONE',  ( -0.9378221735089291577, 21.00000000000001421, -47.86007260463890844 ) ) ;
#8298=CARTESIAN_POINT ( 'NONE',  ( -3.500000000000000888, 19.52072594216370760, -63.04431413575483845 ) ) ;
#8299=CARTESIAN_POINT ( 'NONE',  ( -1.750000000000002220, 14.46891108675448123, -71.79431413575483134 ) ) ;
#8300=CARTESIAN_POINT ( 'NONE',  ( 1.655278471875001101, 20.36702641396248481, -34.09743913623280775 ) ) ;
#8301=CARTESIAN_POINT ( 'NONE',  ( -1.655278471874999990, 20.36702641396249192, -90.01827246956612782 ) ) ;
#8302=CARTESIAN_POINT ( 'NONE',  ( -7.424026671074350129E-16, 13.45854811567263454, -54.40473080337742573 ) ) ;
#8304=CARTESIAN_POINT ( 'NONE',  ( -3.310556943750002201, 15.58864905735837425, -107.7682724695661278 ) ) ;
#8305=CARTESIAN_POINT ( 'NONE',  ( 1.655278471875001101, 20.36702641396248481, -37.18493913623280633 ) ) ;
#8307=CARTESIAN_POINT ( 'NONE',  ( 1.750000000000001110, 20.53108891324556140, -135.2943141357548598 ) ) ;
#8311=CARTESIAN_POINT ( 'NONE',  ( -1.749999999999999778, 20.53108891324555074, -50.12764746908818125 ) ) ;
#8313=CARTESIAN_POINT ( 'NONE',  ( 3.310556943750001313, 19.41135094264166838, -89.18077246956613635 ) ) ;
#8314=CARTESIAN_POINT ( 'NONE',  ( 0.9378221735089455890, 14.00000000000003197, -117.3600726046389298 ) ) ;
#8316=ORIENTED_EDGE ( 'NONE', *, *, #13375, .T. ) ;
#8318=CARTESIAN_POINT ( 'NONE',  ( 0.9378221735089300459, 21.00000000000001421, -74.25563900116003424 ) ) ;
#8319=ORIENTED_EDGE ( 'NONE', *, *, #12982, .F. ) ;
#8331=ORIENTED_EDGE ( 'NONE', *, *, #20521, .T. ) ;
#8333=CARTESIAN_POINT ( 'NONE',  ( 3.310556943749999981, 15.58864905735837425, -135.3474391362328220 ) ) ;
#8335=CARTESIAN_POINT ( 'NONE',  ( 1.750000000000001110, 20.53108891324556140, -133.2943141357548598 ) ) ;
#8336=CARTESIAN_POINT ( 'NONE',  ( -1.749999999999999778, 20.53108891324555074, -63.82139747004410424 ) ) ;
#8337=CARTESIAN_POINT ( 'NONE',  ( -3.310556943750001313, 17.50000000000002132, -127.8516058028994422 ) ) ;
#8338=CARTESIAN_POINT ( 'NONE',  ( 2.340729813953370519E-16, 21.32270188528330834, -56.10160580289946353 ) ) ;
#8341=CARTESIAN_POINT ( 'NONE',  ( 1.749999999999998224, 14.46891108675448656, -135.3213974700441042 ) ) ;
#8344=CARTESIAN_POINT ( 'NONE',  ( -1.750000000000002220, 14.46891108675448834, -128.7943141357548313 ) ) ;
#8345=CARTESIAN_POINT ( 'NONE',  ( -3.310556943750001313, 17.50000000000002132, -111.7641058028994649 ) ) ;
#8349=CARTESIAN_POINT ( 'NONE',  ( 3.500000000000001776, 19.52072594216371115, -78.37764746908818836 ) ) ;
#8351=CARTESIAN_POINT ( 'NONE',  ( -1.655278471875002211, 14.63297358603754184, -46.59743913623280775 ) ) ;
#8352=CARTESIAN_POINT ( 'NONE',  ( -1.655278471874999990, 20.36702641396249547, -108.0182724695661278 ) ) ;
#8353=CARTESIAN_POINT ( 'NONE',  ( -0.9378221735089310451, 14.00000000000002309, -130.4493890021159359 ) ) ;
#8356=CARTESIAN_POINT ( 'NONE',  ( -3.310556943750001313, 17.50000000000002132, -120.8516058028994706 ) ) ;
#8359=CARTESIAN_POINT ( 'NONE',  ( -4.648177544792955347E-16, 21.00000000000002487, -142.9047308033773902 ) ) ;
#8360=CARTESIAN_POINT ( 'NONE',  ( 3.500000000000001332, 17.50000000000002487, -130.1547308033774186 ) ) ;
#8361=CARTESIAN_POINT ( 'NONE',  ( -3.310556943750002645, 15.58864905735836892, -59.76827246956613493 ) ) ;
#8362=ORIENTED_EDGE ( 'NONE', *, *, #4092, .F. ) ;
#8363=CARTESIAN_POINT ( 'NONE',  ( 1.655278471874998436, 14.63297358603754361, -80.51827246956614204 ) ) ;
#8365=CARTESIAN_POINT ( 'NONE',  ( 0.9378221735089281585, 14.00000000000001599, -77.36007260463890134 ) ) ;
#8368=CARTESIAN_POINT ( 'NONE',  ( 4.648177544792955347E-16, 21.00000000000001066, -46.21098080242150274 ) ) ;
#8372=CARTESIAN_POINT ( 'NONE',  ( -7.022189441860112050E-16, 13.67729811471671653, -39.51410580289947916 ) ) ;
#8376=ORIENTED_EDGE ( 'NONE', *, *, #20819, .T. ) ;
#8378=CARTESIAN_POINT ( 'NONE',  ( 3.310556943750001313, 17.50000000000001421, -49.26410580289947205 ) ) ;
#8379=ORIENTED_EDGE ( 'NONE', *, *, #11036, .F. ) ;
#8383=( BOUNDED_CURVE ( )  B_SPLINE_CURVE ( 2, ( #29711, #3764, #16748, #13545, #16955, #26533, #39707, #30554, #17999 ),
 .UNSPECIFIED., .F., .F. ) 
 B_SPLINE_CURVE_WITH_KNOTS ( ( 3, 2, 2, 2, 3 ),
 ( 0.8770833333333333259, 0.8777777777777777679, 0.8791666666666666519, 0.8805555555555555358, 0.8812499999999999778 ),
 .UNSPECIFIED. ) 
 CURVE ( )  GEOMETRIC_REPRESENTATION_ITEM ( )  RATIONAL_B_SPLINE_CURVE ( ( 0.9330127018922194093, 0.9330127018922194093, 1.000000000000000000, 0.8660254037844387076, 1.000000000000000000, 0.8660254037844387076, 1.000000000000000000, 0.9330127018922194093, 0.9330127018922194093 ) ) 
 REPRESENTATION_ITEM ( '' )  );
#8384=CARTESIAN_POINT ( 'NONE',  ( 3.500000000000001332, 17.50000000000001776, -97.46098080242150274 ) ) ;
#8385=CARTESIAN_POINT ( 'NONE',  ( -7.424026671074350129E-16, 13.45854811567263276, -40.71098080242150985 ) ) ;
#8386=FACE_OUTER_BOUND ( 'NONE', #30197, .T. ) ;
#8387=CARTESIAN_POINT ( 'NONE',  ( -1.749999999999999778, 20.53108891324555074, -64.82139747004410424 ) ) ;
#8390=CARTESIAN_POINT ( 'NONE',  ( 3.500000000000001776, 19.52072594216372181, -142.3776474690881741 ) ) ;
#8391=CARTESIAN_POINT ( 'NONE',  ( -0.9378221735089291577, 21.00000000000001421, -59.86007260463892266 ) ) ;
#8392=CARTESIAN_POINT ( 'NONE',  ( 3.310556943750001313, 19.41135094264166838, -126.1807724695661221 ) ) ;
#8395=CARTESIAN_POINT ( 'NONE',  ( -7.022189441860112050E-16, 13.67729811471672718, -124.6016058028994564 ) ) ;
#8397=CARTESIAN_POINT ( 'NONE',  ( 3.500000000000001776, 19.52072594216370405, -39.07139747004409713 ) ) ;
#8401=CARTESIAN_POINT ( 'NONE',  ( 3.310556943750001313, 19.41135094264167549, -138.2682724695661420 ) ) ;
#8402=CARTESIAN_POINT ( 'NONE',  ( -1.750000000000002220, 14.46891108675448123, -67.48806413671076143 ) ) ;
#8405=CARTESIAN_POINT ( 'NONE',  ( -3.310556943750001313, 17.50000000000001421, -48.85160580289946353 ) ) ;
#8407=CARTESIAN_POINT ( 'NONE',  ( -3.500000000000001332, 17.50000000000001421, -72.96098080242151696 ) ) ;
#8408=CARTESIAN_POINT ( 'NONE',  ( 2.340729813953370519E-16, 21.32270188528331190, -77.10160580289947063 ) ) ;
#8410=CARTESIAN_POINT ( 'NONE',  ( -3.310556943750000425, 19.41135094264166838, -102.8474391362328220 ) ) ;
#8411=CARTESIAN_POINT ( 'NONE',  ( 3.310556943750001313, 19.41135094264166128, -71.18077246956613635 ) ) ;
#8413=CARTESIAN_POINT ( 'NONE',  ( 3.310556943749999981, 15.58864905735837070, -98.43493913623279923 ) ) ;
#8416=CARTESIAN_POINT ( 'NONE',  ( 1.749999999999998224, 14.46891108675447590, -51.32139747004409003 ) ) ;
#8418=CARTESIAN_POINT ( 'NONE',  ( 1.655278471875001101, 20.36702641396248836, -58.09743913623280065 ) ) ;
#8420=CARTESIAN_POINT ( 'NONE',  ( 1.655278471875001101, 20.36702641396249547, -111.0974391362328078 ) ) ;
#8422=VECTOR ( 'NONE', #32379, 1000.000000000000000 ) ;
#8425=ORIENTED_EDGE ( 'NONE', *, *, #5390, .F. ) ;
#8427=CARTESIAN_POINT ( 'NONE',  ( 3.310556943750001313, 19.41135094264166128, -63.18077246956614346 ) ) ;
#8430=EDGE_CURVE ( 'NONE', #30683, #12197, #1192, .T. ) ;
#8436=( GEOMETRIC_REPRESENTATION_CONTEXT ( 3 ) GLOBAL_UNCERTAINTY_ASSIGNED_CONTEXT ( ( #19910 ) ) GLOBAL_UNIT_ASSIGNED_CONTEXT ( ( #38027, #24860, #35049 ) ) REPRESENTATION_CONTEXT ( 'NONE', 'WORKASPACE' ) );
#8438=CARTESIAN_POINT ( 'NONE',  ( -1.394453263437886604E-15, 14.00000000000001421, -54.71098080242151696 ) ) ;
#8439=CARTESIAN_POINT ( 'NONE',  ( -1.655278471875002211, 14.63297358603755249, -130.5974391362328220 ) ) ;
#8440=CARTESIAN_POINT ( 'NONE',  ( -3.500000000000000000, 19.52072594216371826, -116.0443141357548171 ) ) ;
#8441=CARTESIAN_POINT ( 'NONE',  ( -1.655278471875002211, 14.63297358603754184, -42.68493913623279212 ) ) ;
#8442=CARTESIAN_POINT ( 'NONE',  ( -7.022189441860112050E-16, 13.67729811471671475, -33.60160580289946353 ) ) ;
#8443=CARTESIAN_POINT ( 'NONE',  ( 2.340729813953370519E-16, 21.32270188528331190, -94.10160580289948484 ) ) ;
#8444=CARTESIAN_POINT ( 'NONE',  ( -3.500000000000002220, 15.47927405783632082, -25.57139747004409713 ) ) ;
#8445=ORIENTED_EDGE ( 'NONE', *, *, #24367, .T. ) ;
#8448=CARTESIAN_POINT ( 'NONE',  ( -1.655278471875002211, 14.63297358603755427, -140.6849391362327708 ) ) ;
#8449=AXIS2_PLACEMENT_3D ( 'NONE', #15690, #35035, #6100 ) ;
#8451=CARTESIAN_POINT ( 'NONE',  ( 3.500000000000001776, 19.52072594216371115, -96.37764746908815994 ) ) ;
#8452=CARTESIAN_POINT ( 'NONE',  ( -0.9378221735089310451, 14.00000000000001599, -73.44938900211595012 ) ) ;
#8453=CARTESIAN_POINT ( 'NONE',  ( 1.655278471875001101, 20.36702641396248836, -57.09743913623280065 ) ) ;
#8454=DIRECTION ( 'NONE',  ( 0.000000000000000000, 1.000000000000000000, 0.000000000000000000 ) ) ;
#8455=CARTESIAN_POINT ( 'NONE',  ( -1.749999999999999778, 20.53108891324555429, -87.82139747004409003 ) ) ;
#8456=CARTESIAN_POINT ( 'NONE',  ( 3.310556943750001313, 19.41135094264166483, -71.26827246956612782 ) ) ;
#8457=( BOUNDED_CURVE ( )  B_SPLINE_CURVE ( 2, ( #7777, #7560, #39885, #24161, #10746, #36486, #7348, #20320, #33287 ),
 .UNSPECIFIED., .F., .T. ) 
 B_SPLINE_CURVE_WITH_KNOTS ( ( 3, 2, 2, 2, 3 ),
 ( 0.5395833333333333037, 0.5402777777777777457, 0.5416666666666666297, 0.5430555555555555136, 0.5437499999999999556 ),
 .UNSPECIFIED. ) 
 CURVE ( )  GEOMETRIC_REPRESENTATION_ITEM ( )  RATIONAL_B_SPLINE_CURVE ( ( 0.9330127018922194093, 0.9330127018922194093, 1.000000000000000000, 0.8660254037844387076, 1.000000000000000000, 0.8660254037844387076, 1.000000000000000000, 0.9330127018922194093, 0.9330127018922194093 ) ) 
 REPRESENTATION_ITEM ( '' )  );
#8459=LINE ( 'NONE', #28651, #1075 ) ;
#8460=CARTESIAN_POINT ( 'NONE',  ( -1.750000000000002220, 14.46891108675447768, -47.79431413575484555 ) ) ;
#8461=CARTESIAN_POINT ( 'NONE',  ( -1.655278471874999990, 20.36702641396249547, -120.9307724695661364 ) ) ;
#8465=EDGE_CURVE ( 'NONE', #38828, #17229, #41686, .T. ) ;
#8466=CARTESIAN_POINT ( 'NONE',  ( 1.750000000000001110, 20.53108891324555785, -111.9880641367107614 ) ) ;
#8469=DIRECTION ( 'NONE',  ( -0.000000000000000000, 1.259100132267607459E-16, -1.000000000000000000 ) ) ;
#8473=CARTESIAN_POINT ( 'NONE',  ( 3.310556943750001313, 17.50000000000001421, -71.26410580289947916 ) ) ;
#8474=LINE ( 'NONE', #32069, #4307 ) ;
#8475=CYLINDRICAL_SURFACE ( 'NONE', #30511, 3.499999999999999556 ) ;
#8477=CARTESIAN_POINT ( 'NONE',  ( -3.310556943750002201, 15.58864905735836182, -24.68077246956613990 ) ) ;
#8479=CARTESIAN_POINT ( 'NONE',  ( -3.310556943750001313, 17.50000000000001776, -76.76410580289946495 ) ) ;
#8480=ORIENTED_EDGE ( 'NONE', *, *, #30839, .F. ) ;
#8481=VERTEX_POINT ( 'NONE', #23766 ) ;
#8485=CARTESIAN_POINT ( 'NONE',  ( -1.394453263437886604E-15, 14.00000000000002132, -118.7109808024215170 ) ) ;
#8488=EDGE_CURVE ( 'NONE', #10678, #23833, #3915, .T. ) ;
#8489=ORIENTED_EDGE ( 'NONE', *, *, #31575, .T. ) ;
#8491=CARTESIAN_POINT ( 'NONE',  ( -3.310556943750002645, 15.58864905735836714, -47.76827246956612782 ) ) ;
#8492=CARTESIAN_POINT ( 'NONE',  ( 1.655278471875001101, 20.36702641396249547, -109.1849391362327992 ) ) ;
#8494=CARTESIAN_POINT ( 'NONE',  ( -3.310556943750000425, 19.41135094264165772, -35.84743913623281486 ) ) ;
#8495=CARTESIAN_POINT ( 'NONE',  ( -1.655278471874999990, 20.36702641396248836, -62.01827246956613493 ) ) ;
#8496=CARTESIAN_POINT ( 'NONE',  ( 2.474675557024783212E-16, 21.54145188432740099, -114.2109808024215027 ) ) ;
#8498=CARTESIAN_POINT ( 'NONE',  ( 1.655278471874998436, 14.63297358603754716, -96.43077246956613635 ) ) ;
#8500=CARTESIAN_POINT ( 'NONE',  ( -1.750000000000002220, 14.46891108675448834, -124.4880641367107614 ) ) ;
#8501=CARTESIAN_POINT ( 'NONE',  ( -1.394453263437886604E-15, 14.00000000000001421, -56.40473080337742573 ) ) ;
#8503=CARTESIAN_POINT ( 'NONE',  ( -1.749999999999999778, 20.53108891324555074, -64.12764746908817415 ) ) ;
#8504=CARTESIAN_POINT ( 'NONE',  ( 4.648177544792955347E-16, 21.00000000000001421, -72.21098080242150274 ) ) ;
#8505=CARTESIAN_POINT ( 'NONE',  ( -3.310556943750002645, 15.58864905735836537, -32.68077246956614346 ) ) ;
#8506=( BOUNDED_CURVE ( )  B_SPLINE_CURVE ( 2, ( #37448, #18091, #37242, #8509, #1719, #27863, #36827, #7688, #20661 ),
 .UNSPECIFIED., .F., .T. ) 
 B_SPLINE_CURVE_WITH_KNOTS ( ( 3, 2, 2, 2, 3 ),
 ( 0.04375000000000000416, 0.04444444444444444614, 0.04583333333333333010, 0.04722222222222222099, 0.04791666666666666990 ),
 .UNSPECIFIED. ) 
 CURVE ( )  GEOMETRIC_REPRESENTATION_ITEM ( )  RATIONAL_B_SPLINE_CURVE ( ( 0.9330127018922192983, 0.9330127018922196314, 1.000000000000000000, 0.8660254037844387076, 1.000000000000000000, 0.8660254037844387076, 1.000000000000000000, 0.9330127018922189652, 0.9330127018922192983 ) ) 
 REPRESENTATION_ITEM ( '' )  );
#8508=CARTESIAN_POINT ( 'NONE',  ( -7.424026671074350129E-16, 13.45854811567263454, -55.40473080337743994 ) ) ;
#8509=CARTESIAN_POINT ( 'NONE',  ( -3.500000000000000000, 19.52072594216371826, -138.0443141357548598 ) ) ;
#8510=CARTESIAN_POINT ( 'NONE',  ( -1.655278471875002211, 14.63297358603754894, -107.6849391362327992 ) ) ;
#8511=CARTESIAN_POINT ( 'NONE',  ( -7.022189441860112050E-16, 13.67729811471671653, -36.60160580289946353 ) ) ;
#8513=CARTESIAN_POINT ( 'NONE',  ( 1.749999999999998224, 14.46891108675447768, -66.32139747004409003 ) ) ;
#8519=CARTESIAN_POINT ( 'NONE',  ( -3.310556943750002201, 15.58864905735837247, -85.68077246956613635 ) ) ;
#8525=AXIS2_PLACEMENT_3D ( 'NONE', #11645, #27820, #18672 ) ;
#8526=ORIENTED_EDGE ( 'NONE', *, *, #19787, .F. ) ;
#8532=VERTEX_POINT ( 'NONE', #33324 ) ;
#8541=CARTESIAN_POINT ( 'NONE',  ( 4.286263797015737581E-16, 14.00000000000002487, -149.5231586289125687 ) ) ;
#8542=CARTESIAN_POINT ( 'NONE',  ( 3.310556943750001313, 17.50000000000002487, -135.2641058028994507 ) ) ;
#8543=CARTESIAN_POINT ( 'NONE',  ( 3.500000000000000000, 15.47927405783632970, -104.2380641367107756 ) ) ;
#8547=CARTESIAN_POINT ( 'NONE',  ( 1.655278471874998436, 14.63297358603755072, -125.5182724695661278 ) ) ;
#8548=CARTESIAN_POINT ( 'NONE',  ( -3.310556943750001313, 17.50000000000001421, -56.85160580289947063 ) ) ;
#8549=ORIENTED_EDGE ( 'NONE', *, *, #7671, .F. ) ;
#8551=CARTESIAN_POINT ( 'NONE',  ( -3.500000000000000888, 19.52072594216372181, -137.7380641367107614 ) ) ;
#8554=CARTESIAN_POINT ( 'NONE',  ( -3.310556943750001313, 17.50000000000001776, -75.85160580289945642 ) ) ;
#8555=CARTESIAN_POINT ( 'NONE',  ( -1.749999999999999778, 20.53108891324555785, -126.1276474690881599 ) ) ;
#8556=CARTESIAN_POINT ( 'NONE',  ( -3.310556943750000425, 19.41135094264166838, -112.8474391362328078 ) ) ;
#8557=EDGE_CURVE ( 'NONE', #32641, #12883, #21189, .T. ) ;
#8561=CARTESIAN_POINT ( 'NONE',  ( -3.500000000000002220, 15.47927405783632615, -79.87764746908818836 ) ) ;
#8563=CARTESIAN_POINT ( 'NONE',  ( -0.9378221735089291577, 21.00000000000001421, -62.16632260368297835 ) ) ;
#8564=CARTESIAN_POINT ( 'NONE',  ( 3.310556943750001313, 17.50000000000001066, -46.26410580289947205 ) ) ;
#8565=CARTESIAN_POINT ( 'NONE',  ( 2.340729813953370519E-16, 21.32270188528331900, -105.1016058028994564 ) ) ;
#8566=CARTESIAN_POINT ( 'NONE',  ( 0.000000000000000000, 17.50000000000002487, -149.5231586289125687 ) ) ;
#8569=CARTESIAN_POINT ( 'NONE',  ( 3.310556943750001313, 19.41135094264166838, -124.2682724695661278 ) ) ;
#8572=CARTESIAN_POINT ( 'NONE',  ( 7.367361408496833051E-14, 14.00000000000001776, -93.71098080242150274 ) ) ;
#8574=CYLINDRICAL_SURFACE ( 'NONE', #218, 3.499999999999999556 ) ;
#8575=CARTESIAN_POINT ( 'NONE',  ( 2.340729813953370519E-16, 21.32270188528330834, -57.10160580289947063 ) ) ;
#8577=CARTESIAN_POINT ( 'NONE',  ( -3.310556943750000425, 19.41135094264166838, -76.93493913623278502 ) ) ;
#8580=CARTESIAN_POINT ( 'NONE',  ( -3.500000000000001332, 17.50000000000001421, -55.96098080242150985 ) ) ;
#8582=CARTESIAN_POINT ( 'NONE',  ( 3.500000000000001332, 17.50000000000001421, -74.15473080337743284 ) ) ;
#8584=CARTESIAN_POINT ( 'NONE',  ( 3.310556943750001313, 17.50000000000001066, -41.26410580289947916 ) ) ;
#8588=ORIENTED_EDGE ( 'NONE', *, *, #35404, .T. ) ;
#8589=EDGE_CURVE ( 'NONE', #11168, #4551, #14243, .T. ) ;
#8591=CARTESIAN_POINT ( 'NONE',  ( -7.022189441860112050E-16, 13.67729811471671653, -47.51410580289947205 ) ) ;
#8592=ORIENTED_EDGE ( 'NONE', *, *, #18892, .F. ) ;
#8593=VERTEX_POINT ( 'NONE', #40130 ) ;
#8595=CYLINDRICAL_SURFACE ( 'NONE', #25509, 3.499999999999999556 ) ;
#8598=CARTESIAN_POINT ( 'NONE',  ( 4.648177544792955347E-16, 21.00000000000001066, -43.21098080242150985 ) ) ;
#8599=CARTESIAN_POINT ( 'NONE',  ( -3.500000000000002220, 15.47927405783632260, -40.87764746908817415 ) ) ;
#8601=CARTESIAN_POINT ( 'NONE',  ( -3.500000000000000000, 19.52072594216371115, -77.04431413575484555 ) ) ;
#8604=CARTESIAN_POINT ( 'NONE',  ( 3.310556943749999981, 15.58864905735836182, -26.43493913623279212 ) ) ;
#8605=CARTESIAN_POINT ( 'NONE',  ( -3.500000000000002220, 15.47927405783632615, -59.57139747004409713 ) ) ;
#8606=CARTESIAN_POINT ( 'NONE',  ( 1.655278471875001101, 20.36702641396249547, -126.0974391362328078 ) ) ;
#8610=CARTESIAN_POINT ( 'NONE',  ( 3.500000000000001332, 19.52072594216371115, -94.07139747004409003 ) ) ;
#8611=CARTESIAN_POINT ( 'NONE',  ( 1.655278471875001101, 20.36702641396249547, -120.1849391362327992 ) ) ;
#8612=CARTESIAN_POINT ( 'NONE',  ( 2.474675557024783212E-16, 21.54145188432739033, -36.90473080337743284 ) ) ;
#8615=CARTESIAN_POINT ( 'NONE',  ( 1.655278471874998436, 14.63297358603755249, -137.5182724695661420 ) ) ;
#8616=CARTESIAN_POINT ( 'NONE',  ( 4.648177544792955347E-16, 21.00000000000001066, -29.21098080242150630 ) ) ;
#8617=CARTESIAN_POINT ( 'NONE',  ( 3.310556943750001313, 19.41135094264166483, -48.26827246956613493 ) ) ;
#8619=CARTESIAN_POINT ( 'NONE',  ( -3.500000000000000000, 19.52072594216371826, -114.7380641367107614 ) ) ;
#8620=CARTESIAN_POINT ( 'NONE',  ( 2.340729813953370519E-16, 21.32270188528331190, -75.10160580289947063 ) ) ;
#8622=CARTESIAN_POINT ( 'NONE',  ( 3.310556943750001313, 19.41135094264166838, -102.1807724695661364 ) ) ;
#8623=CARTESIAN_POINT ( 'NONE',  ( 2.340729813953370519E-16, 21.32270188528330834, -71.01410580289947916 ) ) ;
#8625=CARTESIAN_POINT ( 'NONE',  ( -1.655278471875002211, 14.63297358603754716, -89.68493913623279923 ) ) ;
#8627=CARTESIAN_POINT ( 'NONE',  ( -1.394453263437886604E-15, 14.00000000000001776, -107.7109808024215170 ) ) ;
#8630=CARTESIAN_POINT ( 'NONE',  ( -7.022189441860112050E-16, 13.67729811471672186, -57.51410580289947916 ) ) ;
#8631=CARTESIAN_POINT ( 'NONE',  ( -0.9378221735089268263, 14.00000000000002309, -137.4493890021159928 ) ) ;
#8632=CARTESIAN_POINT ( 'NONE',  ( -1.655278471874999990, 20.36702641396249547, -110.9307724695661506 ) ) ;
#8633=CARTESIAN_POINT ( 'NONE',  ( 4.648177544792955347E-16, 21.00000000000001776, -101.9047308033774186 ) ) ;
#8635=( BOUNDED_CURVE ( )  B_SPLINE_CURVE ( 2, ( #22584, #38329, #35559, #6421, #15584, #9192, #21954, #41531, #12384 ),
 .UNSPECIFIED., .F., .T. ) 
 B_SPLINE_CURVE_WITH_KNOTS ( ( 3, 2, 2, 2, 3 ),
 ( 0.2437499999999999944, 0.2444444444444444364, 0.2458333333333333204, 0.2472222222222222321, 0.2479166666666666741 ),
 .UNSPECIFIED. ) 
 CURVE ( )  GEOMETRIC_REPRESENTATION_ITEM ( )  RATIONAL_B_SPLINE_CURVE ( ( 0.9330127018922194093, 0.9330127018922194093, 1.000000000000000000, 0.8660254037844387076, 1.000000000000000000, 0.8660254037844387076, 1.000000000000000000, 0.9330127018922194093, 0.9330127018922194093 ) ) 
 REPRESENTATION_ITEM ( '' )  );
#8640=CARTESIAN_POINT ( 'NONE',  ( 1.655278471874998436, 14.63297358603754184, -63.43077246956614346 ) ) ;
#8644=FACE_OUTER_BOUND ( 'NONE', #6562, .T. ) ;
#8646=CARTESIAN_POINT ( 'NONE',  ( 4.648177544792955347E-16, 21.00000000000001421, -48.90473080337742573 ) ) ;
#8647=ORIENTED_EDGE ( 'NONE', *, *, #21452, .T. ) ;
#8649=CARTESIAN_POINT ( 'NONE',  ( 3.310556943749999981, 15.58864905735837425, -130.3474391362328220 ) ) ;
#8650=CARTESIAN_POINT ( 'NONE',  ( -0.9378221735089640188, 21.00000000000000000, -103.1663226036829855 ) ) ;
#8651=CARTESIAN_POINT ( 'NONE',  ( 1.655278471874998436, 14.63297358603753828, -39.51827246956612782 ) ) ;
#8652=CARTESIAN_POINT ( 'NONE',  ( 2.340729813953370519E-16, 21.32270188528330479, -35.10160580289946353 ) ) ;
#8653=CARTESIAN_POINT ( 'NONE',  ( -3.310556943750002645, 15.58864905735837247, -91.76827246956615625 ) ) ;
#8654=CARTESIAN_POINT ( 'NONE',  ( 1.750000000000001110, 20.53108891324554719, -23.98806413671077209 ) ) ;
#8655=ORIENTED_EDGE ( 'NONE', *, *, #19615, .F. ) ;
#8657=CARTESIAN_POINT ( 'NONE',  ( -1.655278471875002211, 14.63297358603755427, -137.6849391362327992 ) ) ;
#8659=CARTESIAN_POINT ( 'NONE',  ( 0.9378221735089300459, 21.00000000000001776, -86.94938900211596433 ) ) ;
#8660=CARTESIAN_POINT ( 'NONE',  ( -1.655278471874999990, 20.36702641396248836, -58.93077246956614346 ) ) ;
#8661=CARTESIAN_POINT ( 'NONE',  ( -1.394453263437886604E-15, 14.00000000000002132, -122.4047308033774044 ) ) ;
#8662=CARTESIAN_POINT ( 'NONE',  ( -7.424026671074350129E-16, 13.45854811567263631, -82.40473080337743284 ) ) ;
#8663=CARTESIAN_POINT ( 'NONE',  ( -3.310556943750002201, 15.58864905735836892, -64.76827246956614204 ) ) ;
#8667=ORIENTED_EDGE ( 'NONE', *, *, #31643, .T. ) ;
#8668=CARTESIAN_POINT ( 'NONE',  ( -3.310556943750002201, 15.58864905735837780, -121.6807724695661364 ) ) ;
#8669=CARTESIAN_POINT ( 'NONE',  ( 4.286263797015737581E-16, 14.00000000000002487, -149.5231586289125687 ) ) ;
#8670=CARTESIAN_POINT ( 'NONE',  ( 1.749999999999998224, 14.46891108675447768, -62.32139747004410424 ) ) ;
#8671=EDGE_LOOP ( 'NONE', ( #29962, #27585, #4248, #38985 ) ) ;
#8673=CARTESIAN_POINT ( 'NONE',  ( -1.749999999999999778, 20.53108891324555785, -113.8213974700440900 ) ) ;
#8674=CARTESIAN_POINT ( 'NONE',  ( -3.500000000000002220, 15.47927405783633503, -139.8776474690881741 ) ) ;
#8676=CARTESIAN_POINT ( 'NONE',  ( 3.500000000000001332, 19.52072594216370760, -61.07139747004409713 ) ) ;
#8679=CARTESIAN_POINT ( 'NONE',  ( 3.310556943750001313, 19.41135094264166483, -69.18077246956613635 ) ) ;
#8681=CARTESIAN_POINT ( 'NONE',  ( 4.648177544792955347E-16, 21.00000000000001776, -79.21098080242148853 ) ) ;
#8683=ORIENTED_EDGE ( 'NONE', *, *, #3658, .T. ) ;
#8684=CARTESIAN_POINT ( 'NONE',  ( -7.022189441860112050E-16, 13.67729811471671297, -23.51410580289947561 ) ) ;
#8686=CARTESIAN_POINT ( 'NONE',  ( 1.655278471874998436, 14.63297358603754361, -77.43077246956615056 ) ) ;
#8690=CARTESIAN_POINT ( 'NONE',  ( -0.9378221735089291577, 21.00000000000002132, -128.1663226036829712 ) ) ;
#8693=CARTESIAN_POINT ( 'NONE',  ( 0.000000000000000000, 17.50000000000002487, -149.5231586289125687 ) ) ;
#8694=ADVANCED_FACE ( 'NONE', ( #38189 ), #24815, .T. ) ;
#8695=EDGE_LOOP ( 'NONE', ( #23298, #11624, #13554, #19895 ) ) ;
#8697=CARTESIAN_POINT ( 'NONE',  ( -1.655278471874999990, 20.36702641396248836, -48.01827246956613493 ) ) ;
#8698=CARTESIAN_POINT ( 'NONE',  ( -3.310556943750000425, 19.41135094264166838, -109.9349391362327992 ) ) ;
#8700=( BOUNDED_CURVE ( )  B_SPLINE_CURVE ( 2, ( #34318, #38344, #5600, #14964, #34943, #22183, #34733, #35152, #18992 ),
 .UNSPECIFIED., .F., .T. ) 
 B_SPLINE_CURVE_WITH_KNOTS ( ( 3, 2, 2, 2, 3 ),
 ( 0.8562499999999999556, 0.8569444444444443976, 0.8583333333333332815, 0.8597222222222222765, 0.8604166666666667185 ),
 .UNSPECIFIED. ) 
 CURVE ( )  GEOMETRIC_REPRESENTATION_ITEM ( )  RATIONAL_B_SPLINE_CURVE ( ( 0.9330127018922194093, 0.9330127018922194093, 1.000000000000000000, 0.8660254037844387076, 1.000000000000000000, 0.8660254037844387076, 1.000000000000000000, 0.9330127018922194093, 0.9330127018922194093 ) ) 
 REPRESENTATION_ITEM ( '' )  );
#8701=CARTESIAN_POINT ( 'NONE',  ( -7.022189441860112050E-16, 13.67729811471671475, -36.51410580289947205 ) ) ;
#8702=CARTESIAN_POINT ( 'NONE',  ( -7.022189441860112050E-16, 13.67729811471671830, -61.60160580289946353 ) ) ;
#8703=AXIS2_PLACEMENT_3D ( 'NONE', #35731, #4026, #622 ) ;
#8704=CARTESIAN_POINT ( 'NONE',  ( -3.500000000000001332, 17.50000000000002132, -110.9609808024215027 ) ) ;
#8706=CARTESIAN_POINT ( 'NONE',  ( 3.310556943750001313, 17.50000000000001776, -90.26410580289947916 ) ) ;
#8707=CARTESIAN_POINT ( 'NONE',  ( 1.749999999999998224, 14.46891108675447768, -63.62764746908818125 ) ) ;
#8709=EDGE_CURVE ( 'NONE', #25746, #21455, #15657, .T. ) ;
#8711=CARTESIAN_POINT ( 'NONE',  ( -7.424026671074350129E-16, 13.45854811567263454, -66.71098080242150274 ) ) ;
#8713=CARTESIAN_POINT ( 'NONE',  ( 3.310556943749999981, 15.58864905735836182, -29.34743913623280775 ) ) ;
#8715=CARTESIAN_POINT ( 'NONE',  ( -3.500000000000002220, 15.47927405783632437, -55.57139747004409713 ) ) ;
#8717=CARTESIAN_POINT ( 'NONE',  ( -3.310556943750001313, 17.50000000000002132, -104.8516058028994564 ) ) ;
#8718=CARTESIAN_POINT ( 'NONE',  ( -1.655278471875002211, 14.63297358603754006, -37.68493913623280633 ) ) ;
#8720=CARTESIAN_POINT ( 'NONE',  ( 0.000000000000000000, 17.50000000000002487, -149.5231586289125687 ) ) ;
#8725=CARTESIAN_POINT ( 'NONE',  ( 3.310556943750001313, 17.50000000000001776, -90.26410580289947916 ) ) ;
#8728=ORIENTED_EDGE ( 'NONE', *, *, #14862, .T. ) ;
#8730=CARTESIAN_POINT ( 'NONE',  ( 0.9378221735089281585, 14.00000000000002309, -133.3600726046389013 ) ) ;
#8735=CARTESIAN_POINT ( 'NONE',  ( -1.655278471874999990, 20.36702641396249192, -94.93077246956613635 ) ) ;
#8739=VERTEX_POINT ( 'NONE', #11819 ) ;
#8746=ORIENTED_EDGE ( 'NONE', *, *, #38564, .F. ) ;
#8750=CARTESIAN_POINT ( 'NONE',  ( -1.655278471874999990, 20.36702641396249902, -134.9307724695661364 ) ) ;
#8751=DIRECTION ( 'NONE',  ( -0.000000000000000000, 1.259100132267607459E-16, -1.000000000000000000 ) ) ;
#8753=CARTESIAN_POINT ( 'NONE',  ( -1.394453263437886604E-15, 14.00000000000001066, -26.40473080337743284 ) ) ;
#8754=CARTESIAN_POINT ( 'NONE',  ( 2.340729813953370519E-16, 21.32270188528331900, -123.1016058028994564 ) ) ;
#8755=CARTESIAN_POINT ( 'NONE',  ( 1.655278471875001101, 20.36702641396248836, -56.18493913623279212 ) ) ;
#8756=VERTEX_POINT ( 'NONE', #18211 ) ;
#8758=CARTESIAN_POINT ( 'NONE',  ( -1.749999999999999778, 20.53108891324556140, -135.8213974700441042 ) ) ;
#8759=( BOUNDED_CURVE ( )  B_SPLINE_CURVE ( 2, ( #23086, #16923, #26921, #6922, #13728, #23731, #7140, #26708, #3941 ),
 .UNSPECIFIED., .F., .F. ) 
 B_SPLINE_CURVE_WITH_KNOTS ( ( 3, 2, 2, 2, 3 ),
 ( 0.07708333333333333703, 0.07777777777777777901, 0.07916666666666666297, 0.08055555555555556080, 0.08125000000000000278 ),
 .UNSPECIFIED. ) 
 CURVE ( )  GEOMETRIC_REPRESENTATION_ITEM ( )  RATIONAL_B_SPLINE_CURVE ( ( 0.9330127018922194093, 0.9330127018922194093, 1.000000000000000000, 0.8660254037844387076, 1.000000000000000000, 0.8660254037844387076, 1.000000000000000000, 0.9330127018922194093, 0.9330127018922194093 ) ) 
 REPRESENTATION_ITEM ( '' )  );
#8761=CARTESIAN_POINT ( 'NONE',  ( -1.655278471875002211, 14.63297358603754539, -77.68493913623279923 ) ) ;
#8762=CARTESIAN_POINT ( 'NONE',  ( 2.474675557024783212E-16, 21.54145188432740099, -127.2109808024215027 ) ) ;
#8763=CARTESIAN_POINT ( 'NONE',  ( -1.655278471875002211, 14.63297358603755072, -112.5974391362328078 ) ) ;
#8767=CARTESIAN_POINT ( 'NONE',  ( -7.424026671074350129E-16, 13.45854811567263454, -80.71098080242150274 ) ) ;
#8768=AXIS2_PLACEMENT_3D ( 'NONE', #2518, #34427, #28039 ) ;
#8769=CARTESIAN_POINT ( 'NONE',  ( -1.749999999999999778, 20.53108891324555074, -62.12764746908818125 ) ) ;
#8770=CARTESIAN_POINT ( 'NONE',  ( -1.655278471874999990, 20.36702641396248836, -48.93077246956615056 ) ) ;
#8771=CARTESIAN_POINT ( 'NONE',  ( 1.655278471875001101, 20.36702641396249192, -99.18493913623279923 ) ) ;
#8774=ORIENTED_EDGE ( 'NONE', *, *, #11524, .F. ) ;
#8776=CARTESIAN_POINT ( 'NONE',  ( -7.022189441860112050E-16, 13.67729811471672896, -122.6016058028994706 ) ) ;
#8781=CARTESIAN_POINT ( 'NONE',  ( 4.648177544792955347E-16, 21.00000000000002487, -129.9047308033774186 ) ) ;
#8782=FACE_OUTER_BOUND ( 'NONE', #14047, .T. ) ;
#8784=VECTOR ( 'NONE', #30220, 1000.000000000000000 ) ;
#8786=CARTESIAN_POINT ( 'NONE',  ( 3.310556943749999981, 15.58864905735836714, -73.43493913623279923 ) ) ;
#8787=ADVANCED_FACE ( 'NONE', ( #12239 ), #31179, .T. ) ;
#8789=DIRECTION ( 'NONE',  ( -0.000000000000000000, 1.259100132267607459E-16, -1.000000000000000000 ) ) ;
#8790=CARTESIAN_POINT ( 'NONE',  ( 4.648177544792955347E-16, 21.00000000000001066, -39.90473080337742573 ) ) ;
#8791=CARTESIAN_POINT ( 'NONE',  ( 3.500000000000001332, 17.50000000000001776, -99.15473080337743284 ) ) ;
#8792=EDGE_CURVE ( 'NONE', #37609, #38089, #2307, .T. ) ;
#8796=CARTESIAN_POINT ( 'NONE',  ( 2.340729813953370519E-16, 21.32270188528330834, -33.01410580289947205 ) ) ;
#8800=EDGE_CURVE ( 'NONE', #2506, #31803, #6893, .T. ) ;
#8801=CARTESIAN_POINT ( 'NONE',  ( 3.310556943750001313, 17.50000000000001421, -48.26410580289947205 ) ) ;
#8802=ORIENTED_EDGE ( 'NONE', *, *, #7554, .T. ) ;
#8804=DIRECTION ( 'NONE',  ( -0.000000000000000000, 1.259100132267607459E-16, -1.000000000000000000 ) ) ;
#8807=CARTESIAN_POINT ( 'NONE',  ( 0.9378221735089281585, 14.00000000000002132, -97.66632260368298546 ) ) ;
#8808=DIRECTION ( 'NONE',  ( 0.000000000000000000, 1.000000000000000000, 0.000000000000000000 ) ) ;
#8809=CARTESIAN_POINT ( 'NONE',  ( -3.500000000000002220, 15.47927405783632082, -36.87764746908817415 ) ) ;
#8810=CARTESIAN_POINT ( 'NONE',  ( 3.500000000000001332, 19.52072594216371115, -86.37764746908817415 ) ) ;
#8816=CARTESIAN_POINT ( 'NONE',  ( 3.310556943749999981, 15.58864905735836004, -25.43493913623279212 ) ) ;
#8817=DIRECTION ( 'NONE',  ( -0.000000000000000000, 1.259100132267607459E-16, -1.000000000000000000 ) ) ;
#8818=CARTESIAN_POINT ( 'NONE',  ( -1.655278471874999990, 20.36702641396249902, -130.9307724695661364 ) ) ;
#8821=CARTESIAN_POINT ( 'NONE',  ( 3.405278471875001323, 17.50000000000001066, -23.40629330266049024 ) ) ;
#8822=CARTESIAN_POINT ( 'NONE',  ( -3.310556943750001313, 17.50000000000002132, -115.8516058028994706 ) ) ;
#8824=CARTESIAN_POINT ( 'NONE',  ( 1.749999999999998224, 14.46891108675447590, -40.32139747004409713 ) ) ;
#8827=CARTESIAN_POINT ( 'NONE',  ( -7.022189441860112050E-16, 13.67729811471673074, -137.6016058028994564 ) ) ;
#8829=CARTESIAN_POINT ( 'NONE',  ( 1.655278471874998436, 14.63297358603754006, -50.51827246956612782 ) ) ;
#8831=CARTESIAN_POINT ( 'NONE',  ( -1.655278471875002211, 14.63297358603754539, -76.68493913623279923 ) ) ;
#8833=CARTESIAN_POINT ( 'NONE',  ( 1.655278471875001101, 20.36702641396249192, -98.09743913623280775 ) ) ;
#8834=CARTESIAN_POINT ( 'NONE',  ( 3.310556943749999981, 15.58864905735836714, -68.34743913623280775 ) ) ;
#8836=CARTESIAN_POINT ( 'NONE',  ( -7.022189441860112050E-16, 13.67729811471672363, -90.60160580289947063 ) ) ;
#8838=CARTESIAN_POINT ( 'NONE',  ( 1.749999999999998224, 14.46891108675447590, -49.62764746908818125 ) ) ;
#8840=CARTESIAN_POINT ( 'NONE',  ( 3.310556943750001313, 19.41135094264166483, -56.18077246956613635 ) ) ;
#8841=CARTESIAN_POINT ( 'NONE',  ( -3.500000000000002220, 15.47927405783632082, -24.57139747004409713 ) ) ;
#8842=CARTESIAN_POINT ( 'NONE',  ( -3.310556943750000425, 19.41135094264166838, -111.8474391362328220 ) ) ;
#8843=CARTESIAN_POINT ( 'NONE',  ( -3.500000000000002220, 15.47927405783633326, -101.5713974700440900 ) ) ;
#8846=EDGE_LOOP ( 'NONE', ( #33963, #13397, #19051, #30922 ) ) ;
#8847=ORIENTED_EDGE ( 'NONE', *, *, #30838, .T. ) ;
#8849=ORIENTED_EDGE ( 'NONE', *, *, #34065, .T. ) ;
#8852=CARTESIAN_POINT ( 'NONE',  ( 3.310556943750001313, 17.50000000000001421, -64.26410580289946495 ) ) ;
#8853=ORIENTED_EDGE ( 'NONE', *, *, #22215, .F. ) ;
#8854=ORIENTED_EDGE ( 'NONE', *, *, #42020, .F. ) ;
#8861=CARTESIAN_POINT ( 'NONE',  ( -7.022189441860112050E-16, 13.67729811471672896, -130.5141058028994507 ) ) ;
#8864=CARTESIAN_POINT ( 'NONE',  ( -3.310556943750000425, 19.41135094264165772, -40.93493913623278502 ) ) ;
#8865=CARTESIAN_POINT ( 'NONE',  ( 3.310556943750001313, 17.50000000000001066, -25.35160580289946708 ) ) ;
#8866=CARTESIAN_POINT ( 'NONE',  ( 1.655278471875001101, 20.36702641396249192, -93.18493913623279923 ) ) ;
#8867=CARTESIAN_POINT ( 'NONE',  ( 2.474675557024783212E-16, 21.54145188432739033, -23.90473080337743284 ) ) ;
#8868=VERTEX_POINT ( 'NONE', #3403 ) ;
#8873=CARTESIAN_POINT ( 'NONE',  ( -1.655278471874999990, 20.36702641396249902, -137.0182724695661420 ) ) ;
#8877=CARTESIAN_POINT ( 'NONE',  ( 3.500000000000001776, 19.52072594216371115, -81.07139747004410424 ) ) ;
#8878=CARTESIAN_POINT ( 'NONE',  ( -3.310556943750001313, 17.50000000000001421, -66.85160580289947063 ) ) ;
#8882=CARTESIAN_POINT ( 'NONE',  ( -3.500000000000000000, 19.52072594216370760, -60.04431413575483845 ) ) ;
#8884=CARTESIAN_POINT ( 'NONE',  ( -1.655278471875002211, 14.63297358603755072, -120.5974391362328078 ) ) ;
#8885=( BOUNDED_CURVE ( )  B_SPLINE_CURVE ( 2, ( #27497, #31095, #1753, #8543, #1950, #37686, #21521, #8961, #5349 ),
 .UNSPECIFIED., .F., .T. ) 
 B_SPLINE_CURVE_WITH_KNOTS ( ( 3, 2, 2, 2, 3 ),
 ( 0.3229166666666666852, 0.3236111111111111271, 0.3250000000000000111, 0.3263888888888888951, 0.3270833333333333370 ),
 .UNSPECIFIED. ) 
 CURVE ( )  GEOMETRIC_REPRESENTATION_ITEM ( )  RATIONAL_B_SPLINE_CURVE ( ( 0.9330127018922194093, 0.9330127018922194093, 1.000000000000000000, 0.8660254037844387076, 1.000000000000000000, 0.8660254037844387076, 1.000000000000000000, 0.9330127018922194093, 0.9330127018922194093 ) ) 
 REPRESENTATION_ITEM ( '' )  );
#8887=VERTEX_POINT ( 'NONE', #4032 ) ;
#8888=CARTESIAN_POINT ( 'NONE',  ( 1.749999999999998224, 14.46891108675448301, -107.3213974700441042 ) ) ;
#8890=( BOUNDED_CURVE ( )  B_SPLINE_CURVE ( 2, ( #13721, #33066, #20312, #40511, #748, #29882, #27119, #26699, #4569 ),
 .UNSPECIFIED., .F., .T. ) 
 B_SPLINE_CURVE_WITH_KNOTS ( ( 3, 2, 2, 2, 3 ),
 ( 0.3937499999999999889, 0.3944444444444444309, 0.3958333333333333148, 0.3972222222222221988, 0.3979166666666666963 ),
 .UNSPECIFIED. ) 
 CURVE ( )  GEOMETRIC_REPRESENTATION_ITEM ( )  RATIONAL_B_SPLINE_CURVE ( ( 0.9330127018922194093, 0.9330127018922194093, 1.000000000000000000, 0.8660254037844387076, 1.000000000000000000, 0.8660254037844387076, 1.000000000000000000, 0.9330127018922167448, 0.9330127018922194093 ) ) 
 REPRESENTATION_ITEM ( '' )  );
#8893=CARTESIAN_POINT ( 'NONE',  ( 1.750000000000001110, 20.53108891324555074, -58.98806413671076143 ) ) ;
#8895=CARTESIAN_POINT ( 'NONE',  ( 3.310556943749999981, 15.58864905735836714, -71.34743913623280775 ) ) ;
#8898=CARTESIAN_POINT ( 'NONE',  ( 1.750000000000001110, 20.53108891324555074, -69.29431413575484555 ) ) ;
#8900=CARTESIAN_POINT ( 'NONE',  ( 1.655278471874998436, 14.63297358603753651, -24.43077246956613990 ) ) ;
#8902=CARTESIAN_POINT ( 'NONE',  ( -3.310556943750000425, 19.41135094264166483, -79.84743913623279354 ) ) ;
#8904=CIRCLE ( 'NONE', #20480, 3.500000000000003109 ) ;
#8905=CARTESIAN_POINT ( 'NONE',  ( -0.9378221735089310451, 14.00000000000002309, -127.7556390011600200 ) ) ;
#8908=CARTESIAN_POINT ( 'NONE',  ( -3.500000000000002220, 15.47927405783633503, -113.5713974700440900 ) ) ;
#8909=CARTESIAN_POINT ( 'NONE',  ( -3.310556943750001313, 17.50000000000001421, -48.85160580289946353 ) ) ;
#8910=CARTESIAN_POINT ( 'NONE',  ( 3.310556943749999981, 15.58864905735837070, -107.4349391362327992 ) ) ;
#8912=CARTESIAN_POINT ( 'NONE',  ( 2.340729813953370519E-16, 21.32270188528330479, -37.01410580289946495 ) ) ;
#8913=CARTESIAN_POINT ( 'NONE',  ( 3.310556943749999981, 15.58864905735836537, -60.43493913623279212 ) ) ;
#8914=CARTESIAN_POINT ( 'NONE',  ( -3.500000000000002220, 15.47927405783632970, -105.8776474690881741 ) ) ;
#8916=CARTESIAN_POINT ( 'NONE',  ( -1.655278471874999990, 20.36702641396249192, -89.93077246956613635 ) ) ;
#8917=CARTESIAN_POINT ( 'NONE',  ( 2.474675557024783212E-16, 21.54145188432739744, -96.90473080337741862 ) ) ;
#8921=CARTESIAN_POINT ( 'NONE',  ( -1.749999999999999778, 20.53108891324555074, -58.12764746908817415 ) ) ;
#8923=CARTESIAN_POINT ( 'NONE',  ( -3.310556943750002645, 15.58864905735836537, -27.68077246956613990 ) ) ;
#8924=VECTOR ( 'NONE', #1504, 1000.000000000000000 ) ;
#8925=CARTESIAN_POINT ( 'NONE',  ( -3.500000000000002220, 15.47927405783632260, -46.57139747004410424 ) ) ;
#8927=CARTESIAN_POINT ( 'NONE',  ( 1.655278471874998436, 14.63297358603754716, -106.5182724695661278 ) ) ;
#8928=CARTESIAN_POINT ( 'NONE',  ( -3.310556943750002201, 15.58864905735836537, -31.76827246956613493 ) ) ;
#8935=CARTESIAN_POINT ( 'NONE',  ( -1.655278471875002211, 14.63297358603754716, -86.59743913623280775 ) ) ;
#8939=CARTESIAN_POINT ( 'NONE',  ( 3.500000000000000000, 15.47927405783632615, -74.54431413575483134 ) ) ;
#8943=CARTESIAN_POINT ( 'NONE',  ( -3.310556943750001313, 17.50000000000001776, -97.76410580289947916 ) ) ;
#8947=ORIENTED_EDGE ( 'NONE', *, *, #26195, .T. ) ;
#8950=DIRECTION ( 'NONE',  ( -0.000000000000000000, 1.259100132267607459E-16, -1.000000000000000000 ) ) ;
#8953=( BOUNDED_CURVE ( )  B_SPLINE_CURVE ( 2, ( #26930, #1607, #36924, #1398, #27347, #33517, #17359, #39683, #14587 ),
 .UNSPECIFIED., .F., .T. ) 
 B_SPLINE_CURVE_WITH_KNOTS ( ( 3, 2, 2, 2, 3 ),
 ( 0.8687500000000000222, 0.8694444444444444642, 0.8708333333333333481, 0.8722222222222222321, 0.8729166666666666741 ),
 .UNSPECIFIED. ) 
 CURVE ( )  GEOMETRIC_REPRESENTATION_ITEM ( )  RATIONAL_B_SPLINE_CURVE ( ( 0.9330127018922194093, 0.9330127018922194093, 1.000000000000000000, 0.8660254037844387076, 1.000000000000000000, 0.8660254037844387076, 1.000000000000000000, 0.9330127018922194093, 0.9330127018922194093 ) ) 
 REPRESENTATION_ITEM ( '' )  );
#8954=ORIENTED_EDGE ( 'NONE', *, *, #12848, .F. ) ;
#8955=ADVANCED_FACE ( 'NONE', ( #20206 ), #38927, .T. ) ;
#8956=DIRECTION ( 'NONE',  ( -0.000000000000000000, 1.259100132267607459E-16, -1.000000000000000000 ) ) ;
#8957=VECTOR ( 'NONE', #1627, 1000.000000000000000 ) ;
#8958=CARTESIAN_POINT ( 'NONE',  ( 4.286263797015737581E-16, 14.00000000000002487, -149.5231586289125687 ) ) ;
#8959=EDGE_CURVE ( 'NONE', #28471, #35272, #31365, .T. ) ;
#8960=CARTESIAN_POINT ( 'NONE',  ( -3.310556943750000425, 19.41135094264167549, -136.8474391362328220 ) ) ;
#8961=CARTESIAN_POINT ( 'NONE',  ( 0.9378221735089300459, 21.00000000000002132, -103.9493890021159501 ) ) ;
#8964=CARTESIAN_POINT ( 'NONE',  ( 1.655278471874998436, 14.63297358603754006, -50.51827246956612782 ) ) ;
#8965=ORIENTED_EDGE ( 'NONE', *, *, #38624, .F. ) ;
#8967=CARTESIAN_POINT ( 'NONE',  ( 3.500000000000000000, 15.47927405783633503, -134.2380641367107614 ) ) ;
#8970=CARTESIAN_POINT ( 'NONE',  ( -7.022189441860112050E-16, 13.67729811471672186, -76.60160580289945642 ) ) ;
#8971=CARTESIAN_POINT ( 'NONE',  ( 3.500000000000001776, 19.52072594216371826, -123.3776474690881884 ) ) ;
#8972=CARTESIAN_POINT ( 'NONE',  ( 2.340729813953370519E-16, 21.32270188528331900, -108.0141058028994649 ) ) ;
#8974=CARTESIAN_POINT ( 'NONE',  ( -1.394453263437886604E-15, 14.00000000000001776, -107.4047308033774328 ) ) ;
#8976=AXIS2_PLACEMENT_3D ( 'NONE', #35189, #3697, #6886 ) ;
#8978=CARTESIAN_POINT ( 'NONE',  ( -3.500000000000001332, 17.50000000000001776, -82.96098080242150274 ) ) ;
#8979=CARTESIAN_POINT ( 'NONE',  ( 3.500000000000000000, 15.47927405783632970, -103.2380641367107472 ) ) ;
#8980=CARTESIAN_POINT ( 'NONE',  ( -3.310556943750002645, 15.58864905735836714, -43.68077246956613635 ) ) ;
#8981=CARTESIAN_POINT ( 'NONE',  ( 2.340729813953370519E-16, 21.32270188528331900, -103.1016058028994564 ) ) ;
#8983=ORIENTED_EDGE ( 'NONE', *, *, #39427, .T. ) ;
#8984=CARTESIAN_POINT ( 'NONE',  ( -1.655278471875002211, 14.63297358603755249, -124.6849391362327992 ) ) ;
#8989=CARTESIAN_POINT ( 'NONE',  ( 3.500000000000000000, 15.47927405783632437, -60.54431413575484555 ) ) ;
#8990=CARTESIAN_POINT ( 'NONE',  ( -0.9378221735089291577, 21.00000000000001421, -63.16632260368299256 ) ) ;
#8993=CARTESIAN_POINT ( 'NONE',  ( -1.655278471874999990, 20.36702641396248836, -73.01827246956612782 ) ) ;
#8995=DIRECTION ( 'NONE',  ( -0.000000000000000000, 1.259100132267607459E-16, -1.000000000000000000 ) ) ;
#8996=CARTESIAN_POINT ( 'NONE',  ( -3.500000000000002220, 15.47927405783633503, -139.5713974700441042 ) ) ;
#8999=CARTESIAN_POINT ( 'NONE',  ( -1.655278471875002211, 14.63297358603754006, -36.59743913623281486 ) ) ;
#9003=ORIENTED_EDGE ( 'NONE', *, *, #5048, .T. ) ;
#9005=AXIS2_PLACEMENT_3D ( 'NONE', #20161, #29723, #7189 ) ;
#9006=CARTESIAN_POINT ( 'NONE',  ( 3.310556943749999981, 15.58864905735836182, -48.34743913623281486 ) ) ;
#9008=ORIENTED_EDGE ( 'NONE', *, *, #15735, .T. ) ;
#9010=( BOUNDED_CURVE ( )  B_SPLINE_CURVE ( 2, ( #40279, #14959, #1154, #37503, #7956, #4755, #40065, #1572, #37717 ),
 .UNSPECIFIED., .F., .T. ) 
 B_SPLINE_CURVE_WITH_KNOTS ( ( 3, 2, 2, 2, 3 ),
 ( 0.4979166666666666741, 0.4986111111111111160, 0.5000000000000000000, 0.5013888888888888840, 0.5020833333333333259 ),
 .UNSPECIFIED. ) 
 CURVE ( )  GEOMETRIC_REPRESENTATION_ITEM ( )  RATIONAL_B_SPLINE_CURVE ( ( 0.9330127018922194093, 0.9330127018922194093, 1.000000000000000000, 0.8660254037844387076, 1.000000000000000000, 0.8660254037844387076, 1.000000000000000000, 0.9330127018922194093, 0.9330127018922194093 ) ) 
 REPRESENTATION_ITEM ( '' )  );
#9011=CARTESIAN_POINT ( 'NONE',  ( 1.750000000000001110, 20.53108891324554719, -24.29431413575484910 ) ) ;
#9014=DIRECTION ( 'NONE',  ( 0.000000000000000000, 1.000000000000000000, 0.000000000000000000 ) ) ;
#9015=CARTESIAN_POINT ( 'NONE',  ( -3.500000000000000888, 19.52072594216370405, -32.04431413575484555 ) ) ;
#9017=DIRECTION ( 'NONE',  ( -0.000000000000000000, 1.259100132267607459E-16, -1.000000000000000000 ) ) ;
#9019=LINE ( 'NONE', #15201, #9850 ) ;
#9021=CARTESIAN_POINT ( 'NONE',  ( 3.500000000000001332, 17.50000000000002487, -143.4609808024215170 ) ) ;
#9023=CARTESIAN_POINT ( 'NONE',  ( -1.394453263437886604E-15, 14.00000000000001421, -60.71098080242150985 ) ) ;
#9024=CARTESIAN_POINT ( 'NONE',  ( 2.340729813953370519E-16, 21.32270188528331900, -125.0141058028994792 ) ) ;
#9027=CARTESIAN_POINT ( 'NONE',  ( 1.750000000000001110, 20.53108891324554719, -23.98806413671077209 ) ) ;
#9028=CARTESIAN_POINT ( 'NONE',  ( 1.655278471874998436, 14.63297358603754894, -116.5182724695661278 ) ) ;
#9029=CARTESIAN_POINT ( 'NONE',  ( -0.9378221735089291577, 21.00000000000001421, -55.86007260463891555 ) ) ;
#9030=CARTESIAN_POINT ( 'NONE',  ( -3.500000000000002220, 15.47927405783632082, -35.57139747004409003 ) ) ;
#9033=CARTESIAN_POINT ( 'NONE',  ( -1.655278471875002211, 14.63297358603755427, -140.6849391362327708 ) ) ;
#9034=EDGE_CURVE ( 'NONE', #41304, #33169, #30194, .T. ) ;
#9037=CARTESIAN_POINT ( 'NONE',  ( 0.000000000000000000, 17.50000000000002487, -149.5231586289125687 ) ) ;
#9038=CARTESIAN_POINT ( 'NONE',  ( 3.310556943750001313, 19.41135094264166128, -46.26827246956613493 ) ) ;
#9040=CARTESIAN_POINT ( 'NONE',  ( 3.500000000000001332, 19.52072594216371826, -104.3776474690881741 ) ) ;
#9041=AXIS2_PLACEMENT_3D ( 'NONE', #14098, #39831, #695 ) ;
#9042=CARTESIAN_POINT ( 'NONE',  ( -1.655278471874999990, 20.36702641396248836, -68.01827246956612782 ) ) ;
#9044=CARTESIAN_POINT ( 'NONE',  ( -1.655278471874999990, 20.36702641396248836, -67.93077246956613635 ) ) ;
#9046=CARTESIAN_POINT ( 'NONE',  ( -1.655278471874999990, 20.36702641396249192, -93.01827246956612782 ) ) ;
#9047=EDGE_CURVE ( 'NONE', #28655, #217, #15362, .T. ) ;
#9050=DIRECTION ( 'NONE',  ( -0.000000000000000000, 1.259100132267607459E-16, -1.000000000000000000 ) ) ;
#9051=CARTESIAN_POINT ( 'NONE',  ( 3.500000000000000000, 15.47927405783633503, -131.5443141357548598 ) ) ;
#9052=CARTESIAN_POINT ( 'NONE',  ( 1.655278471875001101, 20.36702641396248836, -51.09743913623280775 ) ) ;
#9053=DIRECTION ( 'NONE',  ( -0.000000000000000000, 1.259100132267607459E-16, -1.000000000000000000 ) ) ;
#9054=CARTESIAN_POINT ( 'NONE',  ( 3.310556943750001313, 19.41135094264166838, -109.1807724695661506 ) ) ;
#9055=CYLINDRICAL_SURFACE ( 'NONE', #3309, 3.499999999999999556 ) ;
#9056=EDGE_LOOP ( 'NONE', ( #13001, #35006, #21827, #13699 ) ) ;
#9061=CARTESIAN_POINT ( 'NONE',  ( 1.655278471874998436, 14.63297358603754184, -64.43077246956615056 ) ) ;
#9063=ORIENTED_EDGE ( 'NONE', *, *, #14724, .T. ) ;
#9070=CARTESIAN_POINT ( 'NONE',  ( 0.000000000000000000, 21.00000000000002487, -149.5231586289125687 ) ) ;
#9071=CARTESIAN_POINT ( 'NONE',  ( -3.310556943750001313, 17.50000000000002132, -128.7641058028994792 ) ) ;
#9074=CARTESIAN_POINT ( 'NONE',  ( -3.310556943750002645, 15.58864905735836537, -39.76827246956612072 ) ) ;
#9076=CARTESIAN_POINT ( 'NONE',  ( -3.310556943750000425, 19.41135094264165772, -27.93493913623279568 ) ) ;
#9077=CARTESIAN_POINT ( 'NONE',  ( 3.310556943750001313, 17.50000000000001776, -93.35160580289947063 ) ) ;
#9078=CARTESIAN_POINT ( 'NONE',  ( -3.310556943750002645, 15.58864905735837958, -142.6807724695661364 ) ) ;
#9080=CARTESIAN_POINT ( 'NONE',  ( 1.655278471875001101, 20.36702641396249902, -134.1849391362327992 ) ) ;
#9083=CARTESIAN_POINT ( 'NONE',  ( -0.9378221735089310451, 14.00000000000002309, -122.7556390011600342 ) ) ;
#9084=CARTESIAN_POINT ( 'NONE',  ( -0.9378221735089291577, 21.00000000000002132, -122.8600726046389155 ) ) ;
#9085=CARTESIAN_POINT ( 'NONE',  ( 3.500000000000000000, 15.47927405783632615, -82.23806413671076143 ) ) ;
#9086=EDGE_CURVE ( 'NONE', #24957, #28471, #33228, .T. ) ;
#9087=CARTESIAN_POINT ( 'NONE',  ( 3.310556943749999981, 15.58864905735836537, -63.43493913623279923 ) ) ;
#9091=CARTESIAN_POINT ( 'NONE',  ( -3.310556943750002645, 15.58864905735837247, -89.76827246956612782 ) ) ;
#9092=LINE ( 'NONE', #2292, #41146 ) ;
#9093=CARTESIAN_POINT ( 'NONE',  ( -1.655278471874999990, 20.36702641396249547, -113.9307724695661364 ) ) ;
#9095=CARTESIAN_POINT ( 'NONE',  ( 0.9378221735089300459, 21.00000000000001421, -61.94938900211595723 ) ) ;
#9097=CARTESIAN_POINT ( 'NONE',  ( -3.500000000000000888, 19.52072594216371826, -110.7380641367107756 ) ) ;
#9100=CARTESIAN_POINT ( 'NONE',  ( 4.648177544792955347E-16, 21.00000000000001066, -32.90473080337742573 ) ) ;
#9104=CARTESIAN_POINT ( 'NONE',  ( -3.310556943750000425, 19.41135094264166483, -65.84743913623280775 ) ) ;
#9110=CARTESIAN_POINT ( 'NONE',  ( 3.310556943750001313, 17.50000000000001066, -23.26410580289947561 ) ) ;
#9111=CARTESIAN_POINT ( 'NONE',  ( -0.9378221735089310451, 14.00000000000002132, -104.7556390011600342 ) ) ;
#9112=CARTESIAN_POINT ( 'NONE',  ( 2.340729813953370519E-16, 21.32270188528331190, -81.01410580289947916 ) ) ;
#9113=VERTEX_POINT ( 'NONE', #17449 ) ;
#9114=ORIENTED_EDGE ( 'NONE', *, *, #3721, .T. ) ;
#9120=CARTESIAN_POINT ( 'NONE',  ( -1.655278471874999990, 20.36702641396248481, -42.01827246956612782 ) ) ;
#9121=CARTESIAN_POINT ( 'NONE',  ( 2.340729813953370519E-16, 21.32270188528331900, -107.1016058028994706 ) ) ;
#9123=( BOUNDED_CURVE ( )  B_SPLINE_CURVE ( 2, ( #346, #26307, #30325, #23743, #7791, #13958, #26726, #33739, #7157 ),
 .UNSPECIFIED., .F., .T. ) 
 B_SPLINE_CURVE_WITH_KNOTS ( ( 3, 2, 2, 2, 3 ),
 ( 0.9895833333333333703, 0.9902777777777778123, 0.9916666666666666963, 0.9930555555555555802, 0.9937500000000000222 ),
 .UNSPECIFIED. ) 
 CURVE ( )  GEOMETRIC_REPRESENTATION_ITEM ( )  RATIONAL_B_SPLINE_CURVE ( ( 0.9330127018922194093, 0.9330127018922194093, 1.000000000000000000, 0.8660254037844387076, 1.000000000000000000, 0.8660254037844387076, 1.000000000000000000, 0.9330127018922194093, 0.9330127018922194093 ) ) 
 REPRESENTATION_ITEM ( '' )  );
#9124=CARTESIAN_POINT ( 'NONE',  ( 2.340729813953370519E-16, 21.32270188528330479, -28.01410580289947916 ) ) ;
#9126=CARTESIAN_POINT ( 'NONE',  ( -3.310556943750001313, 17.50000000000001421, -62.85160580289946353 ) ) ;
#9127=CARTESIAN_POINT ( 'NONE',  ( -7.424026671074350129E-16, 13.45854811567263809, -106.7109808024214885 ) ) ;
#9129=CARTESIAN_POINT ( 'NONE',  ( 1.750000000000001110, 20.53108891324555429, -97.98806413671076143 ) ) ;
#9130=EDGE_CURVE ( 'NONE', #25349, #22966, #19685, .T. ) ;
#9131=CARTESIAN_POINT ( 'NONE',  ( -0.9378221735088960731, 14.00000000000000000, -108.4493890021159359 ) ) ;
#9134=CARTESIAN_POINT ( 'NONE',  ( 1.750000000000001110, 20.53108891324555074, -58.29431413575483845 ) ) ;
#9136=CARTESIAN_POINT ( 'NONE',  ( 2.340729813953370519E-16, 21.32270188528330479, -26.01410580289947916 ) ) ;
#9137=CARTESIAN_POINT ( 'NONE',  ( -7.424026671074350129E-16, 13.45854811567263276, -49.40473080337743284 ) ) ;
#9140=CARTESIAN_POINT ( 'NONE',  ( 3.310556943750001313, 17.50000000000001776, -101.3516058028994706 ) ) ;
#9141=CARTESIAN_POINT ( 'NONE',  ( -3.310556943750001313, 17.50000000000001066, -32.85160580289946353 ) ) ;
#9144=CARTESIAN_POINT ( 'NONE',  ( -0.9378221735089291577, 21.00000000000001421, -57.16632260368298546 ) ) ;
#9148=CARTESIAN_POINT ( 'NONE',  ( 1.655278471874998436, 14.63297358603754539, -89.43077246956613635 ) ) ;
#9153=ORIENTED_EDGE ( 'NONE', *, *, #25985, .F. ) ;
#9156=CARTESIAN_POINT ( 'NONE',  ( -3.310556943750002645, 15.58864905735837247, -93.68077246956612214 ) ) ;
#9158=VERTEX_POINT ( 'NONE', #1685 ) ;
#9159=CYLINDRICAL_SURFACE ( 'NONE', #41330, 3.499999999999999556 ) ;
#9162=CARTESIAN_POINT ( 'NONE',  ( 1.750000000000001110, 20.53108891324556140, -139.2943141357548313 ) ) ;
#9169=LINE ( 'NONE', #12141, #21938 ) ;
#9170=DIRECTION ( 'NONE',  ( -0.000000000000000000, 1.259100132267607459E-16, -1.000000000000000000 ) ) ;
#9171=CARTESIAN_POINT ( 'NONE',  ( -7.022189441860112050E-16, 13.67729811471672718, -132.5141058028994792 ) ) ;
#9172=CARTESIAN_POINT ( 'NONE',  ( -1.394453263437886604E-15, 14.00000000000001066, -33.40473080337742573 ) ) ;
#9174=CARTESIAN_POINT ( 'NONE',  ( -3.500000000000000000, 19.52072594216370405, -31.73806413671076498 ) ) ;
#9175=CARTESIAN_POINT ( 'NONE',  ( 2.340729813953370519E-16, 21.32270188528331900, -127.1016058028994706 ) ) ;
#9176=CARTESIAN_POINT ( 'NONE',  ( -1.655278471875002211, 14.63297358603754184, -49.68493913623279923 ) ) ;
#9178=CARTESIAN_POINT ( 'NONE',  ( -1.750000000000002220, 14.46891108675448834, -134.4880641367107614 ) ) ;
#9181=CARTESIAN_POINT ( 'NONE',  ( 3.310556943749999981, 15.58864905735836714, -79.43493913623279923 ) ) ;
#9182=CARTESIAN_POINT ( 'NONE',  ( 3.500000000000001332, 17.50000000000002132, -124.4609808024215027 ) ) ;
#9183=CARTESIAN_POINT ( 'NONE',  ( -3.310556943750000425, 19.41135094264166838, -105.8474391362327935 ) ) ;
#9184=CARTESIAN_POINT ( 'NONE',  ( 4.648177544792955347E-16, 21.00000000000001776, -92.90473080337741862 ) ) ;
#9187=CARTESIAN_POINT ( 'NONE',  ( 2.474675557024783212E-16, 21.54145188432739744, -77.21098080242150274 ) ) ;
#9189=CARTESIAN_POINT ( 'NONE',  ( 1.749999999999998224, 14.46891108675447590, -51.62764746908816704 ) ) ;
#9190=CARTESIAN_POINT ( 'NONE',  ( 3.310556943750001313, 19.41135094264165772, -42.18077246956614346 ) ) ;
#9191=CARTESIAN_POINT ( 'NONE',  ( -1.655278471874999990, 20.36702641396249192, -101.0182724695661278 ) ) ;
#9192=CARTESIAN_POINT ( 'NONE',  ( -3.500000000000002220, 15.47927405783633503, -113.8776474690881741 ) ) ;
#9193=CARTESIAN_POINT ( 'NONE',  ( 2.474675557024783212E-16, 21.54145188432739388, -64.90473080337743284 ) ) ;
#9196=CARTESIAN_POINT ( 'NONE',  ( -7.022189441860112050E-16, 13.67729811471672896, -123.6016058028994564 ) ) ;
#9197=CARTESIAN_POINT ( 'NONE',  ( -0.9378221735089291577, 21.00000000000001776, -92.16632260368299967 ) ) ;
#9201=DIRECTION ( 'NONE',  ( 0.000000000000000000, -1.259100132267607459E-16, 1.000000000000000000 ) ) ;
#9202=CARTESIAN_POINT ( 'NONE',  ( -3.500000000000001332, 17.50000000000001421, -62.96098080242150274 ) ) ;
#9203=EDGE_CURVE ( 'NONE', #10062, #7031, #25669, .T. ) ;
#9206=CARTESIAN_POINT ( 'NONE',  ( -1.655278471875002211, 14.63297358603754539, -73.68493913623279923 ) ) ;
#9211=CARTESIAN_POINT ( 'NONE',  ( 4.648177544792955347E-16, 21.00000000000001421, -56.21098080242151696 ) ) ;
#9214=CARTESIAN_POINT ( 'NONE',  ( -1.655278471874999990, 20.36702641396248481, -31.93077246956614701 ) ) ;
#9215=( BOUNDED_CURVE ( )  B_SPLINE_CURVE ( 2, ( #4592, #27353, #11189, #13526, #24173, #37143, #7996, #20967, #4799 ),
 .UNSPECIFIED., .F., .T. ) 
 B_SPLINE_CURVE_WITH_KNOTS ( ( 3, 2, 2, 2, 3 ),
 ( 0.6479166666666666963, 0.6486111111111111382, 0.6500000000000000222, 0.6513888888888889062, 0.6520833333333333481 ),
 .UNSPECIFIED. ) 
 CURVE ( )  GEOMETRIC_REPRESENTATION_ITEM ( )  RATIONAL_B_SPLINE_CURVE ( ( 0.9330127018922194093, 0.9330127018922194093, 1.000000000000000000, 0.8660254037844387076, 1.000000000000000000, 0.8660254037844387076, 1.000000000000000000, 0.9330127018922194093, 0.9330127018922194093 ) ) 
 REPRESENTATION_ITEM ( '' )  );
#9218=VERTEX_POINT ( 'NONE', #38249 ) ;
#9221=EDGE_CURVE ( 'NONE', #24347, #40555, #41444, .T. ) ;
#9223=CARTESIAN_POINT ( 'NONE',  ( 3.500000000000001332, 17.50000000000001421, -56.15473080337743284 ) ) ;
#9224=CARTESIAN_POINT ( 'NONE',  ( 3.500000000000001332, 17.50000000000001776, -90.46098080242151696 ) ) ;
#9226=CARTESIAN_POINT ( 'NONE',  ( -1.394453263437886604E-15, 14.00000000000001776, -97.71098080242148853 ) ) ;
#9228=CARTESIAN_POINT ( 'NONE',  ( -3.500000000000002220, 15.47927405783633503, -117.5713974700440900 ) ) ;
#9230=CARTESIAN_POINT ( 'NONE',  ( 4.648177544792955347E-16, 21.00000000000001066, -34.21098080242150985 ) ) ;
#9231=CARTESIAN_POINT ( 'NONE',  ( -7.424026671074350129E-16, 13.45854811567263098, -33.71098080242150274 ) ) ;
#9233=CARTESIAN_POINT ( 'NONE',  ( 3.500000000000001332, 17.50000000000001066, -35.46098080242150985 ) ) ;
#9236=CARTESIAN_POINT ( 'NONE',  ( 3.500000000000001332, 17.50000000000001066, -37.15473080337743284 ) ) ;
#9238=CARTESIAN_POINT ( 'NONE',  ( -7.424026671074350129E-16, 13.45854811567264164, -138.7109808024214885 ) ) ;
#9239=CARTESIAN_POINT ( 'NONE',  ( -3.310556943750001313, 17.50000000000002132, -121.7641058028994792 ) ) ;
#9242=CARTESIAN_POINT ( 'NONE',  ( -1.394453263437886604E-15, 14.00000000000001066, -27.40473080337743284 ) ) ;
#9243=CARTESIAN_POINT ( 'NONE',  ( -1.749999999999999778, 20.53108891324555429, -92.12764746908815994 ) ) ;
#9244=CARTESIAN_POINT ( 'NONE',  ( 2.340729813953370519E-16, 21.32270188528331900, -118.1016058028994706 ) ) ;
#9246=CARTESIAN_POINT ( 'NONE',  ( 3.500000000000001776, 19.52072594216370405, -34.07139747004410424 ) ) ;
#9247=CARTESIAN_POINT ( 'NONE',  ( 0.9378221735089300459, 21.00000000000001776, -91.94938900211593591 ) ) ;
#9249=CARTESIAN_POINT ( 'NONE',  ( -3.310556943750000425, 19.41135094264167549, -139.9349391362327708 ) ) ;
#9252=CARTESIAN_POINT ( 'NONE',  ( -1.655278471874999990, 20.36702641396248836, -49.01827246956613493 ) ) ;
#9255=CARTESIAN_POINT ( 'NONE',  ( 3.310556943750001313, 19.41135094264166128, -70.26827246956612782 ) ) ;
#9257=CARTESIAN_POINT ( 'NONE',  ( -3.310556943750002645, 15.58864905735837070, -68.68077246956613635 ) ) ;
#9258=EDGE_LOOP ( 'NONE', ( #29089, #15917, #17067, #16332 ) ) ;
#9259=CARTESIAN_POINT ( 'NONE',  ( -3.310556943750000425, 19.41135094264166838, -89.93493913623279923 ) ) ;
#9263=CARTESIAN_POINT ( 'NONE',  ( 4.648177544792955347E-16, 21.00000000000001421, -62.21098080242150274 ) ) ;
#9264=DIRECTION ( 'NONE',  ( 0.000000000000000000, 1.000000000000000000, 0.000000000000000000 ) ) ;
#9265=LINE ( 'NONE', #15446, #36127 ) ;
#9266=CARTESIAN_POINT ( 'NONE',  ( -3.310556943750000425, 19.41135094264166483, -52.84743913623281486 ) ) ;
#9267=CARTESIAN_POINT ( 'NONE',  ( -3.500000000000001332, 17.50000000000001066, -24.65473080337743284 ) ) ;
#9268=CARTESIAN_POINT ( 'NONE',  ( -3.310556943750002645, 15.58864905735837425, -105.6807724695661364 ) ) ;
#9269=CARTESIAN_POINT ( 'NONE',  ( -3.500000000000002220, 15.47927405783632082, -35.87764746908816704 ) ) ;
#9270=( BOUNDED_CURVE ( )  B_SPLINE_CURVE ( 2, ( #672, #17272, #29596, #23007, #39163, #17055, #7698, #893, #30235 ),
 .UNSPECIFIED., .F., .T. ) 
 B_SPLINE_CURVE_WITH_KNOTS ( ( 3, 2, 2, 2, 3 ),
 ( 0.6729166666666667185, 0.6736111111111111605, 0.6750000000000000444, 0.6763888888888889284, 0.6770833333333333703 ),
 .UNSPECIFIED. ) 
 CURVE ( )  GEOMETRIC_REPRESENTATION_ITEM ( )  RATIONAL_B_SPLINE_CURVE ( ( 0.9330127018922194093, 0.9330127018922194093, 1.000000000000000000, 0.8660254037844387076, 1.000000000000000000, 0.8660254037844387076, 1.000000000000000000, 0.9330127018922194093, 0.9330127018922194093 ) ) 
 REPRESENTATION_ITEM ( '' )  );
#9271=EDGE_LOOP ( 'NONE', ( #10017, #19528, #8683, #32338 ) ) ;
#9276=CARTESIAN_POINT ( 'NONE',  ( 1.655278471874998436, 14.63297358603754184, -61.43077246956614346 ) ) ;
#9280=CARTESIAN_POINT ( 'NONE',  ( -1.749999999999999778, 20.53108891324556140, -142.8213974700441042 ) ) ;
#9282=DIRECTION ( 'NONE',  ( -0.000000000000000000, 1.259100132267607459E-16, -1.000000000000000000 ) ) ;
#9284=EDGE_CURVE ( 'NONE', #3209, #19458, #5528, .T. ) ;
#9285=FACE_OUTER_BOUND ( 'NONE', #20740, .T. ) ;
#9286=CARTESIAN_POINT ( 'NONE',  ( -1.655278471875002211, 14.63297358603755249, -124.5974391362328078 ) ) ;
#9287=CARTESIAN_POINT ( 'NONE',  ( 4.648177544792955347E-16, 21.00000000000002132, -119.2109808024215170 ) ) ;
#9290=CARTESIAN_POINT ( 'NONE',  ( -3.310556943750001313, 17.50000000000001066, -35.85160580289946353 ) ) ;
#9291=CARTESIAN_POINT ( 'NONE',  ( 3.310556943750001313, 19.41135094264165772, -26.26827246956613138 ) ) ;
#9292=CARTESIAN_POINT ( 'NONE',  ( 3.310556943750001313, 17.50000000000001776, -87.35160580289947063 ) ) ;
#9293=CARTESIAN_POINT ( 'NONE',  ( -1.655278471874999990, 20.36702641396249902, -140.9307724695661364 ) ) ;
#9297=CARTESIAN_POINT ( 'NONE',  ( -7.022189441860112050E-16, 13.67729811471672718, -134.6016058028994564 ) ) ;
#9299=CARTESIAN_POINT ( 'NONE',  ( 0.000000000000000000, 17.50000000000002487, -149.5231586289125687 ) ) ;
#9302=CARTESIAN_POINT ( 'NONE',  ( 3.500000000000001332, 17.50000000000001776, -82.15473080337743284 ) ) ;
#9303=CARTESIAN_POINT ( 'NONE',  ( 3.310556943750001313, 19.41135094264166483, -66.26827246956612782 ) ) ;
#9307=CARTESIAN_POINT ( 'NONE',  ( 3.310556943750001313, 17.50000000000001776, -87.35160580289947063 ) ) ;
#9308=CARTESIAN_POINT ( 'NONE',  ( -1.750000000000002220, 14.46891108675448656, -116.4880641367107614 ) ) ;
#9309=CARTESIAN_POINT ( 'NONE',  ( 3.310556943749999981, 15.58864905735837247, -115.3474391362327935 ) ) ;
#9312=VERTEX_POINT ( 'NONE', #41661 ) ;
#9313=CARTESIAN_POINT ( 'NONE',  ( -3.500000000000002220, 15.47927405783633503, -109.5713974700441042 ) ) ;
#9316=CARTESIAN_POINT ( 'NONE',  ( 4.648177544792955347E-16, 21.00000000000001421, -67.21098080242148853 ) ) ;
#9317=CYLINDRICAL_SURFACE ( 'NONE', #32592, 3.499999999999999556 ) ;
#9320=CARTESIAN_POINT ( 'NONE',  ( 1.655278471874998436, 14.63297358603754184, -67.43077246956613635 ) ) ;
#9321=CARTESIAN_POINT ( 'NONE',  ( 1.750000000000001110, 20.53108891324555074, -59.29431413575483845 ) ) ;
#9322=CARTESIAN_POINT ( 'NONE',  ( 2.340729813953370519E-16, 21.32270188528331900, -120.0141058028994792 ) ) ;
#9327=ADVANCED_FACE ( 'NONE', ( #31443 ), #15298, .T. ) ;
#9330=CARTESIAN_POINT ( 'NONE',  ( -7.022189441860112050E-16, 13.67729811471672186, -77.51410580289945074 ) ) ;
#9331=ORIENTED_EDGE ( 'NONE', *, *, #41548, .T. ) ;
#9332=ORIENTED_EDGE ( 'NONE', *, *, #15882, .F. ) ;
#9333=CARTESIAN_POINT ( 'NONE',  ( -3.500000000000002220, 15.47927405783632437, -48.57139747004410424 ) ) ;
#9334=ADVANCED_FACE ( 'NONE', ( #16762 ), #13144, .T. ) ;
#9335=( BOUNDED_CURVE ( )  B_SPLINE_CURVE ( 2, ( #10371, #17388, #1221, #14190, #40132, #7816, #6964, #8015, #40753 ),
 .UNSPECIFIED., .F., .F. ) 
 B_SPLINE_CURVE_WITH_KNOTS ( ( 3, 2, 2, 2, 3 ),
 ( 0.8895833333333332815, 0.8902777777777777235, 0.8916666666666667185, 0.8930555555555556024, 0.8937500000000000444 ),
 .UNSPECIFIED. ) 
 CURVE ( )  GEOMETRIC_REPRESENTATION_ITEM ( )  RATIONAL_B_SPLINE_CURVE ( ( 0.9330127018922194093, 0.9330127018922194093, 1.000000000000000000, 0.8660254037844387076, 1.000000000000000000, 0.8660254037844387076, 1.000000000000000000, 0.9330127018922194093, 0.9330127018922194093 ) ) 
 REPRESENTATION_ITEM ( '' )  );
#9336=CARTESIAN_POINT ( 'NONE',  ( 1.655278471874998436, 14.63297358603755249, -138.4307724695661364 ) ) ;
#9339=CARTESIAN_POINT ( 'NONE',  ( 1.655278471875001101, 20.36702641396248481, -44.18493913623279212 ) ) ;
#9340=CARTESIAN_POINT ( 'NONE',  ( -1.655278471874999990, 20.36702641396249547, -104.0182724695661278 ) ) ;
#9342=CARTESIAN_POINT ( 'NONE',  ( 3.310556943750001313, 17.50000000000001066, -30.26410580289948271 ) ) ;
#9343=CARTESIAN_POINT ( 'NONE',  ( 3.310556943749999981, 15.58864905735836537, -63.43493913623279923 ) ) ;
#9344=CARTESIAN_POINT ( 'NONE',  ( -7.424026671074350129E-16, 13.45854811567263809, -104.7109808024215027 ) ) ;
#9346=CARTESIAN_POINT ( 'NONE',  ( -3.500000000000000888, 19.52072594216371115, -94.73806413671076143 ) ) ;
#9347=CARTESIAN_POINT ( 'NONE',  ( -1.394453263437886604E-15, 14.00000000000001421, -63.71098080242150274 ) ) ;
#9350=CARTESIAN_POINT ( 'NONE',  ( 3.500000000000000000, 15.47927405783632260, -59.54431413575483845 ) ) ;
#9352=CARTESIAN_POINT ( 'NONE',  ( 2.340729813953370519E-16, 21.32270188528330479, -29.01410580289947916 ) ) ;
#9353=CARTESIAN_POINT ( 'NONE',  ( -3.500000000000002220, 15.47927405783632260, -49.57139747004410424 ) ) ;
#9355=EDGE_CURVE ( 'NONE', #7495, #33952, #5286, .T. ) ;
#9356=CARTESIAN_POINT ( 'NONE',  ( -3.310556943750002201, 15.58864905735836537, -33.76827246956613493 ) ) ;
#9361=DIRECTION ( 'NONE',  ( 0.000000000000000000, 1.000000000000000000, 0.000000000000000000 ) ) ;
#9363=CARTESIAN_POINT ( 'NONE',  ( 2.340729813953370519E-16, 21.32270188528331190, -80.01410580289946495 ) ) ;
#9366=ORIENTED_EDGE ( 'NONE', *, *, #6867, .F. ) ;
#9367=CARTESIAN_POINT ( 'NONE',  ( -1.750000000000002220, 14.46891108675448834, -123.7943141357548456 ) ) ;
#9368=CARTESIAN_POINT ( 'NONE',  ( 1.749999999999998224, 14.46891108675448123, -87.62764746908817415 ) ) ;
#9369=ORIENTED_EDGE ( 'NONE', *, *, #24236, .T. ) ;
#9372=CARTESIAN_POINT ( 'NONE',  ( 1.655278471875001101, 20.36702641396249192, -93.09743913623280775 ) ) ;
#9375=CARTESIAN_POINT ( 'NONE',  ( 0.9378221735089281585, 14.00000000000002132, -121.3600726046389155 ) ) ;
#9378=CARTESIAN_POINT ( 'NONE',  ( -4.648177544792955347E-16, 21.00000000000002487, -142.9047308033773902 ) ) ;
#9383=CARTESIAN_POINT ( 'NONE',  ( -3.500000000000000000, 19.52072594216371826, -127.7380641367107614 ) ) ;
#9384=( BOUNDED_CURVE ( )  B_SPLINE_CURVE ( 2, ( #9211, #15398, #2196, #35154, #8580, #2616, #1984, #31335, #18157 ),
 .UNSPECIFIED., .F., .F. ) 
 B_SPLINE_CURVE_WITH_KNOTS ( ( 3, 2, 2, 2, 3 ),
 ( 0.7270833333333333037, 0.7277777777777777457, 0.7291666666666666297, 0.7305555555555555136, 0.7312499999999999556 ),
 .UNSPECIFIED. ) 
 CURVE ( )  GEOMETRIC_REPRESENTATION_ITEM ( )  RATIONAL_B_SPLINE_CURVE ( ( 0.9330127018922194093, 0.9330127018922194093, 1.000000000000000000, 0.8660254037844387076, 1.000000000000000000, 0.8660254037844387076, 1.000000000000000000, 0.9330127018922194093, 0.9330127018922194093 ) ) 
 REPRESENTATION_ITEM ( '' )  );
#9385=DIRECTION ( 'NONE',  ( 0.000000000000000000, 1.000000000000000000, 0.000000000000000000 ) ) ;
#9386=CARTESIAN_POINT ( 'NONE',  ( -7.022189441860112050E-16, 13.67729811471672718, -130.5141058028994507 ) ) ;
#9388=VERTEX_POINT ( 'NONE', #6758 ) ;
#9389=CARTESIAN_POINT ( 'NONE',  ( -0.9378221735089291577, 21.00000000000002487, -141.1663226036829712 ) ) ;
#9390=CARTESIAN_POINT ( 'NONE',  ( 3.310556943750001313, 19.41135094264166838, -125.2682724695661136 ) ) ;
#9391=CARTESIAN_POINT ( 'NONE',  ( 3.310556943750001313, 19.41135094264166128, -51.26827246956612782 ) ) ;
#9392=EDGE_LOOP ( 'NONE', ( #17798, #5329, #25076, #33801 ) ) ;
#9393=CARTESIAN_POINT ( 'NONE',  ( 3.500000000000001776, 19.52072594216372181, -130.0713974700441042 ) ) ;
#9394=VECTOR ( 'NONE', #14955, 1000.000000000000000 ) ;
#9396=CARTESIAN_POINT ( 'NONE',  ( -3.310556943750002645, 15.58864905735837070, -75.76827246956612782 ) ) ;
#9397=CARTESIAN_POINT ( 'NONE',  ( 3.500000000000001776, 19.52072594216371826, -125.3776474690881599 ) ) ;
#9398=CARTESIAN_POINT ( 'NONE',  ( -7.022189441860112050E-16, 13.67729811471672541, -107.5141058028994507 ) ) ;
#9399=CARTESIAN_POINT ( 'NONE',  ( 1.749999999999998224, 14.46891108675448123, -93.32139747004409003 ) ) ;
#9402=CARTESIAN_POINT ( 'NONE',  ( -7.424026671074350129E-16, 13.45854811567263454, -75.71098080242151696 ) ) ;
#9404=CARTESIAN_POINT ( 'NONE',  ( 1.655278471875001101, 20.36702641396248481, -42.09743913623280065 ) ) ;
#9405=CARTESIAN_POINT ( 'NONE',  ( 3.310556943750001313, 17.50000000000001776, -101.3516058028994706 ) ) ;
#9406=CARTESIAN_POINT ( 'NONE',  ( 3.500000000000000000, 15.47927405783632615, -73.54431413575483134 ) ) ;
#9407=CARTESIAN_POINT ( 'NONE',  ( 3.500000000000001332, 17.50000000000001421, -64.15473080337743284 ) ) ;
#9410=CARTESIAN_POINT ( 'NONE',  ( 3.310556943750001313, 17.50000000000002132, -119.3516058028994706 ) ) ;
#9416=LINE ( 'NONE', #28967, #14514 ) ;
#9418=VECTOR ( 'NONE', #50, 1000.000000000000000 ) ;
#9419=VERTEX_POINT ( 'NONE', #26337 ) ;
#9420=CARTESIAN_POINT ( 'NONE',  ( 3.500000000000001332, 19.52072594216371826, -136.3776474690881741 ) ) ;
#9421=CARTESIAN_POINT ( 'NONE',  ( 1.749999999999998224, 14.46891108675447590, -40.32139747004409713 ) ) ;
#9425=CARTESIAN_POINT ( 'NONE',  ( 1.655278471874998436, 14.63297358603753828, -35.43077246956613635 ) ) ;
#9430=CARTESIAN_POINT ( 'NONE',  ( -0.9378221735089291577, 21.00000000000001776, -100.1663226036829855 ) ) ;
#9433=CARTESIAN_POINT ( 'NONE',  ( -0.9378221735089291577, 21.00000000000002132, -115.1663226036829997 ) ) ;
#9435=FACE_OUTER_BOUND ( 'NONE', #5560, .T. ) ;
#9436=CARTESIAN_POINT ( 'NONE',  ( -1.750000000000002220, 14.46891108675448656, -119.4880641367107614 ) ) ;
#9438=CARTESIAN_POINT ( 'NONE',  ( 1.750000000000001110, 20.53108891324554719, -35.29431413575484555 ) ) ;
#9439=CARTESIAN_POINT ( 'NONE',  ( -1.749999999999999778, 20.53108891324555074, -66.12764746908817415 ) ) ;
#9443=CARTESIAN_POINT ( 'NONE',  ( -1.749999999999999778, 20.53108891324556140, -140.1276474690881741 ) ) ;
#9444=CARTESIAN_POINT ( 'NONE',  ( 0.9378221735089300459, 21.00000000000002132, -120.2556390011600342 ) ) ;
#9445=CARTESIAN_POINT ( 'NONE',  ( 3.310556943750001313, 19.41135094264166838, -121.1807724695661506 ) ) ;
#9450=CARTESIAN_POINT ( 'NONE',  ( -3.500000000000002220, 15.47927405783632793, -92.87764746908815994 ) ) ;
#9451=CARTESIAN_POINT ( 'NONE',  ( 1.749999999999998224, 14.46891108675447413, -33.32139747004410424 ) ) ;
#9452=CARTESIAN_POINT ( 'NONE',  ( -3.310556943750001313, 17.50000000000001421, -58.76410580289947916 ) ) ;
#9454=CARTESIAN_POINT ( 'NONE',  ( 2.340729813953370519E-16, 21.32270188528331900, -119.1016058028994564 ) ) ;
#9455=CARTESIAN_POINT ( 'NONE',  ( -1.394453263437886604E-15, 14.00000000000001421, -79.40473080337741862 ) ) ;
#9456=CARTESIAN_POINT ( 'NONE',  ( 1.749999999999998224, 14.46891108675447413, -33.32139747004410424 ) ) ;
#9457=DIRECTION ( 'NONE',  ( 0.000000000000000000, 1.000000000000000000, 0.000000000000000000 ) ) ;
#9459=CARTESIAN_POINT ( 'NONE',  ( 3.310556943750001313, 17.50000000000002487, -136.3516058028994564 ) ) ;
#9461=CARTESIAN_POINT ( 'NONE',  ( -3.500000000000002220, 15.47927405783632615, -66.57139747004409003 ) ) ;
#9462=CARTESIAN_POINT ( 'NONE',  ( -3.310556943750002201, 15.58864905735836714, -42.76827246956613493 ) ) ;
#9464=LINE ( 'NONE', #22430, #33980 ) ;
#9465=CARTESIAN_POINT ( 'NONE',  ( -3.310556943750001313, 17.50000000000001421, -67.85160580289947063 ) ) ;
#9467=CARTESIAN_POINT ( 'NONE',  ( -1.655278471874999990, 20.36702641396248836, -62.93077246956614346 ) ) ;
#9469=CARTESIAN_POINT ( 'NONE',  ( 3.310556943749999981, 15.58864905735836892, -92.43493913623279923 ) ) ;
#9471=CARTESIAN_POINT ( 'NONE',  ( -1.394453263437886604E-15, 14.00000000000001421, -67.71098080242148853 ) ) ;
#9473=CARTESIAN_POINT ( 'NONE',  ( -3.500000000000001332, 17.50000000000001421, -69.96098080242151696 ) ) ;
#9474=CARTESIAN_POINT ( 'NONE',  ( 1.655278471875001101, 20.36702641396248836, -48.09743913623280775 ) ) ;
#9477=CARTESIAN_POINT ( 'NONE',  ( 1.655278471875001101, 20.36702641396249547, -108.0974391362328078 ) ) ;
#9478=CARTESIAN_POINT ( 'NONE',  ( -0.9378221735089310451, 14.00000000000002132, -101.4493890021159501 ) ) ;
#9485=CARTESIAN_POINT ( 'NONE',  ( -3.310556943750001313, 17.50000000000001421, -57.76410580289947916 ) ) ;
#9487=ORIENTED_EDGE ( 'NONE', *, *, #27816, .F. ) ;
#9488=FACE_OUTER_BOUND ( 'NONE', #15544, .T. ) ;
#9489=CARTESIAN_POINT ( 'NONE',  ( -3.500000000000000000, 19.52072594216370405, -40.73806413671076143 ) ) ;
#9491=FACE_OUTER_BOUND ( 'NONE', #24094, .T. ) ;
#9492=ORIENTED_EDGE ( 'NONE', *, *, #27667, .T. ) ;
#9493=CARTESIAN_POINT ( 'NONE',  ( 3.500000000000001332, 17.50000000000002487, -143.4609808024215170 ) ) ;
#9494=CARTESIAN_POINT ( 'NONE',  ( 2.340729813953370519E-16, 21.32270188528331900, -125.0141058028994792 ) ) ;
#9499=CARTESIAN_POINT ( 'NONE',  ( -7.022189441860112050E-16, 13.67729811471671475, -35.60160580289946353 ) ) ;
#9500=CARTESIAN_POINT ( 'NONE',  ( -3.310556943750002645, 15.58864905735836537, -26.76827246956613493 ) ) ;
#9501=CARTESIAN_POINT ( 'NONE',  ( 2.340729813953370519E-16, 21.32270188528331190, -89.10160580289947063 ) ) ;
#9502=CARTESIAN_POINT ( 'NONE',  ( -1.655278471874999990, 20.36702641396249902, -136.9307724695661364 ) ) ;
#9506=( BOUNDED_CURVE ( )  B_SPLINE_CURVE ( 2, ( #9230, #35169, #6034, #25819, #19010, #31977, #38783, #22616, #6457 ),
 .UNSPECIFIED., .F., .T. ) 
 B_SPLINE_CURVE_WITH_KNOTS ( ( 3, 2, 2, 2, 3 ),
 ( 0.9104166666666666519, 0.9111111111111110938, 0.9124999999999999778, 0.9138888888888888618, 0.9145833333333333037 ),
 .UNSPECIFIED. ) 
 CURVE ( )  GEOMETRIC_REPRESENTATION_ITEM ( )  RATIONAL_B_SPLINE_CURVE ( ( 0.9330127018922194093, 0.9330127018922194093, 1.000000000000000000, 0.8660254037844387076, 1.000000000000000000, 0.8660254037844387076, 1.000000000000000000, 0.9330127018922194093, 0.9330127018922194093 ) ) 
 REPRESENTATION_ITEM ( '' )  );
#9507=CARTESIAN_POINT ( 'NONE',  ( -3.310556943750001313, 17.50000000000002487, -132.8516058028994564 ) ) ;
#9510=CARTESIAN_POINT ( 'NONE',  ( -3.500000000000000000, 19.52072594216371115, -76.04431413575484555 ) ) ;
#9512=CARTESIAN_POINT ( 'NONE',  ( 3.500000000000001332, 17.50000000000001776, -81.15473080337743284 ) ) ;
#9513=CARTESIAN_POINT ( 'NONE',  ( -3.310556943750001313, 17.50000000000001421, -64.85160580289945642 ) ) ;
#9516=DIRECTION ( 'NONE',  ( -0.000000000000000000, 1.259100132267607459E-16, -1.000000000000000000 ) ) ;
#9517=CARTESIAN_POINT ( 'NONE',  ( 1.655278471875001101, 20.36702641396249192, -83.18493913623278502 ) ) ;
#9519=CARTESIAN_POINT ( 'NONE',  ( -3.310556943750001313, 17.50000000000002132, -116.7641058028994792 ) ) ;
#9521=CARTESIAN_POINT ( 'NONE',  ( 0.9378221735089300459, 21.00000000000001421, -56.94938900211595012 ) ) ;
#9523=( BOUNDED_CURVE ( )  B_SPLINE_CURVE ( 2, ( #29599, #38764, #39374, #3443, #3870, #9420, #6639, #19407, #10251 ),
 .UNSPECIFIED., .F., .T. ) 
 B_SPLINE_CURVE_WITH_KNOTS ( ( 3, 2, 2, 2, 3 ),
 ( 0.05625000000000000139, 0.05694444444444444337, 0.05833333333333333426, 0.05972222222222222515, 0.06041666666666666713 ),
 .UNSPECIFIED. ) 
 CURVE ( )  GEOMETRIC_REPRESENTATION_ITEM ( )  RATIONAL_B_SPLINE_CURVE ( ( 0.9330127018922192983, 0.9330127018922196314, 1.000000000000000000, 0.8660254037844387076, 1.000000000000000000, 0.8660254037844387076, 1.000000000000000000, 0.9330127018922194093, 0.9330127018922194093 ) ) 
 REPRESENTATION_ITEM ( '' )  );
#9524=VECTOR ( 'NONE', #34205, 1000.000000000000000 ) ;
#9525=CARTESIAN_POINT ( 'NONE',  ( -3.500000000000001332, 17.50000000000002132, -108.6547308033774186 ) ) ;
#9529=CARTESIAN_POINT ( 'NONE',  ( 1.749999999999998224, 14.46891108675447590, -48.62764746908818125 ) ) ;
#9533=CARTESIAN_POINT ( 'NONE',  ( -3.310556943750001313, 17.50000000000001421, -66.76410580289947916 ) ) ;
#9534=EDGE_CURVE ( 'NONE', #16391, #14818, #29995, .T. ) ;
#9535=EDGE_CURVE ( 'NONE', #9312, #16027, #36100, .T. ) ;
#9537=CARTESIAN_POINT ( 'NONE',  ( -3.310556943750001313, 17.50000000000002132, -120.7641058028994792 ) ) ;
#9542=CARTESIAN_POINT ( 'NONE',  ( 3.500000000000001332, 19.52072594216371115, -99.37764746908815994 ) ) ;
#9543=CARTESIAN_POINT ( 'NONE',  ( -3.500000000000001332, 17.50000000000001066, -31.96098080242150274 ) ) ;
#9544=CARTESIAN_POINT ( 'NONE',  ( 1.655278471875001101, 20.36702641396248836, -72.09743913623280775 ) ) ;
#9549=CARTESIAN_POINT ( 'NONE',  ( 3.310556943750001313, 17.50000000000002487, -140.2641058028994792 ) ) ;
#9550=CARTESIAN_POINT ( 'NONE',  ( -1.749999999999999778, 20.53108891324555074, -51.82139747004409003 ) ) ;
#9552=CARTESIAN_POINT ( 'NONE',  ( -1.749999999999999778, 20.53108891324555785, -113.8213974700440900 ) ) ;
#9553=CARTESIAN_POINT ( 'NONE',  ( 2.340729813953370519E-16, 21.32270188528330479, -42.10160580289947063 ) ) ;
#9554=CARTESIAN_POINT ( 'NONE',  ( -1.655278471875002211, 14.63297358603754894, -101.6849391362327992 ) ) ;
#9555=EDGE_CURVE ( 'NONE', #33623, #8219, #21559, .T. ) ;
#9556=CARTESIAN_POINT ( 'NONE',  ( -1.655278471875002211, 14.63297358603754006, -27.59743913623280420 ) ) ;
#9557=CARTESIAN_POINT ( 'NONE',  ( -1.749999999999999778, 20.53108891324555785, -112.1276474690881884 ) ) ;
#9558=CARTESIAN_POINT ( 'NONE',  ( 3.500000000000001332, 17.50000000000002132, -107.4609808024215027 ) ) ;
#9561=CARTESIAN_POINT ( 'NONE',  ( 0.9378221735089287137, 14.00000000000002665, -142.3600726046389298 ) ) ;
#9562=CARTESIAN_POINT ( 'NONE',  ( -3.500000000000002220, 15.47927405783632793, -94.57139747004409003 ) ) ;
#9566=CARTESIAN_POINT ( 'NONE',  ( 1.749999999999998224, 14.46891108675447768, -61.62764746908818125 ) ) ;
#9569=CARTESIAN_POINT ( 'NONE',  ( 1.655278471874998436, 14.63297358603753828, -29.43077246956614346 ) ) ;
#9570=CARTESIAN_POINT ( 'NONE',  ( 1.749999999999998224, 14.46891108675447590, -51.32139747004409003 ) ) ;
#9571=CARTESIAN_POINT ( 'NONE',  ( 0.9378221735089281585, 14.00000000000001599, -77.66632260368297125 ) ) ;
#9572=CARTESIAN_POINT ( 'NONE',  ( -1.655278471874999990, 20.36702641396248481, -31.01827246956613493 ) ) ;
#9579=CARTESIAN_POINT ( 'NONE',  ( 1.655278471874998436, 14.63297358603754539, -81.43077246956615056 ) ) ;
#9584=EDGE_CURVE ( 'NONE', #30046, #23990, #11257, .T. ) ;
#9585=ORIENTED_EDGE ( 'NONE', *, *, #41964, .T. ) ;
#9588=CARTESIAN_POINT ( 'NONE',  ( -3.310556943750000425, 19.41135094264166483, -88.84743913623279354 ) ) ;
#9589=( BOUNDED_CURVE ( )  B_SPLINE_CURVE ( 2, ( #38176, #34364, #21592, #18825, #34566, #9040, #41170, #12016, #25008 ),
 .UNSPECIFIED., .F., .T. ) 
 B_SPLINE_CURVE_WITH_KNOTS ( ( 3, 2, 2, 2, 3 ),
 ( 0.3229166666666666852, 0.3236111111111111271, 0.3250000000000000111, 0.3263888888888888951, 0.3270833333333333370 ),
 .UNSPECIFIED. ) 
 CURVE ( )  GEOMETRIC_REPRESENTATION_ITEM ( )  RATIONAL_B_SPLINE_CURVE ( ( 0.9330127018922194093, 0.9330127018922194093, 1.000000000000000000, 0.8660254037844387076, 1.000000000000000000, 0.8660254037844387076, 1.000000000000000000, 0.9330127018922194093, 0.9330127018922194093 ) ) 
 REPRESENTATION_ITEM ( '' )  );
#9597=ORIENTED_EDGE ( 'NONE', *, *, #40769, .F. ) ;
#9599=CARTESIAN_POINT ( 'NONE',  ( -1.749999999999999778, 20.53108891324555429, -88.82139747004410424 ) ) ;
#9601=CARTESIAN_POINT ( 'NONE',  ( -1.655278471875002211, 14.63297358603755249, -132.5974391362328220 ) ) ;
#9602=EDGE_LOOP ( 'NONE', ( #7613, #27939, #14830, #40469 ) ) ;
#9604=CARTESIAN_POINT ( 'NONE',  ( 1.655278471874998436, 14.63297358603754894, -117.5182724695661278 ) ) ;
#9605=CARTESIAN_POINT ( 'NONE',  ( -7.022189441860112050E-16, 13.67729811471671653, -52.60160580289947063 ) ) ;
#9607=CARTESIAN_POINT ( 'NONE',  ( 3.500000000000000000, 15.47927405783633503, -133.2380641367107899 ) ) ;
#9610=CARTESIAN_POINT ( 'NONE',  ( -3.310556943750001313, 17.50000000000001421, -70.85160580289947063 ) ) ;
#9611=CARTESIAN_POINT ( 'NONE',  ( -3.500000000000002220, 15.47927405783633503, -124.8776474690881599 ) ) ;
#9612=CARTESIAN_POINT ( 'NONE',  ( -1.655278471875002211, 14.63297358603754894, -107.5974391362328078 ) ) ;
#9613=CARTESIAN_POINT ( 'NONE',  ( -1.394453263437886604E-15, 14.00000000000001421, -74.40473080337743284 ) ) ;
#9616=CARTESIAN_POINT ( 'NONE',  ( 3.500000000000001776, 19.52072594216371115, -77.37764746908817415 ) ) ;
#9617=CARTESIAN_POINT ( 'NONE',  ( -0.9378221735089310451, 14.00000000000001066, -50.75563900116003424 ) ) ;
#9618=CARTESIAN_POINT ( 'NONE',  ( 3.310556943750001313, 19.41135094264165772, -45.18077246956613635 ) ) ;
#9619=CARTESIAN_POINT ( 'NONE',  ( -1.655278471875002211, 14.63297358603754894, -100.6849391362327992 ) ) ;
#9621=CARTESIAN_POINT ( 'NONE',  ( -1.749999999999999778, 20.53108891324555074, -62.82139747004410424 ) ) ;
#9623=EDGE_LOOP ( 'NONE', ( #28896, #2674, #18488, #16851 ) ) ;
#9624=CARTESIAN_POINT ( 'NONE',  ( -3.310556943750001313, 17.50000000000002132, -116.8516058028994706 ) ) ;
#9625=CARTESIAN_POINT ( 'NONE',  ( -1.750000000000002220, 14.46891108675449011, -136.4880641367107614 ) ) ;
#9631=CARTESIAN_POINT ( 'NONE',  ( -1.655278471875002211, 14.63297358603754894, -98.59743913623280775 ) ) ;
#9635=DIRECTION ( 'NONE',  ( 0.000000000000000000, 1.000000000000000000, 0.000000000000000000 ) ) ;
#9636=CARTESIAN_POINT ( 'NONE',  ( -3.500000000000001332, 17.50000000000002132, -118.6547308033774328 ) ) ;
#9640=CARTESIAN_POINT ( 'NONE',  ( -1.655278471875002211, 14.63297358603754006, -33.59743913623280775 ) ) ;
#9642=( BOUNDED_CURVE ( )  B_SPLINE_CURVE ( 2, ( #21908, #34676, #18730, #38077, #12120, #31692, #18303, #31275, #2138 ),
 .UNSPECIFIED., .F., .F. ) 
 B_SPLINE_CURVE_WITH_KNOTS ( ( 3, 2, 2, 2, 3 ),
 ( 0.9937500000000000222, 0.9944444444444444642, 0.9958333333333333481, 0.9972222222222222321, 0.9979166666666666741 ),
 .UNSPECIFIED. ) 
 CURVE ( )  GEOMETRIC_REPRESENTATION_ITEM ( )  RATIONAL_B_SPLINE_CURVE ( ( 0.9330127018922194093, 0.9330127018922194093, 1.000000000000000000, 0.8660254037844387076, 1.000000000000000000, 0.8660254037844387076, 1.000000000000000000, 0.9330127018922194093, 0.9330127018922194093 ) ) 
 REPRESENTATION_ITEM ( '' )  );
#9645=ORIENTED_EDGE ( 'NONE', *, *, #8280, .T. ) ;
#9647=CARTESIAN_POINT ( 'NONE',  ( -1.394453263437886604E-15, 14.00000000000001776, -99.71098080242150274 ) ) ;
#9648=ORIENTED_EDGE ( 'NONE', *, *, #28793, .F. ) ;
#9650=DIRECTION ( 'NONE',  ( 0.000000000000000000, 1.000000000000000000, 0.000000000000000000 ) ) ;
#9653=CARTESIAN_POINT ( 'NONE',  ( -3.500000000000000888, 19.52072594216371826, -116.7380641367107472 ) ) ;
#9654=EDGE_CURVE ( 'NONE', #14503, #3516, #27789, .T. ) ;
#9657=CARTESIAN_POINT ( 'NONE',  ( 3.310556943749999981, 15.58864905735837425, -136.4349391362327992 ) ) ;
#9658=CARTESIAN_POINT ( 'NONE',  ( -1.750000000000002220, 14.46891108675447590, -30.79431413575484200 ) ) ;
#9661=CARTESIAN_POINT ( 'NONE',  ( -1.394453263437886604E-15, 14.00000000000001776, -106.4047308033774328 ) ) ;
#9663=CARTESIAN_POINT ( 'NONE',  ( -1.750000000000002220, 14.46891108675449011, -137.7943141357548598 ) ) ;
#9664=CARTESIAN_POINT ( 'NONE',  ( 3.500000000000001332, 19.52072594216371826, -120.3776474690881599 ) ) ;
#9665=CARTESIAN_POINT ( 'NONE',  ( -3.310556943750000425, 19.41135094264166838, -124.8474391362328078 ) ) ;
#9667=ORIENTED_EDGE ( 'NONE', *, *, #42080, .T. ) ;
#9669=CARTESIAN_POINT ( 'NONE',  ( -1.750000000000002220, 14.46891108675448301, -81.79431413575484555 ) ) ;
#9670=CARTESIAN_POINT ( 'NONE',  ( 3.500000000000001332, 17.50000000000001776, -92.46098080242151696 ) ) ;
#9671=FACE_OUTER_BOUND ( 'NONE', #29022, .T. ) ;
#9672=CARTESIAN_POINT ( 'NONE',  ( -3.310556943750002645, 15.58864905735836892, -59.68077246956615056 ) ) ;
#9673=CARTESIAN_POINT ( 'NONE',  ( 3.310556943750001313, 19.41135094264166838, -119.2682724695661278 ) ) ;
#9674=DIRECTION ( 'NONE',  ( 0.000000000000000000, 1.000000000000000000, 0.000000000000000000 ) ) ;
#9675=CARTESIAN_POINT ( 'NONE',  ( -1.750000000000002220, 14.46891108675447590, -31.48806413671076498 ) ) ;
#9676=CARTESIAN_POINT ( 'NONE',  ( 3.500000000000000000, 15.47927405783632793, -92.23806413671076143 ) ) ;
#9678=CARTESIAN_POINT ( 'NONE',  ( 2.340729813953370519E-16, 21.32270188528332255, -134.1016058028994564 ) ) ;
#9679=EDGE_CURVE ( 'NONE', #18588, #19149, #40354, .T. ) ;
#9681=DIRECTION ( 'NONE',  ( 0.000000000000000000, 1.000000000000000000, 0.000000000000000000 ) ) ;
#9682=CARTESIAN_POINT ( 'NONE',  ( -3.310556943750001313, 17.50000000000001066, -45.85160580289945642 ) ) ;
#9684=CARTESIAN_POINT ( 'NONE',  ( -3.310556943750002645, 15.58864905735837070, -70.76827246956612782 ) ) ;
#9686=CARTESIAN_POINT ( 'NONE',  ( -3.310556943750000425, 19.41135094264166128, -65.84743913623280775 ) ) ;
#9687=ORIENTED_EDGE ( 'NONE', *, *, #30841, .T. ) ;
#9688=CARTESIAN_POINT ( 'NONE',  ( -7.022189441860112050E-16, 13.67729811471672363, -83.60160580289947063 ) ) ;
#9692=CARTESIAN_POINT ( 'NONE',  ( -0.9378221735089310451, 14.00000000000002132, -84.75563900116002003 ) ) ;
#9694=CARTESIAN_POINT ( 'NONE',  ( -3.500000000000000000, 19.52072594216370405, -42.04431413575483845 ) ) ;
#9695=CARTESIAN_POINT ( 'NONE',  ( -3.310556943750001313, 17.50000000000001421, -47.76410580289947205 ) ) ;
#9698=CARTESIAN_POINT ( 'NONE',  ( 2.340729813953370519E-16, 21.32270188528331900, -107.0141058028994649 ) ) ;
#9699=ORIENTED_EDGE ( 'NONE', *, *, #15882, .T. ) ;
#9702=VERTEX_POINT ( 'NONE', #30986 ) ;
#9704=CARTESIAN_POINT ( 'NONE',  ( -1.655278471874999990, 20.36702641396248836, -59.93077246956614346 ) ) ;
#9707=CARTESIAN_POINT ( 'NONE',  ( 0.000000000000000000, 17.50000000000002487, -149.5231586289125687 ) ) ;
#9710=CARTESIAN_POINT ( 'NONE',  ( -3.500000000000002220, 15.47927405783633503, -140.5713974700441042 ) ) ;
#9712=FACE_OUTER_BOUND ( 'NONE', #37065, .T. ) ;
#9713=CARTESIAN_POINT ( 'NONE',  ( -7.022189441860112050E-16, 13.67729811471672896, -125.5141058028994792 ) ) ;
#9716=CARTESIAN_POINT ( 'NONE',  ( -3.310556943750002645, 15.58864905735836537, -35.76827246956612782 ) ) ;
#9717=CARTESIAN_POINT ( 'NONE',  ( 3.310556943749999981, 15.58864905735836182, -29.43493913623279923 ) ) ;
#9719=CARTESIAN_POINT ( 'NONE',  ( -3.310556943750002645, 15.58864905735837247, -85.76827246956612782 ) ) ;
#9720=CARTESIAN_POINT ( 'NONE',  ( 3.310556943749999981, 15.58864905735837780, -140.3474391362327935 ) ) ;
#9722=EDGE_CURVE ( 'NONE', #29810, #8481, #3663, .T. ) ;
#9726=CARTESIAN_POINT ( 'NONE',  ( 3.310556943750001313, 17.50000000000002487, -133.3516058028994564 ) ) ;
#9727=CARTESIAN_POINT ( 'NONE',  ( 3.500000000000001332, 17.50000000000001421, -56.46098080242150985 ) ) ;
#9728=CARTESIAN_POINT ( 'NONE',  ( 3.310556943749999981, 15.58864905735836892, -91.34743913623280775 ) ) ;
#9730=CARTESIAN_POINT ( 'NONE',  ( -0.9378221735089310451, 14.00000000000001599, -75.75563900116003424 ) ) ;
#9731=DIRECTION ( 'NONE',  ( 0.000000000000000000, 1.000000000000000000, 0.000000000000000000 ) ) ;
#9732=CARTESIAN_POINT ( 'NONE',  ( 2.474675557024783212E-16, 21.54145188432739388, -73.90473080337743284 ) ) ;
#9733=CARTESIAN_POINT ( 'NONE',  ( 1.655278471874998436, 14.63297358603754184, -60.51827246956613493 ) ) ;
#9737=CARTESIAN_POINT ( 'NONE',  ( 3.310556943750001313, 17.50000000000001776, -83.35160580289947063 ) ) ;
#9738=CARTESIAN_POINT ( 'NONE',  ( 3.310556943750001313, 19.41135094264167549, -143.2682724695661420 ) ) ;
#9739=CARTESIAN_POINT ( 'NONE',  ( -1.655278471874999990, 20.36702641396249547, -116.9307724695661364 ) ) ;
#9740=CARTESIAN_POINT ( 'NONE',  ( 1.655278471874998436, 14.63297358603754539, -83.43077246956615056 ) ) ;
#9741=FACE_OUTER_BOUND ( 'NONE', #23670, .T. ) ;
#9742=ORIENTED_EDGE ( 'NONE', *, *, #4871, .T. ) ;
#9743=CARTESIAN_POINT ( 'NONE',  ( -3.500000000000000888, 19.52072594216371826, -108.7380641367107614 ) ) ;
#9746=CARTESIAN_POINT ( 'NONE',  ( 0.9378221735089281585, 14.00000000000002132, -105.3600726046389155 ) ) ;
#9748=CARTESIAN_POINT ( 'NONE',  ( -1.750000000000002220, 14.46891108675447590, -32.48806413671076143 ) ) ;
#9750=CARTESIAN_POINT ( 'NONE',  ( 3.310556943750001313, 17.50000000000001421, -64.26410580289946495 ) ) ;
#9753=CARTESIAN_POINT ( 'NONE',  ( 3.310556943750001313, 19.41135094264166838, -124.1807724695661364 ) ) ;
#9758=CARTESIAN_POINT ( 'NONE',  ( 4.648177544792955347E-16, 21.00000000000001066, -43.21098080242150985 ) ) ;
#9760=CARTESIAN_POINT ( 'NONE',  ( 3.500000000000001332, 19.52072594216371826, -128.0713974700441042 ) ) ;
#9761=CARTESIAN_POINT ( 'NONE',  ( 1.655278471875001101, 20.36702641396249192, -76.09743913623280775 ) ) ;
#9764=VERTEX_POINT ( 'NONE', #32824 ) ;
#9767=CARTESIAN_POINT ( 'NONE',  ( 1.655278471875001101, 20.36702641396249902, -140.0974391362327935 ) ) ;
#9769=( BOUNDED_CURVE ( )  B_SPLINE_CURVE ( 2, ( #10702, #17085, #13676, #7514, #33456, #17716, #20905, #33877, #20702 ),
 .UNSPECIFIED., .F., .F. ) 
 B_SPLINE_CURVE_WITH_KNOTS ( ( 3, 2, 2, 2, 3 ),
 ( 0.1645833333333333315, 0.1652777777777777735, 0.1666666666666666574, 0.1680555555555555691, 0.1687500000000000111 ),
 .UNSPECIFIED. ) 
 CURVE ( )  GEOMETRIC_REPRESENTATION_ITEM ( )  RATIONAL_B_SPLINE_CURVE ( ( 0.9330127018922194093, 0.9330127018922194093, 1.000000000000000000, 0.8660254037844387076, 1.000000000000000000, 0.8660254037844387076, 1.000000000000000000, 0.9330127018922194093, 0.9330127018922194093 ) ) 
 REPRESENTATION_ITEM ( '' )  );
#9770=EDGE_CURVE ( 'NONE', #3209, #38468, #6677, .T. ) ;
#9771=DIRECTION ( 'NONE',  ( -0.000000000000000000, 1.259100132267607459E-16, -1.000000000000000000 ) ) ;
#9772=CARTESIAN_POINT ( 'NONE',  ( 2.340729813953370519E-16, 21.32270188528330479, -44.10160580289946353 ) ) ;
#9773=CARTESIAN_POINT ( 'NONE',  ( 3.310556943750001313, 17.50000000000002132, -105.3516058028994564 ) ) ;
#9774=EDGE_CURVE ( 'NONE', #21610, #29219, #40069, .T. ) ;
#9775=CARTESIAN_POINT ( 'NONE',  ( 1.655278471874998436, 14.63297358603753828, -31.43077246956614701 ) ) ;
#9777=CARTESIAN_POINT ( 'NONE',  ( -3.500000000000000888, 19.52072594216371826, -108.0443141357548740 ) ) ;
#9779=DIRECTION ( 'NONE',  ( 0.000000000000000000, 1.000000000000000000, 0.000000000000000000 ) ) ;
#9780=CARTESIAN_POINT ( 'NONE',  ( 3.500000000000001332, 17.50000000000001776, -94.15473080337744705 ) ) ;
#9784=CARTESIAN_POINT ( 'NONE',  ( 3.500000000000001332, 17.50000000000001421, -61.46098080242150274 ) ) ;
#9787=CARTESIAN_POINT ( 'NONE',  ( 3.500000000000000000, 15.47927405783632082, -47.23806413671076854 ) ) ;
#9790=CARTESIAN_POINT ( 'NONE',  ( -1.655278471874999990, 20.36702641396248481, -35.01827246956614204 ) ) ;
#9793=CARTESIAN_POINT ( 'NONE',  ( -1.394453263437886604E-15, 14.00000000000002132, -120.7109808024215170 ) ) ;
#9797=CARTESIAN_POINT ( 'NONE',  ( -3.310556943750001313, 17.50000000000001776, -80.76410580289946495 ) ) ;
#9798=CYLINDRICAL_SURFACE ( 'NONE', #8703, 3.499999999999999556 ) ;
#9799=ORIENTED_EDGE ( 'NONE', *, *, #7183, .T. ) ;
#9801=LINE ( 'NONE', #22759, #18972 ) ;
#9803=DIRECTION ( 'NONE',  ( 0.000000000000000000, 1.000000000000000000, 0.000000000000000000 ) ) ;
#9804=CARTESIAN_POINT ( 'NONE',  ( 1.655278471874998436, 14.63297358603754539, -89.43077246956613635 ) ) ;
#9805=ORIENTED_EDGE ( 'NONE', *, *, #15775, .T. ) ;
#9807=VERTEX_POINT ( 'NONE', #37295 ) ;
#9811=EDGE_CURVE ( 'NONE', #32641, #35947, #21310, .T. ) ;
#9813=CARTESIAN_POINT ( 'NONE',  ( -3.500000000000002220, 15.47927405783633503, -127.5713974700440900 ) ) ;
#9814=CARTESIAN_POINT ( 'NONE',  ( 3.500000000000001332, 19.52072594216371826, -129.3776474690881741 ) ) ;
#9815=CARTESIAN_POINT ( 'NONE',  ( -3.310556943750001313, 17.50000000000002487, -129.7641058028994507 ) ) ;
#9818=ORIENTED_EDGE ( 'NONE', *, *, #904, .F. ) ;
#9819=CARTESIAN_POINT ( 'NONE',  ( 0.9378221735089300459, 21.00000000000002487, -138.9493890021159643 ) ) ;
#9820=CARTESIAN_POINT ( 'NONE',  ( 1.655278471875001101, 20.36702641396249547, -122.1849391362327992 ) ) ;
#9821=CARTESIAN_POINT ( 'NONE',  ( 1.655278471875001101, 20.36702641396248836, -48.18493913623279923 ) ) ;
#9822=VERTEX_POINT ( 'NONE', #4542 ) ;
#9823=ADVANCED_FACE ( 'NONE', ( #11749 ), #36879, .T. ) ;
#9824=CARTESIAN_POINT ( 'NONE',  ( -3.500000000000002220, 15.47927405783633503, -128.5713974700440758 ) ) ;
#9826=CARTESIAN_POINT ( 'NONE',  ( -3.310556943750002645, 15.58864905735837070, -69.76827246956612782 ) ) ;
#9827=CARTESIAN_POINT ( 'NONE',  ( 1.749999999999998224, 14.46891108675448478, -121.6276474690881741 ) ) ;
#9828=CARTESIAN_POINT ( 'NONE',  ( -3.310556943750000425, 19.41135094264166838, -104.8474391362328078 ) ) ;
#9829=CARTESIAN_POINT ( 'NONE',  ( 7.367361408496833051E-14, 14.00000000000001776, -93.40473080337741862 ) ) ;
#9832=CARTESIAN_POINT ( 'NONE',  ( -3.500000000000001332, 17.50000000000001776, -76.96098080242150274 ) ) ;
#9833=CARTESIAN_POINT ( 'NONE',  ( 0.000000000000000000, 17.50000000000002487, -149.5231586289125687 ) ) ;
#9834=CARTESIAN_POINT ( 'NONE',  ( -3.310556943750000425, 19.41135094264165772, -36.84743913623281486 ) ) ;
#9835=CARTESIAN_POINT ( 'NONE',  ( 3.310556943749999981, 15.58864905735837070, -95.43493913623279923 ) ) ;
#9837=CARTESIAN_POINT ( 'NONE',  ( -1.750000000000002220, 14.46891108675447946, -63.48806413671076143 ) ) ;
#9839=CARTESIAN_POINT ( 'NONE',  ( -3.310556943750001313, 17.50000000000002132, -118.8516058028994706 ) ) ;
#9840=CARTESIAN_POINT ( 'NONE',  ( 0.000000000000000000, 21.00000000000002487, -149.5231586289125687 ) ) ;
#9843=CARTESIAN_POINT ( 'NONE',  ( 3.500000000000001332, 17.50000000000001776, -79.46098080242150274 ) ) ;
#9844=LINE ( 'NONE', #22592, #17032 ) ;
#9845=CARTESIAN_POINT ( 'NONE',  ( -1.655278471874999990, 20.36702641396249192, -100.9307724695661364 ) ) ;
#9846=( BOUNDED_CURVE ( )  B_SPLINE_CURVE ( 2, ( #12460, #35207, #41820, #103, #18634, #9269, #35422, #6071, #31599 ),
 .UNSPECIFIED., .F., .T. ) 
 B_SPLINE_CURVE_WITH_KNOTS ( ( 3, 2, 2, 2, 3 ),
 ( 0.8937500000000000444, 0.8944444444444444864, 0.8958333333333333703, 0.8972222222222222543, 0.8979166666666666963 ),
 .UNSPECIFIED. ) 
 CURVE ( )  GEOMETRIC_REPRESENTATION_ITEM ( )  RATIONAL_B_SPLINE_CURVE ( ( 0.9330127018922194093, 0.9330127018922194093, 1.000000000000000000, 0.8660254037844387076, 1.000000000000000000, 0.8660254037844387076, 1.000000000000000000, 0.9330127018922194093, 0.9330127018922194093 ) ) 
 REPRESENTATION_ITEM ( '' )  );
#9850=VECTOR ( 'NONE', #14210, 1000.000000000000000 ) ;
#9854=CARTESIAN_POINT ( 'NONE',  ( -0.9378221735089310451, 14.00000000000002132, -105.4493890021159643 ) ) ;
#9857=CARTESIAN_POINT ( 'NONE',  ( 3.500000000000001332, 19.52072594216370760, -74.07139747004410424 ) ) ;
#9859=CARTESIAN_POINT ( 'NONE',  ( 1.655278471875001101, 20.36702641396248481, -27.09743913623280420 ) ) ;
#9860=CARTESIAN_POINT ( 'NONE',  ( -3.500000000000001332, 17.50000000000002132, -109.6547308033774328 ) ) ;
#9863=EDGE_CURVE ( 'NONE', #36251, #3661, #18583, .T. ) ;
#9866=ORIENTED_EDGE ( 'NONE', *, *, #2782, .T. ) ;
#9868=FACE_OUTER_BOUND ( 'NONE', #40142, .T. ) ;
#9871=CARTESIAN_POINT ( 'NONE',  ( 1.749999999999998224, 14.46891108675448478, -118.3213974700440900 ) ) ;
#9874=CARTESIAN_POINT ( 'NONE',  ( 3.310556943750001313, 19.41135094264167549, -133.2682724695661136 ) ) ;
#9875=CARTESIAN_POINT ( 'NONE',  ( 1.750000000000001110, 20.53108891324554719, -32.29431413575484555 ) ) ;
#9878=CARTESIAN_POINT ( 'NONE',  ( 3.500000000000001332, 17.50000000000002487, -142.4609808024215170 ) ) ;
#9880=CARTESIAN_POINT ( 'NONE',  ( 2.474675557024783212E-16, 21.54145188432740810, -139.2109808024214885 ) ) ;
#9881=CARTESIAN_POINT ( 'NONE',  ( -1.655278471874999990, 20.36702641396249547, -124.9307724695661364 ) ) ;
#9884=LINE ( 'NONE', #22212, #7569 ) ;
#9885=CARTESIAN_POINT ( 'NONE',  ( 1.749999999999998224, 14.46891108675448123, -91.62764746908817415 ) ) ;
#9886=CARTESIAN_POINT ( 'NONE',  ( 1.655278471874998436, 14.63297358603754184, -56.43077246956614346 ) ) ;
#9887=CARTESIAN_POINT ( 'NONE',  ( -1.655278471875002211, 14.63297358603755072, -109.6849391362327992 ) ) ;
#9889=CARTESIAN_POINT ( 'NONE',  ( -3.500000000000000888, 19.52072594216370405, -33.73806413671076854 ) ) ;
#9892=CARTESIAN_POINT ( 'NONE',  ( 3.310556943750001313, 19.41135094264167549, -135.2682724695661420 ) ) ;
#9894=FACE_OUTER_BOUND ( 'NONE', #9056, .T. ) ;
#9896=CARTESIAN_POINT ( 'NONE',  ( 1.655278471875001101, 20.36702641396248836, -69.18493913623279923 ) ) ;
#9898=CARTESIAN_POINT ( 'NONE',  ( -3.310556943750001313, 17.50000000000001421, -65.76410580289947916 ) ) ;
#9900=( BOUNDED_CURVE ( )  B_SPLINE_CURVE ( 2, ( #23823, #11053, #14242, #30401, #24037, #30820, #20837, #7437, #17645 ),
 .UNSPECIFIED., .F., .T. ) 
 B_SPLINE_CURVE_WITH_KNOTS ( ( 3, 2, 2, 2, 3 ),
 ( 0.3729166666666666741, 0.3736111111111111160, 0.3750000000000000000, 0.3763888888888888840, 0.3770833333333333259 ),
 .UNSPECIFIED. ) 
 CURVE ( )  GEOMETRIC_REPRESENTATION_ITEM ( )  RATIONAL_B_SPLINE_CURVE ( ( 0.9330127018922194093, 0.9330127018922194093, 1.000000000000000000, 0.8660254037844387076, 1.000000000000000000, 0.8660254037844387076, 1.000000000000000000, 0.9330127018922194093, 0.9330127018922194093 ) ) 
 REPRESENTATION_ITEM ( '' )  );
#9901=CARTESIAN_POINT ( 'NONE',  ( -3.310556943750002201, 15.58864905735837247, -86.76827246956612782 ) ) ;
#9903=EDGE_CURVE ( 'NONE', #41613, #3604, #28379, .T. ) ;
#9906=CARTESIAN_POINT ( 'NONE',  ( 3.310556943749999981, 15.58864905735836182, -51.34743913623281486 ) ) ;
#9908=CARTESIAN_POINT ( 'NONE',  ( -1.655278471874999990, 20.36702641396249547, -107.9307724695661506 ) ) ;
#9909=ORIENTED_EDGE ( 'NONE', *, *, #41666, .F. ) ;
#9910=AXIS2_PLACEMENT_3D ( 'NONE', #27414, #17211, #17630 ) ;
#9915=CARTESIAN_POINT ( 'NONE',  ( -1.655278471875002211, 14.63297358603754361, -60.59743913623280775 ) ) ;
#9916=ORIENTED_EDGE ( 'NONE', *, *, #31639, .T. ) ;
#9917=EDGE_LOOP ( 'NONE', ( #12552, #25957, #7322, #10802 ) ) ;
#9919=CARTESIAN_POINT ( 'NONE',  ( -3.500000000000001332, 17.50000000000001066, -40.65473080337743284 ) ) ;
#9922=AXIS2_PLACEMENT_3D ( 'NONE', #27097, #11148, #17732 ) ;
#9925=CARTESIAN_POINT ( 'NONE',  ( 7.785697387528201340E-15, 14.00000000000002487, -138.7109808024215170 ) ) ;
#9926=CARTESIAN_POINT ( 'NONE',  ( -3.310556943750001313, 17.50000000000002132, -122.7641058028994649 ) ) ;
#9927=CARTESIAN_POINT ( 'NONE',  ( -1.750000000000002220, 14.46891108675448656, -117.4880641367107614 ) ) ;
#9929=CARTESIAN_POINT ( 'NONE',  ( 1.655278471875001101, 20.36702641396248481, -35.18493913623279923 ) ) ;
#9930=CARTESIAN_POINT ( 'NONE',  ( 2.340729813953370519E-16, 21.32270188528330479, -24.10160580289947063 ) ) ;
#9931=CARTESIAN_POINT ( 'NONE',  ( -3.310556943750000425, 19.41135094264166483, -86.93493913623278502 ) ) ;
#9932=CARTESIAN_POINT ( 'NONE',  ( -3.310556943750002645, 15.58864905735837958, -136.6807724695661364 ) ) ;
#9936=CARTESIAN_POINT ( 'NONE',  ( -7.022189441860112050E-16, 13.67729811471672718, -135.6016058028994564 ) ) ;
#9938=CARTESIAN_POINT ( 'NONE',  ( 3.500000000000001332, 19.52072594216370760, -56.37764746908817415 ) ) ;
#9939=CARTESIAN_POINT ( 'NONE',  ( -3.310556943750001313, 17.50000000000001776, -92.76410580289947916 ) ) ;
#9941=CARTESIAN_POINT ( 'NONE',  ( 4.286263797015737581E-16, 14.00000000000002487, -149.5231586289125687 ) ) ;
#9942=CARTESIAN_POINT ( 'NONE',  ( 1.750000000000001110, 20.53108891324555785, -111.2943141357548456 ) ) ;
#9943=CARTESIAN_POINT ( 'NONE',  ( -1.749999999999999778, 20.53108891324555429, -74.82139747004410424 ) ) ;
#9944=CARTESIAN_POINT ( 'NONE',  ( 3.310556943749999981, 15.58864905735836537, -58.43493913623279212 ) ) ;
#9948=CARTESIAN_POINT ( 'NONE',  ( 3.310556943750001313, 17.50000000000001776, -85.35160580289947063 ) ) ;
#9950=CARTESIAN_POINT ( 'NONE',  ( 3.310556943749999981, 15.58864905735837247, -112.3474391362328078 ) ) ;
#9951=CARTESIAN_POINT ( 'NONE',  ( 1.655278471874998436, 14.63297358603754539, -81.43077246956615056 ) ) ;
#9954=CARTESIAN_POINT ( 'NONE',  ( 3.310556943749999981, 15.58864905735837070, -104.4349391362328134 ) ) ;
#9955=CARTESIAN_POINT ( 'NONE',  ( -3.500000000000001332, 17.50000000000002132, -104.6547308033774186 ) ) ;
#9958=CARTESIAN_POINT ( 'NONE',  ( -0.9378221735089291577, 21.00000000000001776, -95.86007260463891555 ) ) ;
#9959=CARTESIAN_POINT ( 'NONE',  ( -1.394453263437886604E-15, 14.00000000000001421, -54.40473080337742573 ) ) ;
#9961=CARTESIAN_POINT ( 'NONE',  ( -3.310556943750000425, 19.41135094264166483, -67.84743913623280775 ) ) ;
#9962=CARTESIAN_POINT ( 'NONE',  ( 4.648177544792955347E-16, 21.00000000000001066, -30.21098080242151340 ) ) ;
#9963=CARTESIAN_POINT ( 'NONE',  ( 3.310556943750001313, 19.41135094264166838, -123.1807724695661364 ) ) ;
#9964=LINE ( 'NONE', #35056, #27747 ) ;
#9965=EDGE_LOOP ( 'NONE', ( #25170, #40174, #33392, #4625 ) ) ;
#9966=CARTESIAN_POINT ( 'NONE',  ( 4.648177544792955347E-16, 21.00000000000002487, -132.9047308033774186 ) ) ;
#9967=CARTESIAN_POINT ( 'NONE',  ( 0.9378221735089300459, 21.00000000000002132, -127.9493890021159359 ) ) ;
#9968=CARTESIAN_POINT ( 'NONE',  ( 3.310556943750001313, 17.50000000000001421, -72.26410580289947916 ) ) ;
#9972=CARTESIAN_POINT ( 'NONE',  ( -3.310556943750001313, 17.50000000000002487, -140.7641058028994792 ) ) ;
#9974=CARTESIAN_POINT ( 'NONE',  ( 1.655278471875001101, 20.36702641396248481, -46.18493913623279923 ) ) ;
#9975=CARTESIAN_POINT ( 'NONE',  ( 3.310556943749999981, 15.58864905735837070, -101.4349391362328134 ) ) ;
#9977=CARTESIAN_POINT ( 'NONE',  ( 2.340729813953370519E-16, 21.32270188528330479, -27.01410580289947916 ) ) ;
#9978=CARTESIAN_POINT ( 'NONE',  ( 3.500000000000001332, 17.50000000000001066, -23.15473080337743284 ) ) ;
#9979=CARTESIAN_POINT ( 'NONE',  ( 2.474675557024783212E-16, 21.54145188432740099, -102.2109808024214885 ) ) ;
#9982=CARTESIAN_POINT ( 'NONE',  ( -3.500000000000002220, 15.47927405783632793, -90.57139747004409003 ) ) ;
#9983=CARTESIAN_POINT ( 'NONE',  ( 4.648177544792955347E-16, 21.00000000000001776, -96.21098080242150274 ) ) ;
#9986=CARTESIAN_POINT ( 'NONE',  ( -3.500000000000000888, 19.52072594216370760, -55.04431413575484555 ) ) ;
#9988=CARTESIAN_POINT ( 'NONE',  ( -1.655278471874999990, 20.36702641396248481, -23.93077246956613990 ) ) ;
#9989=CARTESIAN_POINT ( 'NONE',  ( 1.749999999999998224, 14.46891108675447590, -41.32139747004409713 ) ) ;
#9991=CARTESIAN_POINT ( 'NONE',  ( 3.310556943749999981, 15.58864905735836182, -26.43493913623279212 ) ) ;
#9998=CARTESIAN_POINT ( 'NONE',  ( 3.310556943749999981, 15.58864905735836892, -82.34743913623279354 ) ) ;
#9999=CARTESIAN_POINT ( 'NONE',  ( -1.749999999999999778, 20.53108891324556140, -141.8213974700441042 ) ) ;
#10000=ORIENTED_EDGE ( 'NONE', *, *, #23566, .T. ) ;
#10002=CARTESIAN_POINT ( 'NONE',  ( 4.648177544792955347E-16, 21.00000000000001776, -87.21098080242151696 ) ) ;
#10005=CARTESIAN_POINT ( 'NONE',  ( 1.655278471875001101, 20.36702641396249192, -91.09743913623280775 ) ) ;
#10008=EDGE_LOOP ( 'NONE', ( #34265, #31298, #27239, #38884 ) ) ;
#10016=CARTESIAN_POINT ( 'NONE',  ( -3.310556943750000425, 19.41135094264167549, -131.8474391362327935 ) ) ;
#10017=ORIENTED_EDGE ( 'NONE', *, *, #3474, .F. ) ;
#10018=ORIENTED_EDGE ( 'NONE', *, *, #41246, .F. ) ;
#10019=CARTESIAN_POINT ( 'NONE',  ( -0.9378221735089291577, 21.00000000000001776, -95.16632260368297125 ) ) ;
#10020=CARTESIAN_POINT ( 'NONE',  ( -3.310556943750001313, 17.50000000000002132, -120.8516058028994706 ) ) ;
#10024=CARTESIAN_POINT ( 'NONE',  ( -3.500000000000002220, 15.47927405783633503, -131.5713974700441042 ) ) ;
#10025=ADVANCED_FACE ( 'NONE', ( #15386 ), #5800, .T. ) ;
#10026=CARTESIAN_POINT ( 'NONE',  ( -3.310556943750002645, 15.58864905735837070, -70.76827246956612782 ) ) ;
#10027=CARTESIAN_POINT ( 'NONE',  ( 1.750000000000001110, 20.53108891324555785, -117.2943141357548313 ) ) ;
#10028=CARTESIAN_POINT ( 'NONE',  ( -3.310556943750001313, 17.50000000000002132, -102.7641058028994649 ) ) ;
#10032=CARTESIAN_POINT ( 'NONE',  ( -3.500000000000000888, 19.52072594216370760, -73.04431413575484555 ) ) ;
#10034=CARTESIAN_POINT ( 'NONE',  ( 1.655278471874998436, 14.63297358603753828, -36.43077246956613635 ) ) ;
#10035=CARTESIAN_POINT ( 'NONE',  ( 1.655278471875001101, 20.36702641396249192, -97.18493913623279923 ) ) ;
#10036=CARTESIAN_POINT ( 'NONE',  ( -3.500000000000001332, 17.50000000000001421, -65.65473080337743284 ) ) ;
#10037=CARTESIAN_POINT ( 'NONE',  ( -3.310556943750000425, 19.41135094264166838, -115.9349391362327850 ) ) ;
#10043=CARTESIAN_POINT ( 'NONE',  ( 3.310556943750001313, 19.41135094264166838, -96.18077246956613635 ) ) ;
#10049=CARTESIAN_POINT ( 'NONE',  ( -1.749999999999999778, 20.53108891324555074, -71.12764746908817415 ) ) ;
#10054=CARTESIAN_POINT ( 'NONE',  ( 3.310556943750001313, 17.50000000000001066, -27.26410580289947916 ) ) ;
#10055=ADVANCED_FACE ( 'NONE', ( #12386 ), #31945, .T. ) ;
#10057=ORIENTED_EDGE ( 'NONE', *, *, #30999, .F. ) ;
#10058=CARTESIAN_POINT ( 'NONE',  ( -0.9378221735089310451, 14.00000000000002309, -123.4493890021159501 ) ) ;
#10062=VERTEX_POINT ( 'NONE', #12598 ) ;
#10064=CARTESIAN_POINT ( 'NONE',  ( -1.394453263437886604E-15, 14.00000000000001776, -85.71098080242151696 ) ) ;
#10065=CARTESIAN_POINT ( 'NONE',  ( 3.500000000000001332, 17.50000000000002132, -120.1547308033774328 ) ) ;
#10067=CARTESIAN_POINT ( 'NONE',  ( 1.655278471874998436, 14.63297358603755072, -133.5182724695661420 ) ) ;
#10068=CARTESIAN_POINT ( 'NONE',  ( -1.749999999999999778, 20.53108891324554719, -27.12764746908817415 ) ) ;
#10070=CARTESIAN_POINT ( 'NONE',  ( -1.394453263437886604E-15, 14.00000000000001066, -37.40473080337743284 ) ) ;
#10072=CARTESIAN_POINT ( 'NONE',  ( 3.500000000000001776, 19.52072594216372181, -139.3776474690881741 ) ) ;
#10073=CARTESIAN_POINT ( 'NONE',  ( 2.340729813953370519E-16, 21.32270188528331900, -119.0141058028994792 ) ) ;
#10076=( BOUNDED_CURVE ( )  B_SPLINE_CURVE ( 2, ( #3036, #35574, #32381, #32784, #9636, #10252, #38973, #3652, #12817 ),
 .UNSPECIFIED., .F., .F. ) 
 B_SPLINE_CURVE_WITH_KNOTS ( ( 3, 2, 2, 2, 3 ),
 ( 0.2020833333333333370, 0.2027777777777777790, 0.2041666666666666630, 0.2055555555555555469, 0.2062499999999999889 ),
 .UNSPECIFIED. ) 
 CURVE ( )  GEOMETRIC_REPRESENTATION_ITEM ( )  RATIONAL_B_SPLINE_CURVE ( ( 0.9330127018922194093, 0.9330127018922194093, 1.000000000000000000, 0.8660254037844387076, 1.000000000000000000, 0.8660254037844387076, 1.000000000000000000, 0.9330127018922194093, 0.9330127018922194093 ) ) 
 REPRESENTATION_ITEM ( '' )  );
#10078=CARTESIAN_POINT ( 'NONE',  ( 3.500000000000000000, 15.47927405783632615, -89.54431413575483134 ) ) ;
#10081=CARTESIAN_POINT ( 'NONE',  ( 4.648177544792955347E-16, 21.00000000000001066, -45.90473080337741862 ) ) ;
#10082=CARTESIAN_POINT ( 'NONE',  ( 3.310556943750001313, 19.41135094264166128, -52.18077246956612925 ) ) ;
#10083=CARTESIAN_POINT ( 'NONE',  ( -3.310556943750002645, 15.58864905735837780, -112.7682724695661278 ) ) ;
#10085=CARTESIAN_POINT ( 'NONE',  ( 3.500000000000000000, 15.47927405783632082, -31.23806413671076498 ) ) ;
#10089=CARTESIAN_POINT ( 'NONE',  ( 3.310556943750001313, 19.41135094264167549, -133.2682724695661420 ) ) ;
#10091=DIRECTION ( 'NONE',  ( -0.000000000000000000, 1.259100132267607459E-16, -1.000000000000000000 ) ) ;
#10093=CARTESIAN_POINT ( 'NONE',  ( -3.310556943750002645, 15.58864905735836892, -61.76827246956613493 ) ) ;
#10095=CARTESIAN_POINT ( 'NONE',  ( -3.310556943750001313, 17.50000000000001421, -63.76410580289947205 ) ) ;
#10097=CARTESIAN_POINT ( 'NONE',  ( -1.655278471875002211, 14.63297358603754716, -84.68493913623278502 ) ) ;
#10099=CARTESIAN_POINT ( 'NONE',  ( 4.648177544792955347E-16, 21.00000000000001066, -40.21098080242150274 ) ) ;
#10100=EDGE_CURVE ( 'NONE', #13615, #5149, #3231, .T. ) ;
#10102=CARTESIAN_POINT ( 'NONE',  ( -7.022189441860112050E-16, 13.67729811471671830, -42.51410580289947916 ) ) ;
#10104=CARTESIAN_POINT ( 'NONE',  ( -3.310556943750002645, 15.58864905735837425, -107.6807724695661506 ) ) ;
#10106=ORIENTED_EDGE ( 'NONE', *, *, #35208, .F. ) ;
#10111=CARTESIAN_POINT ( 'NONE',  ( 2.340729813953370519E-16, 21.32270188528330834, -58.01410580289949337 ) ) ;
#10112=ORIENTED_EDGE ( 'NONE', *, *, #41556, .F. ) ;
#10114=CYLINDRICAL_SURFACE ( 'NONE', #28704, 3.499999999999999556 ) ;
#10118=CARTESIAN_POINT ( 'NONE',  ( 4.648177544792955347E-16, 21.00000000000002487, -140.9047308033773902 ) ) ;
#10119=ORIENTED_EDGE ( 'NONE', *, *, #4892, .T. ) ;
#10121=CARTESIAN_POINT ( 'NONE',  ( -3.310556943750000425, 19.41135094264166838, -123.8474391362328078 ) ) ;
#10122=CARTESIAN_POINT ( 'NONE',  ( 4.648177544792955347E-16, 21.00000000000002132, -117.9047308033774328 ) ) ;
#10124=CARTESIAN_POINT ( 'NONE',  ( 3.310556943750001313, 19.41135094264165772, -37.26827246956612072 ) ) ;
#10126=CARTESIAN_POINT ( 'NONE',  ( 3.310556943749999981, 15.58864905735836892, -86.43493913623279923 ) ) ;
#10127=CARTESIAN_POINT ( 'NONE',  ( -3.310556943750002645, 15.58864905735837958, -140.6807724695661364 ) ) ;
#10129=CARTESIAN_POINT ( 'NONE',  ( 1.749999999999998224, 14.46891108675447590, -49.32139747004410424 ) ) ;
#10130=CARTESIAN_POINT ( 'NONE',  ( -1.394453263437886604E-15, 14.00000000000001421, -78.40473080337741862 ) ) ;
#10131=( BOUNDED_CURVE ( )  B_SPLINE_CURVE ( 2, ( #31441, #2312, #14869, #1119, #15296, #27836, #40601, #31652, #12297 ),
 .UNSPECIFIED., .F., .F. ) 
 B_SPLINE_CURVE_WITH_KNOTS ( ( 3, 2, 2, 2, 3 ),
 ( 0.08541666666666666852, 0.08611111111111111049, 0.08749999999999999445, 0.08888888888888889228, 0.08958333333333333426 ),
 .UNSPECIFIED. ) 
 CURVE ( )  GEOMETRIC_REPRESENTATION_ITEM ( )  RATIONAL_B_SPLINE_CURVE ( ( 0.9330127018922194093, 0.9330127018922194093, 1.000000000000000000, 0.8660254037844387076, 1.000000000000000000, 0.8660254037844387076, 1.000000000000000000, 0.9330127018922194093, 0.9330127018922194093 ) ) 
 REPRESENTATION_ITEM ( '' )  );
#10132=CARTESIAN_POINT ( 'NONE',  ( 1.655278471874998436, 14.63297358603755072, -125.5182724695661278 ) ) ;
#10134=CARTESIAN_POINT ( 'NONE',  ( 1.655278471874998436, 14.63297358603754539, -90.43077246956613635 ) ) ;
#10136=CARTESIAN_POINT ( 'NONE',  ( 0.000000000000000000, 17.50000000000002487, -149.5231586289125687 ) ) ;
#10137=CARTESIAN_POINT ( 'NONE',  ( -1.749999999999999778, 20.53108891324555429, -75.82139747004410424 ) ) ;
#10138=CARTESIAN_POINT ( 'NONE',  ( -3.310556943750001313, 17.50000000000001421, -61.85160580289945642 ) ) ;
#10140=CARTESIAN_POINT ( 'NONE',  ( 0.000000000000000000, 17.50000000000002487, -149.5231586289125687 ) ) ;
#10142=CARTESIAN_POINT ( 'NONE',  ( 3.310556943750001313, 19.41135094264166483, -81.26827246956612782 ) ) ;
#10143=DIRECTION ( 'NONE',  ( -0.000000000000000000, 1.259100132267607459E-16, -1.000000000000000000 ) ) ;
#10146=CARTESIAN_POINT ( 'NONE',  ( 3.310556943749999981, 15.58864905735837247, -109.3474391362328078 ) ) ;
#10147=CARTESIAN_POINT ( 'NONE',  ( -7.022189441860112050E-16, 13.67729811471672186, -78.51410580289946495 ) ) ;
#10148=ORIENTED_EDGE ( 'NONE', *, *, #18485, .T. ) ;
#10149=CARTESIAN_POINT ( 'NONE',  ( 1.655278471875001101, 20.36702641396249547, -103.1849391362327992 ) ) ;
#10150=CARTESIAN_POINT ( 'NONE',  ( 1.750000000000001110, 20.53108891324555429, -100.9880641367107756 ) ) ;
#10152=CARTESIAN_POINT ( 'NONE',  ( 0.000000000000000000, 21.00000000000002487, -149.5231586289125687 ) ) ;
#10153=DIRECTION ( 'NONE',  ( -0.000000000000000000, 1.259100132267607459E-16, -1.000000000000000000 ) ) ;
#10155=EDGE_CURVE ( 'NONE', #23778, #17584, #35954, .T. ) ;
#10157=CARTESIAN_POINT ( 'NONE',  ( 2.340729813953370519E-16, 21.32270188528331190, -61.01410580289945784 ) ) ;
#10159=CARTESIAN_POINT ( 'NONE',  ( -1.655278471874999990, 20.36702641396249547, -123.9307724695661364 ) ) ;
#10161=VECTOR ( 'NONE', #20171, 1000.000000000000000 ) ;
#10164=CARTESIAN_POINT ( 'NONE',  ( 4.648177544792955347E-16, 21.00000000000001066, -31.90473080337742573 ) ) ;
#10166=CARTESIAN_POINT ( 'NONE',  ( 3.310556943749999981, 15.58864905735836714, -71.34743913623279354 ) ) ;
#10167=ORIENTED_EDGE ( 'NONE', *, *, #6401, .T. ) ;
#10168=ORIENTED_EDGE ( 'NONE', *, *, #33385, .T. ) ;
#10171=CARTESIAN_POINT ( 'NONE',  ( 1.655278471874998436, 14.63297358603755249, -140.4307724695661364 ) ) ;
#10176=CARTESIAN_POINT ( 'NONE',  ( -3.500000000000000000, 19.52072594216371826, -111.0443141357548456 ) ) ;
#10177=CARTESIAN_POINT ( 'NONE',  ( -1.655278471874999990, 20.36702641396248481, -36.01827246956612782 ) ) ;
#10178=CARTESIAN_POINT ( 'NONE',  ( -1.655278471875002211, 14.63297358603754894, -104.6849391362327992 ) ) ;
#10180=CARTESIAN_POINT ( 'NONE',  ( 3.310556943750001313, 17.50000000000002487, -142.3516058028994564 ) ) ;
#10182=CARTESIAN_POINT ( 'NONE',  ( -3.500000000000001332, 17.50000000000002132, -102.9609808024215027 ) ) ;
#10184=DIRECTION ( 'NONE',  ( -0.000000000000000000, 1.259100132267607459E-16, -1.000000000000000000 ) ) ;
#10185=CARTESIAN_POINT ( 'NONE',  ( 3.500000000000001332, 17.50000000000001776, -93.15473080337743284 ) ) ;
#10188=CARTESIAN_POINT ( 'NONE',  ( -1.749999999999999778, 20.53108891324555074, -54.12764746908817415 ) ) ;
#10190=CARTESIAN_POINT ( 'NONE',  ( 0.000000000000000000, 17.50000000000002487, -149.5231586289125687 ) ) ;
#10191=CARTESIAN_POINT ( 'NONE',  ( 1.750000000000001110, 20.53108891324554719, -44.98806413671076143 ) ) ;
#10194=CARTESIAN_POINT ( 'NONE',  ( -3.310556943750001313, 17.50000000000001066, -28.85160580289947063 ) ) ;
#10196=CARTESIAN_POINT ( 'NONE',  ( -3.500000000000000000, 19.52072594216370405, -39.73806413671076854 ) ) ;
#10197=FACE_OUTER_BOUND ( 'NONE', #32276, .T. ) ;
#10200=CARTESIAN_POINT ( 'NONE',  ( 1.750000000000001110, 20.53108891324555785, -119.9880641367107614 ) ) ;
#10202=CARTESIAN_POINT ( 'NONE',  ( 1.655278471874998436, 14.63297358603754361, -80.43077246956615056 ) ) ;
#10205=ORIENTED_EDGE ( 'NONE', *, *, #29322, .F. ) ;
#10207=CARTESIAN_POINT ( 'NONE',  ( 3.500000000000001332, 17.50000000000001066, -27.15473080337743639 ) ) ;
#10210=CARTESIAN_POINT ( 'NONE',  ( 1.655278471875001101, 20.36702641396249192, -92.09743913623280775 ) ) ;
#10215=CYLINDRICAL_SURFACE ( 'NONE', #17409, 3.499999999999999556 ) ;
#10216=CARTESIAN_POINT ( 'NONE',  ( 2.340729813953370519E-16, 21.32270188528331900, -126.0141058028994792 ) ) ;
#10217=ORIENTED_EDGE ( 'NONE', *, *, #20753, .T. ) ;
#10218=CARTESIAN_POINT ( 'NONE',  ( 0.9378221735089300459, 21.00000000000001421, -63.94938900211595723 ) ) ;
#10219=CARTESIAN_POINT ( 'NONE',  ( 3.310556943750001313, 19.41135094264166128, -52.26827246956612782 ) ) ;
#10220=CARTESIAN_POINT ( 'NONE',  ( 1.655278471875001101, 20.36702641396249547, -121.1849391362327992 ) ) ;
#10223=CARTESIAN_POINT ( 'NONE',  ( 1.750000000000001110, 20.53108891324555785, -126.9880641367107614 ) ) ;
#10224=AXIS2_PLACEMENT_3D ( 'NONE', #21548, #9201, #27717 ) ;
#10225=CARTESIAN_POINT ( 'NONE',  ( 1.655278471875001101, 20.36702641396248836, -70.18493913623279923 ) ) ;
#10226=CARTESIAN_POINT ( 'NONE',  ( -3.500000000000000888, 19.52072594216371826, -116.0443141357548456 ) ) ;
#10227=CARTESIAN_POINT ( 'NONE',  ( -3.310556943750000425, 19.41135094264166483, -99.84743913623282197 ) ) ;
#10229=LINE ( 'NONE', #30216, #1690 ) ;
#10232=CARTESIAN_POINT ( 'NONE',  ( -7.424026671074350129E-16, 13.45854811567263454, -68.71098080242150274 ) ) ;
#10233=CARTESIAN_POINT ( 'NONE',  ( -3.500000000000001332, 17.50000000000001066, -43.96098080242151696 ) ) ;
#10234=CARTESIAN_POINT ( 'NONE',  ( 1.655278471875001101, 20.36702641396248481, -36.09743913623281486 ) ) ;
#10236=CARTESIAN_POINT ( 'NONE',  ( 3.310556943749999981, 15.58864905735837070, -97.43493913623279923 ) ) ;
#10237=CARTESIAN_POINT ( 'NONE',  ( 1.749999999999998224, 14.46891108675447768, -57.32139747004409713 ) ) ;
#10239=CARTESIAN_POINT ( 'NONE',  ( 1.655278471874998436, 14.63297358603754894, -118.5182724695661278 ) ) ;
#10244=CARTESIAN_POINT ( 'NONE',  ( 4.648177544792955347E-16, 21.00000000000001776, -79.21098080242148853 ) ) ;
#10246=CARTESIAN_POINT ( 'NONE',  ( -1.655278471874999990, 20.36702641396249192, -99.93077246956613635 ) ) ;
#10247=CARTESIAN_POINT ( 'NONE',  ( 0.9378221735089281585, 14.00000000000000888, -39.36007260463890134 ) ) ;
#10250=( BOUNDED_CURVE ( )  B_SPLINE_CURVE ( 2, ( #2437, #38579, #32201, #2853, #15843, #9664, #28787, #9444, #6253 ),
 .UNSPECIFIED., .F., .T. ) 
 B_SPLINE_CURVE_WITH_KNOTS ( ( 3, 2, 2, 2, 3 ),
 ( 0.1895833333333333259, 0.1902777777777777679, 0.1916666666666666796, 0.1930555555555555636, 0.1937500000000000056 ),
 .UNSPECIFIED. ) 
 CURVE ( )  GEOMETRIC_REPRESENTATION_ITEM ( )  RATIONAL_B_SPLINE_CURVE ( ( 0.9330127018922194093, 0.9330127018922194093, 1.000000000000000000, 0.8660254037844387076, 1.000000000000000000, 0.8660254037844387076, 1.000000000000000000, 0.9330127018922194093, 0.9330127018922194093 ) ) 
 REPRESENTATION_ITEM ( '' )  );
#10251=CARTESIAN_POINT ( 'NONE',  ( 4.648177544792955347E-16, 21.00000000000002487, -136.2109808024215170 ) ) ;
#10252=CARTESIAN_POINT ( 'NONE',  ( -3.500000000000002220, 15.47927405783633503, -118.5713974700441184 ) ) ;
#10253=( BOUNDED_CURVE ( )  B_SPLINE_CURVE ( 2, ( #17428, #11244, #1870, #33587, #26785, #24431, #34000, #14226, #36993 ),
 .UNSPECIFIED., .F., .F. ) 
 B_SPLINE_CURVE_WITH_KNOTS ( ( 3, 2, 2, 2, 3 ),
 ( 0.1937500000000000056, 0.1944444444444444475, 0.1958333333333333315, 0.1972222222222222154, 0.1979166666666666574 ),
 .UNSPECIFIED. ) 
 CURVE ( )  GEOMETRIC_REPRESENTATION_ITEM ( )  RATIONAL_B_SPLINE_CURVE ( ( 0.9330127018922194093, 0.9330127018922194093, 1.000000000000000000, 0.8660254037844387076, 1.000000000000000000, 0.8660254037844387076, 1.000000000000000000, 0.9330127018922194093, 0.9330127018922194093 ) ) 
 REPRESENTATION_ITEM ( '' )  );
#10254=CARTESIAN_POINT ( 'NONE',  ( -0.9378221735089291577, 21.00000000000002132, -112.8600726046389013 ) ) ;
#10255=VERTEX_POINT ( 'NONE', #26618 ) ;
#10256=CARTESIAN_POINT ( 'NONE',  ( 1.743066579297357930E-14, 14.00000000000002132, -134.7109808024214885 ) ) ;
#10259=CARTESIAN_POINT ( 'NONE',  ( 3.310556943750001313, 19.41135094264166128, -29.18077246956613990 ) ) ;
#10267=ORIENTED_EDGE ( 'NONE', *, *, #16510, .T. ) ;
#10269=CARTESIAN_POINT ( 'NONE',  ( 4.286263797015737581E-16, 14.00000000000002487, -149.5231586289125687 ) ) ;
#10270=CARTESIAN_POINT ( 'NONE',  ( -3.500000000000001332, 17.50000000000001776, -80.96098080242150274 ) ) ;
#10271=CARTESIAN_POINT ( 'NONE',  ( -1.394453263437886604E-15, 14.00000000000001421, -64.71098080242150274 ) ) ;
#10272=CARTESIAN_POINT ( 'NONE',  ( 1.655278471874998436, 14.63297358603755249, -137.5182724695661420 ) ) ;
#10273=CARTESIAN_POINT ( 'NONE',  ( 2.474675557024783212E-16, 21.54145188432739033, -26.21098080242151340 ) ) ;
#10276=CARTESIAN_POINT ( 'NONE',  ( -1.394453263437886604E-15, 14.00000000000001066, -43.40473080337742573 ) ) ;
#10278=CARTESIAN_POINT ( 'NONE',  ( 3.500000000000000000, 15.47927405783633503, -132.5443141357548598 ) ) ;
#10279=CARTESIAN_POINT ( 'NONE',  ( -3.310556943750001313, 17.50000000000002132, -119.7641058028994792 ) ) ;
#10284=CARTESIAN_POINT ( 'NONE',  ( 3.500000000000000000, 15.47927405783632615, -85.54431413575483134 ) ) ;
#10285=CARTESIAN_POINT ( 'NONE',  ( -3.500000000000001332, 17.50000000000001066, -40.96098080242150985 ) ) ;
#10286=CARTESIAN_POINT ( 'NONE',  ( 3.310556943750001313, 17.50000000000001421, -53.26410580289947205 ) ) ;
#10288=CARTESIAN_POINT ( 'NONE',  ( 1.655278471875001101, 20.36702641396249547, -112.1849391362327992 ) ) ;
#10289=CARTESIAN_POINT ( 'NONE',  ( -1.394453263437886604E-15, 14.00000000000001421, -58.40473080337741862 ) ) ;
#10290=CARTESIAN_POINT ( 'NONE',  ( 1.749999999999998224, 14.46891108675447413, -27.32139747004409713 ) ) ;
#10291=CARTESIAN_POINT ( 'NONE',  ( 3.500000000000001332, 17.50000000000002132, -116.4609808024215170 ) ) ;
#10293=CARTESIAN_POINT ( 'NONE',  ( 1.655278471874998436, 14.63297358603755072, -131.5182724695661136 ) ) ;
#10297=CARTESIAN_POINT ( 'NONE',  ( -1.655278471875002211, 14.63297358603754361, -65.68493913623279923 ) ) ;
#10299=CARTESIAN_POINT ( 'NONE',  ( 3.310556943749999981, 15.58864905735836537, -66.34743913623280775 ) ) ;
#10302=CARTESIAN_POINT ( 'NONE',  ( 1.655278471875001101, 20.36702641396249192, -85.18493913623278502 ) ) ;
#10306=CARTESIAN_POINT ( 'NONE',  ( 3.310556943749999981, 15.58864905735836182, -47.34743913623280775 ) ) ;
#10308=CARTESIAN_POINT ( 'NONE',  ( -1.655278471874999990, 20.36702641396249192, -101.9307724695661364 ) ) ;
#10310=ORIENTED_EDGE ( 'NONE', *, *, #27015, .T. ) ;
#10313=ORIENTED_EDGE ( 'NONE', *, *, #5423, .F. ) ;
#10315=CARTESIAN_POINT ( 'NONE',  ( 3.310556943749999981, 15.58864905735836182, -50.34743913623281486 ) ) ;
#10316=VERTEX_POINT ( 'NONE', #13635 ) ;
#10318=DIRECTION ( 'NONE',  ( -0.000000000000000000, 1.259100132267607459E-16, -1.000000000000000000 ) ) ;
#10320=CARTESIAN_POINT ( 'NONE',  ( 0.9378221735089300459, 21.00000000000001066, -31.25563900116002358 ) ) ;
#10323=CARTESIAN_POINT ( 'NONE',  ( 0.9378221735089300459, 21.00000000000001421, -46.94938900211595012 ) ) ;
#10324=ADVANCED_FACE ( 'NONE', ( #14491 ), #40629, .T. ) ;
#10325=VERTEX_POINT ( 'NONE', #7900 ) ;
#10327=CARTESIAN_POINT ( 'NONE',  ( 3.500000000000001332, 17.50000000000001066, -46.46098080242150274 ) ) ;
#10328=CARTESIAN_POINT ( 'NONE',  ( -1.655278471874999990, 20.36702641396248481, -42.93077246956614346 ) ) ;
#10329=( BOUNDED_CURVE ( )  B_SPLINE_CURVE ( 2, ( #1885, #34843, #21453, #2309, #14867, #27834, #15077, #11258, #31439 ),
 .UNSPECIFIED., .F., .T. ) 
 B_SPLINE_CURVE_WITH_KNOTS ( ( 3, 2, 2, 2, 3 ),
 ( 0.5895833333333333481, 0.5902777777777777901, 0.5916666666666666741, 0.5930555555555555580, 0.5937500000000000000 ),
 .UNSPECIFIED. ) 
 CURVE ( )  GEOMETRIC_REPRESENTATION_ITEM ( )  RATIONAL_B_SPLINE_CURVE ( ( 0.9330127018922194093, 0.9330127018922194093, 1.000000000000000000, 0.8660254037844387076, 1.000000000000000000, 0.8660254037844387076, 1.000000000000000000, 0.9330127018922194093, 0.9330127018922194093 ) ) 
 REPRESENTATION_ITEM ( '' )  );
#10330=LINE ( 'NONE', #23302, #20123 ) ;
#10331=CARTESIAN_POINT ( 'NONE',  ( 3.500000000000001332, 17.50000000000001776, -97.15473080337743284 ) ) ;
#10334=CARTESIAN_POINT ( 'NONE',  ( -7.022189441860112050E-16, 13.67729811471671475, -29.60160580289947418 ) ) ;
#10336=CARTESIAN_POINT ( 'NONE',  ( 3.310556943750001313, 19.41135094264166483, -80.26827246956614204 ) ) ;
#10337=CARTESIAN_POINT ( 'NONE',  ( 3.310556943750001313, 17.50000000000002487, -135.2641058028994507 ) ) ;
#10340=CARTESIAN_POINT ( 'NONE',  ( 4.648177544792955347E-16, 21.00000000000001421, -67.21098080242148853 ) ) ;
#10341=EDGE_CURVE ( 'NONE', #23778, #42029, #8096, .T. ) ;
#10342=CARTESIAN_POINT ( 'NONE',  ( -7.022189441860112050E-16, 13.67729811471672718, -127.6016058028994706 ) ) ;
#10344=CARTESIAN_POINT ( 'NONE',  ( 3.310556943749999981, 15.58864905735836892, -85.34743913623279354 ) ) ;
#10345=LINE ( 'NONE', #10560, #10415 ) ;
#10346=DIRECTION ( 'NONE',  ( -0.000000000000000000, 1.259100132267607459E-16, -1.000000000000000000 ) ) ;
#10347=CARTESIAN_POINT ( 'NONE',  ( 4.648177544792955347E-16, 21.00000000000001421, -52.90473080337743284 ) ) ;
#10348=CARTESIAN_POINT ( 'NONE',  ( -1.749999999999999778, 20.53108891324555074, -73.82139747004410424 ) ) ;
#10350=CARTESIAN_POINT ( 'NONE',  ( 1.655278471875001101, 20.36702641396248836, -58.18493913623279212 ) ) ;
#10354=CARTESIAN_POINT ( 'NONE',  ( -3.310556943750002645, 15.58864905735837070, -79.76827246956612782 ) ) ;
#10357=CARTESIAN_POINT ( 'NONE',  ( 1.655278471874998436, 14.63297358603754894, -110.4307724695661506 ) ) ;
#10358=CARTESIAN_POINT ( 'NONE',  ( -3.310556943750001313, 17.50000000000001776, -79.76410580289946495 ) ) ;
#10359=CARTESIAN_POINT ( 'NONE',  ( -1.394453263437886604E-15, 14.00000000000001776, -96.40473080337741862 ) ) ;
#10361=CARTESIAN_POINT ( 'NONE',  ( 1.655278471874998436, 14.63297358603754716, -101.5182724695661278 ) ) ;
#10362=CARTESIAN_POINT ( 'NONE',  ( 3.500000000000001776, 19.52072594216371115, -101.0713974700440900 ) ) ;
#10364=LINE ( 'NONE', #10152, #38099 ) ;
#10365=CARTESIAN_POINT ( 'NONE',  ( -1.394453263437886604E-15, 14.00000000000001776, -105.4047308033774186 ) ) ;
#10368=CARTESIAN_POINT ( 'NONE',  ( 2.340729813953370519E-16, 21.32270188528331190, -60.01410580289947916 ) ) ;
#10370=CARTESIAN_POINT ( 'NONE',  ( 3.310556943750001313, 19.41135094264166838, -118.1807724695661364 ) ) ;
#10371=CARTESIAN_POINT ( 'NONE',  ( -1.394453263437886604E-15, 14.00000000000001066, -36.71098080242150985 ) ) ;
#10373=ORIENTED_EDGE ( 'NONE', *, *, #14997, .T. ) ;
#10377=CARTESIAN_POINT ( 'NONE',  ( -3.500000000000002220, 15.47927405783632970, -89.87764746908818836 ) ) ;
#10378=CARTESIAN_POINT ( 'NONE',  ( -3.310556943750000425, 19.41135094264166128, -72.84743913623279354 ) ) ;
#10380=ORIENTED_EDGE ( 'NONE', *, *, #33165, .T. ) ;
#10384=VECTOR ( 'NONE', #7188, 1000.000000000000000 ) ;
#10385=ADVANCED_FACE ( 'NONE', ( #27045 ), #40839, .T. ) ;
#10386=ORIENTED_EDGE ( 'NONE', *, *, #19073, .F. ) ;
#10387=AXIS2_PLACEMENT_3D ( 'NONE', #34334, #8804, #37736 ) ;
#10388=CARTESIAN_POINT ( 'NONE',  ( -3.310556943750000425, 19.41135094264167549, -133.8474391362328220 ) ) ;
#10389=CARTESIAN_POINT ( 'NONE',  ( 1.750000000000001110, 20.53108891324556140, -141.2943141357548313 ) ) ;
#10390=( BOUNDED_CURVE ( )  B_SPLINE_CURVE ( 2, ( #37599, #33581, #4441, #21433, #27407, #24425, #14432, #11238, #30800 ),
 .UNSPECIFIED., .F., .T. ) 
 B_SPLINE_CURVE_WITH_KNOTS ( ( 3, 2, 2, 2, 3 ),
 ( 0.6562500000000000000, 0.6569444444444444420, 0.6583333333333333259, 0.6597222222222222099, 0.6604166666666666519 ),
 .UNSPECIFIED. ) 
 CURVE ( )  GEOMETRIC_REPRESENTATION_ITEM ( )  RATIONAL_B_SPLINE_CURVE ( ( 0.9330127018922194093, 0.9330127018922194093, 1.000000000000000000, 0.8660254037844387076, 1.000000000000000000, 0.8660254037844387076, 1.000000000000000000, 0.9330127018922194093, 0.9330127018922194093 ) ) 
 REPRESENTATION_ITEM ( '' )  );
#10391=CARTESIAN_POINT ( 'NONE',  ( 3.310556943750001313, 19.41135094264165772, -36.26827246956612782 ) ) ;
#10392=EDGE_CURVE ( 'NONE', #5239, #41707, #37587, .T. ) ;
#10393=CARTESIAN_POINT ( 'NONE',  ( 2.340729813953370519E-16, 21.32270188528331190, -99.10160580289947063 ) ) ;
#10395=CARTESIAN_POINT ( 'NONE',  ( 3.310556943750001313, 17.50000000000001066, -26.26410580289947916 ) ) ;
#10397=CARTESIAN_POINT ( 'NONE',  ( -1.749999999999999778, 20.53108891324555429, -101.1276474690881741 ) ) ;
#10400=CARTESIAN_POINT ( 'NONE',  ( -1.750000000000002220, 14.46891108675448301, -92.48806413671076143 ) ) ;
#10404=CARTESIAN_POINT ( 'NONE',  ( 1.749999999999998224, 14.46891108675447946, -73.62764746908817415 ) ) ;
#10405=CARTESIAN_POINT ( 'NONE',  ( 3.500000000000000000, 15.47927405783632260, -54.54431413575485266 ) ) ;
#10406=CARTESIAN_POINT ( 'NONE',  ( -0.9378221735089291577, 21.00000000000001776, -89.16632260368299967 ) ) ;
#10407=FACE_OUTER_BOUND ( 'NONE', #18518, .T. ) ;
#10409=CARTESIAN_POINT ( 'NONE',  ( 3.500000000000001776, 19.52072594216370405, -43.07139747004409713 ) ) ;
#10410=CARTESIAN_POINT ( 'NONE',  ( -3.500000000000002220, 15.47927405783633503, -131.8776474690881741 ) ) ;
#10411=CARTESIAN_POINT ( 'NONE',  ( 3.310556943750001313, 17.50000000000001066, -25.35160580289946708 ) ) ;
#10414=CARTESIAN_POINT ( 'NONE',  ( -1.749999999999999778, 20.53108891324555429, -90.82139747004410424 ) ) ;
#10415=VECTOR ( 'NONE', #23962, 1000.000000000000000 ) ;
#10418=CARTESIAN_POINT ( 'NONE',  ( -3.310556943750002201, 15.58864905735837070, -79.68077246956615056 ) ) ;
#10419=CARTESIAN_POINT ( 'NONE',  ( -1.394453263437886604E-15, 14.00000000000001066, -52.71098080242150985 ) ) ;
#10422=CARTESIAN_POINT ( 'NONE',  ( 4.286263797015737581E-16, 14.00000000000002487, -149.5231586289125687 ) ) ;
#10423=ORIENTED_EDGE ( 'NONE', *, *, #34727, .F. ) ;
#10424=CARTESIAN_POINT ( 'NONE',  ( -1.749999999999999778, 20.53108891324555429, -88.12764746908817415 ) ) ;
#10425=CARTESIAN_POINT ( 'NONE',  ( 3.310556943750001313, 17.50000000000001776, -92.26410580289947916 ) ) ;
#10426=ORIENTED_EDGE ( 'NONE', *, *, #21268, .F. ) ;
#10427=VERTEX_POINT ( 'NONE', #37040 ) ;
#10431=CARTESIAN_POINT ( 'NONE',  ( -3.310556943750001313, 17.50000000000002132, -125.7641058028994792 ) ) ;
#10432=VECTOR ( 'NONE', #36722, 1000.000000000000000 ) ;
#10433=ORIENTED_EDGE ( 'NONE', *, *, #9584, .T. ) ;
#10435=CARTESIAN_POINT ( 'NONE',  ( 3.310556943750001313, 17.50000000000001421, -54.35160580289946353 ) ) ;
#10436=EDGE_CURVE ( 'NONE', #29352, #8739, #30857, .T. ) ;
#10437=CARTESIAN_POINT ( 'NONE',  ( 2.340729813953370519E-16, 21.32270188528331900, -118.1016058028994706 ) ) ;
#10438=ORIENTED_EDGE ( 'NONE', *, *, #11486, .T. ) ;
#10439=VERTEX_POINT ( 'NONE', #1512 ) ;
#10440=CARTESIAN_POINT ( 'NONE',  ( -3.500000000000002220, 15.47927405783633503, -123.5713974700440900 ) ) ;
#10441=CARTESIAN_POINT ( 'NONE',  ( 3.310556943750001313, 17.50000000000001066, -37.26410580289947205 ) ) ;
#10443=CARTESIAN_POINT ( 'NONE',  ( 3.310556943750001313, 19.41135094264166128, -72.26827246956612782 ) ) ;
#10444=CARTESIAN_POINT ( 'NONE',  ( -7.424026671074350129E-16, 13.45854811567263987, -117.7109808024215170 ) ) ;
#10445=CARTESIAN_POINT ( 'NONE',  ( 3.310556943750001313, 19.41135094264166838, -102.1807724695661364 ) ) ;
#10449=CARTESIAN_POINT ( 'NONE',  ( -1.750000000000002220, 14.46891108675448123, -68.79431413575484555 ) ) ;
#10450=CARTESIAN_POINT ( 'NONE',  ( 3.500000000000000000, 15.47927405783633326, -122.5443141357548456 ) ) ;
#10451=CARTESIAN_POINT ( 'NONE',  ( 3.310556943749999981, 15.58864905735836182, -35.34743913623280775 ) ) ;
#10452=CARTESIAN_POINT ( 'NONE',  ( -1.655278471875002211, 14.63297358603754894, -95.68493913623279923 ) ) ;
#10453=CARTESIAN_POINT ( 'NONE',  ( 3.500000000000000000, 15.47927405783632260, -61.23806413671076143 ) ) ;
#10454=CARTESIAN_POINT ( 'NONE',  ( 3.310556943750001313, 17.50000000000002132, -110.3516058028994564 ) ) ;
#10455=CARTESIAN_POINT ( 'NONE',  ( -7.022189441860112050E-16, 13.67729811471671830, -44.60160580289947063 ) ) ;
#10457=CARTESIAN_POINT ( 'NONE',  ( -1.750000000000002220, 14.46891108675447946, -60.79431413575483845 ) ) ;
#10462=CARTESIAN_POINT ( 'NONE',  ( -1.655278471875002211, 14.63297358603754716, -93.59743913623280775 ) ) ;
#10468=CARTESIAN_POINT ( 'NONE',  ( -3.500000000000000000, 19.52072594216371826, -112.7380641367107614 ) ) ;
#10473=CARTESIAN_POINT ( 'NONE',  ( 2.340729813953370519E-16, 21.32270188528330834, -28.01410580289947916 ) ) ;
#10475=CARTESIAN_POINT ( 'NONE',  ( 4.648177544792955347E-16, 21.00000000000002132, -109.9047308033774186 ) ) ;
#10479=ORIENTED_EDGE ( 'NONE', *, *, #10625, .F. ) ;
#10481=CARTESIAN_POINT ( 'NONE',  ( 2.340729813953370519E-16, 21.32270188528332255, -142.0141058028994792 ) ) ;
#10483=CARTESIAN_POINT ( 'NONE',  ( 1.655278471875001101, 20.36702641396249902, -135.1849391362327992 ) ) ;
#10484=CARTESIAN_POINT ( 'NONE',  ( 3.500000000000001776, 19.52072594216370405, -28.37764746908817770 ) ) ;
#10486=CARTESIAN_POINT ( 'NONE',  ( -3.500000000000002220, 15.47927405783633503, -141.5713974700441042 ) ) ;
#10490=CARTESIAN_POINT ( 'NONE',  ( -1.749999999999999778, 20.53108891324556140, -135.1276474690881741 ) ) ;
#10491=CARTESIAN_POINT ( 'NONE',  ( -7.022189441860112050E-16, 13.67729811471672718, -116.5141058028994792 ) ) ;
#10494=EDGE_CURVE ( 'NONE', #41304, #36906, #8506, .T. ) ;
#10496=CARTESIAN_POINT ( 'NONE',  ( -1.750000000000002220, 14.46891108675448301, -87.79431413575483134 ) ) ;
#10497=( BOUNDED_CURVE ( )  B_SPLINE_CURVE ( 2, ( #6607, #28723, #12572, #9383, #3615, #9813, #41717, #13, #2999 ),
 .UNSPECIFIED., .F., .F. ) 
 B_SPLINE_CURVE_WITH_KNOTS ( ( 3, 2, 2, 2, 3 ),
 ( 0.1270833333333333259, 0.1277777777777777679, 0.1291666666666666796, 0.1305555555555555636, 0.1312500000000000056 ),
 .UNSPECIFIED. ) 
 CURVE ( )  GEOMETRIC_REPRESENTATION_ITEM ( )  RATIONAL_B_SPLINE_CURVE ( ( 0.9330127018922194093, 0.9330127018922194093, 1.000000000000000000, 0.8660254037844387076, 1.000000000000000000, 0.8660254037844387076, 1.000000000000000000, 0.9330127018922194093, 0.9330127018922194093 ) ) 
 REPRESENTATION_ITEM ( '' )  );
#10498=DIRECTION ( 'NONE',  ( -0.000000000000000000, 1.259100132267607459E-16, -1.000000000000000000 ) ) ;
#10499=CARTESIAN_POINT ( 'NONE',  ( -1.655278471874999990, 20.36702641396248836, -51.93077246956613635 ) ) ;
#10500=CARTESIAN_POINT ( 'NONE',  ( 1.655278471875001101, 20.36702641396249547, -114.1849391362327850 ) ) ;
#10501=EDGE_CURVE ( 'NONE', #29511, #14868, #12869, .T. ) ;
#10502=CARTESIAN_POINT ( 'NONE',  ( 0.9378221735089300459, 21.00000000000001066, -38.25563900116003424 ) ) ;
#10503=CARTESIAN_POINT ( 'NONE',  ( 3.500000000000000000, 15.47927405783632082, -29.23806413671076498 ) ) ;
#10505=AXIS2_PLACEMENT_3D ( 'NONE', #2003, #31352, #34128 ) ;
#10507=CARTESIAN_POINT ( 'NONE',  ( 3.310556943749999981, 15.58864905735837425, -130.4349391362327992 ) ) ;
#10510=CARTESIAN_POINT ( 'NONE',  ( 1.750000000000001110, 20.53108891324555074, -58.29431413575483845 ) ) ;
#10511=CARTESIAN_POINT ( 'NONE',  ( 1.655278471875001101, 20.36702641396248836, -64.18493913623279923 ) ) ;
#10513=CARTESIAN_POINT ( 'NONE',  ( 1.655278471875001101, 20.36702641396248836, -62.09743913623280775 ) ) ;
#10515=CARTESIAN_POINT ( 'NONE',  ( 3.310556943750001313, 17.50000000000001776, -87.35160580289947063 ) ) ;
#10518=DIRECTION ( 'NONE',  ( -0.000000000000000000, 1.259100132267607459E-16, -1.000000000000000000 ) ) ;
#10520=CARTESIAN_POINT ( 'NONE',  ( 1.655278471875001101, 20.36702641396248836, -47.09743913623280775 ) ) ;
#10522=CARTESIAN_POINT ( 'NONE',  ( -3.310556943750000425, 19.41135094264166483, -100.8474391362328220 ) ) ;
#10523=CARTESIAN_POINT ( 'NONE',  ( 0.9378221735089281585, 14.00000000000001066, -53.36007260463890844 ) ) ;
#10528=CARTESIAN_POINT ( 'NONE',  ( -3.310556943750001313, 17.50000000000001421, -53.76410580289947916 ) ) ;
#10529=EDGE_CURVE ( 'NONE', #39031, #2767, #13996, .T. ) ;
#10532=CARTESIAN_POINT ( 'NONE',  ( 4.648177544792955347E-16, 21.00000000000001776, -91.90473080337741862 ) ) ;
#10537=CARTESIAN_POINT ( 'NONE',  ( 4.648177544792955347E-16, 21.00000000000002132, -113.2109808024214885 ) ) ;
#10541=CARTESIAN_POINT ( 'NONE',  ( -7.424026671074350129E-16, 13.45854811567263276, -45.71098080242150274 ) ) ;
#10542=CARTESIAN_POINT ( 'NONE',  ( -3.310556943750002645, 15.58864905735836714, -42.68077246956614346 ) ) ;
#10543=DIRECTION ( 'NONE',  ( 0.000000000000000000, 1.000000000000000000, 0.000000000000000000 ) ) ;
#10546=CARTESIAN_POINT ( 'NONE',  ( -3.310556943750002645, 15.58864905735836537, -27.76827246956613138 ) ) ;
#10547=CARTESIAN_POINT ( 'NONE',  ( 3.310556943750001313, 19.41135094264165772, -24.26827246956612782 ) ) ;
#10548=CARTESIAN_POINT ( 'NONE',  ( 1.655278471875001101, 20.36702641396249192, -84.18493913623278502 ) ) ;
#10549=CARTESIAN_POINT ( 'NONE',  ( -1.655278471874999990, 20.36702641396249902, -133.9307724695661364 ) ) ;
#10555=CARTESIAN_POINT ( 'NONE',  ( -1.655278471875002211, 14.63297358603755249, -127.6849391362327992 ) ) ;
#10558=CARTESIAN_POINT ( 'NONE',  ( 3.500000000000000000, 15.47927405783633503, -141.2380641367107614 ) ) ;
#10559=CARTESIAN_POINT ( 'NONE',  ( -3.310556943750000425, 19.41135094264166483, -87.84743913623279354 ) ) ;
#10560=CARTESIAN_POINT ( 'NONE',  ( 0.000000000000000000, 21.00000000000002487, -149.5231586289125687 ) ) ;
#10563=CARTESIAN_POINT ( 'NONE',  ( 3.500000000000001332, 17.50000000000001776, -75.15473080337743284 ) ) ;
#10564=CARTESIAN_POINT ( 'NONE',  ( -3.310556943750001313, 17.50000000000001421, -57.85160580289947063 ) ) ;
#10568=CARTESIAN_POINT ( 'NONE',  ( 3.310556943749999981, 15.58864905735836714, -78.43493913623278502 ) ) ;
#10569=CARTESIAN_POINT ( 'NONE',  ( -3.310556943750001313, 17.50000000000002487, -141.8516058028994564 ) ) ;
#10571=CARTESIAN_POINT ( 'NONE',  ( 2.340729813953370519E-16, 21.32270188528331900, -109.0141058028994792 ) ) ;
#10572=CARTESIAN_POINT ( 'NONE',  ( 3.310556943750001313, 17.50000000000001421, -74.26410580289947916 ) ) ;
#10574=ORIENTED_EDGE ( 'NONE', *, *, #28049, .F. ) ;
#10575=CARTESIAN_POINT ( 'NONE',  ( 2.340729813953370519E-16, 21.32270188528331900, -103.1016058028994564 ) ) ;
#10576=CARTESIAN_POINT ( 'NONE',  ( -1.749999999999999778, 20.53108891324555429, -101.8213974700440900 ) ) ;
#10580=CARTESIAN_POINT ( 'NONE',  ( -0.9378221735088960731, 14.00000000000000000, -95.44938900211595012 ) ) ;
#10581=CARTESIAN_POINT ( 'NONE',  ( 3.500000000000001332, 17.50000000000001421, -58.15473080337743284 ) ) ;
#10583=CARTESIAN_POINT ( 'NONE',  ( 2.340729813953370519E-16, 21.32270188528331190, -59.01410580289947916 ) ) ;
#10584=CARTESIAN_POINT ( 'NONE',  ( 4.648177544792955347E-16, 21.00000000000002132, -113.2109808024214885 ) ) ;
#10585=CARTESIAN_POINT ( 'NONE',  ( -1.655278471874999990, 20.36702641396249547, -116.9307724695661364 ) ) ;
#10586=CARTESIAN_POINT ( 'NONE',  ( 0.000000000000000000, 17.50000000000002487, -149.5231586289125687 ) ) ;
#10588=EDGE_LOOP ( 'NONE', ( #22504, #38763, #30297, #14602 ) ) ;
#10589=VERTEX_POINT ( 'NONE', #31889 ) ;
#10592=CARTESIAN_POINT ( 'NONE',  ( -1.750000000000002220, 14.46891108675448301, -89.79431413575483134 ) ) ;
#10593=CARTESIAN_POINT ( 'NONE',  ( 2.340729813953370519E-16, 21.32270188528330834, -66.01410580289946495 ) ) ;
#10594=ADVANCED_FACE ( 'NONE', ( #5317 ), #32106, .T. ) ;
#10595=( BOUNDED_CURVE ( )  B_SPLINE_CURVE ( 2, ( #39835, #10695, #18126, #2376, #17916, #30892, #14733, #18538, #18326 ),
 .UNSPECIFIED., .F., .T. ) 
 B_SPLINE_CURVE_WITH_KNOTS ( ( 3, 2, 2, 2, 3 ),
 ( 0.5395833333333333037, 0.5402777777777777457, 0.5416666666666666297, 0.5430555555555555136, 0.5437499999999999556 ),
 .UNSPECIFIED. ) 
 CURVE ( )  GEOMETRIC_REPRESENTATION_ITEM ( )  RATIONAL_B_SPLINE_CURVE ( ( 0.9330127018922194093, 0.9330127018922194093, 1.000000000000000000, 0.8660254037844387076, 1.000000000000000000, 0.8660254037844387076, 1.000000000000000000, 0.9330127018922194093, 0.9330127018922194093 ) ) 
 REPRESENTATION_ITEM ( '' )  );
#10596=VERTEX_POINT ( 'NONE', #41907 ) ;
#10602=CARTESIAN_POINT ( 'NONE',  ( 3.310556943750001313, 17.50000000000002487, -136.2641058028994792 ) ) ;
#10603=DIRECTION ( 'NONE',  ( 0.000000000000000000, 1.000000000000000000, 0.000000000000000000 ) ) ;
#10605=CARTESIAN_POINT ( 'NONE',  ( -3.310556943750002645, 15.58864905735836714, -43.76827246956612782 ) ) ;
#10606=CARTESIAN_POINT ( 'NONE',  ( -3.310556943750001313, 17.50000000000001066, -37.85160580289946353 ) ) ;
#10607=CARTESIAN_POINT ( 'NONE',  ( 1.655278471875001101, 20.36702641396249192, -98.18493913623279923 ) ) ;
#10608=CARTESIAN_POINT ( 'NONE',  ( -3.310556943750001313, 17.50000000000001066, -23.76410580289947561 ) ) ;
#10610=CARTESIAN_POINT ( 'NONE',  ( -1.750000000000002220, 14.46891108675448478, -101.7943141357548456 ) ) ;
#10611=CARTESIAN_POINT ( 'NONE',  ( -3.500000000000000000, 19.52072594216370760, -73.73806413671076143 ) ) ;
#10613=CARTESIAN_POINT ( 'NONE',  ( 1.750000000000001110, 20.53108891324555429, -90.98806413671076143 ) ) ;
#10618=CARTESIAN_POINT ( 'NONE',  ( 1.749999999999998224, 14.46891108675447590, -51.62764746908816704 ) ) ;
#10623=CARTESIAN_POINT ( 'NONE',  ( 3.500000000000000000, 15.47927405783632082, -43.23806413671076143 ) ) ;
#10624=CARTESIAN_POINT ( 'NONE',  ( 1.749999999999998224, 14.46891108675448301, -106.6276474690881741 ) ) ;
#10625=EDGE_CURVE ( 'NONE', #4823, #10596, #17231, .T. ) ;
#10626=CARTESIAN_POINT ( 'NONE',  ( -1.655278471875002211, 14.63297358603753828, -25.68493913623279212 ) ) ;
#10627=CARTESIAN_POINT ( 'NONE',  ( 3.500000000000001332, 17.50000000000001776, -75.15473080337743284 ) ) ;
#10628=CARTESIAN_POINT ( 'NONE',  ( -0.9378221735089291577, 21.00000000000001776, -90.86007260463890134 ) ) ;
#10630=CARTESIAN_POINT ( 'NONE',  ( -0.9378221735089291577, 21.00000000000001066, -33.86007260463891555 ) ) ;
#10632=CARTESIAN_POINT ( 'NONE',  ( -1.655278471875002211, 14.63297358603754539, -77.59743913623280775 ) ) ;
#10633=CARTESIAN_POINT ( 'NONE',  ( -3.500000000000001332, 17.50000000000002487, -133.9609808024214885 ) ) ;
#10634=ORIENTED_EDGE ( 'NONE', *, *, #29002, .F. ) ;
#10635=CARTESIAN_POINT ( 'NONE',  ( 0.000000000000000000, 17.50000000000002487, -149.5231586289125687 ) ) ;
#10636=CARTESIAN_POINT ( 'NONE',  ( -3.500000000000002220, 15.47927405783632615, -54.57139747004410424 ) ) ;
#10639=CARTESIAN_POINT ( 'NONE',  ( -3.500000000000002220, 15.47927405783632970, -87.87764746908817415 ) ) ;
#10640=CARTESIAN_POINT ( 'NONE',  ( -1.655278471875002211, 14.63297358603754716, -82.59743913623279354 ) ) ;
#10643=( BOUNDED_CURVE ( )  B_SPLINE_CURVE ( 2, ( #27222, #40185, #37008, #7231, #16314, #35448, #38637, #35857, #39248 ),
 .UNSPECIFIED., .F., .T. ) 
 B_SPLINE_CURVE_WITH_KNOTS ( ( 3, 2, 2, 2, 3 ),
 ( 0.1312500000000000056, 0.1319444444444444475, 0.1333333333333333315, 0.1347222222222222154, 0.1354166666666666574 ),
 .UNSPECIFIED. ) 
 CURVE ( )  GEOMETRIC_REPRESENTATION_ITEM ( )  RATIONAL_B_SPLINE_CURVE ( ( 0.9330127018922194093, 0.9330127018922194093, 1.000000000000000000, 0.8660254037844387076, 1.000000000000000000, 0.8660254037844387076, 1.000000000000000000, 0.9330127018922194093, 0.9330127018922194093 ) ) 
 REPRESENTATION_ITEM ( '' )  );
#10647=CARTESIAN_POINT ( 'NONE',  ( 1.655278471874998436, 14.63297358603755072, -125.4307724695661364 ) ) ;
#10648=CARTESIAN_POINT ( 'NONE',  ( 4.648177544792955347E-16, 21.00000000000001421, -63.90473080337742573 ) ) ;
#10649=CARTESIAN_POINT ( 'NONE',  ( 1.655278471874998436, 14.63297358603754184, -55.51827246956612782 ) ) ;
#10650=CARTESIAN_POINT ( 'NONE',  ( -3.310556943750000425, 19.41135094264166838, -116.9349391362327850 ) ) ;
#10652=VERTEX_POINT ( 'NONE', #22747 ) ;
#10653=CARTESIAN_POINT ( 'NONE',  ( 3.500000000000001332, 17.50000000000002132, -125.1547308033774328 ) ) ;
#10654=CARTESIAN_POINT ( 'NONE',  ( -3.310556943750001313, 17.50000000000001066, -41.76410580289947916 ) ) ;
#10655=CARTESIAN_POINT ( 'NONE',  ( -7.022189441860112050E-16, 13.67729811471672186, -68.60160580289945642 ) ) ;
#10656=CARTESIAN_POINT ( 'NONE',  ( -1.750000000000002220, 14.46891108675448656, -118.7943141357548313 ) ) ;
#10657=CARTESIAN_POINT ( 'NONE',  ( -3.310556943750002645, 15.58864905735837425, -101.6807724695661364 ) ) ;
#10658=CARTESIAN_POINT ( 'NONE',  ( 0.9378221735089300459, 21.00000000000001421, -59.94938900211595012 ) ) ;
#10660=CARTESIAN_POINT ( 'NONE',  ( 4.648177544792955347E-16, 21.00000000000001776, -85.21098080242151696 ) ) ;
#10662=CARTESIAN_POINT ( 'NONE',  ( 3.500000000000001332, 17.50000000000001421, -67.46098080242150274 ) ) ;
#10663=CARTESIAN_POINT ( 'NONE',  ( 3.500000000000001332, 17.50000000000002132, -122.4609808024215170 ) ) ;
#10664=CARTESIAN_POINT ( 'NONE',  ( -3.310556943750000425, 19.41135094264165772, -35.84743913623281486 ) ) ;
#10665=CARTESIAN_POINT ( 'NONE',  ( 1.655278471874998436, 14.63297358603754716, -98.51827246956612782 ) ) ;
#10666=CARTESIAN_POINT ( 'NONE',  ( 1.750000000000001110, 20.53108891324555074, -59.98806413671076143 ) ) ;
#10668=CARTESIAN_POINT ( 'NONE',  ( 2.340729813953370519E-16, 21.32270188528331900, -115.1016058028994706 ) ) ;
#10669=CARTESIAN_POINT ( 'NONE',  ( -3.310556943750000425, 19.41135094264166128, -42.93493913623279923 ) ) ;
#10676=CARTESIAN_POINT ( 'NONE',  ( 3.310556943749999981, 15.58864905735836892, -92.34743913623282197 ) ) ;
#10678=VERTEX_POINT ( 'NONE', #3186 ) ;
#10681=DIRECTION ( 'NONE',  ( -0.000000000000000000, 1.259100132267607459E-16, -1.000000000000000000 ) ) ;
#10682=EDGE_LOOP ( 'NONE', ( #2585, #28212, #29555, #41175 ) ) ;
#10684=EDGE_CURVE ( 'NONE', #18319, #21133, #27285, .T. ) ;
#10686=CARTESIAN_POINT ( 'NONE',  ( 1.655278471874998436, 14.63297358603753828, -28.43077246956614346 ) ) ;
#10693=CARTESIAN_POINT ( 'NONE',  ( 4.286263797015737581E-16, 14.00000000000002487, -149.5231586289125687 ) ) ;
#10694=CARTESIAN_POINT ( 'NONE',  ( 1.655278471875001101, 20.36702641396249902, -143.0974391362327935 ) ) ;
#10695=CARTESIAN_POINT ( 'NONE',  ( 0.9378221735089281585, 14.00000000000001599, -78.66632260368298546 ) ) ;
#10696=DIRECTION ( 'NONE',  ( -0.000000000000000000, 1.259100132267607459E-16, -1.000000000000000000 ) ) ;
#10697=CARTESIAN_POINT ( 'NONE',  ( 3.310556943750001313, 19.41135094264167549, -130.2682724695661136 ) ) ;
#10698=CARTESIAN_POINT ( 'NONE',  ( -7.424026671074350129E-16, 13.45854811567263098, -30.71098080242150630 ) ) ;
#10699=( BOUNDED_CURVE ( )  B_SPLINE_CURVE ( 2, ( #19699, #32667, #28850, #131, #9727, #9938, #41849, #22263, #26096 ),
 .UNSPECIFIED., .F., .T. ) 
 B_SPLINE_CURVE_WITH_KNOTS ( ( 3, 2, 2, 2, 3 ),
 ( 0.7229166666666666519, 0.7236111111111110938, 0.7249999999999999778, 0.7263888888888888618, 0.7270833333333333037 ),
 .UNSPECIFIED. ) 
 CURVE ( )  GEOMETRIC_REPRESENTATION_ITEM ( )  RATIONAL_B_SPLINE_CURVE ( ( 0.9330127018922194093, 0.9330127018922194093, 1.000000000000000000, 0.8660254037844387076, 1.000000000000000000, 0.8660254037844387076, 1.000000000000000000, 0.9330127018922194093, 0.9330127018922194093 ) ) 
 REPRESENTATION_ITEM ( '' )  );
#10701=CARTESIAN_POINT ( 'NONE',  ( 1.750000000000001110, 20.53108891324556140, -142.9880641367107614 ) ) ;
#10702=CARTESIAN_POINT ( 'NONE',  ( -1.394453263437886604E-15, 14.00000000000002132, -123.7109808024214885 ) ) ;
#10704=CARTESIAN_POINT ( 'NONE',  ( 2.474675557024783212E-16, 21.54145188432740810, -132.2109808024214885 ) ) ;
#10705=CARTESIAN_POINT ( 'NONE',  ( 3.310556943750001313, 17.50000000000002132, -116.2641058028994792 ) ) ;
#10708=CARTESIAN_POINT ( 'NONE',  ( -7.424026671074350129E-16, 13.45854811567263631, -84.71098080242150274 ) ) ;
#10709=CARTESIAN_POINT ( 'NONE',  ( 1.655278471874998436, 14.63297358603754184, -55.43077246956613635 ) ) ;
#10710=CARTESIAN_POINT ( 'NONE',  ( 3.310556943750001313, 17.50000000000002132, -112.3516058028994564 ) ) ;
#10713=CARTESIAN_POINT ( 'NONE',  ( -3.310556943750000425, 19.41135094264166838, -127.9349391362327992 ) ) ;
#10716=FACE_OUTER_BOUND ( 'NONE', #38971, .T. ) ;
#10717=CARTESIAN_POINT ( 'NONE',  ( 3.310556943749999981, 15.58864905735836537, -65.43493913623279923 ) ) ;
#10721=CARTESIAN_POINT ( 'NONE',  ( -1.655278471875002211, 14.63297358603754539, -80.68493913623279923 ) ) ;
#10724=CARTESIAN_POINT ( 'NONE',  ( 0.000000000000000000, 17.50000000000002487, -149.5231586289125687 ) ) ;
#10726=CARTESIAN_POINT ( 'NONE',  ( 2.340729813953370519E-16, 21.32270188528330834, -46.01410580289947205 ) ) ;
#10728=CARTESIAN_POINT ( 'NONE',  ( 3.310556943750001313, 19.41135094264166483, -99.18077246956613635 ) ) ;
#10729=CARTESIAN_POINT ( 'NONE',  ( 4.648177544792955347E-16, 21.00000000000001066, -41.90473080337742573 ) ) ;
#10733=VERTEX_POINT ( 'NONE', #26792 ) ;
#10735=CARTESIAN_POINT ( 'NONE',  ( 3.310556943749999981, 15.58864905735836537, -54.34743913623282907 ) ) ;
#10738=CARTESIAN_POINT ( 'NONE',  ( 4.648177544792955347E-16, 21.00000000000001776, -98.90473080337744705 ) ) ;
#10741=DIRECTION ( 'NONE',  ( -0.000000000000000000, 1.259100132267607459E-16, -1.000000000000000000 ) ) ;
#10744=CARTESIAN_POINT ( 'NONE',  ( 3.500000000000001776, 19.52072594216370405, -45.37764746908817415 ) ) ;
#10745=CARTESIAN_POINT ( 'NONE',  ( 3.500000000000001332, 19.52072594216371115, -97.07139747004409003 ) ) ;
#10746=CARTESIAN_POINT ( 'NONE',  ( 3.500000000000001332, 17.50000000000001776, -78.15473080337741862 ) ) ;
#10747=( BOUNDED_CURVE ( )  B_SPLINE_CURVE ( 2, ( #14826, #13997, #7828, #27793, #26971, #4421, #14410, #27178, #39934 ),
 .UNSPECIFIED., .F., .T. ) 
 B_SPLINE_CURVE_WITH_KNOTS ( ( 3, 2, 2, 2, 3 ),
 ( 0.4687500000000000000, 0.4694444444444444420, 0.4708333333333333259, 0.4722222222222222099, 0.4729166666666666519 ),
 .UNSPECIFIED. ) 
 CURVE ( )  GEOMETRIC_REPRESENTATION_ITEM ( )  RATIONAL_B_SPLINE_CURVE ( ( 0.9330127018922194093, 0.9330127018922194093, 1.000000000000000000, 0.8660254037844387076, 1.000000000000000000, 0.8660254037844387076, 1.000000000000000000, 0.9330127018922194093, 0.9330127018922194093 ) ) 
 REPRESENTATION_ITEM ( '' )  );
#10749=CARTESIAN_POINT ( 'NONE',  ( 1.655278471874998436, 14.63297358603753828, -28.51827246956613493 ) ) ;
#10751=CARTESIAN_POINT ( 'NONE',  ( -1.655278471875002211, 14.63297358603754716, -84.68493913623278502 ) ) ;
#10752=CARTESIAN_POINT ( 'NONE',  ( 2.340729813953370519E-16, 21.32270188528332255, -132.0141058028994507 ) ) ;
#10757=CARTESIAN_POINT ( 'NONE',  ( -1.655278471875002211, 14.63297358603755249, -126.6849391362327992 ) ) ;
#10758=CARTESIAN_POINT ( 'NONE',  ( -3.500000000000000000, 19.52072594216370760, -69.04431413575484555 ) ) ;
#10759=CARTESIAN_POINT ( 'NONE',  ( 3.310556943750001313, 17.50000000000001776, -87.26410580289947916 ) ) ;
#10760=CARTESIAN_POINT ( 'NONE',  ( 0.000000000000000000, 17.50000000000002487, -149.5231586289125687 ) ) ;
#10761=CARTESIAN_POINT ( 'NONE',  ( 0.9378221735089281585, 14.00000000000001599, -75.66632260368298546 ) ) ;
#10763=CARTESIAN_POINT ( 'NONE',  ( -3.500000000000000888, 19.52072594216370760, -70.73806413671074722 ) ) ;
#10765=CARTESIAN_POINT ( 'NONE',  ( 1.655278471874998436, 14.63297358603754006, -51.51827246956612782 ) ) ;
#10769=CARTESIAN_POINT ( 'NONE',  ( 3.310556943750001313, 17.50000000000001776, -81.35160580289945642 ) ) ;
#10770=CARTESIAN_POINT ( 'NONE',  ( -1.655278471875002211, 14.63297358603755427, -142.6849391362327992 ) ) ;
#10772=CARTESIAN_POINT ( 'NONE',  ( 3.310556943749999981, 15.58864905735837070, -107.3474391362328220 ) ) ;
#10773=CARTESIAN_POINT ( 'NONE',  ( 3.310556943749999981, 15.58864905735836714, -76.34743913623280775 ) ) ;
#10774=CARTESIAN_POINT ( 'NONE',  ( -3.500000000000001332, 17.50000000000002132, -115.6547308033774328 ) ) ;
#10776=CARTESIAN_POINT ( 'NONE',  ( -1.655278471875002211, 14.63297358603754894, -96.68493913623279923 ) ) ;
#10777=CARTESIAN_POINT ( 'NONE',  ( 1.749999999999998224, 14.46891108675448301, -102.3213974700440900 ) ) ;
#10780=CARTESIAN_POINT ( 'NONE',  ( 0.000000000000000000, 17.50000000000002487, -149.5231586289125687 ) ) ;
#10782=CARTESIAN_POINT ( 'NONE',  ( 1.655278471874998436, 14.63297358603754184, -63.43077246956614346 ) ) ;
#10783=CARTESIAN_POINT ( 'NONE',  ( -3.500000000000000000, 19.52072594216371826, -125.0443141357548456 ) ) ;
#10784=CARTESIAN_POINT ( 'NONE',  ( 3.310556943750001313, 17.50000000000002132, -116.2641058028994792 ) ) ;
#10789=ORIENTED_EDGE ( 'NONE', *, *, #35900, .F. ) ;
#10793=CARTESIAN_POINT ( 'NONE',  ( 1.655278471874998436, 14.63297358603754361, -69.43077246956613635 ) ) ;
#10795=ORIENTED_EDGE ( 'NONE', *, *, #33888, .T. ) ;
#10802=ORIENTED_EDGE ( 'NONE', *, *, #31612, .T. ) ;
#10803=CARTESIAN_POINT ( 'NONE',  ( -1.655278471874999990, 20.36702641396249902, -136.9307724695661364 ) ) ;
#10805=CARTESIAN_POINT ( 'NONE',  ( -3.310556943750002645, 15.58864905735836714, -45.76827246956613493 ) ) ;
#10806=CARTESIAN_POINT ( 'NONE',  ( 1.749999999999998224, 14.46891108675448656, -134.6276474690881741 ) ) ;
#10807=CARTESIAN_POINT ( 'NONE',  ( 2.340729813953370519E-16, 21.32270188528330479, -37.10160580289946353 ) ) ;
#10808=CARTESIAN_POINT ( 'NONE',  ( -7.022189441860112050E-16, 13.67729811471672541, -97.60160580289945642 ) ) ;
#10810=AXIS2_PLACEMENT_3D ( 'NONE', #7844, #823, #27195 ) ;
#10811=CARTESIAN_POINT ( 'NONE',  ( -1.655278471875002211, 14.63297358603755427, -142.6849391362327992 ) ) ;
#10812=CARTESIAN_POINT ( 'NONE',  ( -3.500000000000000888, 19.52072594216371826, -103.0443141357548456 ) ) ;
#10815=CARTESIAN_POINT ( 'NONE',  ( 3.500000000000001332, 17.50000000000001776, -89.15473080337743284 ) ) ;
#10817=CARTESIAN_POINT ( 'NONE',  ( 1.655278471874998436, 14.63297358603754361, -70.51827246956612782 ) ) ;
#10819=CARTESIAN_POINT ( 'NONE',  ( -3.500000000000000000, 19.52072594216371826, -111.7380641367107756 ) ) ;
#10822=CARTESIAN_POINT ( 'NONE',  ( 1.749999999999998224, 14.46891108675448478, -110.6276474690881741 ) ) ;
#10823=CARTESIAN_POINT ( 'NONE',  ( -3.500000000000002220, 15.47927405783632260, -52.87764746908816704 ) ) ;
#10824=CARTESIAN_POINT ( 'NONE',  ( -3.500000000000000000, 19.52072594216370760, -74.04431413575484555 ) ) ;
#10826=CARTESIAN_POINT ( 'NONE',  ( -3.500000000000001332, 17.50000000000001066, -34.96098080242150985 ) ) ;
#10829=EDGE_CURVE ( 'NONE', #18643, #15608, #27827, .T. ) ;
#10830=CARTESIAN_POINT ( 'NONE',  ( 1.750000000000001110, 20.53108891324554719, -43.98806413671076143 ) ) ;
#10831=CARTESIAN_POINT ( 'NONE',  ( 3.310556943749999981, 15.58864905735836182, -29.43493913623279923 ) ) ;
#10835=CARTESIAN_POINT ( 'NONE',  ( 3.500000000000001332, 17.50000000000001066, -36.15473080337743284 ) ) ;
#10837=CARTESIAN_POINT ( 'NONE',  ( 2.340729813953370519E-16, 21.32270188528331190, -79.01410580289945074 ) ) ;
#10840=CYLINDRICAL_SURFACE ( 'NONE', #20678, 3.499999999999999556 ) ;
#10841=CARTESIAN_POINT ( 'NONE',  ( 3.500000000000001332, 17.50000000000001776, -90.15473080337743284 ) ) ;
#10843=CARTESIAN_POINT ( 'NONE',  ( -7.460324959392693302E-14, 21.00000000000001776, -88.21098080242150274 ) ) ;
#10844=CARTESIAN_POINT ( 'NONE',  ( 2.340729813953370519E-16, 21.32270188528331190, -82.01410580289947916 ) ) ;
#10846=ORIENTED_EDGE ( 'NONE', *, *, #37107, .F. ) ;
#10853=CARTESIAN_POINT ( 'NONE',  ( 3.310556943749999981, 15.58864905735837425, -128.3474391362328220 ) ) ;
#10856=CARTESIAN_POINT ( 'NONE',  ( 3.310556943750001313, 19.41135094264166128, -56.26827246956613493 ) ) ;
#10857=CARTESIAN_POINT ( 'NONE',  ( 2.340729813953370519E-16, 21.32270188528331900, -117.1016058028994564 ) ) ;
#10859=ORIENTED_EDGE ( 'NONE', *, *, #634, .F. ) ;
#10860=CARTESIAN_POINT ( 'NONE',  ( -1.750000000000002220, 14.46891108675448834, -127.4880641367107614 ) ) ;
#10861=CARTESIAN_POINT ( 'NONE',  ( 1.655278471875001101, 20.36702641396248481, -40.09743913623281486 ) ) ;
#10862=CARTESIAN_POINT ( 'NONE',  ( 3.310556943749999981, 15.58864905735836537, -65.43493913623279923 ) ) ;
#10863=CARTESIAN_POINT ( 'NONE',  ( 3.500000000000000000, 15.47927405783632970, -115.5443141357548313 ) ) ;
#10864=CARTESIAN_POINT ( 'NONE',  ( -7.022189441860112050E-16, 13.67729811471672541, -102.5141058028994649 ) ) ;
#10865=EDGE_CURVE ( 'NONE', #34369, #36839, #30255, .T. ) ;
#10866=CARTESIAN_POINT ( 'NONE',  ( 4.648177544792955347E-16, 21.00000000000001421, -68.90473080337741862 ) ) ;
#10870=CARTESIAN_POINT ( 'NONE',  ( 3.500000000000000000, 15.47927405783632437, -69.54431413575484555 ) ) ;
#10871=AXIS2_PLACEMENT_3D ( 'NONE', #18155, #31333, #2194 ) ;
#10872=CARTESIAN_POINT ( 'NONE',  ( 0.9378221735089300459, 21.00000000000001776, -100.2556390011600342 ) ) ;
#10873=CARTESIAN_POINT ( 'NONE',  ( -1.655278471875002211, 14.63297358603754006, -29.59743913623280775 ) ) ;
#10874=CARTESIAN_POINT ( 'NONE',  ( 2.340729813953370519E-16, 21.32270188528331190, -90.10160580289947063 ) ) ;
#10876=( BOUNDED_CURVE ( )  B_SPLINE_CURVE ( 2, ( #37159, #23763, #20982, #13978, #30977, #1833, #40748, #17383, #4609 ),
 .UNSPECIFIED., .F., .F. ) 
 B_SPLINE_CURVE_WITH_KNOTS ( ( 3, 2, 2, 2, 3 ),
 ( 0.5104166666666666297, 0.5111111111111110716, 0.5124999999999999556, 0.5138888888888888395, 0.5145833333333332815 ),
 .UNSPECIFIED. ) 
 CURVE ( )  GEOMETRIC_REPRESENTATION_ITEM ( )  RATIONAL_B_SPLINE_CURVE ( ( 0.9330127018922194093, 0.9330127018922194093, 1.000000000000000000, 0.8660254037844387076, 1.000000000000000000, 0.8660254037844387076, 1.000000000000000000, 0.9330127018922194093, 0.9330127018922194093 ) ) 
 REPRESENTATION_ITEM ( '' )  );
#10877=CARTESIAN_POINT ( 'NONE',  ( 3.500000000000001776, 19.52072594216370760, -58.07139747004409713 ) ) ;
#10879=CARTESIAN_POINT ( 'NONE',  ( 1.655278471875001101, 20.36702641396249547, -115.1849391362327850 ) ) ;
#10880=CARTESIAN_POINT ( 'NONE',  ( 1.655278471874998436, 14.63297358603754006, -44.51827246956613493 ) ) ;
#10887=CARTESIAN_POINT ( 'NONE',  ( 2.340729813953370519E-16, 21.32270188528331190, -92.01410580289947916 ) ) ;
#10890=ORIENTED_EDGE ( 'NONE', *, *, #2898, .F. ) ;
#10900=DIRECTION ( 'NONE',  ( 0.000000000000000000, 1.000000000000000000, 0.000000000000000000 ) ) ;
#10904=ORIENTED_EDGE ( 'NONE', *, *, #28473, .F. ) ;
#10908=CARTESIAN_POINT ( 'NONE',  ( 7.367361408496833051E-14, 14.00000000000002132, -110.4047308033774328 ) ) ;
#10910=CARTESIAN_POINT ( 'NONE',  ( -3.500000000000002220, 15.47927405783632793, -74.87764746908817415 ) ) ;
#10911=CARTESIAN_POINT ( 'NONE',  ( -3.310556943750002645, 15.58864905735837780, -129.7682724695661420 ) ) ;
#10912=CARTESIAN_POINT ( 'NONE',  ( -3.500000000000000888, 19.52072594216370405, -30.04431413575484200 ) ) ;
#10914=CARTESIAN_POINT ( 'NONE',  ( -1.749999999999999778, 20.53108891324556140, -139.8213974700441042 ) ) ;
#10918=CARTESIAN_POINT ( 'NONE',  ( -1.749999999999999778, 20.53108891324556140, -132.1276474690881741 ) ) ;
#10919=CARTESIAN_POINT ( 'NONE',  ( 1.655278471874998436, 14.63297358603754894, -118.4307724695661364 ) ) ;
#10922=CARTESIAN_POINT ( 'NONE',  ( -1.749999999999999778, 20.53108891324555429, -84.12764746908818836 ) ) ;
#10923=CARTESIAN_POINT ( 'NONE',  ( -1.394453263437886604E-15, 14.00000000000001421, -69.40473080337741862 ) ) ;
#10924=CARTESIAN_POINT ( 'NONE',  ( 3.310556943750001313, 17.50000000000001421, -54.26410580289947916 ) ) ;
#10925=CARTESIAN_POINT ( 'NONE',  ( 1.655278471875001101, 20.36702641396249547, -106.1849391362327992 ) ) ;
#10929=CARTESIAN_POINT ( 'NONE',  ( -3.310556943750002201, 15.58864905735837780, -129.7682724695661136 ) ) ;
#10931=CARTESIAN_POINT ( 'NONE',  ( 0.000000000000000000, 21.00000000000002487, -149.5231586289125687 ) ) ;
#10932=LINE ( 'NONE', #20720, #18746 ) ;
#10933=CARTESIAN_POINT ( 'NONE',  ( 0.9378221735088952959, 21.00000000000003908, -85.94938900211593591 ) ) ;
#10934=CARTESIAN_POINT ( 'NONE',  ( 3.310556943750001313, 19.41135094264166128, -64.26827246956614204 ) ) ;
#10935=VECTOR ( 'NONE', #35470, 1000.000000000000000 ) ;
#10936=ORIENTED_EDGE ( 'NONE', *, *, #39614, .T. ) ;
#10937=CARTESIAN_POINT ( 'NONE',  ( -7.022189441860112050E-16, 13.67729811471672363, -82.60160580289947063 ) ) ;
#10939=CARTESIAN_POINT ( 'NONE',  ( 4.648177544792955347E-16, 21.00000000000002132, -113.9047308033774186 ) ) ;
#10942=CARTESIAN_POINT ( 'NONE',  ( -1.655278471875002211, 14.63297358603754184, -46.59743913623280775 ) ) ;
#10943=CARTESIAN_POINT ( 'NONE',  ( 3.310556943750001313, 17.50000000000001776, -99.26410580289947916 ) ) ;
#10945=EDGE_LOOP ( 'NONE', ( #37376, #7883, #26372, #17736 ) ) ;
#10947=EDGE_LOOP ( 'NONE', ( #36573, #12302, #1538, #20363 ) ) ;
#10949=CARTESIAN_POINT ( 'NONE',  ( 3.310556943750001313, 17.50000000000001421, -54.26410580289947916 ) ) ;
#10950=( BOUNDED_CURVE ( )  B_SPLINE_CURVE ( 2, ( #24137, #8365, #37308, #1159, #14556, #33702, #11552, #27934, #1983 ),
 .UNSPECIFIED., .F., .F. ) 
 B_SPLINE_CURVE_WITH_KNOTS ( ( 3, 2, 2, 2, 3 ),
 ( 0.5479166666666667185, 0.5486111111111111605, 0.5500000000000000444, 0.5513888888888889284, 0.5520833333333333703 ),
 .UNSPECIFIED. ) 
 CURVE ( )  GEOMETRIC_REPRESENTATION_ITEM ( )  RATIONAL_B_SPLINE_CURVE ( ( 0.9330127018922194093, 0.9330127018922194093, 1.000000000000000000, 0.8660254037844387076, 1.000000000000000000, 0.8660254037844387076, 1.000000000000000000, 0.9330127018922194093, 0.9330127018922194093 ) ) 
 REPRESENTATION_ITEM ( '' )  );
#10952=ORIENTED_EDGE ( 'NONE', *, *, #41015, .F. ) ;
#10954=CARTESIAN_POINT ( 'NONE',  ( 7.367361408496833051E-14, 14.00000000000001776, -93.71098080242150274 ) ) ;
#10960=CARTESIAN_POINT ( 'NONE',  ( 3.500000000000000000, 15.47927405783632082, -45.54431413575483845 ) ) ;
#10962=CARTESIAN_POINT ( 'NONE',  ( -1.394453263437886604E-15, 14.00000000000001421, -71.71098080242150274 ) ) ;
#10964=CARTESIAN_POINT ( 'NONE',  ( -1.655278471875002211, 14.63297358603754006, -28.68493913623279568 ) ) ;
#10965=DIRECTION ( 'NONE',  ( 6.123233995736763571E-17, 0.4999999999999997224, 0.8660254037844388186 ) ) ;
#10966=CARTESIAN_POINT ( 'NONE',  ( -1.655278471875002211, 14.63297358603754716, -83.68493913623278502 ) ) ;
#10967=CARTESIAN_POINT ( 'NONE',  ( 3.310556943750001313, 19.41135094264167549, -132.1807724695661364 ) ) ;
#10968=EDGE_CURVE ( 'NONE', #36901, #20880, #4237, .T. ) ;
#10971=CARTESIAN_POINT ( 'NONE',  ( -1.749999999999999778, 20.53108891324555429, -75.82139747004410424 ) ) ;
#10972=VECTOR ( 'NONE', #4272, 1000.000000000000000 ) ;
#10973=CARTESIAN_POINT ( 'NONE',  ( 2.340729813953370519E-16, 21.32270188528331900, -128.1016058028994848 ) ) ;
#10974=DIRECTION ( 'NONE',  ( -0.000000000000000000, 1.259100132267607459E-16, -1.000000000000000000 ) ) ;
#10975=CARTESIAN_POINT ( 'NONE',  ( -1.655278471874999990, 20.36702641396249192, -84.93077246956613635 ) ) ;
#10976=CARTESIAN_POINT ( 'NONE',  ( 4.648177544792955347E-16, 21.00000000000001776, -98.90473080337743284 ) ) ;
#10977=DIRECTION ( 'NONE',  ( 0.000000000000000000, 1.000000000000000000, 0.000000000000000000 ) ) ;
#10978=CARTESIAN_POINT ( 'NONE',  ( -1.394453263437886604E-15, 14.00000000000001421, -67.40473080337741862 ) ) ;
#10979=CARTESIAN_POINT ( 'NONE',  ( -3.500000000000002220, 15.47927405783632615, -70.57139747004409003 ) ) ;
#10980=CARTESIAN_POINT ( 'NONE',  ( 1.655278471874998436, 14.63297358603754184, -54.51827246956612782 ) ) ;
#10982=CARTESIAN_POINT ( 'NONE',  ( -1.749999999999999778, 20.53108891324555074, -67.82139747004409003 ) ) ;
#10983=CARTESIAN_POINT ( 'NONE',  ( -3.500000000000000000, 19.52072594216370760, -49.04431413575484555 ) ) ;
#10984=CARTESIAN_POINT ( 'NONE',  ( -7.022189441860112050E-16, 13.67729811471672186, -79.60160580289945642 ) ) ;
#10985=CARTESIAN_POINT ( 'NONE',  ( 1.655278471875001101, 20.36702641396249902, -139.1849391362327708 ) ) ;
#10987=CARTESIAN_POINT ( 'NONE',  ( 2.340729813953370519E-16, 21.32270188528331900, -102.0141058028994649 ) ) ;
#10988=CARTESIAN_POINT ( 'NONE',  ( -1.655278471874999990, 20.36702641396249192, -76.93077246956615056 ) ) ;
#10989=DIRECTION ( 'NONE',  ( 0.000000000000000000, 1.000000000000000000, 0.000000000000000000 ) ) ;
#10990=ORIENTED_EDGE ( 'NONE', *, *, #1469, .T. ) ;
#10991=CARTESIAN_POINT ( 'NONE',  ( -3.310556943750000425, 19.41135094264166838, -94.93493913623281344 ) ) ;
#10992=CARTESIAN_POINT ( 'NONE',  ( 1.749999999999998224, 14.46891108675448301, -99.32139747004409003 ) ) ;
#10994=CARTESIAN_POINT ( 'NONE',  ( -3.500000000000002220, 15.47927405783632970, -85.57139747004409003 ) ) ;
#10997=CARTESIAN_POINT ( 'NONE',  ( -1.655278471874999990, 20.36702641396248836, -58.93077246956614346 ) ) ;
#10998=DIRECTION ( 'NONE',  ( -0.000000000000000000, 1.259100132267607459E-16, -1.000000000000000000 ) ) ;
#10999=CARTESIAN_POINT ( 'NONE',  ( 3.310556943750001313, 17.50000000000002132, -114.2641058028994792 ) ) ;
#11005=CARTESIAN_POINT ( 'NONE',  ( -1.394453263437886604E-15, 14.00000000000001776, -97.40473080337741862 ) ) ;
#11006=CARTESIAN_POINT ( 'NONE',  ( 4.648177544792955347E-16, 21.00000000000002132, -110.2109808024215170 ) ) ;
#11007=CARTESIAN_POINT ( 'NONE',  ( 3.310556943750001313, 19.41135094264166128, -67.18077246956613635 ) ) ;
#11010=( BOUNDED_CURVE ( )  B_SPLINE_CURVE ( 2, ( #3029, #35146, #21547, #2187, #18985, #2403, #28342, #15169, #28134 ),
 .UNSPECIFIED., .F., .T. ) 
 B_SPLINE_CURVE_WITH_KNOTS ( ( 3, 2, 2, 2, 3 ),
 ( 0.7729166666666666963, 0.7736111111111111382, 0.7750000000000000222, 0.7763888888888889062, 0.7770833333333333481 ),
 .UNSPECIFIED. ) 
 CURVE ( )  GEOMETRIC_REPRESENTATION_ITEM ( )  RATIONAL_B_SPLINE_CURVE ( ( 0.9330127018922194093, 0.9330127018922194093, 1.000000000000000000, 0.8660254037844387076, 1.000000000000000000, 0.8660254037844387076, 1.000000000000000000, 0.9330127018922194093, 0.9330127018922194093 ) ) 
 REPRESENTATION_ITEM ( '' )  );
#11011=CARTESIAN_POINT ( 'NONE',  ( 0.000000000000000000, 17.50000000000002487, -149.5231586289125687 ) ) ;
#11012=AXIS2_PLACEMENT_3D ( 'NONE', #36930, #30114, #991 ) ;
#11018=CARTESIAN_POINT ( 'NONE',  ( -1.655278471874999990, 20.36702641396249902, -134.9307724695661364 ) ) ;
#11019=CARTESIAN_POINT ( 'NONE',  ( -0.9378221735089310451, 14.00000000000002309, -115.7556390011600058 ) ) ;
#11020=CARTESIAN_POINT ( 'NONE',  ( 1.655278471875001101, 20.36702641396248481, -46.18493913623279923 ) ) ;
#11022=CARTESIAN_POINT ( 'NONE',  ( -7.022189441860112050E-16, 13.67729811471671475, -37.60160580289947063 ) ) ;
#11024=CARTESIAN_POINT ( 'NONE',  ( -1.655278471874999990, 20.36702641396249192, -96.01827246956612782 ) ) ;
#11027=CARTESIAN_POINT ( 'NONE',  ( -3.310556943750002645, 15.58864905735836182, -23.68077246956613635 ) ) ;
#11029=CARTESIAN_POINT ( 'NONE',  ( 1.750000000000001110, 20.53108891324555429, -97.29431413575484555 ) ) ;
#11032=CARTESIAN_POINT ( 'NONE',  ( -7.424026671074350129E-16, 13.45854811567263631, -84.40473080337743284 ) ) ;
#11033=CARTESIAN_POINT ( 'NONE',  ( 3.310556943750001313, 19.41135094264166483, -67.26827246956612782 ) ) ;
#11036=EDGE_CURVE ( 'NONE', #5090, #22963, #31619, .T. ) ;
#11039=CARTESIAN_POINT ( 'NONE',  ( 2.474675557024783212E-16, 21.54145188432739388, -50.21098080242150985 ) ) ;
#11040=CARTESIAN_POINT ( 'NONE',  ( -3.500000000000000000, 19.52072594216370405, -30.73806413671076143 ) ) ;
#11043=ORIENTED_EDGE ( 'NONE', *, *, #12967, .T. ) ;
#11045=CARTESIAN_POINT ( 'NONE',  ( 1.749999999999998224, 14.46891108675448478, -113.3213974700440900 ) ) ;
#11046=CARTESIAN_POINT ( 'NONE',  ( 4.648177544792955347E-16, 21.00000000000001421, -54.90473080337742573 ) ) ;
#11047=CARTESIAN_POINT ( 'NONE',  ( 3.310556943750001313, 17.50000000000001066, -24.35160580289946708 ) ) ;
#11048=CARTESIAN_POINT ( 'NONE',  ( 0.000000000000000000, 17.50000000000002487, -149.5231586289125687 ) ) ;
#11052=CARTESIAN_POINT ( 'NONE',  ( 3.310556943750001313, 19.41135094264166838, -79.18077246956615056 ) ) ;
#11053=CARTESIAN_POINT ( 'NONE',  ( 0.9378221735089281585, 14.00000000000002132, -98.66632260368298546 ) ) ;
#11059=DIRECTION ( 'NONE',  ( -0.000000000000000000, 1.259100132267607459E-16, -1.000000000000000000 ) ) ;
#11060=CARTESIAN_POINT ( 'NONE',  ( 3.310556943750001313, 19.41135094264166483, -85.18077246956613635 ) ) ;
#11062=EDGE_LOOP ( 'NONE', ( #8655, #31022, #35985, #6182 ) ) ;
#11063=VERTEX_POINT ( 'NONE', #37818 ) ;
#11067=CARTESIAN_POINT ( 'NONE',  ( -1.750000000000002220, 14.46891108675447946, -58.79431413575483845 ) ) ;
#11068=EDGE_CURVE ( 'NONE', #23575, #1891, #40321, .T. ) ;
#11070=CARTESIAN_POINT ( 'NONE',  ( -3.310556943750001313, 17.50000000000001421, -54.85160580289946353 ) ) ;
#11071=CARTESIAN_POINT ( 'NONE',  ( -1.655278471874999990, 20.36702641396249547, -112.0182724695661420 ) ) ;
#11072=EDGE_LOOP ( 'NONE', ( #6215, #30516, #27110, #41186 ) ) ;
#11073=CARTESIAN_POINT ( 'NONE',  ( 2.474675557024783212E-16, 21.54145188432740099, -124.9047308033774328 ) ) ;
#11074=CARTESIAN_POINT ( 'NONE',  ( 1.655278471875001101, 20.36702641396248481, -41.09743913623280065 ) ) ;
#11075=CARTESIAN_POINT ( 'NONE',  ( -3.310556943750002645, 15.58864905735837070, -67.76827246956612782 ) ) ;
#11076=CARTESIAN_POINT ( 'NONE',  ( -1.750000000000002220, 14.46891108675448656, -114.7943141357548313 ) ) ;
#11077=CARTESIAN_POINT ( 'NONE',  ( 1.655278471874998436, 14.63297358603754716, -99.43077246956613635 ) ) ;
#11079=FACE_OUTER_BOUND ( 'NONE', #32914, .T. ) ;
#11081=DIRECTION ( 'NONE',  ( -0.000000000000000000, 1.259100132267607459E-16, -1.000000000000000000 ) ) ;
#11085=CARTESIAN_POINT ( 'NONE',  ( -1.749999999999999778, 20.53108891324555074, -70.12764746908817415 ) ) ;
#11086=DIRECTION ( 'NONE',  ( -0.000000000000000000, 1.259100132267607459E-16, -1.000000000000000000 ) ) ;
#11087=CARTESIAN_POINT ( 'NONE',  ( -3.310556943750002645, 15.58864905735836537, -30.68077246956614346 ) ) ;
#11088=CARTESIAN_POINT ( 'NONE',  ( -7.022189441860112050E-16, 13.67729811471672363, -89.60160580289947063 ) ) ;
#11089=CARTESIAN_POINT ( 'NONE',  ( -3.500000000000002220, 15.47927405783632437, -57.57139747004410424 ) ) ;
#11090=CARTESIAN_POINT ( 'NONE',  ( 1.749999999999998224, 14.46891108675448123, -92.62764746908815994 ) ) ;
#11091=CARTESIAN_POINT ( 'NONE',  ( -3.310556943750001313, 17.50000000000002132, -112.8516058028994564 ) ) ;
#11092=CARTESIAN_POINT ( 'NONE',  ( 3.310556943749999981, 15.58864905735836182, -38.43493913623280633 ) ) ;
#11099=CARTESIAN_POINT ( 'NONE',  ( 3.310556943750001313, 17.50000000000001776, -95.26410580289946495 ) ) ;
#11105=DIRECTION ( 'NONE',  ( 0.000000000000000000, 1.000000000000000000, 0.000000000000000000 ) ) ;
#11106=EDGE_LOOP ( 'NONE', ( #4976, #20220, #5658, #31966 ) ) ;
#11116=EDGE_CURVE ( 'NONE', #41462, #17447, #38452, .T. ) ;
#11121=CARTESIAN_POINT ( 'NONE',  ( 3.310556943750001313, 19.41135094264167549, -140.1807724695661364 ) ) ;
#11122=AXIS2_PLACEMENT_3D ( 'NONE', #11048, #34010, #33804 ) ;
#11123=CARTESIAN_POINT ( 'NONE',  ( 4.648177544792955347E-16, 21.00000000000002132, -109.9047308033774186 ) ) ;
#11124=FACE_OUTER_BOUND ( 'NONE', #17347, .T. ) ;
#11125=CARTESIAN_POINT ( 'NONE',  ( -1.655278471875002211, 14.63297358603755249, -132.6849391362327992 ) ) ;
#11126=CARTESIAN_POINT ( 'NONE',  ( -3.310556943750001313, 17.50000000000001421, -54.85160580289946353 ) ) ;
#11127=VERTEX_POINT ( 'NONE', #28241 ) ;
#11129=CARTESIAN_POINT ( 'NONE',  ( 3.500000000000000000, 15.47927405783633503, -139.2380641367107330 ) ) ;
#11130=( BOUNDED_CURVE ( )  B_SPLINE_CURVE ( 2, ( #2429, #37326, #21780, #25194, #1596, #34341, #4987, #21365, #8598 ),
 .UNSPECIFIED., .F., .F. ) 
 B_SPLINE_CURVE_WITH_KNOTS ( ( 3, 2, 2, 2, 3 ),
 ( 0.8312500000000000444, 0.8319444444444444864, 0.8333333333333333703, 0.8347222222222222543, 0.8354166666666666963 ),
 .UNSPECIFIED. ) 
 CURVE ( )  GEOMETRIC_REPRESENTATION_ITEM ( )  RATIONAL_B_SPLINE_CURVE ( ( 0.9330127018922194093, 0.9330127018922194093, 1.000000000000000000, 0.8660254037844387076, 1.000000000000000000, 0.8660254037844387076, 1.000000000000000000, 0.9330127018922194093, 0.9330127018922194093 ) ) 
 REPRESENTATION_ITEM ( '' )  );
#11131=CARTESIAN_POINT ( 'NONE',  ( 0.000000000000000000, 0.000000000000000000, 0.000000000000000000 ) ) ;
#11133=CARTESIAN_POINT ( 'NONE',  ( -3.500000000000000888, 19.52072594216372181, -132.0443141357548598 ) ) ;
#11134=CARTESIAN_POINT ( 'NONE',  ( -1.655278471875002211, 14.63297358603755072, -114.5974391362327935 ) ) ;
#11137=CARTESIAN_POINT ( 'NONE',  ( 3.500000000000001332, 17.50000000000001776, -87.46098080242151696 ) ) ;
#11139=CARTESIAN_POINT ( 'NONE',  ( -3.310556943750001313, 17.50000000000001421, -47.76410580289947205 ) ) ;
#11140=CARTESIAN_POINT ( 'NONE',  ( -3.310556943750001313, 17.50000000000002132, -105.8516058028994564 ) ) ;
#11141=CARTESIAN_POINT ( 'NONE',  ( 1.750000000000001110, 20.53108891324554719, -38.29431413575484555 ) ) ;
#11145=CARTESIAN_POINT ( 'NONE',  ( -1.655278471874999990, 20.36702641396249547, -127.0182724695661278 ) ) ;
#11148=DIRECTION ( 'NONE',  ( -0.000000000000000000, 1.259100132267607459E-16, -1.000000000000000000 ) ) ;
#11150=CARTESIAN_POINT ( 'NONE',  ( 3.310556943750001313, 17.50000000000001421, -61.35160580289945642 ) ) ;
#11151=ORIENTED_EDGE ( 'NONE', *, *, #9654, .F. ) ;
#11152=CARTESIAN_POINT ( 'NONE',  ( -3.310556943750001313, 17.50000000000001776, -81.85160580289945642 ) ) ;
#11155=CARTESIAN_POINT ( 'NONE',  ( 1.749999999999998224, 14.46891108675447413, -30.32139747004410069 ) ) ;
#11156=CARTESIAN_POINT ( 'NONE',  ( 3.500000000000000000, 15.47927405783632082, -44.54431413575483845 ) ) ;
#11157=EDGE_CURVE ( 'NONE', #23995, #2733, #19951, .T. ) ;
#11159=CARTESIAN_POINT ( 'NONE',  ( -1.655278471875002211, 14.63297358603754184, -41.59743913623280065 ) ) ;
#11160=CARTESIAN_POINT ( 'NONE',  ( -3.310556943750001313, 17.50000000000001776, -99.76410580289947916 ) ) ;
#11163=VERTEX_POINT ( 'NONE', #14269 ) ;
#11165=ADVANCED_FACE ( 'NONE', ( #11079 ), #33629, .T. ) ;
#11166=CARTESIAN_POINT ( 'NONE',  ( 2.340729813953370519E-16, 21.32270188528330834, -54.01410580289947916 ) ) ;
#11167=VERTEX_POINT ( 'NONE', #21272 ) ;
#11168=VERTEX_POINT ( 'NONE', #10866 ) ;
#11169=CARTESIAN_POINT ( 'NONE',  ( -1.394453263437886604E-15, 14.00000000000001776, -98.40473080337743284 ) ) ;
#11173=CYLINDRICAL_SURFACE ( 'NONE', #7513, 3.499999999999999556 ) ;
#11175=CARTESIAN_POINT ( 'NONE',  ( 3.500000000000001776, 19.52072594216370405, -36.37764746908816704 ) ) ;
#11177=DIRECTION ( 'NONE',  ( 0.000000000000000000, 1.000000000000000000, 0.000000000000000000 ) ) ;
#11180=CARTESIAN_POINT ( 'NONE',  ( -3.310556943750002645, 15.58864905735836537, -30.76827246956613848 ) ) ;
#11182=CARTESIAN_POINT ( 'NONE',  ( -3.310556943750000425, 19.41135094264167549, -134.8474391362328220 ) ) ;
#11186=CARTESIAN_POINT ( 'NONE',  ( -3.310556943750002645, 15.58864905735837780, -124.7682724695661136 ) ) ;
#11187=CARTESIAN_POINT ( 'NONE',  ( 1.749999999999998224, 14.46891108675447590, -42.62764746908817415 ) ) ;
#11188=CARTESIAN_POINT ( 'NONE',  ( -3.310556943750001313, 17.50000000000001776, -85.76410580289947916 ) ) ;
#11189=CARTESIAN_POINT ( 'NONE',  ( 1.749999999999998224, 14.46891108675447768, -65.32139747004410424 ) ) ;
#11190=CARTESIAN_POINT ( 'NONE',  ( -1.655278471874999990, 20.36702641396249902, -143.0182724695661420 ) ) ;
#11191=EDGE_CURVE ( 'NONE', #31753, #20208, #32975, .T. ) ;
#11192=CARTESIAN_POINT ( 'NONE',  ( -7.424026671074350129E-16, 13.45854811567263454, -69.40473080337743284 ) ) ;
#11193=CARTESIAN_POINT ( 'NONE',  ( 3.310556943750001313, 17.50000000000001421, -55.35160580289947063 ) ) ;
#11196=CARTESIAN_POINT ( 'NONE',  ( -1.749999999999999778, 20.53108891324555074, -49.12764746908818125 ) ) ;
#11197=CARTESIAN_POINT ( 'NONE',  ( 3.310556943749999981, 15.58864905735836714, -75.43493913623281344 ) ) ;
#11198=CARTESIAN_POINT ( 'NONE',  ( -7.022189441860112050E-16, 13.67729811471672896, -139.6016058028994564 ) ) ;
#11200=CARTESIAN_POINT ( 'NONE',  ( -3.310556943750000425, 19.41135094264166838, -104.8474391362328078 ) ) ;
#11201=CARTESIAN_POINT ( 'NONE',  ( -3.310556943750000425, 19.41135094264166483, -76.84743913623280775 ) ) ;
#11203=CARTESIAN_POINT ( 'NONE',  ( 2.340729813953370519E-16, 21.32270188528331190, -95.10160580289944221 ) ) ;
#11204=VECTOR ( 'NONE', #41258, 1000.000000000000227 ) ;
#11206=CARTESIAN_POINT ( 'NONE',  ( -0.9378221735089310451, 14.00000000000002132, -86.44938900211597854 ) ) ;
#11207=CARTESIAN_POINT ( 'NONE',  ( 1.749999999999998224, 14.46891108675447413, -26.62764746908817415 ) ) ;
#11209=CARTESIAN_POINT ( 'NONE',  ( -1.655278471875002211, 14.63297358603754361, -54.59743913623281486 ) ) ;
#11210=( BOUNDED_CURVE ( )  B_SPLINE_CURVE ( 2, ( #34314, #5377, #5178, #14960, #18150, #41327, #18566, #25167, #31535 ),
 .UNSPECIFIED., .F., .T. ) 
 B_SPLINE_CURVE_WITH_KNOTS ( ( 3, 2, 2, 2, 3 ),
 ( 0.7104166666666666963, 0.7111111111111111382, 0.7125000000000000222, 0.7138888888888889062, 0.7145833333333333481 ),
 .UNSPECIFIED. ) 
 CURVE ( )  GEOMETRIC_REPRESENTATION_ITEM ( )  RATIONAL_B_SPLINE_CURVE ( ( 0.9330127018922194093, 0.9330127018922194093, 1.000000000000000000, 0.8660254037844387076, 1.000000000000000000, 0.8660254037844387076, 1.000000000000000000, 0.9330127018922194093, 0.9330127018922194093 ) ) 
 REPRESENTATION_ITEM ( '' )  );
#11212=CARTESIAN_POINT ( 'NONE',  ( 1.655278471874998436, 14.63297358603754894, -116.4307724695661364 ) ) ;
#11215=ORIENTED_EDGE ( 'NONE', *, *, #9534, .T. ) ;
#11218=EDGE_CURVE ( 'NONE', #38312, #26191, #37339, .T. ) ;
#11219=CARTESIAN_POINT ( 'NONE',  ( 1.655278471875001101, 20.36702641396248836, -69.09743913623280775 ) ) ;
#11221=ORIENTED_EDGE ( 'NONE', *, *, #40184, .T. ) ;
#11228=CARTESIAN_POINT ( 'NONE',  ( 1.655278471875001101, 20.36702641396249902, -136.0974391362328220 ) ) ;
#11229=CARTESIAN_POINT ( 'NONE',  ( -3.310556943750001313, 17.50000000000001066, -46.85160580289945642 ) ) ;
#11230=CARTESIAN_POINT ( 'NONE',  ( 3.310556943750001313, 19.41135094264165772, -34.26827246956613493 ) ) ;
#11231=CARTESIAN_POINT ( 'NONE',  ( 3.310556943750001313, 17.50000000000001776, -100.3516058028994706 ) ) ;
#11233=CARTESIAN_POINT ( 'NONE',  ( 3.310556943750001313, 19.41135094264167549, -141.2682724695661420 ) ) ;
#11235=CYLINDRICAL_SURFACE ( 'NONE', #10810, 3.499999999999999556 ) ;
#11236=CARTESIAN_POINT ( 'NONE',  ( -1.749999999999999778, 20.53108891324555429, -96.12764746908817415 ) ) ;
#11238=CARTESIAN_POINT ( 'NONE',  ( 0.9378221735089300459, 21.00000000000001421, -64.25563900116002003 ) ) ;
#11239=CARTESIAN_POINT ( 'NONE',  ( -3.500000000000000888, 19.52072594216371115, -83.73806413671076143 ) ) ;
#11240=CARTESIAN_POINT ( 'NONE',  ( 1.655278471874998436, 14.63297358603754361, -72.51827246956612782 ) ) ;
#11244=CARTESIAN_POINT ( 'NONE',  ( -0.9378221735089291577, 21.00000000000002132, -120.1663226036829855 ) ) ;
#11245=CARTESIAN_POINT ( 'NONE',  ( -3.500000000000001332, 17.50000000000001066, -46.96098080242150274 ) ) ;
#11246=CARTESIAN_POINT ( 'NONE',  ( 3.310556943749999981, 15.58864905735837247, -121.3474391362328078 ) ) ;
#11249=ORIENTED_EDGE ( 'NONE', *, *, #25593, .F. ) ;
#11250=CARTESIAN_POINT ( 'NONE',  ( 1.750000000000001110, 20.53108891324555785, -113.9880641367107472 ) ) ;
#11252=CARTESIAN_POINT ( 'NONE',  ( -1.750000000000002220, 14.46891108675448301, -83.48806413671076143 ) ) ;
#11253=CYLINDRICAL_SURFACE ( 'NONE', #28497, 3.499999999999999556 ) ;
#11256=CARTESIAN_POINT ( 'NONE',  ( 1.655278471874998436, 14.63297358603754361, -75.43077246956613635 ) ) ;
#11257=( BOUNDED_CURVE ( )  B_SPLINE_CURVE ( 2, ( #1636, #34169, #1227, #40139, #36962, #14197, #8222, #14619, #21199 ),
 .UNSPECIFIED., .F., .F. ) 
 B_SPLINE_CURVE_WITH_KNOTS ( ( 3, 2, 2, 2, 3 ),
 ( 0.9145833333333333037, 0.9152777777777777457, 0.9166666666666666297, 0.9180555555555555136, 0.9187499999999999556 ),
 .UNSPECIFIED. ) 
 CURVE ( )  GEOMETRIC_REPRESENTATION_ITEM ( )  RATIONAL_B_SPLINE_CURVE ( ( 0.9330127018922194093, 0.9330127018922194093, 1.000000000000000000, 0.8660254037844387076, 1.000000000000000000, 0.8660254037844387076, 1.000000000000000000, 0.9330127018922194093, 0.9330127018922194093 ) ) 
 REPRESENTATION_ITEM ( '' )  );
#11258=CARTESIAN_POINT ( 'NONE',  ( 0.9378221735089300459, 21.00000000000001421, -72.25563900116002003 ) ) ;
#11259=ORIENTED_EDGE ( 'NONE', *, *, #9221, .F. ) ;
#11261=CARTESIAN_POINT ( 'NONE',  ( 3.310556943750001313, 19.41135094264166483, -87.18077246956613635 ) ) ;
#11263=ORIENTED_EDGE ( 'NONE', *, *, #41198, .T. ) ;
#11264=VECTOR ( 'NONE', #41295, 1000.000000000000000 ) ;
#11267=DIRECTION ( 'NONE',  ( 0.000000000000000000, 1.000000000000000000, 0.000000000000000000 ) ) ;
#11270=CARTESIAN_POINT ( 'NONE',  ( 3.310556943749999981, 15.58864905735836182, -46.43493913623279212 ) ) ;
#11271=CARTESIAN_POINT ( 'NONE',  ( -1.655278471874999990, 20.36702641396249547, -113.0182724695661278 ) ) ;
#11272=EDGE_LOOP ( 'NONE', ( #33496, #22970, #17397, #33445 ) ) ;
#11273=CARTESIAN_POINT ( 'NONE',  ( -7.424026671074350129E-16, 13.45854811567263987, -122.4047308033774328 ) ) ;
#11274=CARTESIAN_POINT ( 'NONE',  ( -3.310556943750000425, 19.41135094264165772, -38.84743913623281486 ) ) ;
#11275=CARTESIAN_POINT ( 'NONE',  ( 2.340729813953370519E-16, 21.32270188528330834, -64.10160580289945642 ) ) ;
#11276=CARTESIAN_POINT ( 'NONE',  ( 3.500000000000001776, 19.52072594216371826, -111.3776474690881599 ) ) ;
#11278=CARTESIAN_POINT ( 'NONE',  ( 1.655278471874998436, 14.63297358603754716, -95.43077246956613635 ) ) ;
#11279=CARTESIAN_POINT ( 'NONE',  ( 3.500000000000001332, 19.52072594216370760, -60.07139747004409713 ) ) ;
#11280=CARTESIAN_POINT ( 'NONE',  ( 4.648177544792955347E-16, 21.00000000000001066, -26.21098080242150985 ) ) ;
#11283=CARTESIAN_POINT ( 'NONE',  ( -3.500000000000001332, 17.50000000000001421, -61.96098080242150274 ) ) ;
#11284=CARTESIAN_POINT ( 'NONE',  ( 2.340729813953370519E-16, 21.32270188528330479, -32.01410580289947205 ) ) ;
#11285=CARTESIAN_POINT ( 'NONE',  ( 1.655278471874998436, 14.63297358603754539, -89.51827246956612782 ) ) ;
#11286=CARTESIAN_POINT ( 'NONE',  ( 3.500000000000001776, 19.52072594216370760, -56.07139747004409003 ) ) ;
#11288=CARTESIAN_POINT ( 'NONE',  ( -1.655278471874999990, 20.36702641396249547, -112.0182724695661420 ) ) ;
#11289=CARTESIAN_POINT ( 'NONE',  ( 1.655278471874998436, 14.63297358603753828, -37.51827246956612782 ) ) ;
#11297=CARTESIAN_POINT ( 'NONE',  ( -3.310556943750002201, 15.58864905735837247, -93.68077246956613635 ) ) ;
#11298=CARTESIAN_POINT ( 'NONE',  ( 4.648177544792955347E-16, 21.00000000000001776, -81.90473080337743284 ) ) ;
#11302=ADVANCED_FACE ( 'NONE', ( #1092 ), #14063, .T. ) ;
#11304=CARTESIAN_POINT ( 'NONE',  ( 0.9378221735089300459, 21.00000000000001066, -46.25563900116002714 ) ) ;
#11305=VERTEX_POINT ( 'NONE', #31830 ) ;
#11309=CARTESIAN_POINT ( 'NONE',  ( -1.394453263437886604E-15, 14.00000000000001066, -34.71098080242151696 ) ) ;
#11319=CARTESIAN_POINT ( 'NONE',  ( -7.022189441860112050E-16, 13.67729811471672896, -139.5141058028994507 ) ) ;
#11320=CYLINDRICAL_SURFACE ( 'NONE', #4040, 3.499999999999999556 ) ;
#11321=CARTESIAN_POINT ( 'NONE',  ( 3.500000000000000000, 15.47927405783632970, -101.5443141357548456 ) ) ;
#11322=CARTESIAN_POINT ( 'NONE',  ( 1.655278471875001101, 20.36702641396249902, -131.1849391362327992 ) ) ;
#11323=CARTESIAN_POINT ( 'NONE',  ( -3.310556943750002645, 15.58864905735836892, -55.76827246956613493 ) ) ;
#11326=FACE_OUTER_BOUND ( 'NONE', #24666, .T. ) ;
#11329=CARTESIAN_POINT ( 'NONE',  ( -1.750000000000002220, 14.46891108675448834, -126.7943141357548456 ) ) ;
#11330=CARTESIAN_POINT ( 'NONE',  ( 3.310556943750001313, 17.50000000000002132, -115.2641058028994792 ) ) ;
#11333=CARTESIAN_POINT ( 'NONE',  ( -3.500000000000002220, 15.47927405783632793, -82.87764746908818836 ) ) ;
#11334=LINE ( 'NONE', #33464, #18504 ) ;
#11335=CARTESIAN_POINT ( 'NONE',  ( -3.310556943750002645, 15.58864905735836714, -46.68077246956614346 ) ) ;
#11336=CARTESIAN_POINT ( 'NONE',  ( -3.310556943750001313, 17.50000000000002132, -107.8516058028994564 ) ) ;
#11341=CARTESIAN_POINT ( 'NONE',  ( 3.310556943749999981, 15.58864905735837425, -129.4349391362327992 ) ) ;
#11344=CARTESIAN_POINT ( 'NONE',  ( -0.9378221735089291577, 21.00000000000002132, -117.1663226036829997 ) ) ;
#11345=CARTESIAN_POINT ( 'NONE',  ( 1.750000000000001110, 20.53108891324555429, -85.98806413671076143 ) ) ;
#11346=ADVANCED_FACE ( 'NONE', ( #35033 ), #35237, .T. ) ;
#11347=CARTESIAN_POINT ( 'NONE',  ( 3.310556943750001313, 19.41135094264166128, -60.26827246956613493 ) ) ;
#11350=CARTESIAN_POINT ( 'NONE',  ( -1.655278471875002211, 14.63297358603754539, -78.68493913623279923 ) ) ;
#11354=CARTESIAN_POINT ( 'NONE',  ( 4.648177544792955347E-16, 21.00000000000001066, -25.90473080337743284 ) ) ;
#11355=CARTESIAN_POINT ( 'NONE',  ( 0.000000000000000000, 21.00000000000002487, -149.5231586289125687 ) ) ;
#11357=CARTESIAN_POINT ( 'NONE',  ( -3.310556943750001313, 17.50000000000001066, -40.76410580289947916 ) ) ;
#11359=CARTESIAN_POINT ( 'NONE',  ( 2.340729813953370519E-16, 21.32270188528331190, -94.01410580289947916 ) ) ;
#11360=CARTESIAN_POINT ( 'NONE',  ( -3.500000000000002220, 15.47927405783632970, -93.57139747004410424 ) ) ;
#11364=CARTESIAN_POINT ( 'NONE',  ( -3.310556943750001313, 17.50000000000001066, -45.76410580289946495 ) ) ;
#11365=VERTEX_POINT ( 'NONE', #39056 ) ;
#11370=( BOUNDED_CURVE ( )  B_SPLINE_CURVE ( 2, ( #574, #9958, #3551, #39491, #30133, #19721, #12928, #10580, #20148 ),
 .UNSPECIFIED., .F., .F. ) 
 B_SPLINE_CURVE_WITH_KNOTS ( ( 3, 2, 2, 2, 3 ),
 ( 0.3937499999999999889, 0.3944444444444444309, 0.3958333333333333148, 0.3972222222222221988, 0.3979166666666666963 ),
 .UNSPECIFIED. ) 
 CURVE ( )  GEOMETRIC_REPRESENTATION_ITEM ( )  RATIONAL_B_SPLINE_CURVE ( ( 0.9330127018922194093, 0.9330127018922194093, 1.000000000000000000, 0.8660254037844387076, 1.000000000000000000, 0.8660254037844387076, 1.000000000000000000, 0.9330127018922167448, 0.9330127018922194093 ) ) 
 REPRESENTATION_ITEM ( '' )  );
#11372=VERTEX_POINT ( 'NONE', #32046 ) ;
#11373=CARTESIAN_POINT ( 'NONE',  ( 0.000000000000000000, 17.50000000000002487, -149.5231586289125687 ) ) ;
#11374=CARTESIAN_POINT ( 'NONE',  ( 1.750000000000001110, 20.53108891324554719, -39.29431413575484555 ) ) ;
#11375=LINE ( 'NONE', #37530, #18021 ) ;
#11376=CARTESIAN_POINT ( 'NONE',  ( 0.9378221735089128375, 21.00000000000003553, -125.2556390011600485 ) ) ;
#11379=CARTESIAN_POINT ( 'NONE',  ( -7.022189441860112050E-16, 13.67729811471671297, -23.60160580289946353 ) ) ;
#11380=EDGE_CURVE ( 'NONE', #22963, #3824, #12619, .T. ) ;
#11381=CARTESIAN_POINT ( 'NONE',  ( -0.9378221735089310451, 14.00000000000001599, -59.44938900211595012 ) ) ;
#11382=CARTESIAN_POINT ( 'NONE',  ( -3.310556943750001313, 17.50000000000002487, -130.7641058028994507 ) ) ;
#11385=CARTESIAN_POINT ( 'NONE',  ( 1.655278471875001101, 20.36702641396249547, -122.1849391362327992 ) ) ;
#11386=CARTESIAN_POINT ( 'NONE',  ( 0.000000000000000000, 21.00000000000002487, -149.5231586289125687 ) ) ;
#11387=CARTESIAN_POINT ( 'NONE',  ( -3.500000000000001332, 17.50000000000001066, -36.65473080337743284 ) ) ;
#11389=CARTESIAN_POINT ( 'NONE',  ( 2.340729813953370519E-16, 21.32270188528332255, -142.1016058028994564 ) ) ;
#11390=CARTESIAN_POINT ( 'NONE',  ( 2.474675557024783212E-16, 21.54145188432739388, -67.90473080337743284 ) ) ;
#11392=CARTESIAN_POINT ( 'NONE',  ( -3.310556943750002201, 15.58864905735836714, -51.76827246956612072 ) ) ;
#11395=CARTESIAN_POINT ( 'NONE',  ( -3.310556943750002645, 15.58864905735837070, -75.76827246956612782 ) ) ;
#11397=CARTESIAN_POINT ( 'NONE',  ( -3.310556943750000425, 19.41135094264166838, -101.8474391362328078 ) ) ;
#11398=CARTESIAN_POINT ( 'NONE',  ( -1.655278471875002211, 14.63297358603754539, -76.59743913623280775 ) ) ;
#11399=ORIENTED_EDGE ( 'NONE', *, *, #30553, .T. ) ;
#11400=CARTESIAN_POINT ( 'NONE',  ( -1.655278471874999990, 20.36702641396249192, -94.01827246956612782 ) ) ;
#11403=CARTESIAN_POINT ( 'NONE',  ( -1.750000000000002220, 14.46891108675447768, -51.79431413575484555 ) ) ;
#11405=CARTESIAN_POINT ( 'NONE',  ( 2.340729813953370519E-16, 21.32270188528331190, -55.01410580289947205 ) ) ;
#11406=CARTESIAN_POINT ( 'NONE',  ( -1.394453263437886604E-15, 14.00000000000002132, -112.7109808024214885 ) ) ;
#11407=CARTESIAN_POINT ( 'NONE',  ( -3.310556943750002645, 15.58864905735837780, -111.6807724695661506 ) ) ;
#11412=DIRECTION ( 'NONE',  ( -0.000000000000000000, 1.259100132267607459E-16, -1.000000000000000000 ) ) ;
#11413=CARTESIAN_POINT ( 'NONE',  ( 3.310556943750001313, 17.50000000000001421, -71.26410580289947916 ) ) ;
#11416=CARTESIAN_POINT ( 'NONE',  ( -1.394453263437886604E-15, 14.00000000000001066, -48.71098080242150274 ) ) ;
#11422=CARTESIAN_POINT ( 'NONE',  ( 1.655278471874998436, 14.63297358603755072, -129.4307724695661364 ) ) ;
#11424=CARTESIAN_POINT ( 'NONE',  ( -7.022189441860112050E-16, 13.67729811471671653, -45.60160580289945642 ) ) ;
#11425=CARTESIAN_POINT ( 'NONE',  ( -3.310556943750002645, 15.58864905735836537, -34.76827246956614204 ) ) ;
#11426=CARTESIAN_POINT ( 'NONE',  ( -1.655278471875002211, 14.63297358603754716, -93.68493913623279923 ) ) ;
#11427=CARTESIAN_POINT ( 'NONE',  ( 3.310556943750001313, 19.41135094264167549, -142.1807724695661364 ) ) ;
#11429=CARTESIAN_POINT ( 'NONE',  ( 3.310556943749999981, 15.58864905735837780, -139.4349391362327708 ) ) ;
#11430=CARTESIAN_POINT ( 'NONE',  ( 3.500000000000000000, 15.47927405783633326, -121.5443141357548456 ) ) ;
#11431=CARTESIAN_POINT ( 'NONE',  ( 3.500000000000001776, 19.52072594216371115, -97.37764746908817415 ) ) ;
#11432=DIRECTION ( 'NONE',  ( -0.000000000000000000, 1.259100132267607459E-16, -1.000000000000000000 ) ) ;
#11433=CARTESIAN_POINT ( 'NONE',  ( 2.474675557024783212E-16, 21.54145188432739744, -85.90473080337743284 ) ) ;
#11435=CARTESIAN_POINT ( 'NONE',  ( -3.310556943750002201, 15.58864905735837070, -71.76827246956612782 ) ) ;
#11436=( BOUNDED_CURVE ( )  B_SPLINE_CURVE ( 2, ( #19313, #28665, #35694, #6556, #22087, #41657, #35891, #32493, #39083 ),
 .UNSPECIFIED., .F., .T. ) 
 B_SPLINE_CURVE_WITH_KNOTS ( ( 3, 2, 2, 2, 3 ),
 ( 0.1437499999999999889, 0.1444444444444444309, 0.1458333333333333426, 0.1472222222222222265, 0.1479166666666666685 ),
 .UNSPECIFIED. ) 
 CURVE ( )  GEOMETRIC_REPRESENTATION_ITEM ( )  RATIONAL_B_SPLINE_CURVE ( ( 0.9330127018922194093, 0.9330127018922194093, 1.000000000000000000, 0.8660254037844387076, 1.000000000000000000, 0.8660254037844387076, 1.000000000000000000, 0.9330127018922194093, 0.9330127018922194093 ) ) 
 REPRESENTATION_ITEM ( '' )  );
#11441=CARTESIAN_POINT ( 'NONE',  ( -1.750000000000002220, 14.46891108675447768, -50.79431413575484555 ) ) ;
#11443=CARTESIAN_POINT ( 'NONE',  ( 2.340729813953370519E-16, 21.32270188528331900, -118.0141058028994792 ) ) ;
#11445=CARTESIAN_POINT ( 'NONE',  ( -7.460324959392693302E-14, 21.00000000000002132, -103.2109808024215027 ) ) ;
#11446=ORIENTED_EDGE ( 'NONE', *, *, #18638, .T. ) ;
#11447=CARTESIAN_POINT ( 'NONE',  ( -3.500000000000001332, 17.50000000000002132, -112.6547308033774328 ) ) ;
#11448=CARTESIAN_POINT ( 'NONE',  ( 0.9378221735089300459, 21.00000000000001421, -54.94938900211595723 ) ) ;
#11449=DIRECTION ( 'NONE',  ( -0.000000000000000000, 1.259100132267607459E-16, -1.000000000000000000 ) ) ;
#11453=CARTESIAN_POINT ( 'NONE',  ( -3.310556943750001313, 17.50000000000001421, -73.76410580289947916 ) ) ;
#11457=CARTESIAN_POINT ( 'NONE',  ( 4.286263797015737581E-16, 14.00000000000002487, -149.5231586289125687 ) ) ;
#11458=CARTESIAN_POINT ( 'NONE',  ( -1.394453263437886604E-15, 14.00000000000000711, -25.71098080242150630 ) ) ;
#11459=CARTESIAN_POINT ( 'NONE',  ( 3.310556943749999981, 15.58864905735836892, -85.34743913623279354 ) ) ;
#11460=VERTEX_POINT ( 'NONE', #30113 ) ;
#11463=ADVANCED_FACE ( 'NONE', ( #3955 ), #16935, .T. ) ;
#11466=VECTOR ( 'NONE', #30586, 1000.000000000000000 ) ;
#11467=EDGE_LOOP ( 'NONE', ( #4929, #23945, #36526, #31980 ) ) ;
#11468=CARTESIAN_POINT ( 'NONE',  ( 0.000000000000000000, 21.00000000000002487, -149.5231586289125687 ) ) ;
#11469=CARTESIAN_POINT ( 'NONE',  ( -3.310556943750001313, 17.50000000000001421, -49.85160580289946353 ) ) ;
#11470=CARTESIAN_POINT ( 'NONE',  ( -1.655278471875002211, 14.63297358603754894, -106.6849391362327992 ) ) ;
#11472=CARTESIAN_POINT ( 'NONE',  ( 3.310556943750001313, 17.50000000000001066, -34.26410580289947205 ) ) ;
#11473=CARTESIAN_POINT ( 'NONE',  ( -3.310556943750002645, 15.58864905735836892, -66.76827246956612782 ) ) ;
#11474=CARTESIAN_POINT ( 'NONE',  ( 3.500000000000000000, 15.47927405783632970, -111.5443141357548456 ) ) ;
#11476=CARTESIAN_POINT ( 'NONE',  ( 3.310556943750001313, 17.50000000000001776, -99.26410580289947916 ) ) ;
#11478=ADVANCED_FACE ( 'NONE', ( #20766 ), #773, .T. ) ;
#11479=CARTESIAN_POINT ( 'NONE',  ( -1.394453263437886604E-15, 14.00000000000002132, -124.4047308033774044 ) ) ;
#11480=CARTESIAN_POINT ( 'NONE',  ( 1.749999999999998224, 14.46891108675448656, -124.6276474690881599 ) ) ;
#11482=CARTESIAN_POINT ( 'NONE',  ( -3.500000000000002220, 15.47927405783632437, -61.87764746908817415 ) ) ;
#11484=CARTESIAN_POINT ( 'NONE',  ( 1.655278471875001101, 20.36702641396248481, -33.09743913623280775 ) ) ;
#11485=( BOUNDED_CURVE ( )  B_SPLINE_CURVE ( 2, ( #39004, #6473, #9451, #29006, #32207, #35396, #16065, #22419, #498 ),
 .UNSPECIFIED., .F., .T. ) 
 B_SPLINE_CURVE_WITH_KNOTS ( ( 3, 2, 2, 2, 3 ),
 ( 0.9145833333333333037, 0.9152777777777777457, 0.9166666666666666297, 0.9180555555555555136, 0.9187499999999999556 ),
 .UNSPECIFIED. ) 
 CURVE ( )  GEOMETRIC_REPRESENTATION_ITEM ( )  RATIONAL_B_SPLINE_CURVE ( ( 0.9330127018922194093, 0.9330127018922194093, 1.000000000000000000, 0.8660254037844387076, 1.000000000000000000, 0.8660254037844387076, 1.000000000000000000, 0.9330127018922194093, 0.9330127018922194093 ) ) 
 REPRESENTATION_ITEM ( '' )  );
#11486=EDGE_CURVE ( 'NONE', #11365, #35484, #32879, .T. ) ;
#11487=CARTESIAN_POINT ( 'NONE',  ( -1.655278471875002211, 14.63297358603754716, -88.68493913623279923 ) ) ;
#11488=CARTESIAN_POINT ( 'NONE',  ( 3.500000000000001776, 19.52072594216370760, -52.07139747004409003 ) ) ;
#11489=CARTESIAN_POINT ( 'NONE',  ( -1.655278471875002211, 14.63297358603754894, -104.6849391362327992 ) ) ;
#11490=CARTESIAN_POINT ( 'NONE',  ( 1.655278471875001101, 20.36702641396248481, -38.18493913623280633 ) ) ;
#11496=CARTESIAN_POINT ( 'NONE',  ( -1.655278471875002211, 14.63297358603754716, -87.59743913623280775 ) ) ;
#11500=EDGE_LOOP ( 'NONE', ( #23071, #21854, #22373, #23136 ) ) ;
#11502=CARTESIAN_POINT ( 'NONE',  ( 1.749999999999998224, 14.46891108675448478, -109.6276474690881741 ) ) ;
#11503=VERTEX_POINT ( 'NONE', #10976 ) ;
#11512=LINE ( 'NONE', #25130, #28541 ) ;
#11517=DIRECTION ( 'NONE',  ( -0.000000000000000000, 1.259100132267607459E-16, -1.000000000000000000 ) ) ;
#11518=CARTESIAN_POINT ( 'NONE',  ( 1.655278471874998436, 14.63297358603755249, -136.4307724695661364 ) ) ;
#11519=CARTESIAN_POINT ( 'NONE',  ( 0.9378221735089281585, 14.00000000000000888, -38.36007260463890844 ) ) ;
#11521=CARTESIAN_POINT ( 'NONE',  ( 1.655278471875001101, 20.36702641396249547, -128.1849391362327992 ) ) ;
#11522=CARTESIAN_POINT ( 'NONE',  ( 1.655278471875001101, 20.36702641396248836, -58.18493913623279212 ) ) ;
#11524=EDGE_CURVE ( 'NONE', #9419, #14300, #9123, .T. ) ;
#11526=CARTESIAN_POINT ( 'NONE',  ( -3.500000000000002220, 15.47927405783633503, -134.5713974700441042 ) ) ;
#11529=CARTESIAN_POINT ( 'NONE',  ( 3.500000000000001332, 17.50000000000002487, -130.4609808024214885 ) ) ;
#11530=CARTESIAN_POINT ( 'NONE',  ( -1.655278471875002211, 14.63297358603755072, -113.5974391362328078 ) ) ;
#11534=CARTESIAN_POINT ( 'NONE',  ( -1.750000000000002220, 14.46891108675448123, -78.79431413575484555 ) ) ;
#11536=CARTESIAN_POINT ( 'NONE',  ( 2.340729813953370519E-16, 21.32270188528330834, -50.01410580289947205 ) ) ;
#11538=CARTESIAN_POINT ( 'NONE',  ( 3.310556943749999981, 15.58864905735837070, -105.4349391362327850 ) ) ;
#11539=CARTESIAN_POINT ( 'NONE',  ( 4.286263797015737581E-16, 14.00000000000002487, -149.5231586289125687 ) ) ;
#11541=CARTESIAN_POINT ( 'NONE',  ( -3.500000000000001332, 17.50000000000001421, -72.65473080337743284 ) ) ;
#11542=CARTESIAN_POINT ( 'NONE',  ( -3.310556943750002201, 15.58864905735837780, -120.7682724695661278 ) ) ;
#11545=CARTESIAN_POINT ( 'NONE',  ( 3.500000000000001332, 17.50000000000002132, -124.1547308033774186 ) ) ;
#11546=CARTESIAN_POINT ( 'NONE',  ( -1.655278471874999990, 20.36702641396248836, -58.01827246956613493 ) ) ;
#11548=VERTEX_POINT ( 'NONE', #16729 ) ;
#11549=CARTESIAN_POINT ( 'NONE',  ( 1.655278471874998436, 14.63297358603754539, -82.51827246956614204 ) ) ;
#11550=EDGE_CURVE ( 'NONE', #10596, #18958, #10345, .T. ) ;
#11551=FACE_OUTER_BOUND ( 'NONE', #11500, .T. ) ;
#11552=CARTESIAN_POINT ( 'NONE',  ( 1.750000000000001110, 20.53108891324555429, -76.98806413671076143 ) ) ;
#11553=CARTESIAN_POINT ( 'NONE',  ( 4.648177544792955347E-16, 21.00000000000001776, -98.90473080337744705 ) ) ;
#11556=CARTESIAN_POINT ( 'NONE',  ( 1.655278471874998436, 14.63297358603753828, -38.43077246956613635 ) ) ;
#11562=CARTESIAN_POINT ( 'NONE',  ( 2.340729813953370519E-16, 21.32270188528330479, -46.01410580289946495 ) ) ;
#11564=ORIENTED_EDGE ( 'NONE', *, *, #19328, .T. ) ;
#11566=AXIS2_PLACEMENT_3D ( 'NONE', #15890, #2478, #28418 ) ;
#11567=CARTESIAN_POINT ( 'NONE',  ( -7.424026671074350129E-16, 13.45854811567263098, -23.71098080242150985 ) ) ;
#11569=CARTESIAN_POINT ( 'NONE',  ( 4.648177544792955347E-16, 21.00000000000002132, -112.9047308033774186 ) ) ;
#11571=CARTESIAN_POINT ( 'NONE',  ( -2.324088772396477673E-16, 14.00000000000002309, -142.7109808024215170 ) ) ;
#11572=CARTESIAN_POINT ( 'NONE',  ( 3.500000000000000000, 15.47927405783632082, -40.54431413575484555 ) ) ;
#11574=CARTESIAN_POINT ( 'NONE',  ( 0.9378221735089300459, 21.00000000000001421, -70.25563900116006266 ) ) ;
#11577=CARTESIAN_POINT ( 'NONE',  ( 3.310556943750001313, 19.41135094264165772, -24.26827246956612782 ) ) ;
#11578=CARTESIAN_POINT ( 'NONE',  ( -3.500000000000001332, 17.50000000000001421, -59.65473080337743994 ) ) ;
#11579=CARTESIAN_POINT ( 'NONE',  ( 3.310556943750001313, 17.50000000000002132, -129.2641058028994507 ) ) ;
#11582=CARTESIAN_POINT ( 'NONE',  ( 0.000000000000000000, 17.50000000000002487, -149.5231586289125687 ) ) ;
#11584=CARTESIAN_POINT ( 'NONE',  ( -1.655278471875002211, 14.63297358603755249, -123.6849391362327992 ) ) ;
#11585=DIRECTION ( 'NONE',  ( -0.000000000000000000, 1.259100132267607459E-16, -1.000000000000000000 ) ) ;
#11586=CARTESIAN_POINT ( 'NONE',  ( -3.500000000000002220, 15.47927405783632082, -37.57139747004409713 ) ) ;
#11588=CARTESIAN_POINT ( 'NONE',  ( 0.9378221735089281585, 14.00000000000002309, -130.6663226036829712 ) ) ;
#11589=CARTESIAN_POINT ( 'NONE',  ( 0.9378221735089281585, 14.00000000000001776, -89.36007260463888713 ) ) ;
#11590=CARTESIAN_POINT ( 'NONE',  ( -3.500000000000000888, 19.52072594216370760, -67.73806413671076143 ) ) ;
#11592=CARTESIAN_POINT ( 'NONE',  ( 3.310556943750001313, 19.41135094264166483, -53.26827246956613493 ) ) ;
#11594=CARTESIAN_POINT ( 'NONE',  ( -1.394453263437886604E-15, 14.00000000000001066, -41.40473080337741862 ) ) ;
#11595=CARTESIAN_POINT ( 'NONE',  ( 2.340729813953370519E-16, 21.32270188528330834, -73.10160580289948484 ) ) ;
#11597=CARTESIAN_POINT ( 'NONE',  ( 2.340729813953370519E-16, 21.32270188528331900, -105.0141058028994649 ) ) ;
#11598=CARTESIAN_POINT ( 'NONE',  ( 2.340729813953370519E-16, 21.32270188528330834, -70.01410580289947916 ) ) ;
#11601=CARTESIAN_POINT ( 'NONE',  ( -3.310556943750001313, 17.50000000000001776, -97.85160580289945642 ) ) ;
#11603=CARTESIAN_POINT ( 'NONE',  ( -1.394453263437886604E-15, 14.00000000000001066, -32.71098080242150274 ) ) ;
#11604=CARTESIAN_POINT ( 'NONE',  ( 4.648177544792955347E-16, 21.00000000000001421, -50.90473080337743284 ) ) ;
#11606=CARTESIAN_POINT ( 'NONE',  ( 3.310556943749999981, 15.58864905735836537, -54.34743913623282907 ) ) ;
#11608=CARTESIAN_POINT ( 'NONE',  ( -3.310556943750002645, 15.58864905735837780, -109.6807724695661364 ) ) ;
#11609=( BOUNDED_CURVE ( )  B_SPLINE_CURVE ( 2, ( #23529, #23310, #20323, #978, #545, #36699, #4375, #13948, #16926 ),
 .UNSPECIFIED., .F., .T. ) 
 B_SPLINE_CURVE_WITH_KNOTS ( ( 3, 2, 2, 2, 3 ),
 ( 0.3770833333333333259, 0.3777777777777777679, 0.3791666666666666519, 0.3805555555555555358, 0.3812499999999999778 ),
 .UNSPECIFIED. ) 
 CURVE ( )  GEOMETRIC_REPRESENTATION_ITEM ( )  RATIONAL_B_SPLINE_CURVE ( ( 0.9330127018922194093, 0.9330127018922194093, 1.000000000000000000, 0.8660254037844387076, 1.000000000000000000, 0.8660254037844387076, 1.000000000000000000, 0.9330127018922194093, 0.9330127018922194093 ) ) 
 REPRESENTATION_ITEM ( '' )  );
#11610=ORIENTED_EDGE ( 'NONE', *, *, #30018, .F. ) ;
#11611=( BOUNDED_CURVE ( )  B_SPLINE_CURVE ( 2, ( #3517, #16922, #35437, #33074, #6297, #29674, #539, #16508, #3940 ),
 .UNSPECIFIED., .F., .T. ) 
 B_SPLINE_CURVE_WITH_KNOTS ( ( 3, 2, 2, 2, 3 ),
 ( 0.8979166666666666963, 0.8986111111111111382, 0.9000000000000000222, 0.9013888888888889062, 0.9020833333333333481 ),
 .UNSPECIFIED. ) 
 CURVE ( )  GEOMETRIC_REPRESENTATION_ITEM ( )  RATIONAL_B_SPLINE_CURVE ( ( 0.9330127018922194093, 0.9330127018922194093, 1.000000000000000000, 0.8660254037844387076, 1.000000000000000000, 0.8660254037844387076, 1.000000000000000000, 0.9330127018922194093, 0.9330127018922194093 ) ) 
 REPRESENTATION_ITEM ( '' )  );
#11615=EDGE_LOOP ( 'NONE', ( #34890, #27738, #40566, #959 ) ) ;
#11616=CARTESIAN_POINT ( 'NONE',  ( -0.9378221735089310451, 14.00000000000002309, -109.7556390011600342 ) ) ;
#11617=CARTESIAN_POINT ( 'NONE',  ( 1.655278471874998436, 14.63297358603754184, -65.43077246956615056 ) ) ;
#11618=ORIENTED_EDGE ( 'NONE', *, *, #12052, .T. ) ;
#11619=ORIENTED_EDGE ( 'NONE', *, *, #5096, .T. ) ;
#11623=CARTESIAN_POINT ( 'NONE',  ( 0.000000000000000000, 21.00000000000002487, -149.5231586289125687 ) ) ;
#11624=ORIENTED_EDGE ( 'NONE', *, *, #39042, .T. ) ;
#11625=DIRECTION ( 'NONE',  ( 0.000000000000000000, 1.000000000000000000, 0.000000000000000000 ) ) ;
#11626=CARTESIAN_POINT ( 'NONE',  ( -1.655278471875002211, 14.63297358603755249, -131.5974391362328220 ) ) ;
#11627=CARTESIAN_POINT ( 'NONE',  ( -0.9378221735089291577, 21.00000000000002132, -116.1663226036829997 ) ) ;
#11630=CARTESIAN_POINT ( 'NONE',  ( 3.310556943750001313, 17.50000000000001066, -42.35160580289947063 ) ) ;
#11631=CARTESIAN_POINT ( 'NONE',  ( -3.310556943750001313, 17.50000000000001776, -95.85160580289945642 ) ) ;
#11632=CARTESIAN_POINT ( 'NONE',  ( -1.749999999999999778, 20.53108891324554719, -23.82139747004409358 ) ) ;
#11633=ORIENTED_EDGE ( 'NONE', *, *, #41785, .F. ) ;
#11635=CARTESIAN_POINT ( 'NONE',  ( 2.340729813953370519E-16, 21.32270188528332255, -139.1016058028994564 ) ) ;
#11637=CARTESIAN_POINT ( 'NONE',  ( -1.750000000000002220, 14.46891108675448478, -98.79431413575484555 ) ) ;
#11638=CARTESIAN_POINT ( 'NONE',  ( -3.500000000000002220, 15.47927405783632793, -73.57139747004410424 ) ) ;
#11639=CARTESIAN_POINT ( 'NONE',  ( -3.310556943750000425, 19.41135094264166128, -59.84743913623280775 ) ) ;
#11640=DIRECTION ( 'NONE',  ( -0.000000000000000000, 1.259100132267607459E-16, -1.000000000000000000 ) ) ;
#11641=CARTESIAN_POINT ( 'NONE',  ( 3.500000000000001776, 19.52072594216371115, -88.07139747004409003 ) ) ;
#11642=CARTESIAN_POINT ( 'NONE',  ( -3.310556943750000425, 19.41135094264166483, -71.93493913623279923 ) ) ;
#11645=CARTESIAN_POINT ( 'NONE',  ( 0.000000000000000000, 17.50000000000002487, -149.5231586289125687 ) ) ;
#11646=CARTESIAN_POINT ( 'NONE',  ( 3.500000000000001776, 19.52072594216370760, -49.37764746908818836 ) ) ;
#11647=CARTESIAN_POINT ( 'NONE',  ( 1.655278471874998436, 14.63297358603754894, -120.4307724695661364 ) ) ;
#11648=CARTESIAN_POINT ( 'NONE',  ( 0.000000000000000000, 17.50000000000002487, -149.5231586289125687 ) ) ;
#11651=CARTESIAN_POINT ( 'NONE',  ( -7.424026671074350129E-16, 13.45854811567263987, -113.4047308033774328 ) ) ;
#11652=CARTESIAN_POINT ( 'NONE',  ( -1.750000000000002220, 14.46891108675449011, -139.7943141357548313 ) ) ;
#11653=DIRECTION ( 'NONE',  ( -0.000000000000000000, 1.259100132267607459E-16, -1.000000000000000000 ) ) ;
#11654=CARTESIAN_POINT ( 'NONE',  ( 3.500000000000000000, 15.47927405783632082, -37.54431413575484555 ) ) ;
#11657=CARTESIAN_POINT ( 'NONE',  ( -3.310556943750000425, 19.41135094264166483, -71.84743913623280775 ) ) ;
#11658=CARTESIAN_POINT ( 'NONE',  ( 0.000000000000000000, 21.00000000000002487, -149.5231586289125687 ) ) ;
#11659=VECTOR ( 'NONE', #12703, 1000.000000000000000 ) ;
#11660=CARTESIAN_POINT ( 'NONE',  ( 4.648177544792955347E-16, 21.00000000000001421, -69.21098080242148853 ) ) ;
#11662=EDGE_CURVE ( 'NONE', #14972, #3661, #4167, .T. ) ;
#11663=CARTESIAN_POINT ( 'NONE',  ( 4.286263797015737581E-16, 14.00000000000002487, -149.5231586289125687 ) ) ;
#11665=CARTESIAN_POINT ( 'NONE',  ( 3.310556943750001313, 19.41135094264166483, -79.18077246956615056 ) ) ;
#11666=ORIENTED_EDGE ( 'NONE', *, *, #12891, .F. ) ;
#11672=CARTESIAN_POINT ( 'NONE',  ( 3.500000000000001332, 17.50000000000002132, -129.1547308033774186 ) ) ;
#11674=CARTESIAN_POINT ( 'NONE',  ( 4.648177544792955347E-16, 21.00000000000002132, -126.9047308033774186 ) ) ;
#11675=CARTESIAN_POINT ( 'NONE',  ( -3.310556943750000425, 19.41135094264166128, -47.93493913623279212 ) ) ;
#11676=CARTESIAN_POINT ( 'NONE',  ( -3.310556943750002645, 15.58864905735837425, -108.7682724695661420 ) ) ;
#11678=( BOUNDED_CURVE ( )  B_SPLINE_CURVE ( 2, ( #36914, #17350, #30311, #1599, #13944, #8184, #40095, #21157, #34131 ),
 .UNSPECIFIED., .F., .T. ) 
 B_SPLINE_CURVE_WITH_KNOTS ( ( 3, 2, 2, 2, 3 ),
 ( 0.2687499999999999889, 0.2694444444444444309, 0.2708333333333333148, 0.2722222222222221988, 0.2729166666666666963 ),
 .UNSPECIFIED. ) 
 CURVE ( )  GEOMETRIC_REPRESENTATION_ITEM ( )  RATIONAL_B_SPLINE_CURVE ( ( 0.9330127018922194093, 0.9330127018922194093, 1.000000000000000000, 0.8660254037844387076, 1.000000000000000000, 0.8660254037844387076, 1.000000000000000000, 0.9330127018922167448, 0.9330127018922194093 ) ) 
 REPRESENTATION_ITEM ( '' )  );
#11679=CARTESIAN_POINT ( 'NONE',  ( -3.310556943750002645, 15.58864905735836537, -35.68077246956613635 ) ) ;
#11680=CARTESIAN_POINT ( 'NONE',  ( 3.310556943750001313, 17.50000000000001421, -63.35160580289946353 ) ) ;
#11681=CARTESIAN_POINT ( 'NONE',  ( 1.750000000000001110, 20.53108891324555785, -112.2943141357548456 ) ) ;
#11683=CARTESIAN_POINT ( 'NONE',  ( -3.310556943750001313, 17.50000000000001776, -96.76410580289947916 ) ) ;
#11684=DIRECTION ( 'NONE',  ( 0.000000000000000000, 1.000000000000000000, 0.000000000000000000 ) ) ;
#11685=CARTESIAN_POINT ( 'NONE',  ( 1.750000000000001110, 20.53108891324555429, -84.98806413671076143 ) ) ;
#11687=CARTESIAN_POINT ( 'NONE',  ( -1.749999999999999778, 20.53108891324555074, -67.12764746908817415 ) ) ;
#11689=CARTESIAN_POINT ( 'NONE',  ( 3.310556943749999981, 15.58864905735836182, -34.34743913623281486 ) ) ;
#11690=CARTESIAN_POINT ( 'NONE',  ( -1.750000000000002220, 14.46891108675447946, -55.48806413671075433 ) ) ;
#11691=CARTESIAN_POINT ( 'NONE',  ( 4.286263797015737581E-16, 14.00000000000002487, -149.5231586289125687 ) ) ;
#11692=CARTESIAN_POINT ( 'NONE',  ( 3.310556943750001313, 19.41135094264166838, -108.2682724695661278 ) ) ;
#11693=CARTESIAN_POINT ( 'NONE',  ( -1.655278471875002211, 14.63297358603754006, -36.68493913623279923 ) ) ;
#11695=CARTESIAN_POINT ( 'NONE',  ( 3.500000000000001332, 19.52072594216370760, -53.37764746908817415 ) ) ;
#11696=AXIS2_PLACEMENT_3D ( 'NONE', #25160, #25372, #35561 ) ;
#11700=CARTESIAN_POINT ( 'NONE',  ( -3.500000000000001332, 17.50000000000001421, -49.96098080242150274 ) ) ;
#11702=CARTESIAN_POINT ( 'NONE',  ( -3.310556943750002201, 15.58864905735837247, -88.68077246956613635 ) ) ;
#11704=VECTOR ( 'NONE', #6859, 1000.000000000000000 ) ;
#11707=CARTESIAN_POINT ( 'NONE',  ( -1.394453263437886604E-15, 14.00000000000001776, -90.71098080242150274 ) ) ;
#11708=CARTESIAN_POINT ( 'NONE',  ( 3.500000000000001332, 19.52072594216371826, -133.0713974700441042 ) ) ;
#11709=VERTEX_POINT ( 'NONE', #555 ) ;
#11711=CARTESIAN_POINT ( 'NONE',  ( -1.394453263437886604E-15, 14.00000000000001066, -30.71098080242150630 ) ) ;
#11715=CARTESIAN_POINT ( 'NONE',  ( -0.9378221735089291577, 21.00000000000001776, -78.86007260463891555 ) ) ;
#11721=ADVANCED_FACE ( 'NONE', ( #14163 ), #36710, .T. ) ;
#11724=CARTESIAN_POINT ( 'NONE',  ( -3.310556943750001313, 17.50000000000002487, -135.7641058028994792 ) ) ;
#11725=VECTOR ( 'NONE', #28253, 1000.000000000000000 ) ;
#11726=DIRECTION ( 'NONE',  ( 0.000000000000000000, 1.000000000000000000, 0.000000000000000000 ) ) ;
#11730=CARTESIAN_POINT ( 'NONE',  ( 1.655278471875001101, 20.36702641396249547, -124.1849391362327992 ) ) ;
#11731=CARTESIAN_POINT ( 'NONE',  ( 3.310556943750001313, 17.50000000000001421, -54.35160580289946353 ) ) ;
#11732=ORIENTED_EDGE ( 'NONE', *, *, #26875, .F. ) ;
#11733=AXIS2_PLACEMENT_3D ( 'NONE', #19571, #22347, #28934 ) ;
#11735=CARTESIAN_POINT ( 'NONE',  ( -1.749999999999999778, 20.53108891324556140, -134.8213974700441042 ) ) ;
#11738=CARTESIAN_POINT ( 'NONE',  ( -7.022189441860112050E-16, 13.67729811471672363, -82.60160580289945642 ) ) ;
#11739=CARTESIAN_POINT ( 'NONE',  ( -3.500000000000002220, 15.47927405783633503, -129.8776474690881741 ) ) ;
#11740=CARTESIAN_POINT ( 'NONE',  ( -1.655278471874999990, 20.36702641396249547, -114.9307724695661364 ) ) ;
#11744=CARTESIAN_POINT ( 'NONE',  ( -7.424026671074350129E-16, 13.45854811567263454, -79.71098080242151696 ) ) ;
#11746=CARTESIAN_POINT ( 'NONE',  ( 1.655278471874998436, 14.63297358603754006, -46.43077246956614346 ) ) ;
#11747=CARTESIAN_POINT ( 'NONE',  ( -1.655278471875002211, 14.63297358603754894, -108.6849391362327992 ) ) ;
#11748=CYLINDRICAL_SURFACE ( 'NONE', #18703, 3.499999999999999556 ) ;
#11749=FACE_OUTER_BOUND ( 'NONE', #5245, .T. ) ;
#11750=CARTESIAN_POINT ( 'NONE',  ( -1.750000000000002220, 14.46891108675448123, -72.48806413671076143 ) ) ;
#11751=CARTESIAN_POINT ( 'NONE',  ( -3.310556943750000425, 19.41135094264166838, -121.9349391362327992 ) ) ;
#11754=CARTESIAN_POINT ( 'NONE',  ( 3.500000000000001332, 17.50000000000002487, -143.1547308033774186 ) ) ;
#11756=CARTESIAN_POINT ( 'NONE',  ( -3.500000000000000000, 19.52072594216371115, -101.0443141357548456 ) ) ;
#11757=CARTESIAN_POINT ( 'NONE',  ( 2.340729813953370519E-16, 21.32270188528330834, -58.10160580289947063 ) ) ;
#11758=ORIENTED_EDGE ( 'NONE', *, *, #32081, .T. ) ;
#11759=CARTESIAN_POINT ( 'NONE',  ( -3.310556943750002201, 15.58864905735837070, -72.76827246956612782 ) ) ;
#11760=LINE ( 'NONE', #34524, #33948 ) ;
#11767=CARTESIAN_POINT ( 'NONE',  ( -3.310556943750002201, 15.58864905735836537, -37.68077246956613635 ) ) ;
#11768=AXIS2_PLACEMENT_3D ( 'NONE', #26801, #32328, #25956 ) ;
#11770=ORIENTED_EDGE ( 'NONE', *, *, #16758, .F. ) ;
#11774=CARTESIAN_POINT ( 'NONE',  ( -3.310556943750001313, 17.50000000000001066, -44.76410580289947916 ) ) ;
#11775=VERTEX_POINT ( 'NONE', #27139 ) ;
#11776=EDGE_LOOP ( 'NONE', ( #34940, #10438, #8667, #33366 ) ) ;
#11780=CARTESIAN_POINT ( 'NONE',  ( 1.749999999999998224, 14.46891108675448478, -113.3213974700440900 ) ) ;
#11783=CARTESIAN_POINT ( 'NONE',  ( -7.424026671074350129E-16, 13.45854811567263098, -37.71098080242150985 ) ) ;
#11784=CYLINDRICAL_SURFACE ( 'NONE', #34997, 3.499999999999999556 ) ;
#11785=FACE_OUTER_BOUND ( 'NONE', #6892, .T. ) ;
#11790=CARTESIAN_POINT ( 'NONE',  ( 2.474675557024783212E-16, 21.54145188432740810, -142.2109808024214885 ) ) ;
#11791=CARTESIAN_POINT ( 'NONE',  ( -1.750000000000002220, 14.46891108675448478, -106.4880641367107614 ) ) ;
#11792=CARTESIAN_POINT ( 'NONE',  ( -1.655278471874999990, 20.36702641396249547, -126.9307724695661364 ) ) ;
#11796=CARTESIAN_POINT ( 'NONE',  ( 0.9378221735089281585, 14.00000000000001776, -94.36007260463890134 ) ) ;
#11797=CARTESIAN_POINT ( 'NONE',  ( 3.310556943750001313, 17.50000000000002132, -120.3516058028994706 ) ) ;
#11799=CARTESIAN_POINT ( 'NONE',  ( -3.500000000000002220, 15.47927405783632082, -36.57139747004409003 ) ) ;
#11800=CARTESIAN_POINT ( 'NONE',  ( -1.394453263437886604E-15, 14.00000000000001066, -46.40473080337741862 ) ) ;
#11802=CARTESIAN_POINT ( 'NONE',  ( 3.310556943750001313, 19.41135094264167549, -141.2682724695661420 ) ) ;
#11803=CARTESIAN_POINT ( 'NONE',  ( 0.000000000000000000, 17.50000000000002487, -149.5231586289125687 ) ) ;
#11804=CARTESIAN_POINT ( 'NONE',  ( -3.310556943750001313, 17.50000000000001066, -46.85160580289945642 ) ) ;
#11807=CARTESIAN_POINT ( 'NONE',  ( -1.655278471874999990, 20.36702641396249192, -77.01827246956612782 ) ) ;
#11809=CARTESIAN_POINT ( 'NONE',  ( -1.655278471874999990, 20.36702641396249547, -102.9307724695661364 ) ) ;
#11810=CARTESIAN_POINT ( 'NONE',  ( 1.655278471874998436, 14.63297358603754361, -69.43077246956613635 ) ) ;
#11812=CARTESIAN_POINT ( 'NONE',  ( 2.340729813953370519E-16, 21.32270188528331190, -93.10160580289947063 ) ) ;
#11814=CARTESIAN_POINT ( 'NONE',  ( -0.9378221735089291577, 21.00000000000002132, -108.1663226036829712 ) ) ;
#11815=CARTESIAN_POINT ( 'NONE',  ( -3.500000000000000000, 19.52072594216371826, -106.0443141357548456 ) ) ;
#11817=CARTESIAN_POINT ( 'NONE',  ( -3.310556943750002201, 15.58864905735836892, -54.68077246956613635 ) ) ;
#11819=CARTESIAN_POINT ( 'NONE',  ( 4.648177544792955347E-16, 21.00000000000001421, -71.90473080337743284 ) ) ;
#11820=CARTESIAN_POINT ( 'NONE',  ( -3.310556943750001313, 17.50000000000002132, -111.7641058028994649 ) ) ;
#11822=ORIENTED_EDGE ( 'NONE', *, *, #17861, .T. ) ;
#11827=CARTESIAN_POINT ( 'NONE',  ( 3.310556943749999981, 15.58864905735836537, -64.34743913623280775 ) ) ;
#11828=VERTEX_POINT ( 'NONE', #40531 ) ;
#11830=DIRECTION ( 'NONE',  ( -0.000000000000000000, 1.259100132267607459E-16, -1.000000000000000000 ) ) ;
#11835=ORIENTED_EDGE ( 'NONE', *, *, #12153, .F. ) ;
#11837=CARTESIAN_POINT ( 'NONE',  ( -3.310556943750002201, 15.58864905735837780, -128.6807724695661364 ) ) ;
#11838=EDGE_CURVE ( 'NONE', #8593, #20942, #27887, .T. ) ;
#11839=CARTESIAN_POINT ( 'NONE',  ( -7.022189441860112050E-16, 13.67729811471671653, -41.60160580289947063 ) ) ;
#11840=CARTESIAN_POINT ( 'NONE',  ( 1.655278471874998436, 14.63297358603753828, -34.51827246956614204 ) ) ;
#11841=CARTESIAN_POINT ( 'NONE',  ( -7.022189441860112050E-16, 13.67729811471672541, -95.60160580289945642 ) ) ;
#11842=CARTESIAN_POINT ( 'NONE',  ( 1.750000000000001110, 20.53108891324554719, -26.98806413671076143 ) ) ;
#11843=ORIENTED_EDGE ( 'NONE', *, *, #29565, .T. ) ;
#11845=CARTESIAN_POINT ( 'NONE',  ( 1.655278471875001101, 20.36702641396249902, -140.1849391362327708 ) ) ;
#11848=CARTESIAN_POINT ( 'NONE',  ( 1.749999999999998224, 14.46891108675448123, -87.32139747004409003 ) ) ;
#11849=CARTESIAN_POINT ( 'NONE',  ( -3.310556943750001313, 17.50000000000001421, -60.76410580289946495 ) ) ;
#11850=CARTESIAN_POINT ( 'NONE',  ( -3.500000000000001332, 17.50000000000002132, -122.6547308033774186 ) ) ;
#11851=CARTESIAN_POINT ( 'NONE',  ( 1.749999999999998224, 14.46891108675448123, -84.32139747004409003 ) ) ;
#11852=CARTESIAN_POINT ( 'NONE',  ( 2.340729813953370519E-16, 21.32270188528331190, -63.10160580289946353 ) ) ;
#11855=CARTESIAN_POINT ( 'NONE',  ( -1.749999999999999778, 20.53108891324555429, -91.12764746908817415 ) ) ;
#11857=CARTESIAN_POINT ( 'NONE',  ( -1.394453263437886604E-15, 14.00000000000001066, -29.40473080337743284 ) ) ;
#11858=CARTESIAN_POINT ( 'NONE',  ( 1.655278471874998436, 14.63297358603754894, -118.4307724695661364 ) ) ;
#11860=( BOUNDED_CURVE ( )  B_SPLINE_CURVE ( 2, ( #3372, #16357, #9550, #16156, #29094, #42093, #41669, #13153, #35901 ),
 .UNSPECIFIED., .F., .T. ) 
 B_SPLINE_CURVE_WITH_KNOTS ( ( 3, 2, 2, 2, 3 ),
 ( 0.7604166666666666297, 0.7611111111111110716, 0.7624999999999999556, 0.7638888888888888395, 0.7645833333333332815 ),
 .UNSPECIFIED. ) 
 CURVE ( )  GEOMETRIC_REPRESENTATION_ITEM ( )  RATIONAL_B_SPLINE_CURVE ( ( 0.9330127018922194093, 0.9330127018922194093, 1.000000000000000000, 0.8660254037844387076, 1.000000000000000000, 0.8660254037844387076, 1.000000000000000000, 0.9330127018922194093, 0.9330127018922194093 ) ) 
 REPRESENTATION_ITEM ( '' )  );
#11863=CARTESIAN_POINT ( 'NONE',  ( 3.500000000000001776, 19.52072594216371826, -111.0713974700441042 ) ) ;
#11865=( BOUNDED_CURVE ( )  B_SPLINE_CURVE ( 2, ( #15276, #28235, #41221, #8882, #16738, #23331, #35676, #38862, #6322 ),
 .UNSPECIFIED., .F., .F. ) 
 B_SPLINE_CURVE_WITH_KNOTS ( ( 3, 2, 2, 2, 3 ),
 ( 0.6937499999999999778, 0.6944444444444444198, 0.6958333333333333037, 0.6972222222222221877, 0.6979166666666666297 ),
 .UNSPECIFIED. ) 
 CURVE ( )  GEOMETRIC_REPRESENTATION_ITEM ( )  RATIONAL_B_SPLINE_CURVE ( ( 0.9330127018922194093, 0.9330127018922194093, 1.000000000000000000, 0.8660254037844387076, 1.000000000000000000, 0.8660254037844387076, 1.000000000000000000, 0.9330127018922194093, 0.9330127018922194093 ) ) 
 REPRESENTATION_ITEM ( '' )  );
#11870=CARTESIAN_POINT ( 'NONE',  ( -1.655278471874999990, 20.36702641396248836, -72.93077246956613635 ) ) ;
#11872=CYLINDRICAL_SURFACE ( 'NONE', #40224, 3.499999999999999556 ) ;
#11874=DIRECTION ( 'NONE',  ( -0.000000000000000000, 1.259100132267607459E-16, -1.000000000000000000 ) ) ;
#11875=ORIENTED_EDGE ( 'NONE', *, *, #12967, .F. ) ;
#11876=CARTESIAN_POINT ( 'NONE',  ( -1.655278471875002211, 14.63297358603753828, -25.59743913623280065 ) ) ;
#11878=CARTESIAN_POINT ( 'NONE',  ( -3.310556943750000425, 19.41135094264166483, -78.84743913623282197 ) ) ;
#11879=ORIENTED_EDGE ( 'NONE', *, *, #23139, .T. ) ;
#11881=DIRECTION ( 'NONE',  ( -0.000000000000000000, 1.259100132267607459E-16, -1.000000000000000000 ) ) ;
#11885=AXIS2_PLACEMENT_3D ( 'NONE', #38159, #5624, #17411 ) ;
#11886=ORIENTED_EDGE ( 'NONE', *, *, #22519, .F. ) ;
#11888=CARTESIAN_POINT ( 'NONE',  ( 1.655278471875001101, 20.36702641396248836, -51.18493913623279923 ) ) ;
#11889=CARTESIAN_POINT ( 'NONE',  ( 2.340729813953370519E-16, 21.32270188528331900, -110.1016058028994706 ) ) ;
#11890=ORIENTED_EDGE ( 'NONE', *, *, #40244, .T. ) ;
#11891=EDGE_CURVE ( 'NONE', #11305, #24713, #4785, .T. ) ;
#11892=CARTESIAN_POINT ( 'NONE',  ( 1.655278471875001101, 20.36702641396248481, -34.09743913623280775 ) ) ;
#11893=CARTESIAN_POINT ( 'NONE',  ( -1.655278471875002211, 14.63297358603754361, -58.68493913623279212 ) ) ;
#11894=CARTESIAN_POINT ( 'NONE',  ( 3.500000000000001332, 17.50000000000002132, -110.4609808024215027 ) ) ;
#11895=EDGE_CURVE ( 'NONE', #19157, #16027, #25171, .T. ) ;
#11897=CARTESIAN_POINT ( 'NONE',  ( 1.655278471875001101, 20.36702641396249192, -96.09743913623280775 ) ) ;
#11898=CARTESIAN_POINT ( 'NONE',  ( -0.9378221735089465882, 21.00000000000001066, -124.8600726046389013 ) ) ;
#11900=CARTESIAN_POINT ( 'NONE',  ( 1.749999999999998224, 14.46891108675447768, -65.62764746908818836 ) ) ;
#11902=CARTESIAN_POINT ( 'NONE',  ( -1.655278471874999990, 20.36702641396248481, -28.93077246956614346 ) ) ;
#11903=CARTESIAN_POINT ( 'NONE',  ( -3.500000000000001332, 17.50000000000001421, -51.65473080337743284 ) ) ;
#11905=CARTESIAN_POINT ( 'NONE',  ( 1.655278471875001101, 20.36702641396249547, -105.1849391362327992 ) ) ;
#11906=CARTESIAN_POINT ( 'NONE',  ( -1.655278471874999990, 20.36702641396248481, -38.01827246956612782 ) ) ;
#11914=CARTESIAN_POINT ( 'NONE',  ( -3.310556943750000425, 19.41135094264166838, -88.84743913623280775 ) ) ;
#11915=CARTESIAN_POINT ( 'NONE',  ( 3.602337597214540226E-14, 14.00000000000002132, -117.4047308033774328 ) ) ;
#11917=VERTEX_POINT ( 'NONE', #14591 ) ;
#11920=CARTESIAN_POINT ( 'NONE',  ( -1.394453263437886604E-15, 14.00000000000001421, -74.71098080242151696 ) ) ;
#11927=CARTESIAN_POINT ( 'NONE',  ( 0.000000000000000000, 17.50000000000002487, -149.5231586289125687 ) ) ;
#11928=VERTEX_POINT ( 'NONE', #5001 ) ;
#11931=DIRECTION ( 'NONE',  ( 0.000000000000000000, 1.000000000000000000, 0.000000000000000000 ) ) ;
#11934=( BOUNDED_CURVE ( )  B_SPLINE_CURVE ( 2, ( #40833, #40621, #31673, #34040, #2541, #21478, #24683, #28481, #8501 ),
 .UNSPECIFIED., .F., .T. ) 
 B_SPLINE_CURVE_WITH_KNOTS ( ( 3, 2, 2, 2, 3 ),
 ( 0.7187500000000000000, 0.7194444444444444420, 0.7208333333333333259, 0.7222222222222222099, 0.7229166666666666519 ),
 .UNSPECIFIED. ) 
 CURVE ( )  GEOMETRIC_REPRESENTATION_ITEM ( )  RATIONAL_B_SPLINE_CURVE ( ( 0.9330127018922194093, 0.9330127018922194093, 1.000000000000000000, 0.8660254037844387076, 1.000000000000000000, 0.8660254037844387076, 1.000000000000000000, 0.9330127018922194093, 0.9330127018922194093 ) ) 
 REPRESENTATION_ITEM ( '' )  );
#11935=EDGE_LOOP ( 'NONE', ( #22881, #28252, #16813, #27336 ) ) ;
#11937=DIRECTION ( 'NONE',  ( -0.000000000000000000, 1.259100132267607459E-16, -1.000000000000000000 ) ) ;
#11938=CARTESIAN_POINT ( 'NONE',  ( 1.655278471874998436, 14.63297358603755072, -135.4307724695661364 ) ) ;
#11939=CYLINDRICAL_SURFACE ( 'NONE', #24437, 3.499999999999999556 ) ;
#11942=CARTESIAN_POINT ( 'NONE',  ( 1.655278471874998436, 14.63297358603755072, -124.5182724695661278 ) ) ;
#11943=CARTESIAN_POINT ( 'NONE',  ( -7.022189441860112050E-16, 13.67729811471671830, -56.60160580289947063 ) ) ;
#11946=CARTESIAN_POINT ( 'NONE',  ( 1.750000000000001110, 20.53108891324556140, -133.9880641367107614 ) ) ;
#11947=VECTOR ( 'NONE', #15466, 1000.000000000000000 ) ;
#11950=CARTESIAN_POINT ( 'NONE',  ( 3.310556943750001313, 17.50000000000001776, -77.35160580289945642 ) ) ;
#11951=CARTESIAN_POINT ( 'NONE',  ( -3.500000000000001332, 17.50000000000002132, -128.9609808024215170 ) ) ;
#11952=CARTESIAN_POINT ( 'NONE',  ( 3.310556943750001313, 17.50000000000002132, -111.2641058028994649 ) ) ;
#11956=CARTESIAN_POINT ( 'NONE',  ( -1.750000000000002220, 14.46891108675448123, -80.79431413575484555 ) ) ;
#11957=CARTESIAN_POINT ( 'NONE',  ( -3.500000000000002220, 15.47927405783632615, -61.87764746908818836 ) ) ;
#11958=CARTESIAN_POINT ( 'NONE',  ( -7.022189441860112050E-16, 13.67729811471671653, -46.51410580289946495 ) ) ;
#11959=CARTESIAN_POINT ( 'NONE',  ( 3.310556943750001313, 17.50000000000001776, -99.35160580289947063 ) ) ;
#11961=CARTESIAN_POINT ( 'NONE',  ( 0.9378221735089281585, 14.00000000000000888, -39.66632260368299256 ) ) ;
#11964=CARTESIAN_POINT ( 'NONE',  ( 1.655278471874998436, 14.63297358603754894, -121.5182724695661278 ) ) ;
#11972=ORIENTED_EDGE ( 'NONE', *, *, #12153, .T. ) ;
#11973=CARTESIAN_POINT ( 'NONE',  ( -3.310556943750001313, 17.50000000000001421, -73.85160580289947063 ) ) ;
#11979=CARTESIAN_POINT ( 'NONE',  ( -1.655278471875002211, 14.63297358603754006, -37.59743913623281486 ) ) ;
#11980=CARTESIAN_POINT ( 'NONE',  ( 1.749999999999998224, 14.46891108675447946, -72.32139747004409003 ) ) ;
#11981=AXIS2_PLACEMENT_3D ( 'NONE', #20586, #23577, #7399 ) ;
#11985=CARTESIAN_POINT ( 'NONE',  ( 3.310556943750001313, 17.50000000000001421, -47.26410580289947205 ) ) ;
#11987=ORIENTED_EDGE ( 'NONE', *, *, #22058, .F. ) ;
#11989=( BOUNDED_CURVE ( )  B_SPLINE_CURVE ( 2, ( #23481, #30056, #36444, #7307, #39847, #23694, #7522, #20495, #1144 ),
 .UNSPECIFIED., .F., .T. ) 
 B_SPLINE_CURVE_WITH_KNOTS ( ( 3, 2, 2, 2, 3 ),
 ( 0.4187500000000000111, 0.4194444444444444531, 0.4208333333333333370, 0.4222222222222222210, 0.4229166666666666630 ),
 .UNSPECIFIED. ) 
 CURVE ( )  GEOMETRIC_REPRESENTATION_ITEM ( )  RATIONAL_B_SPLINE_CURVE ( ( 0.9330127018922194093, 0.9330127018922194093, 1.000000000000000000, 0.8660254037844387076, 1.000000000000000000, 0.8660254037844387076, 1.000000000000000000, 0.9330127018922194093, 0.9330127018922194093 ) ) 
 REPRESENTATION_ITEM ( '' )  );
#11991=CARTESIAN_POINT ( 'NONE',  ( -0.9378221735089291577, 21.00000000000002132, -119.8600726046389013 ) ) ;
#11994=CARTESIAN_POINT ( 'NONE',  ( 0.000000000000000000, 17.50000000000002487, -149.5231586289125687 ) ) ;
#11995=CARTESIAN_POINT ( 'NONE',  ( 1.750000000000001110, 20.53108891324554719, -38.29431413575484555 ) ) ;
#11996=CYLINDRICAL_SURFACE ( 'NONE', #28888, 3.499999999999999556 ) ;
#11997=EDGE_LOOP ( 'NONE', ( #2581, #24553, #27849, #25323 ) ) ;
#11998=DIRECTION ( 'NONE',  ( -0.000000000000000000, 1.000000000000000000, 0.000000000000000000 ) ) ;
#11999=LINE ( 'NONE', #41152, #39034 ) ;
#12001=CARTESIAN_POINT ( 'NONE',  ( -1.655278471874999990, 20.36702641396248481, -24.01827246956612782 ) ) ;
#12002=CARTESIAN_POINT ( 'NONE',  ( -3.500000000000001332, 17.50000000000001776, -100.6547308033774328 ) ) ;
#12003=CARTESIAN_POINT ( 'NONE',  ( -3.310556943750001313, 17.50000000000002132, -126.7641058028994792 ) ) ;
#12006=CARTESIAN_POINT ( 'NONE',  ( -3.500000000000001332, 17.50000000000001776, -76.65473080337741862 ) ) ;
#12007=CARTESIAN_POINT ( 'NONE',  ( 3.310556943750001313, 19.41135094264166838, -124.2682724695661278 ) ) ;
#12009=CARTESIAN_POINT ( 'NONE',  ( 1.749999999999998224, 14.46891108675447413, -38.32139747004409713 ) ) ;
#12012=CARTESIAN_POINT ( 'NONE',  ( -1.655278471874999990, 20.36702641396249902, -140.0182724695661420 ) ) ;
#12013=CARTESIAN_POINT ( 'NONE',  ( 0.9378221735089281585, 14.00000000000000888, -29.66632260368299256 ) ) ;
#12014=CARTESIAN_POINT ( 'NONE',  ( 3.310556943750001313, 17.50000000000001421, -47.35160580289946353 ) ) ;
#12016=CARTESIAN_POINT ( 'NONE',  ( 0.9378221735089300459, 21.00000000000002132, -104.2556390011600342 ) ) ;
#12017=CARTESIAN_POINT ( 'NONE',  ( -3.310556943750001313, 17.50000000000001421, -72.85160580289947063 ) ) ;
#12019=CARTESIAN_POINT ( 'NONE',  ( 2.340729813953370519E-16, 21.32270188528331190, -101.0141058028994792 ) ) ;
#12020=CARTESIAN_POINT ( 'NONE',  ( 1.655278471874998436, 14.63297358603754361, -71.43077246956613635 ) ) ;
#12021=ORIENTED_EDGE ( 'NONE', *, *, #19073, .T. ) ;
#12022=CARTESIAN_POINT ( 'NONE',  ( -3.310556943750000425, 19.41135094264166838, -92.93493913623282765 ) ) ;
#12024=CARTESIAN_POINT ( 'NONE',  ( -3.500000000000000000, 19.52072594216371826, -108.0443141357548740 ) ) ;
#12026=CARTESIAN_POINT ( 'NONE',  ( 3.602337597214540226E-14, 14.00000000000002132, -117.7109808024215027 ) ) ;
#12027=CARTESIAN_POINT ( 'NONE',  ( -7.022189441860112050E-16, 13.67729811471672186, -54.51410580289947916 ) ) ;
#12029=CARTESIAN_POINT ( 'NONE',  ( -1.655278471874999990, 20.36702641396249547, -108.9307724695661506 ) ) ;
#12030=CARTESIAN_POINT ( 'NONE',  ( -3.500000000000001332, 17.50000000000001776, -101.6547308033774328 ) ) ;
#12032=ORIENTED_EDGE ( 'NONE', *, *, #425, .T. ) ;
#12034=ORIENTED_EDGE ( 'NONE', *, *, #634, .T. ) ;
#12036=CARTESIAN_POINT ( 'NONE',  ( -7.022189441860112050E-16, 13.67729811471671830, -62.51410580289947205 ) ) ;
#12037=ORIENTED_EDGE ( 'NONE', *, *, #40371, .T. ) ;
#12038=VERTEX_POINT ( 'NONE', #16069 ) ;
#12039=CARTESIAN_POINT ( 'NONE',  ( 4.648177544792955347E-16, 21.00000000000001066, -30.21098080242151340 ) ) ;
#12043=ORIENTED_EDGE ( 'NONE', *, *, #31046, .T. ) ;
#12044=DIRECTION ( 'NONE',  ( 0.000000000000000000, 1.000000000000000000, 0.000000000000000000 ) ) ;
#12045=CARTESIAN_POINT ( 'NONE',  ( -1.655278471874999990, 20.36702641396249902, -130.9307724695661364 ) ) ;
#12047=CARTESIAN_POINT ( 'NONE',  ( 3.310556943750001313, 19.41135094264165772, -41.26827246956613493 ) ) ;
#12048=CARTESIAN_POINT ( 'NONE',  ( 3.310556943749999981, 15.58864905735836182, -33.43493913623279923 ) ) ;
#12049=CARTESIAN_POINT ( 'NONE',  ( -3.310556943750000425, 19.41135094264166483, -90.93493913623279923 ) ) ;
#12050=CARTESIAN_POINT ( 'NONE',  ( -3.500000000000002220, 15.47927405783632082, -24.57139747004409358 ) ) ;
#12051=VERTEX_POINT ( 'NONE', #29011 ) ;
#12052=EDGE_CURVE ( 'NONE', #15295, #10316, #29503, .T. ) ;
#12053=( BOUNDED_CURVE ( )  B_SPLINE_CURVE ( 2, ( #38686, #29737, #9557, #39517, #35499, #3173, #29101, #42100, #12953 ),
 .UNSPECIFIED., .F., .T. ) 
 B_SPLINE_CURVE_WITH_KNOTS ( ( 3, 2, 2, 2, 3 ),
 ( 0.2604166666666666852, 0.2611111111111111271, 0.2625000000000000111, 0.2638888888888888951, 0.2645833333333333370 ),
 .UNSPECIFIED. ) 
 CURVE ( )  GEOMETRIC_REPRESENTATION_ITEM ( )  RATIONAL_B_SPLINE_CURVE ( ( 0.9330127018922194093, 0.9330127018922194093, 1.000000000000000000, 0.8660254037844387076, 1.000000000000000000, 0.8660254037844387076, 1.000000000000000000, 0.9330127018922194093, 0.9330127018922194093 ) ) 
 REPRESENTATION_ITEM ( '' )  );
#12055=CARTESIAN_POINT ( 'NONE',  ( 3.310556943750001313, 17.50000000000002487, -140.3516058028994564 ) ) ;
#12056=CARTESIAN_POINT ( 'NONE',  ( -3.500000000000002220, 15.47927405783632970, -83.87764746908818836 ) ) ;
#12057=CARTESIAN_POINT ( 'NONE',  ( -3.500000000000000000, 19.52072594216371826, -123.0443141357548456 ) ) ;
#12059=CARTESIAN_POINT ( 'NONE',  ( -1.749999999999999778, 20.53108891324555429, -78.82139747004410424 ) ) ;
#12060=CARTESIAN_POINT ( 'NONE',  ( 3.310556943750001313, 17.50000000000001421, -66.35160580289945642 ) ) ;
#12063=CARTESIAN_POINT ( 'NONE',  ( 1.750000000000001110, 20.53108891324555074, -47.29431413575483845 ) ) ;
#12065=ORIENTED_EDGE ( 'NONE', *, *, #15188, .T. ) ;
#12066=CARTESIAN_POINT ( 'NONE',  ( 2.340729813953370519E-16, 21.32270188528331900, -121.0141058028994792 ) ) ;
#12069=CARTESIAN_POINT ( 'NONE',  ( 3.500000000000001332, 17.50000000000002132, -106.1547308033774186 ) ) ;
#12071=LINE ( 'NONE', #42073, #3664 ) ;
#12073=CARTESIAN_POINT ( 'NONE',  ( -1.394453263437886604E-15, 14.00000000000001421, -59.40473080337742573 ) ) ;
#12075=CARTESIAN_POINT ( 'NONE',  ( -3.310556943750002201, 15.58864905735837070, -71.68077246956613635 ) ) ;
#12076=DIRECTION ( 'NONE',  ( -0.000000000000000000, 1.259100132267607459E-16, -1.000000000000000000 ) ) ;
#12077=ADVANCED_FACE ( 'NONE', ( #38803 ), #12436, .T. ) ;
#12078=FACE_OUTER_BOUND ( 'NONE', #2326, .T. ) ;
#12080=EDGE_CURVE ( 'NONE', #7438, #29090, #25416, .T. ) ;
#12082=CARTESIAN_POINT ( 'NONE',  ( 3.310556943750001313, 19.41135094264166128, -24.18077246956613990 ) ) ;
#12083=CARTESIAN_POINT ( 'NONE',  ( -3.500000000000001332, 17.50000000000002132, -104.9609808024215027 ) ) ;
#12084=CARTESIAN_POINT ( 'NONE',  ( -3.310556943750002645, 15.58864905735837070, -78.68077246956613635 ) ) ;
#12085=ORIENTED_EDGE ( 'NONE', *, *, #27235, .T. ) ;
#12089=CYLINDRICAL_SURFACE ( 'NONE', #17877, 3.499999999999999556 ) ;
#12091=CARTESIAN_POINT ( 'NONE',  ( 1.655278471875001101, 20.36702641396248836, -47.18493913623279923 ) ) ;
#12092=CARTESIAN_POINT ( 'NONE',  ( 2.340729813953370519E-16, 21.32270188528331900, -111.1016058028994564 ) ) ;
#12093=VERTEX_POINT ( 'NONE', #32415 ) ;
#12094=VECTOR ( 'NONE', #28303, 1000.000000000000000 ) ;
#12095=( BOUNDED_CURVE ( )  B_SPLINE_CURVE ( 2, ( #33614, #4677, #26812, #39779, #17455, #7879, #11067, #17656, #23623 ),
 .UNSPECIFIED., .F., .F. ) 
 B_SPLINE_CURVE_WITH_KNOTS ( ( 3, 2, 2, 2, 3 ),
 ( 0.7020833333333332815, 0.7027777777777777235, 0.7041666666666667185, 0.7055555555555556024, 0.7062500000000000444 ),
 .UNSPECIFIED. ) 
 CURVE ( )  GEOMETRIC_REPRESENTATION_ITEM ( )  RATIONAL_B_SPLINE_CURVE ( ( 0.9330127018922194093, 0.9330127018922194093, 1.000000000000000000, 0.8660254037844387076, 1.000000000000000000, 0.8660254037844387076, 1.000000000000000000, 0.9330127018922194093, 0.9330127018922194093 ) ) 
 REPRESENTATION_ITEM ( '' )  );
#12096=ADVANCED_FACE ( 'NONE', ( #15638 ), #31578, .T. ) ;
#12097=CARTESIAN_POINT ( 'NONE',  ( -1.655278471874999990, 20.36702641396248481, -35.93077246956613635 ) ) ;
#12098=CARTESIAN_POINT ( 'NONE',  ( -7.022189441860112050E-16, 13.67729811471671830, -60.60160580289945642 ) ) ;
#12099=CARTESIAN_POINT ( 'NONE',  ( 1.749999999999998224, 14.46891108675448301, -106.6276474690881741 ) ) ;
#12101=CARTESIAN_POINT ( 'NONE',  ( 3.310556943750001313, 19.41135094264166483, -94.18077246956613635 ) ) ;
#12102=CARTESIAN_POINT ( 'NONE',  ( 1.750000000000001110, 20.53108891324555429, -95.98806413671076143 ) ) ;
#12104=CARTESIAN_POINT ( 'NONE',  ( 4.648177544792955347E-16, 21.00000000000001776, -84.90473080337743284 ) ) ;
#12106=CARTESIAN_POINT ( 'NONE',  ( -3.500000000000002220, 15.47927405783632437, -62.87764746908818125 ) ) ;
#12107=CARTESIAN_POINT ( 'NONE',  ( -1.394453263437886604E-15, 14.00000000000001421, -80.71098080242148853 ) ) ;
#12108=CARTESIAN_POINT ( 'NONE',  ( -3.310556943750000425, 19.41135094264165772, -27.84743913623280065 ) ) ;
#12109=CARTESIAN_POINT ( 'NONE',  ( -3.500000000000001332, 17.50000000000001421, -52.65473080337743284 ) ) ;
#12110=CARTESIAN_POINT ( 'NONE',  ( -1.750000000000002220, 14.46891108675447768, -45.79431413575483845 ) ) ;
#12111=CARTESIAN_POINT ( 'NONE',  ( 2.340729813953370519E-16, 21.32270188528331900, -105.1016058028994564 ) ) ;
#12112=CARTESIAN_POINT ( 'NONE',  ( 3.310556943750001313, 17.50000000000001066, -32.35160580289946353 ) ) ;
#12117=CARTESIAN_POINT ( 'NONE',  ( 3.500000000000001332, 17.50000000000001421, -48.46098080242150274 ) ) ;
#12119=CARTESIAN_POINT ( 'NONE',  ( -3.310556943750002201, 15.58864905735837247, -86.68077246956613635 ) ) ;
#12120=CARTESIAN_POINT ( 'NONE',  ( -3.500000000000001332, 17.50000000000001066, -23.96098080242150985 ) ) ;
#12121=ORIENTED_EDGE ( 'NONE', *, *, #41964, .F. ) ;
#12122=CARTESIAN_POINT ( 'NONE',  ( 3.369928719974892676E-15, 14.00000000000002309, -139.7109808024214885 ) ) ;
#12123=EDGE_LOOP ( 'NONE', ( #9063, #23014, #16346, #267 ) ) ;
#12125=CARTESIAN_POINT ( 'NONE',  ( -1.750000000000002220, 14.46891108675447590, -30.79431413575484200 ) ) ;
#12127=CARTESIAN_POINT ( 'NONE',  ( -3.310556943750002645, 15.58864905735837425, -96.68077246956612214 ) ) ;
#12129=EDGE_LOOP ( 'NONE', ( #18906, #39339, #35588, #1231 ) ) ;
#12130=DIRECTION ( 'NONE',  ( -0.000000000000000000, 1.259100132267607459E-16, -1.000000000000000000 ) ) ;
#12131=ORIENTED_EDGE ( 'NONE', *, *, #38377, .T. ) ;
#12134=EDGE_CURVE ( 'NONE', #17606, #5180, #28595, .T. ) ;
#12136=DIRECTION ( 'NONE',  ( -0.000000000000000000, 1.259100132267607459E-16, -1.000000000000000000 ) ) ;
#12140=VERTEX_POINT ( 'NONE', #38385 ) ;
#12141=CARTESIAN_POINT ( 'NONE',  ( 0.000000000000000000, 21.00000000000002487, -149.5231586289125687 ) ) ;
#12142=FACE_OUTER_BOUND ( 'NONE', #31343, .T. ) ;
#12144=CARTESIAN_POINT ( 'NONE',  ( -1.655278471874999990, 20.36702641396249902, -137.9307724695661364 ) ) ;
#12145=CARTESIAN_POINT ( 'NONE',  ( 0.9378221735089300459, 21.00000000000001066, -37.94938900211595012 ) ) ;
#12146=ORIENTED_EDGE ( 'NONE', *, *, #3781, .F. ) ;
#12148=CARTESIAN_POINT ( 'NONE',  ( 3.500000000000001332, 19.52072594216370760, -73.07139747004410424 ) ) ;
#12149=CARTESIAN_POINT ( 'NONE',  ( 3.310556943749999981, 15.58864905735837425, -127.4349391362327992 ) ) ;
#12150=CARTESIAN_POINT ( 'NONE',  ( -1.655278471875002211, 14.63297358603754184, -52.68493913623280633 ) ) ;
#12153=EDGE_CURVE ( 'NONE', #5717, #14314, #13468, .T. ) ;
#12154=CARTESIAN_POINT ( 'NONE',  ( -3.500000000000000888, 19.52072594216372181, -135.7380641367107899 ) ) ;
#12155=ADVANCED_FACE ( 'NONE', ( #35615 ), #29209, .T. ) ;
#12157=CARTESIAN_POINT ( 'NONE',  ( -3.310556943750000425, 19.41135094264166483, -78.93493913623279923 ) ) ;
#12158=CARTESIAN_POINT ( 'NONE',  ( -1.750000000000002220, 14.46891108675448834, -127.7943141357548456 ) ) ;
#12159=CARTESIAN_POINT ( 'NONE',  ( 3.310556943750001313, 17.50000000000002132, -108.2641058028994649 ) ) ;
#12160=CARTESIAN_POINT ( 'NONE',  ( 3.500000000000000000, 15.47927405783632793, -93.23806413671076143 ) ) ;
#12163=CARTESIAN_POINT ( 'NONE',  ( 2.474675557024783212E-16, 21.54145188432739744, -80.21098080242150274 ) ) ;
#12165=CARTESIAN_POINT ( 'NONE',  ( -7.460324959392693302E-14, 21.00000000000002132, -102.9047308033774044 ) ) ;
#12166=CARTESIAN_POINT ( 'NONE',  ( -3.310556943750002645, 15.58864905735836714, -41.68077246956614346 ) ) ;
#12167=CARTESIAN_POINT ( 'NONE',  ( -3.310556943750001313, 17.50000000000001776, -98.85160580289947063 ) ) ;
#12168=CARTESIAN_POINT ( 'NONE',  ( 1.750000000000001110, 20.53108891324555785, -110.9880641367107614 ) ) ;
#12169=CARTESIAN_POINT ( 'NONE',  ( 0.000000000000000000, 21.00000000000002487, -149.5231586289125687 ) ) ;
#12171=CARTESIAN_POINT ( 'NONE',  ( -1.655278471875002211, 14.63297358603755072, -122.6849391362327992 ) ) ;
#12175=CARTESIAN_POINT ( 'NONE',  ( -1.394453263437886604E-15, 14.00000000000001066, -44.40473080337743284 ) ) ;
#12176=CARTESIAN_POINT ( 'NONE',  ( 0.9378221735089300459, 21.00000000000002487, -129.9493890021159359 ) ) ;
#12177=CARTESIAN_POINT ( 'NONE',  ( 4.648177544792955347E-16, 21.00000000000001421, -52.90473080337743284 ) ) ;
#12180=CARTESIAN_POINT ( 'NONE',  ( 1.655278471875001101, 20.36702641396248836, -74.18493913623279923 ) ) ;
#12184=CARTESIAN_POINT ( 'NONE',  ( -1.394453263437886604E-15, 14.00000000000001776, -99.40473080337743284 ) ) ;
#12186=DIRECTION ( 'NONE',  ( 0.000000000000000000, 1.000000000000000000, 0.000000000000000000 ) ) ;
#12189=CARTESIAN_POINT ( 'NONE',  ( 2.340729813953370519E-16, 21.32270188528330834, -37.01410580289946495 ) ) ;
#12195=CARTESIAN_POINT ( 'NONE',  ( -1.655278471875002211, 14.63297358603754184, -49.59743913623280775 ) ) ;
#12196=ORIENTED_EDGE ( 'NONE', *, *, #23614, .F. ) ;
#12197=VERTEX_POINT ( 'NONE', #17103 ) ;
#12202=CARTESIAN_POINT ( 'NONE',  ( 3.500000000000001332, 19.52072594216370760, -63.07139747004410424 ) ) ;
#12203=EDGE_CURVE ( 'NONE', #104, #20208, #7105, .T. ) ;
#12204=CARTESIAN_POINT ( 'NONE',  ( 0.9378221735089281585, 14.00000000000001776, -89.66632260368298546 ) ) ;
#12205=CARTESIAN_POINT ( 'NONE',  ( -3.500000000000000888, 19.52072594216370405, -36.04431413575484555 ) ) ;
#12207=CARTESIAN_POINT ( 'NONE',  ( -0.9378221735089310451, 14.00000000000001599, -76.75563900116002003 ) ) ;
#12208=VECTOR ( 'NONE', #32724, 1000.000000000000000 ) ;
#12210=CARTESIAN_POINT ( 'NONE',  ( 1.749999999999998224, 14.46891108675448834, -142.6276474690881741 ) ) ;
#12211=DIRECTION ( 'NONE',  ( 0.000000000000000000, 1.000000000000000000, 0.000000000000000000 ) ) ;
#12212=CARTESIAN_POINT ( 'NONE',  ( 1.655278471874998436, 14.63297358603754894, -122.4307724695661364 ) ) ;
#12215=CARTESIAN_POINT ( 'NONE',  ( 1.749999999999998224, 14.46891108675448123, -94.32139747004409003 ) ) ;
#12216=CARTESIAN_POINT ( 'NONE',  ( -3.310556943750002645, 15.58864905735837780, -119.7682724695661278 ) ) ;
#12217=FACE_OUTER_BOUND ( 'NONE', #32698, .T. ) ;
#12218=CARTESIAN_POINT ( 'NONE',  ( -3.500000000000000888, 19.52072594216370405, -35.73806413671076854 ) ) ;
#12219=CARTESIAN_POINT ( 'NONE',  ( -0.9378221735089291577, 21.00000000000002132, -121.8600726046389013 ) ) ;
#12221=CARTESIAN_POINT ( 'NONE',  ( -1.655278471875002211, 14.63297358603755427, -137.6849391362327992 ) ) ;
#12223=DIRECTION ( 'NONE',  ( 0.000000000000000000, 1.000000000000000000, 0.000000000000000000 ) ) ;
#12224=CARTESIAN_POINT ( 'NONE',  ( -7.022189441860112050E-16, 13.67729811471671830, -46.60160580289946353 ) ) ;
#12226=CARTESIAN_POINT ( 'NONE',  ( -1.750000000000002220, 14.46891108675448123, -72.79431413575483134 ) ) ;
#12227=CARTESIAN_POINT ( 'NONE',  ( 1.655278471874998436, 14.63297358603754361, -70.51827246956612782 ) ) ;
#12230=CARTESIAN_POINT ( 'NONE',  ( 2.340729813953370519E-16, 21.32270188528330834, -69.01410580289947916 ) ) ;
#12232=CARTESIAN_POINT ( 'NONE',  ( -7.022189441860112050E-16, 13.67729811471672363, -92.60160580289947063 ) ) ;
#12234=CARTESIAN_POINT ( 'NONE',  ( -1.749999999999999778, 20.53108891324555785, -108.1276474690881741 ) ) ;
#12238=CARTESIAN_POINT ( 'NONE',  ( -3.310556943750001313, 17.50000000000001421, -49.76410580289947205 ) ) ;
#12239=FACE_OUTER_BOUND ( 'NONE', #22076, .T. ) ;
#12240=CARTESIAN_POINT ( 'NONE',  ( 2.340729813953370519E-16, 21.32270188528331900, -111.0141058028994792 ) ) ;
#12246=ORIENTED_EDGE ( 'NONE', *, *, #21699, .T. ) ;
#12248=CARTESIAN_POINT ( 'NONE',  ( -3.310556943750002645, 15.58864905735836892, -62.68077246956614346 ) ) ;
#12250=ORIENTED_EDGE ( 'NONE', *, *, #7947, .T. ) ;
#12256=EDGE_LOOP ( 'NONE', ( #18058, #36957, #21702, #29879 ) ) ;
#12257=CARTESIAN_POINT ( 'NONE',  ( -1.394453263437886604E-15, 14.00000000000001066, -28.71098080242150985 ) ) ;
#12258=CARTESIAN_POINT ( 'NONE',  ( 3.310556943750001313, 17.50000000000002487, -132.2641058028994507 ) ) ;
#12261=CARTESIAN_POINT ( 'NONE',  ( 3.310556943749999981, 15.58864905735836182, -41.43493913623279212 ) ) ;
#12262=CARTESIAN_POINT ( 'NONE',  ( -1.655278471874999990, 20.36702641396248481, -29.01827246956613493 ) ) ;
#12263=CARTESIAN_POINT ( 'NONE',  ( 1.655278471875001101, 20.36702641396249192, -95.18493913623279923 ) ) ;
#12264=CARTESIAN_POINT ( 'NONE',  ( 3.500000000000001776, 19.52072594216370405, -27.07139747004409713 ) ) ;
#12265=ORIENTED_EDGE ( 'NONE', *, *, #11068, .T. ) ;
#12268=CARTESIAN_POINT ( 'NONE',  ( -7.022189441860112050E-16, 13.67729811471672718, -133.6016058028994564 ) ) ;
#12272=CYLINDRICAL_SURFACE ( 'NONE', #8449, 3.499999999999999556 ) ;
#12273=CARTESIAN_POINT ( 'NONE',  ( -3.500000000000001332, 17.50000000000001776, -80.65473080337743284 ) ) ;
#12274=CARTESIAN_POINT ( 'NONE',  ( -7.022189441860112050E-16, 13.67729811471672186, -63.60160580289946353 ) ) ;
#12277=DIRECTION ( 'NONE',  ( 0.000000000000000000, 1.000000000000000000, 0.000000000000000000 ) ) ;
#12278=CARTESIAN_POINT ( 'NONE',  ( -3.310556943750001313, 17.50000000000001776, -89.85160580289947063 ) ) ;
#12281=CARTESIAN_POINT ( 'NONE',  ( 1.655278471874998436, 14.63297358603754894, -116.4307724695661364 ) ) ;
#12282=CARTESIAN_POINT ( 'NONE',  ( 0.9378221735089281585, 14.00000000000000888, -34.66632260368299256 ) ) ;
#12284=ORIENTED_EDGE ( 'NONE', *, *, #20670, .T. ) ;
#12285=CARTESIAN_POINT ( 'NONE',  ( -7.424026671074350129E-16, 13.45854811567263809, -107.4047308033774186 ) ) ;
#12286=CARTESIAN_POINT ( 'NONE',  ( -4.299564228933483745E-15, 21.00000000000002842, -140.2109808024215170 ) ) ;
#12287=CARTESIAN_POINT ( 'NONE',  ( -3.500000000000000000, 19.52072594216370760, -68.04431413575484555 ) ) ;
#12289=CARTESIAN_POINT ( 'NONE',  ( -3.500000000000001332, 17.50000000000001066, -32.65473080337742573 ) ) ;
#12291=CARTESIAN_POINT ( 'NONE',  ( -7.022189441860112050E-16, 13.67729811471672186, -66.51410580289947916 ) ) ;
#12292=LINE ( 'NONE', #11658, #21976 ) ;
#12296=ORIENTED_EDGE ( 'NONE', *, *, #17839, .T. ) ;
#12297=CARTESIAN_POINT ( 'NONE',  ( -1.394453263437886604E-15, 14.00000000000002132, -132.7109808024214885 ) ) ;
#12298=CARTESIAN_POINT ( 'NONE',  ( -3.500000000000002220, 15.47927405783632082, -31.87764746908818125 ) ) ;
#12299=CARTESIAN_POINT ( 'NONE',  ( 3.310556943750001313, 19.41135094264166483, -77.18077246956613635 ) ) ;
#12302=ORIENTED_EDGE ( 'NONE', *, *, #35828, .T. ) ;
#12305=( BOUNDED_CURVE ( )  B_SPLINE_CURVE ( 2, ( #2871, #40738, #19036, #2658, #18620, #18406, #18198, #2026, #11594 ),
 .UNSPECIFIED., .F., .F. ) 
 B_SPLINE_CURVE_WITH_KNOTS ( ( 3, 2, 2, 2, 3 ),
 ( 0.8437500000000000000, 0.8444444444444444420, 0.8458333333333333259, 0.8472222222222222099, 0.8479166666666666519 ),
 .UNSPECIFIED. ) 
 CURVE ( )  GEOMETRIC_REPRESENTATION_ITEM ( )  RATIONAL_B_SPLINE_CURVE ( ( 0.9330127018922194093, 0.9330127018922194093, 1.000000000000000000, 0.8660254037844387076, 1.000000000000000000, 0.8660254037844387076, 1.000000000000000000, 0.9330127018922194093, 0.9330127018922194093 ) ) 
 REPRESENTATION_ITEM ( '' )  );
#12309=CARTESIAN_POINT ( 'NONE',  ( 1.655278471875001101, 20.36702641396248481, -41.18493913623279212 ) ) ;
#12310=CARTESIAN_POINT ( 'NONE',  ( -3.310556943750001313, 17.50000000000002132, -107.8516058028994564 ) ) ;
#12311=VERTEX_POINT ( 'NONE', #2764 ) ;
#12314=CARTESIAN_POINT ( 'NONE',  ( -7.022189441860112050E-16, 13.67729811471671475, -32.51410580289946495 ) ) ;
#12315=CARTESIAN_POINT ( 'NONE',  ( -1.655278471875002211, 14.63297358603754361, -61.68493913623279923 ) ) ;
#12316=CARTESIAN_POINT ( 'NONE',  ( -7.424026671074350129E-16, 13.45854811567263809, -108.7109808024215027 ) ) ;
#12318=CARTESIAN_POINT ( 'NONE',  ( 1.655278471874998436, 14.63297358603754539, -93.43077246956613635 ) ) ;
#12319=CARTESIAN_POINT ( 'NONE',  ( 3.500000000000001332, 17.50000000000001776, -98.15473080337743284 ) ) ;
#12323=CARTESIAN_POINT ( 'NONE',  ( 3.500000000000000000, 15.47927405783632260, -57.54431413575484555 ) ) ;
#12324=CARTESIAN_POINT ( 'NONE',  ( -3.310556943750001313, 17.50000000000001066, -28.76410580289948271 ) ) ;
#12326=CARTESIAN_POINT ( 'NONE',  ( -7.424026671074350129E-16, 13.45854811567263276, -50.40473080337742573 ) ) ;
#12327=CARTESIAN_POINT ( 'NONE',  ( 4.648177544792955347E-16, 21.00000000000001066, -46.21098080242150274 ) ) ;
#12328=CARTESIAN_POINT ( 'NONE',  ( 1.655278471874998436, 14.63297358603754716, -108.5182724695661420 ) ) ;
#12329=CARTESIAN_POINT ( 'NONE',  ( 1.655278471874998436, 14.63297358603753828, -34.51827246956614204 ) ) ;
#12332=CARTESIAN_POINT ( 'NONE',  ( 4.648177544792955347E-16, 21.00000000000002487, -140.9047308033773902 ) ) ;
#12336=CARTESIAN_POINT ( 'NONE',  ( -3.310556943750002201, 15.58864905735837247, -89.68077246956613635 ) ) ;
#12337=EDGE_LOOP ( 'NONE', ( #2817, #17651, #12943, #16757 ) ) ;
#12339=VERTEX_POINT ( 'NONE', #38707 ) ;
#12340=CARTESIAN_POINT ( 'NONE',  ( -1.394453263437886604E-15, 14.00000000000001776, -101.7109808024215027 ) ) ;
#12341=CARTESIAN_POINT ( 'NONE',  ( 3.500000000000001332, 19.52072594216371826, -109.3776474690881741 ) ) ;
#12342=ORIENTED_EDGE ( 'NONE', *, *, #32293, .T. ) ;
#12344=ADVANCED_FACE ( 'NONE', ( #22535 ), #25954, .T. ) ;
#12346=CARTESIAN_POINT ( 'NONE',  ( -7.022189441860112050E-16, 13.67729811471672363, -94.51410580289946495 ) ) ;
#12348=EDGE_CURVE ( 'NONE', #41707, #31249, #22327, .T. ) ;
#12349=ORIENTED_EDGE ( 'NONE', *, *, #35204, .F. ) ;
#12350=CARTESIAN_POINT ( 'NONE',  ( 3.500000000000001332, 17.50000000000002132, -121.1547308033774328 ) ) ;
#12352=CARTESIAN_POINT ( 'NONE',  ( 3.500000000000001332, 17.50000000000002487, -139.4609808024214885 ) ) ;
#12358=ORIENTED_EDGE ( 'NONE', *, *, #1948, .F. ) ;
#12360=( BOUNDED_CURVE ( )  B_SPLINE_CURVE ( 2, ( #17443, #33809, #40598, #24445, #1477, #37412, #8270, #21245, #14452 ),
 .UNSPECIFIED., .F., .T. ) 
 B_SPLINE_CURVE_WITH_KNOTS ( ( 3, 2, 2, 2, 3 ),
 ( 0.3854166666666666852, 0.3861111111111111271, 0.3875000000000000111, 0.3888888888888888951, 0.3895833333333333370 ),
 .UNSPECIFIED. ) 
 CURVE ( )  GEOMETRIC_REPRESENTATION_ITEM ( )  RATIONAL_B_SPLINE_CURVE ( ( 0.9330127018922194093, 0.9330127018922194093, 1.000000000000000000, 0.8660254037844387076, 1.000000000000000000, 0.8660254037844387076, 1.000000000000000000, 0.9330127018922194093, 0.9330127018922194093 ) ) 
 REPRESENTATION_ITEM ( '' )  );
#12361=VECTOR ( 'NONE', #13346, 1000.000000000000000 ) ;
#12363=CARTESIAN_POINT ( 'NONE',  ( -1.655278471875002211, 14.63297358603755249, -129.5974391362328220 ) ) ;
#12365=ORIENTED_EDGE ( 'NONE', *, *, #39217, .T. ) ;
#12366=CARTESIAN_POINT ( 'NONE',  ( 4.648177544792955347E-16, 21.00000000000001066, -31.90473080337742573 ) ) ;
#12367=CARTESIAN_POINT ( 'NONE',  ( -1.655278471875002211, 14.63297358603755249, -126.6849391362327992 ) ) ;
#12368=CARTESIAN_POINT ( 'NONE',  ( 3.310556943750001313, 17.50000000000001421, -49.35160580289946353 ) ) ;
#12370=CARTESIAN_POINT ( 'NONE',  ( -1.750000000000002220, 14.46891108675448834, -135.4880641367107614 ) ) ;
#12372=CARTESIAN_POINT ( 'NONE',  ( -3.310556943750002645, 15.58864905735837070, -79.76827246956612782 ) ) ;
#12373=CARTESIAN_POINT ( 'NONE',  ( 1.749999999999998224, 14.46891108675448656, -124.6276474690881599 ) ) ;
#12374=CARTESIAN_POINT ( 'NONE',  ( -3.310556943750000425, 19.41135094264166838, -106.8474391362327935 ) ) ;
#12376=CARTESIAN_POINT ( 'NONE',  ( -0.9378221735089310451, 14.00000000000002132, -107.4493890021159501 ) ) ;
#12378=AXIS2_PLACEMENT_3D ( 'NONE', #16852, #30964, #25211 ) ;
#12380=CARTESIAN_POINT ( 'NONE',  ( 3.500000000000000000, 15.47927405783632437, -77.54431413575484555 ) ) ;
#12382=CARTESIAN_POINT ( 'NONE',  ( -1.655278471874999990, 20.36702641396248481, -43.93077246956614346 ) ) ;
#12383=CARTESIAN_POINT ( 'NONE',  ( 1.655278471875001101, 20.36702641396249547, -103.1849391362327992 ) ) ;
#12384=CARTESIAN_POINT ( 'NONE',  ( -1.394453263437886604E-15, 14.00000000000002132, -113.7109808024214743 ) ) ;
#12385=CARTESIAN_POINT ( 'NONE',  ( -3.500000000000000888, 19.52072594216370760, -62.73806413671076143 ) ) ;
#12386=FACE_OUTER_BOUND ( 'NONE', #10682, .T. ) ;
#12387=EDGE_CURVE ( 'NONE', #39176, #644, #35480, .T. ) ;
#12389=CARTESIAN_POINT ( 'NONE',  ( -3.310556943750001313, 17.50000000000002132, -122.8516058028994564 ) ) ;
#12390=CARTESIAN_POINT ( 'NONE',  ( -3.500000000000002220, 15.47927405783632082, -27.87764746908817770 ) ) ;
#12393=CARTESIAN_POINT ( 'NONE',  ( 1.750000000000001110, 20.53108891324555074, -60.29431413575483845 ) ) ;
#12394=CYLINDRICAL_SURFACE ( 'NONE', #936, 3.499999999999999556 ) ;
#12397=CARTESIAN_POINT ( 'NONE',  ( -1.655278471875002211, 14.63297358603754539, -76.68493913623279923 ) ) ;
#12399=CARTESIAN_POINT ( 'NONE',  ( 3.500000000000000000, 15.47927405783632082, -40.23806413671076143 ) ) ;
#12403=CARTESIAN_POINT ( 'NONE',  ( 3.310556943750001313, 17.50000000000001066, -32.26410580289947205 ) ) ;
#12404=ADVANCED_FACE ( 'NONE', ( #39761 ), #40180, .T. ) ;
#12405=EDGE_CURVE ( 'NONE', #21195, #21956, #20573, .T. ) ;
#12408=ORIENTED_EDGE ( 'NONE', *, *, #25232, .F. ) ;
#12411=ORIENTED_EDGE ( 'NONE', *, *, #37306, .F. ) ;
#12412=AXIS2_PLACEMENT_3D ( 'NONE', #30302, #1797, #17961 ) ;
#12415=CARTESIAN_POINT ( 'NONE',  ( 3.500000000000000000, 15.47927405783632793, -90.54431413575484555 ) ) ;
#12417=CARTESIAN_POINT ( 'NONE',  ( 0.9378221735089300459, 21.00000000000001776, -97.25563900116004845 ) ) ;
#12419=CARTESIAN_POINT ( 'NONE',  ( -3.500000000000002220, 15.47927405783632082, -32.87764746908818125 ) ) ;
#12422=PLANE ( 'NONE',  #7427 ) ;
#12423=CYLINDRICAL_SURFACE ( 'NONE', #11885, 3.499999999999999556 ) ;
#12425=CARTESIAN_POINT ( 'NONE',  ( 1.749999999999998224, 14.46891108675448834, -138.6276474690881741 ) ) ;
#12427=CARTESIAN_POINT ( 'NONE',  ( 1.655278471875001101, 20.36702641396249547, -122.0974391362328078 ) ) ;
#12430=CARTESIAN_POINT ( 'NONE',  ( -3.500000000000000000, 19.52072594216371115, -76.73806413671076143 ) ) ;
#12431=CARTESIAN_POINT ( 'NONE',  ( -1.749999999999999778, 20.53108891324555429, -99.12764746908817415 ) ) ;
#12432=EDGE_CURVE ( 'NONE', #31404, #4823, #38200, .T. ) ;
#12433=CARTESIAN_POINT ( 'NONE',  ( -1.655278471875002211, 14.63297358603755072, -115.6849391362327850 ) ) ;
#12435=CARTESIAN_POINT ( 'NONE',  ( 1.749999999999998224, 14.46891108675447413, -30.32139747004410069 ) ) ;
#12436=CYLINDRICAL_SURFACE ( 'NONE', #36918, 3.499999999999999556 ) ;
#12438=EDGE_CURVE ( 'NONE', #217, #39932, #14855, .T. ) ;
#12439=CARTESIAN_POINT ( 'NONE',  ( 3.310556943750001313, 17.50000000000002487, -139.3516058028994564 ) ) ;
#12440=VECTOR ( 'NONE', #14030, 1000.000000000000000 ) ;
#12442=DIRECTION ( 'NONE',  ( -0.000000000000000000, 1.259100132267607459E-16, -1.000000000000000000 ) ) ;
#12443=CARTESIAN_POINT ( 'NONE',  ( 3.310556943750001313, 17.50000000000001066, -46.35160580289945642 ) ) ;
#12445=CARTESIAN_POINT ( 'NONE',  ( -3.500000000000001332, 17.50000000000002132, -114.6547308033774328 ) ) ;
#12446=VECTOR ( 'NONE', #29563, 1000.000000000000000 ) ;
#12447=CARTESIAN_POINT ( 'NONE',  ( -3.310556943750001313, 17.50000000000001421, -71.85160580289947063 ) ) ;
#12449=CARTESIAN_POINT ( 'NONE',  ( -7.022189441860112050E-16, 13.67729811471672186, -70.51410580289947916 ) ) ;
#12451=CARTESIAN_POINT ( 'NONE',  ( 1.655278471874998436, 14.63297358603754539, -91.51827246956612782 ) ) ;
#12454=CARTESIAN_POINT ( 'NONE',  ( -1.394453263437886604E-15, 14.00000000000002132, -112.4047308033774186 ) ) ;
#12456=CARTESIAN_POINT ( 'NONE',  ( 4.648177544792955347E-16, 21.00000000000001066, -42.21098080242150274 ) ) ;
#12457=CARTESIAN_POINT ( 'NONE',  ( -1.655278471875002211, 14.63297358603754184, -50.59743913623280775 ) ) ;
#12458=CARTESIAN_POINT ( 'NONE',  ( -8.715332896486792803E-15, 21.00000000000002842, -137.9047308033774186 ) ) ;
#12459=CARTESIAN_POINT ( 'NONE',  ( 1.655278471874998436, 14.63297358603754716, -107.4307724695661506 ) ) ;
#12460=CARTESIAN_POINT ( 'NONE',  ( 4.648177544792955347E-16, 21.00000000000001066, -36.21098080242150985 ) ) ;
#12462=VERTEX_POINT ( 'NONE', #20621 ) ;
#12464=VERTEX_POINT ( 'NONE', #33600 ) ;
#12466=CARTESIAN_POINT ( 'NONE',  ( -1.655278471874999990, 20.36702641396248836, -61.93077246956614346 ) ) ;
#12468=VERTEX_POINT ( 'NONE', #4459 ) ;
#12475=CARTESIAN_POINT ( 'NONE',  ( 2.340729813953370519E-16, 21.32270188528331900, -127.0141058028994507 ) ) ;
#12477=CARTESIAN_POINT ( 'NONE',  ( 3.310556943750001313, 17.50000000000001066, -32.35160580289946353 ) ) ;
#12478=EDGE_CURVE ( 'NONE', #17447, #25980, #18075, .T. ) ;
#12479=CARTESIAN_POINT ( 'NONE',  ( -7.022189441860112050E-16, 13.67729811471671475, -26.60160580289946708 ) ) ;
#12480=CARTESIAN_POINT ( 'NONE',  ( -7.022189441860112050E-16, 13.67729811471672363, -88.60160580289947063 ) ) ;
#12481=CARTESIAN_POINT ( 'NONE',  ( -3.310556943750001313, 17.50000000000002487, -137.7641058028994792 ) ) ;
#12484=( BOUNDED_CURVE ( )  B_SPLINE_CURVE ( 2, ( #10099, #29437, #36462, #12873, #29026, #16694, #19255, #38817, #29650 ),
 .UNSPECIFIED., .F., .F. ) 
 B_SPLINE_CURVE_WITH_KNOTS ( ( 3, 2, 2, 2, 3 ),
 ( 0.8604166666666667185, 0.8611111111111111605, 0.8625000000000000444, 0.8638888888888889284, 0.8645833333333333703 ),
 .UNSPECIFIED. ) 
 CURVE ( )  GEOMETRIC_REPRESENTATION_ITEM ( )  RATIONAL_B_SPLINE_CURVE ( ( 0.9330127018922194093, 0.9330127018922194093, 1.000000000000000000, 0.8660254037844387076, 1.000000000000000000, 0.8660254037844387076, 1.000000000000000000, 0.9330127018922194093, 0.9330127018922194093 ) ) 
 REPRESENTATION_ITEM ( '' )  );
#12485=CARTESIAN_POINT ( 'NONE',  ( -1.655278471874999990, 20.36702641396249902, -134.0182724695661420 ) ) ;
#12488=CARTESIAN_POINT ( 'NONE',  ( -0.9378221735089291577, 21.00000000000001776, -76.16632260368297125 ) ) ;
#12490=CARTESIAN_POINT ( 'NONE',  ( 3.500000000000001776, 19.52072594216371115, -78.07139747004410424 ) ) ;
#12491=CARTESIAN_POINT ( 'NONE',  ( -3.310556943750002201, 15.58864905735836892, -62.76827246956613493 ) ) ;
#12494=CARTESIAN_POINT ( 'NONE',  ( 4.286263797015737581E-16, 14.00000000000002487, -149.5231586289125687 ) ) ;
#12495=CARTESIAN_POINT ( 'NONE',  ( 3.310556943749999981, 15.58864905735836892, -86.43493913623279923 ) ) ;
#12497=CARTESIAN_POINT ( 'NONE',  ( -3.310556943750000425, 19.41135094264166838, -112.8474391362328078 ) ) ;
#12499=ORIENTED_EDGE ( 'NONE', *, *, #22321, .T. ) ;
#12500=( BOUNDED_CURVE ( )  B_SPLINE_CURVE ( 2, ( #40588, #1261, #14230, #30390, #30178, #40796, #24024, #17837, #11445 ),
 .UNSPECIFIED., .F., .T. ) 
 B_SPLINE_CURVE_WITH_KNOTS ( ( 3, 2, 2, 2, 3 ),
 ( 0.3312499999999999889, 0.3319444444444444309, 0.3333333333333333148, 0.3347222222222221988, 0.3354166666666666963 ),
 .UNSPECIFIED. ) 
 CURVE ( )  GEOMETRIC_REPRESENTATION_ITEM ( )  RATIONAL_B_SPLINE_CURVE ( ( 0.9330127018922194093, 0.9330127018922194093, 1.000000000000000000, 0.8660254037844387076, 1.000000000000000000, 0.8660254037844387076, 1.000000000000000000, 0.9330127018922167448, 0.9330127018922194093 ) ) 
 REPRESENTATION_ITEM ( '' )  );
#12501=CARTESIAN_POINT ( 'NONE',  ( 1.749999999999998224, 14.46891108675448478, -109.3213974700441042 ) ) ;
#12506=CARTESIAN_POINT ( 'NONE',  ( -0.9378221735089310451, 14.00000000000001599, -67.75563900116002003 ) ) ;
#12507=CARTESIAN_POINT ( 'NONE',  ( -3.500000000000001332, 17.50000000000001066, -26.96098080242151340 ) ) ;
#12511=CARTESIAN_POINT ( 'NONE',  ( -3.310556943750002201, 15.58864905735836892, -64.68077246956615056 ) ) ;
#12513=CARTESIAN_POINT ( 'NONE',  ( 0.000000000000000000, 17.50000000000002487, -149.5231586289125687 ) ) ;
#12515=ORIENTED_EDGE ( 'NONE', *, *, #11895, .T. ) ;
#12516=MECHANICAL_DESIGN_GEOMETRIC_PRESENTATION_REPRESENTATION('',(#17947),#8436);
#12519=CARTESIAN_POINT ( 'NONE',  ( -3.310556943750002645, 15.58864905735837247, -81.68077246956616477 ) ) ;
#12520=VERTEX_POINT ( 'NONE', #37821 ) ;
#12522=CARTESIAN_POINT ( 'NONE',  ( -1.750000000000002220, 14.46891108675448834, -127.7943141357548456 ) ) ;
#12523=CARTESIAN_POINT ( 'NONE',  ( -3.310556943750001313, 17.50000000000002487, -138.7641058028994792 ) ) ;
#12527=CARTESIAN_POINT ( 'NONE',  ( 3.310556943750001313, 17.50000000000001066, -43.35160580289947063 ) ) ;
#12528=CARTESIAN_POINT ( 'NONE',  ( -3.310556943750000425, 19.41135094264166838, -104.9349391362327992 ) ) ;
#12529=ORIENTED_EDGE ( 'NONE', *, *, #6136, .F. ) ;
#12530=CARTESIAN_POINT ( 'NONE',  ( 1.655278471874998436, 14.63297358603753828, -29.43077246956614346 ) ) ;
#12531=CARTESIAN_POINT ( 'NONE',  ( -1.655278471874999990, 20.36702641396248836, -61.01827246956613493 ) ) ;
#12532=CARTESIAN_POINT ( 'NONE',  ( -3.500000000000002220, 15.47927405783632970, -108.8776474690881741 ) ) ;
#12534=CARTESIAN_POINT ( 'NONE',  ( 3.500000000000001776, 19.52072594216371115, -97.07139747004409003 ) ) ;
#12538=CARTESIAN_POINT ( 'NONE',  ( -7.424026671074350129E-16, 13.45854811567263454, -56.71098080242151696 ) ) ;
#12540=CARTESIAN_POINT ( 'NONE',  ( 3.310556943749999981, 15.58864905735836004, -24.34743913623281486 ) ) ;
#12541=CARTESIAN_POINT ( 'NONE',  ( 3.500000000000000000, 15.47927405783632082, -46.23806413671076143 ) ) ;
#12542=CARTESIAN_POINT ( 'NONE',  ( 1.750000000000001110, 20.53108891324555429, -77.29431413575484555 ) ) ;
#12543=CARTESIAN_POINT ( 'NONE',  ( 2.340729813953370519E-16, 21.32270188528330834, -35.10160580289946353 ) ) ;
#12546=CYLINDRICAL_SURFACE ( 'NONE', #4711, 3.499999999999999556 ) ;
#12550=CARTESIAN_POINT ( 'NONE',  ( 3.310556943750001313, 19.41135094264166838, -80.18077246956613635 ) ) ;
#12551=CARTESIAN_POINT ( 'NONE',  ( 0.000000000000000000, 17.50000000000002487, -149.5231586289125687 ) ) ;
#12552=ORIENTED_EDGE ( 'NONE', *, *, #41264, .F. ) ;
#12556=ORIENTED_EDGE ( 'NONE', *, *, #1440, .T. ) ;
#12559=CARTESIAN_POINT ( 'NONE',  ( -1.655278471875002211, 14.63297358603754894, -96.59743913623280775 ) ) ;
#12563=CARTESIAN_POINT ( 'NONE',  ( -0.9378221735089310451, 14.00000000000001599, -78.44938900211596433 ) ) ;
#12572=CARTESIAN_POINT ( 'NONE',  ( -1.749999999999999778, 20.53108891324555785, -127.8213974700440900 ) ) ;
#12574=CARTESIAN_POINT ( 'NONE',  ( -1.655278471874999990, 20.36702641396249902, -130.9307724695661364 ) ) ;
#12578=CARTESIAN_POINT ( 'NONE',  ( 2.340729813953370519E-16, 21.32270188528331900, -126.1016058028994706 ) ) ;
#12579=CARTESIAN_POINT ( 'NONE',  ( -1.655278471874999990, 20.36702641396248836, -51.01827246956612782 ) ) ;
#12581=CARTESIAN_POINT ( 'NONE',  ( 3.500000000000001776, 19.52072594216371826, -128.0713974700441042 ) ) ;
#12584=CARTESIAN_POINT ( 'NONE',  ( -3.310556943750001313, 17.50000000000001776, -77.85160580289945642 ) ) ;
#12585=CARTESIAN_POINT ( 'NONE',  ( -1.749999999999999778, 20.53108891324555785, -123.1276474690881741 ) ) ;
#12586=CARTESIAN_POINT ( 'NONE',  ( 1.655278471875001101, 20.36702641396249547, -107.0974391362328078 ) ) ;
#12588=CARTESIAN_POINT ( 'NONE',  ( 0.9378221735089300459, 21.00000000000001776, -80.94938900211593591 ) ) ;
#12591=CARTESIAN_POINT ( 'NONE',  ( -7.424026671074350129E-16, 13.45854811567263454, -73.71098080242151696 ) ) ;
#12592=CARTESIAN_POINT ( 'NONE',  ( -1.749999999999999778, 20.53108891324555074, -51.12764746908816704 ) ) ;
#12593=CARTESIAN_POINT ( 'NONE',  ( -3.310556943750002645, 15.58864905735836714, -44.68077246956615056 ) ) ;
#12595=CARTESIAN_POINT ( 'NONE',  ( -7.022189441860112050E-16, 13.67729811471672541, -99.60160580289947063 ) ) ;
#12597=CARTESIAN_POINT ( 'NONE',  ( -7.424026671074350129E-16, 13.45854811567263454, -66.40473080337743284 ) ) ;
#12598=CARTESIAN_POINT ( 'NONE',  ( -1.394453263437886604E-15, 14.00000000000000711, -25.71098080242150630 ) ) ;
#12601=CARTESIAN_POINT ( 'NONE',  ( 1.655278471874998436, 14.63297358603754894, -119.5182724695661278 ) ) ;
#12602=CARTESIAN_POINT ( 'NONE',  ( -3.500000000000000000, 19.52072594216371115, -92.04431413575484555 ) ) ;
#12606=CARTESIAN_POINT ( 'NONE',  ( 3.500000000000000000, 15.47927405783632970, -107.5443141357548456 ) ) ;
#12610=CARTESIAN_POINT ( 'NONE',  ( -1.655278471874999990, 20.36702641396249192, -76.01827246956612782 ) ) ;
#12611=DIRECTION ( 'NONE',  ( -0.000000000000000000, 1.259100132267607459E-16, -1.000000000000000000 ) ) ;
#12616=CARTESIAN_POINT ( 'NONE',  ( 1.655278471875001101, 20.36702641396248481, -36.09743913623281486 ) ) ;
#12618=CARTESIAN_POINT ( 'NONE',  ( 4.648177544792955347E-16, 21.00000000000001421, -71.90473080337743284 ) ) ;
#12619=( BOUNDED_CURVE ( )  B_SPLINE_CURVE ( 2, ( #41850, #6529, #3530, #3332, #25255, #12702, #29261, #38221, #38437 ),
 .UNSPECIFIED., .F., .T. ) 
 B_SPLINE_CURVE_WITH_KNOTS ( ( 3, 2, 2, 2, 3 ),
 ( 0.9562500000000000444, 0.9569444444444444864, 0.9583333333333333703, 0.9597222222222222543, 0.9604166666666666963 ),
 .UNSPECIFIED. ) 
 CURVE ( )  GEOMETRIC_REPRESENTATION_ITEM ( )  RATIONAL_B_SPLINE_CURVE ( ( 0.9330127018922194093, 0.9330127018922194093, 1.000000000000000000, 0.8660254037844387076, 1.000000000000000000, 0.8660254037844387076, 1.000000000000000000, 0.9330127018922194093, 0.9330127018922194093 ) ) 
 REPRESENTATION_ITEM ( '' )  );
#12624=DIRECTION ( 'NONE',  ( -0.000000000000000000, 1.259100132267607459E-16, -1.000000000000000000 ) ) ;
#12629=CYLINDRICAL_SURFACE ( 'NONE', #34024, 3.499999999999999556 ) ;
#12630=CARTESIAN_POINT ( 'NONE',  ( 3.500000000000001776, 19.52072594216371826, -117.0713974700441042 ) ) ;
#12632=CARTESIAN_POINT ( 'NONE',  ( 2.474675557024783212E-16, 21.54145188432739033, -31.21098080242150274 ) ) ;
#12633=LINE ( 'NONE', #25196, #25982 ) ;
#12634=LINE ( 'NONE', #39399, #15624 ) ;
#12635=CARTESIAN_POINT ( 'NONE',  ( -1.394453263437886604E-15, 14.00000000000002132, -118.7109808024215170 ) ) ;
#12637=CARTESIAN_POINT ( 'NONE',  ( 3.500000000000001332, 17.50000000000002487, -136.4609808024214885 ) ) ;
#12639=CARTESIAN_POINT ( 'NONE',  ( -3.310556943750002645, 15.58864905735837780, -124.6807724695661364 ) ) ;
#12642=EDGE_CURVE ( 'NONE', #24771, #16447, #2050, .T. ) ;
#12645=CARTESIAN_POINT ( 'NONE',  ( 3.500000000000000000, 15.47927405783632615, -91.54431413575483134 ) ) ;
#12647=CARTESIAN_POINT ( 'NONE',  ( -1.655278471875002211, 14.63297358603754361, -59.59743913623280775 ) ) ;
#12649=CARTESIAN_POINT ( 'NONE',  ( 1.655278471875001101, 20.36702641396249547, -119.1849391362327992 ) ) ;
#12650=CARTESIAN_POINT ( 'NONE',  ( 0.000000000000000000, 17.50000000000002487, -149.5231586289125687 ) ) ;
#12651=CARTESIAN_POINT ( 'NONE',  ( -3.500000000000001332, 17.50000000000001066, -32.65473080337742573 ) ) ;
#12652=DIRECTION ( 'NONE',  ( -0.000000000000000000, 1.259100132267607459E-16, -1.000000000000000000 ) ) ;
#12654=CARTESIAN_POINT ( 'NONE',  ( -1.655278471874999990, 20.36702641396249902, -137.0182724695661420 ) ) ;
#12656=CARTESIAN_POINT ( 'NONE',  ( 3.500000000000000000, 15.47927405783633503, -138.2380641367107614 ) ) ;
#12657=CARTESIAN_POINT ( 'NONE',  ( -3.310556943750000425, 19.41135094264166483, -49.93493913623279923 ) ) ;
#12660=CARTESIAN_POINT ( 'NONE',  ( 3.310556943749999981, 15.58864905735836714, -69.43493913623279923 ) ) ;
#12662=CARTESIAN_POINT ( 'NONE',  ( -1.655278471875002211, 14.63297358603754361, -65.59743913623280775 ) ) ;
#12664=CARTESIAN_POINT ( 'NONE',  ( -3.310556943750002201, 15.58864905735837247, -90.76827246956612782 ) ) ;
#12668=CARTESIAN_POINT ( 'NONE',  ( -1.749999999999999778, 20.53108891324555429, -85.12764746908817415 ) ) ;
#12669=CARTESIAN_POINT ( 'NONE',  ( -1.394453263437886604E-15, 14.00000000000002132, -131.7109808024214885 ) ) ;
#12670=CARTESIAN_POINT ( 'NONE',  ( -7.022189441860112050E-16, 13.67729811471671830, -52.51410580289947205 ) ) ;
#12672=CARTESIAN_POINT ( 'NONE',  ( -1.655278471875002211, 14.63297358603754894, -104.5974391362328078 ) ) ;
#12678=CARTESIAN_POINT ( 'NONE',  ( 2.340729813953370519E-16, 21.32270188528330834, -57.01410580289947916 ) ) ;
#12682=EDGE_CURVE ( 'NONE', #40441, #5189, #22418, .T. ) ;
#12683=CARTESIAN_POINT ( 'NONE',  ( -1.394453263437886604E-15, 14.00000000000001421, -55.71098080242150274 ) ) ;
#12685=EDGE_CURVE ( 'NONE', #38468, #1263, #21058, .T. ) ;
#12688=CARTESIAN_POINT ( 'NONE',  ( -3.310556943750000425, 19.41135094264166838, -125.8474391362328078 ) ) ;
#12691=CARTESIAN_POINT ( 'NONE',  ( -3.310556943750000425, 19.41135094264165772, -33.93493913623279923 ) ) ;
#12692=CARTESIAN_POINT ( 'NONE',  ( 3.310556943750001313, 17.50000000000001066, -27.35160580289947063 ) ) ;
#12694=CARTESIAN_POINT ( 'NONE',  ( 3.310556943750001313, 17.50000000000001776, -90.35160580289947063 ) ) ;
#12695=CARTESIAN_POINT ( 'NONE',  ( 3.310556943750001313, 19.41135094264167549, -139.1807724695661364 ) ) ;
#12700=CARTESIAN_POINT ( 'NONE',  ( 3.310556943749999981, 15.58864905735837425, -135.4349391362327992 ) ) ;
#12701=DIRECTION ( 'NONE',  ( -0.000000000000000000, 1.259100132267607459E-16, -1.000000000000000000 ) ) ;
#12702=CARTESIAN_POINT ( 'NONE',  ( 3.500000000000001332, 19.52072594216370405, -28.07139747004409713 ) ) ;
#12703=DIRECTION ( 'NONE',  ( -0.000000000000000000, 1.259100132267607459E-16, -1.000000000000000000 ) ) ;
#12705=CARTESIAN_POINT ( 'NONE',  ( -3.500000000000001332, 17.50000000000001776, -82.65473080337743284 ) ) ;
#12706=CARTESIAN_POINT ( 'NONE',  ( -7.022189441860112050E-16, 13.67729811471672186, -65.60160580289945642 ) ) ;
#12709=CARTESIAN_POINT ( 'NONE',  ( -3.500000000000002220, 15.47927405783632615, -58.57139747004409713 ) ) ;
#12710=CARTESIAN_POINT ( 'NONE',  ( -3.310556943750002645, 15.58864905735837247, -86.76827246956612782 ) ) ;
#12711=CARTESIAN_POINT ( 'NONE',  ( -1.394453263437886604E-15, 14.00000000000001421, -55.71098080242150274 ) ) ;
#12712=CARTESIAN_POINT ( 'NONE',  ( -1.655278471874999990, 20.36702641396249547, -115.9307724695661364 ) ) ;
#12716=CARTESIAN_POINT ( 'NONE',  ( 3.500000000000001776, 19.52072594216371826, -110.0713974700441042 ) ) ;
#12719=CARTESIAN_POINT ( 'NONE',  ( -3.500000000000002220, 15.47927405783632793, -67.87764746908817415 ) ) ;
#12720=LINE ( 'NONE', #19097, #25813 ) ;
#12721=CARTESIAN_POINT ( 'NONE',  ( 3.500000000000000000, 15.47927405783632437, -59.23806413671076854 ) ) ;
#12723=CARTESIAN_POINT ( 'NONE',  ( 3.310556943750001313, 17.50000000000001421, -68.26410580289947916 ) ) ;
#12725=CARTESIAN_POINT ( 'NONE',  ( 1.655278471874998436, 14.63297358603754894, -120.4307724695661364 ) ) ;
#12728=VERTEX_POINT ( 'NONE', #38455 ) ;
#12730=CARTESIAN_POINT ( 'NONE',  ( -1.655278471874999990, 20.36702641396248836, -73.93077246956613635 ) ) ;
#12732=ORIENTED_EDGE ( 'NONE', *, *, #9284, .F. ) ;
#12734=CARTESIAN_POINT ( 'NONE',  ( -1.655278471875002211, 14.63297358603755427, -141.5974391362327935 ) ) ;
#12736=( BOUNDED_CURVE ( )  B_SPLINE_CURVE ( 2, ( #35255, #2300, #25697, #12287, #41868, #12719, #5914, #12506, #25491 ),
 .UNSPECIFIED., .F., .F. ) 
 B_SPLINE_CURVE_WITH_KNOTS ( ( 3, 2, 2, 2, 3 ),
 ( 0.6270833333333333259, 0.6277777777777777679, 0.6291666666666666519, 0.6305555555555555358, 0.6312499999999999778 ),
 .UNSPECIFIED. ) 
 CURVE ( )  GEOMETRIC_REPRESENTATION_ITEM ( )  RATIONAL_B_SPLINE_CURVE ( ( 0.9330127018922194093, 0.9330127018922194093, 1.000000000000000000, 0.8660254037844387076, 1.000000000000000000, 0.8660254037844387076, 1.000000000000000000, 0.9330127018922194093, 0.9330127018922194093 ) ) 
 REPRESENTATION_ITEM ( '' )  );
#12737=CARTESIAN_POINT ( 'NONE',  ( 4.286263797015737581E-16, 14.00000000000002487, -149.5231586289125687 ) ) ;
#12738=CARTESIAN_POINT ( 'NONE',  ( -3.310556943750002645, 15.58864905735836714, -41.76827246956612782 ) ) ;
#12740=CARTESIAN_POINT ( 'NONE',  ( -3.310556943750002645, 15.58864905735837425, -101.7682724695661278 ) ) ;
#12742=CARTESIAN_POINT ( 'NONE',  ( 3.310556943750001313, 19.41135094264165772, -28.18077246956614346 ) ) ;
#12744=CARTESIAN_POINT ( 'NONE',  ( 3.500000000000000000, 15.47927405783632793, -108.5443141357548456 ) ) ;
#12747=CARTESIAN_POINT ( 'NONE',  ( -7.424026671074350129E-16, 13.45854811567263809, -95.40473080337743284 ) ) ;
#12751=CARTESIAN_POINT ( 'NONE',  ( -3.500000000000001332, 17.50000000000001421, -57.96098080242151696 ) ) ;
#12753=CARTESIAN_POINT ( 'NONE',  ( 3.310556943750001313, 17.50000000000001066, -24.26410580289947561 ) ) ;
#12754=CARTESIAN_POINT ( 'NONE',  ( 3.500000000000001332, 17.50000000000001421, -47.15473080337742573 ) ) ;
#12755=CARTESIAN_POINT ( 'NONE',  ( 0.000000000000000000, 17.50000000000002487, -149.5231586289125687 ) ) ;
#12756=CARTESIAN_POINT ( 'NONE',  ( -1.655278471874999990, 20.36702641396248481, -32.01827246956613493 ) ) ;
#12759=CARTESIAN_POINT ( 'NONE',  ( -1.749999999999999778, 20.53108891324556140, -142.1276474690881741 ) ) ;
#12763=CARTESIAN_POINT ( 'NONE',  ( -3.310556943750000425, 19.41135094264166838, -81.84743913623279354 ) ) ;
#12764=CARTESIAN_POINT ( 'NONE',  ( 1.749999999999998224, 14.46891108675447235, -23.32139747004409358 ) ) ;
#12765=ORIENTED_EDGE ( 'NONE', *, *, #30349, .F. ) ;
#12766=CYLINDRICAL_SURFACE ( 'NONE', #30163, 3.499999999999999556 ) ;
#12771=CARTESIAN_POINT ( 'NONE',  ( 3.310556943750001313, 17.50000000000001776, -94.26410580289947916 ) ) ;
#12773=CARTESIAN_POINT ( 'NONE',  ( -1.750000000000002220, 14.46891108675448123, -78.48806413671076143 ) ) ;
#12774=VERTEX_POINT ( 'NONE', #2935 ) ;
#12779=FACE_OUTER_BOUND ( 'NONE', #17057, .T. ) ;
#12780=CARTESIAN_POINT ( 'NONE',  ( 1.655278471875001101, 20.36702641396249902, -133.0974391362328220 ) ) ;
#12782=CARTESIAN_POINT ( 'NONE',  ( 4.648177544792955347E-16, 21.00000000000002487, -138.9047308033774186 ) ) ;
#12784=CARTESIAN_POINT ( 'NONE',  ( -3.310556943750002645, 15.58864905735837780, -118.7682724695661278 ) ) ;
#12785=CARTESIAN_POINT ( 'NONE',  ( -3.310556943750001313, 17.50000000000001421, -51.85160580289946353 ) ) ;
#12787=CARTESIAN_POINT ( 'NONE',  ( 1.749999999999998224, 14.46891108675448656, -130.3213974700441042 ) ) ;
#12790=CARTESIAN_POINT ( 'NONE',  ( -3.310556943750000425, 19.41135094264166128, -69.93493913623279923 ) ) ;
#12791=CARTESIAN_POINT ( 'NONE',  ( 1.750000000000001110, 20.53108891324555785, -121.2943141357548313 ) ) ;
#12792=CARTESIAN_POINT ( 'NONE',  ( -3.310556943750000425, 19.41135094264166838, -107.8474391362328078 ) ) ;
#12793=DIRECTION ( 'NONE',  ( 0.000000000000000000, 1.000000000000000000, 0.000000000000000000 ) ) ;
#12796=CARTESIAN_POINT ( 'NONE',  ( 1.750000000000001110, 20.53108891324555074, -74.29431413575483134 ) ) ;
#12798=CARTESIAN_POINT ( 'NONE',  ( -3.310556943750001313, 17.50000000000001066, -43.76410580289947916 ) ) ;
#12799=CARTESIAN_POINT ( 'NONE',  ( -3.310556943750002645, 15.58864905735837425, -103.7682724695661278 ) ) ;
#12801=CARTESIAN_POINT ( 'NONE',  ( -3.500000000000002220, 15.47927405783632437, -63.57139747004411134 ) ) ;
#12804=CARTESIAN_POINT ( 'NONE',  ( -7.022189441860112050E-16, 13.67729811471672896, -117.6016058028994564 ) ) ;
#12808=CARTESIAN_POINT ( 'NONE',  ( 0.9378221735089300459, 21.00000000000001066, -31.94938900211594657 ) ) ;
#12809=DIRECTION ( 'NONE',  ( -0.000000000000000000, 1.259100132267607459E-16, -1.000000000000000000 ) ) ;
#12810=CARTESIAN_POINT ( 'NONE',  ( 3.310556943749999981, 15.58864905735837070, -99.34743913623280775 ) ) ;
#12815=VERTEX_POINT ( 'NONE', #10939 ) ;
#12816=CARTESIAN_POINT ( 'NONE',  ( -1.750000000000002220, 14.46891108675448301, -87.48806413671076143 ) ) ;
#12817=CARTESIAN_POINT ( 'NONE',  ( -1.394453263437886604E-15, 14.00000000000002132, -118.4047308033774328 ) ) ;
#12818=CARTESIAN_POINT ( 'NONE',  ( 0.9378221735089281585, 14.00000000000001066, -40.36007260463890844 ) ) ;
#12822=CARTESIAN_POINT ( 'NONE',  ( 2.340729813953370519E-16, 21.32270188528330834, -34.01410580289947205 ) ) ;
#12825=VERTEX_POINT ( 'NONE', #30074 ) ;
#12827=CARTESIAN_POINT ( 'NONE',  ( -3.500000000000001332, 17.50000000000001776, -99.96098080242150274 ) ) ;
#12829=ORIENTED_EDGE ( 'NONE', *, *, #9903, .T. ) ;
#12830=LINE ( 'NONE', #32799, #33453 ) ;
#12831=CARTESIAN_POINT ( 'NONE',  ( 0.000000000000000000, 17.50000000000002487, -149.5231586289125687 ) ) ;
#12833=CARTESIAN_POINT ( 'NONE',  ( 4.648177544792955347E-16, 21.00000000000001066, -30.90473080337742928 ) ) ;
#12834=CARTESIAN_POINT ( 'NONE',  ( -7.424026671074350129E-16, 13.45854811567263987, -116.4047308033774328 ) ) ;
#12836=CARTESIAN_POINT ( 'NONE',  ( -7.022189441860112050E-16, 13.67729811471672718, -135.6016058028994564 ) ) ;
#12837=CARTESIAN_POINT ( 'NONE',  ( -3.500000000000001332, 17.50000000000001066, -31.96098080242150274 ) ) ;
#12839=CARTESIAN_POINT ( 'NONE',  ( -1.749999999999999778, 20.53108891324554719, -44.82139747004409713 ) ) ;
#12841=CARTESIAN_POINT ( 'NONE',  ( 1.749999999999998224, 14.46891108675447590, -41.62764746908817415 ) ) ;
#12843=CARTESIAN_POINT ( 'NONE',  ( 1.749999999999998224, 14.46891108675448834, -141.6276474690881741 ) ) ;
#12845=CARTESIAN_POINT ( 'NONE',  ( -3.310556943750002645, 15.58864905735837780, -125.6807724695661506 ) ) ;
#12848=EDGE_CURVE ( 'NONE', #39182, #25342, #29236, .T. ) ;
#12850=CARTESIAN_POINT ( 'NONE',  ( -7.424026671074350129E-16, 13.45854811567263631, -93.71098080242151696 ) ) ;
#12851=CARTESIAN_POINT ( 'NONE',  ( -0.9378221735089310451, 14.00000000000001066, -45.44938900211595012 ) ) ;
#12852=CARTESIAN_POINT ( 'NONE',  ( -3.310556943750001313, 17.50000000000001421, -56.76410580289947916 ) ) ;
#12854=CARTESIAN_POINT ( 'NONE',  ( 3.310556943750001313, 17.50000000000002132, -115.3516058028994706 ) ) ;
#12855=EDGE_CURVE ( 'NONE', #19734, #19419, #428, .T. ) ;
#12856=DIRECTION ( 'NONE',  ( -0.000000000000000000, 1.259100132267607459E-16, -1.000000000000000000 ) ) ;
#12857=CARTESIAN_POINT ( 'NONE',  ( 2.474675557024783212E-16, 21.54145188432739033, -31.90473080337742928 ) ) ;
#12858=CARTESIAN_POINT ( 'NONE',  ( -3.500000000000002220, 15.47927405783633326, -108.8776474690881741 ) ) ;
#12860=CARTESIAN_POINT ( 'NONE',  ( 2.340729813953370519E-16, 21.32270188528332255, -135.1016058028994564 ) ) ;
#12863=CARTESIAN_POINT ( 'NONE',  ( -1.655278471875002211, 14.63297358603754184, -40.68493913623279212 ) ) ;
#12864=CYLINDRICAL_SURFACE ( 'NONE', #16353, 3.499999999999999556 ) ;
#12865=CARTESIAN_POINT ( 'NONE',  ( -3.310556943750001313, 17.50000000000001421, -68.85160580289947063 ) ) ;
#12867=CARTESIAN_POINT ( 'NONE',  ( -3.310556943750001313, 17.50000000000001421, -66.76410580289947916 ) ) ;
#12869=( BOUNDED_CURVE ( )  B_SPLINE_CURVE ( 2, ( #12327, #25735, #28910, #41266, #22115, #34663, #12110, #28281, #2970 ),
 .UNSPECIFIED., .F., .T. ) 
 B_SPLINE_CURVE_WITH_KNOTS ( ( 3, 2, 2, 2, 3 ),
 ( 0.8104166666666666741, 0.8111111111111111160, 0.8125000000000000000, 0.8138888888888888840, 0.8145833333333333259 ),
 .UNSPECIFIED. ) 
 CURVE ( )  GEOMETRIC_REPRESENTATION_ITEM ( )  RATIONAL_B_SPLINE_CURVE ( ( 0.9330127018922194093, 0.9330127018922194093, 1.000000000000000000, 0.8660254037844387076, 1.000000000000000000, 0.8660254037844387076, 1.000000000000000000, 0.9330127018922194093, 0.9330127018922194093 ) ) 
 REPRESENTATION_ITEM ( '' )  );
#12870=CARTESIAN_POINT ( 'NONE',  ( -1.655278471874999990, 20.36702641396249192, -86.01827246956612782 ) ) ;
#12872=CARTESIAN_POINT ( 'NONE',  ( 0.000000000000000000, 17.50000000000002487, -149.5231586289125687 ) ) ;
#12873=CARTESIAN_POINT ( 'NONE',  ( -3.500000000000000000, 19.52072594216370405, -40.04431413575484555 ) ) ;
#12875=CARTESIAN_POINT ( 'NONE',  ( 3.310556943750001313, 19.41135094264166483, -48.18077246956614346 ) ) ;
#12876=ADVANCED_FACE ( 'NONE', ( #24338 ), #21137, .T. ) ;
#12878=CARTESIAN_POINT ( 'NONE',  ( -7.022189441860112050E-16, 13.67729811471672541, -104.5141058028994507 ) ) ;
#12879=CARTESIAN_POINT ( 'NONE',  ( 1.750000000000001110, 20.53108891324555429, -95.98806413671076143 ) ) ;
#12883=VERTEX_POINT ( 'NONE', #37725 ) ;
#12885=CARTESIAN_POINT ( 'NONE',  ( -3.310556943750000425, 19.41135094264166128, -58.84743913623280065 ) ) ;
#12889=VECTOR ( 'NONE', #6110, 1000.000000000000000 ) ;
#12890=CARTESIAN_POINT ( 'NONE',  ( 3.500000000000001332, 19.52072594216370760, -55.37764746908817415 ) ) ;
#12891=EDGE_CURVE ( 'NONE', #40713, #34834, #9384, .T. ) ;
#12894=ORIENTED_EDGE ( 'NONE', *, *, #19329, .T. ) ;
#12895=LINE ( 'NONE', #16304, #22156 ) ;
#12896=CARTESIAN_POINT ( 'NONE',  ( -3.310556943750000425, 19.41135094264166838, -122.8474391362328220 ) ) ;
#12897=LINE ( 'NONE', #542, #21675 ) ;
#12899=CARTESIAN_POINT ( 'NONE',  ( -3.310556943750000425, 19.41135094264165772, -34.93493913623279923 ) ) ;
#12900=CARTESIAN_POINT ( 'NONE',  ( 3.310556943749999981, 15.58864905735836182, -28.43493913623279212 ) ) ;
#12901=CARTESIAN_POINT ( 'NONE',  ( 2.340729813953370519E-16, 21.32270188528331190, -88.10160580289947063 ) ) ;
#12902=CARTESIAN_POINT ( 'NONE',  ( 3.310556943750001313, 17.50000000000002487, -137.2641058028994792 ) ) ;
#12905=CARTESIAN_POINT ( 'NONE',  ( -0.9378221735089291577, 21.00000000000001421, -67.16632260368298546 ) ) ;
#12907=CARTESIAN_POINT ( 'NONE',  ( 3.310556943750001313, 19.41135094264167549, -135.2682724695661420 ) ) ;
#12908=CARTESIAN_POINT ( 'NONE',  ( 0.000000000000000000, 17.50000000000002487, -149.5231586289125687 ) ) ;
#12910=DIRECTION ( 'NONE',  ( -0.000000000000000000, 1.259100132267607459E-16, -1.000000000000000000 ) ) ;
#12911=CARTESIAN_POINT ( 'NONE',  ( -1.394453263437886604E-15, 14.00000000000002132, -126.7109808024214885 ) ) ;
#12912=CARTESIAN_POINT ( 'NONE',  ( -7.424026671074350129E-16, 13.45854811567263454, -74.40473080337744705 ) ) ;
#12913=CARTESIAN_POINT ( 'NONE',  ( -3.310556943750000425, 19.41135094264166483, -59.93493913623279212 ) ) ;
#12916=CARTESIAN_POINT ( 'NONE',  ( -0.9378221735089310451, 14.00000000000002132, -90.75563900116003424 ) ) ;
#12917=CARTESIAN_POINT ( 'NONE',  ( 3.310556943750001313, 17.50000000000001776, -84.35160580289947063 ) ) ;
#12918=CARTESIAN_POINT ( 'NONE',  ( 2.340729813953370519E-16, 21.32270188528332255, -143.1016058028994564 ) ) ;
#12919=CARTESIAN_POINT ( 'NONE',  ( 1.655278471875001101, 20.36702641396249547, -114.0974391362327935 ) ) ;
#12920=CARTESIAN_POINT ( 'NONE',  ( 3.310556943750001313, 19.41135094264166483, -79.18077246956615056 ) ) ;
#12921=CARTESIAN_POINT ( 'NONE',  ( -1.394453263437886604E-15, 14.00000000000001066, -32.40473080337742573 ) ) ;
#12923=VECTOR ( 'NONE', #38513, 1000.000000000000000 ) ;
#12924=CARTESIAN_POINT ( 'NONE',  ( -7.424026671074350129E-16, 13.45854811567263809, -108.4047308033774328 ) ) ;
#12928=CARTESIAN_POINT ( 'NONE',  ( -1.750000000000002220, 14.46891108675448478, -95.48806413671076143 ) ) ;
#12930=CARTESIAN_POINT ( 'NONE',  ( 1.750000000000001110, 20.53108891324555074, -65.29431413575484555 ) ) ;
#12932=CARTESIAN_POINT ( 'NONE',  ( -7.022189441860112050E-16, 13.67729811471672186, -65.51410580289947916 ) ) ;
#12934=CARTESIAN_POINT ( 'NONE',  ( 2.340729813953370519E-16, 21.32270188528331900, -122.0141058028994792 ) ) ;
#12937=EDGE_LOOP ( 'NONE', ( #6194, #10112, #26134, #36811 ) ) ;
#12938=CARTESIAN_POINT ( 'NONE',  ( -1.749999999999999778, 20.53108891324554719, -43.12764746908817415 ) ) ;
#12940=CARTESIAN_POINT ( 'NONE',  ( -1.655278471875002211, 14.63297358603754539, -74.59743913623280775 ) ) ;
#12942=VERTEX_POINT ( 'NONE', #21970 ) ;
#12943=ORIENTED_EDGE ( 'NONE', *, *, #9555, .T. ) ;
#12944=CIRCLE ( 'NONE', #18370, 3.500000000000003109 ) ;
#12947=CARTESIAN_POINT ( 'NONE',  ( 2.340729813953370519E-16, 21.32270188528332255, -142.0141058028994792 ) ) ;
#12950=CARTESIAN_POINT ( 'NONE',  ( -1.655278471874999990, 20.36702641396248481, -41.01827246956612782 ) ) ;
#12951=CARTESIAN_POINT ( 'NONE',  ( 3.310556943750001313, 17.50000000000002132, -103.3516058028994564 ) ) ;
#12952=CARTESIAN_POINT ( 'NONE',  ( 3.310556943750001313, 19.41135094264165772, -29.18077246956613990 ) ) ;
#12953=CARTESIAN_POINT ( 'NONE',  ( -1.394453263437886604E-15, 14.00000000000002132, -111.7109808024214885 ) ) ;
#12954=CARTESIAN_POINT ( 'NONE',  ( -1.749999999999999778, 20.53108891324555785, -108.1276474690881741 ) ) ;
#12956=CYLINDRICAL_SURFACE ( 'NONE', #35635, 3.499999999999999556 ) ;
#12957=CARTESIAN_POINT ( 'NONE',  ( 1.749999999999998224, 14.46891108675448301, -95.32139747004409003 ) ) ;
#12958=DIRECTION ( 'NONE',  ( 0.000000000000000000, 1.000000000000000000, 0.000000000000000000 ) ) ;
#12961=CARTESIAN_POINT ( 'NONE',  ( 1.750000000000001110, 20.53108891324555074, -59.29431413575483845 ) ) ;
#12963=CARTESIAN_POINT ( 'NONE',  ( 4.648177544792955347E-16, 21.00000000000001066, -30.90473080337742928 ) ) ;
#12964=CARTESIAN_POINT ( 'NONE',  ( -0.9378221735089377065, 21.00000000000001421, -134.8600726046389013 ) ) ;
#12965=CARTESIAN_POINT ( 'NONE',  ( 3.500000000000001776, 19.52072594216370760, -48.07139747004410424 ) ) ;
#12967=EDGE_CURVE ( 'NONE', #3661, #11503, #24922, .T. ) ;
#12968=CARTESIAN_POINT ( 'NONE',  ( -1.655278471875002211, 14.63297358603754006, -34.68493913623279923 ) ) ;
#12971=CARTESIAN_POINT ( 'NONE',  ( -1.750000000000002220, 14.46891108675448656, -120.7943141357548313 ) ) ;
#12975=CARTESIAN_POINT ( 'NONE',  ( 3.310556943750001313, 17.50000000000001776, -84.26410580289947916 ) ) ;
#12976=CARTESIAN_POINT ( 'NONE',  ( 4.286263797015737581E-16, 14.00000000000002487, -149.5231586289125687 ) ) ;
#12978=CARTESIAN_POINT ( 'NONE',  ( -3.500000000000001332, 17.50000000000002132, -123.9609808024215027 ) ) ;
#12979=CARTESIAN_POINT ( 'NONE',  ( -1.394453263437886604E-15, 14.00000000000001421, -80.71098080242148853 ) ) ;
#12982=EDGE_CURVE ( 'NONE', #31031, #28716, #17836, .T. ) ;
#12984=CARTESIAN_POINT ( 'NONE',  ( -1.655278471875002211, 14.63297358603754716, -89.59743913623280775 ) ) ;
#12987=ORIENTED_EDGE ( 'NONE', *, *, #26461, .T. ) ;
#12988=( BOUNDED_CURVE ( )  B_SPLINE_CURVE ( 2, ( #16713, #19898, #20111, #7139, #29244, #32652, #116, #25666, #9925 ),
 .UNSPECIFIED., .F., .T. ) 
 B_SPLINE_CURVE_WITH_KNOTS ( ( 3, 2, 2, 2, 3 ),
 ( 0.03541666666666666574, 0.03611111111111110772, 0.03749999999999999861, 0.03888888888888888951, 0.03958333333333333842 ),
 .UNSPECIFIED. ) 
 CURVE ( )  GEOMETRIC_REPRESENTATION_ITEM ( )  RATIONAL_B_SPLINE_CURVE ( ( 0.9330127018922194093, 0.9330127018922194093, 1.000000000000000000, 0.8660254037844387076, 1.000000000000000000, 0.8660254037844387076, 1.000000000000000000, 0.9330127018922189652, 0.9330127018922192983 ) ) 
 REPRESENTATION_ITEM ( '' )  );
#12994=CARTESIAN_POINT ( 'NONE',  ( 3.500000000000001332, 17.50000000000002132, -129.4609808024214885 ) ) ;
#12995=CARTESIAN_POINT ( 'NONE',  ( -3.310556943750000425, 19.41135094264167549, -133.8474391362328220 ) ) ;
#12997=ORIENTED_EDGE ( 'NONE', *, *, #36779, .T. ) ;
#12998=CARTESIAN_POINT ( 'NONE',  ( -1.750000000000002220, 14.46891108675449011, -140.7943141357548313 ) ) ;
#12999=CARTESIAN_POINT ( 'NONE',  ( 3.310556943750001313, 17.50000000000002132, -117.3516058028994706 ) ) ;
#13000=CARTESIAN_POINT ( 'NONE',  ( 1.655278471874998436, 14.63297358603754006, -52.51827246956612782 ) ) ;
#13001=ORIENTED_EDGE ( 'NONE', *, *, #33113, .F. ) ;
#13002=CARTESIAN_POINT ( 'NONE',  ( 3.500000000000001776, 19.52072594216372181, -131.0713974700440758 ) ) ;
#13004=CARTESIAN_POINT ( 'NONE',  ( 3.310556943749999981, 15.58864905735836714, -70.43493913623281344 ) ) ;
#13005=CARTESIAN_POINT ( 'NONE',  ( -1.749999999999999778, 20.53108891324555785, -122.1276474690881741 ) ) ;
#13007=CARTESIAN_POINT ( 'NONE',  ( 2.340729813953370519E-16, 21.32270188528331900, -105.0141058028994649 ) ) ;
#13008=CARTESIAN_POINT ( 'NONE',  ( -0.9378221735089291577, 21.00000000000002132, -107.8600726046389155 ) ) ;
#13009=DIRECTION ( 'NONE',  ( -0.000000000000000000, 1.259100132267607459E-16, -1.000000000000000000 ) ) ;
#13011=CARTESIAN_POINT ( 'NONE',  ( -3.500000000000000888, 19.52072594216371115, -75.04431413575483134 ) ) ;
#13012=CARTESIAN_POINT ( 'NONE',  ( 3.500000000000001332, 19.52072594216371826, -126.0713974700440900 ) ) ;
#13013=CARTESIAN_POINT ( 'NONE',  ( 3.310556943750001313, 17.50000000000001066, -44.26410580289947916 ) ) ;
#13014=CARTESIAN_POINT ( 'NONE',  ( 2.340729813953370519E-16, 21.32270188528331190, -95.10160580289944221 ) ) ;
#13015=CARTESIAN_POINT ( 'NONE',  ( 4.648177544792955347E-16, 21.00000000000001776, -75.90473080337740441 ) ) ;
#13016=CARTESIAN_POINT ( 'NONE',  ( 1.749999999999998224, 14.46891108675447768, -64.32139747004410424 ) ) ;
#13018=CARTESIAN_POINT ( 'NONE',  ( -3.310556943750000425, 19.41135094264166838, -116.9349391362327850 ) ) ;
#13019=CARTESIAN_POINT ( 'NONE',  ( 4.286263797015737581E-16, 14.00000000000002487, -149.5231586289125687 ) ) ;
#13024=CARTESIAN_POINT ( 'NONE',  ( 2.340729813953370519E-16, 21.32270188528331190, -99.01410580289947916 ) ) ;
#13027=ORIENTED_EDGE ( 'NONE', *, *, #5096, .F. ) ;
#13028=CARTESIAN_POINT ( 'NONE',  ( 4.286263797015737581E-16, 14.00000000000002487, -149.5231586289125687 ) ) ;
#13030=CARTESIAN_POINT ( 'NONE',  ( -3.500000000000000000, 19.52072594216370760, -71.04431413575483134 ) ) ;
#13035=CARTESIAN_POINT ( 'NONE',  ( -3.310556943750002201, 15.58864905735836537, -27.68077246956614346 ) ) ;
#13042=CARTESIAN_POINT ( 'NONE',  ( -3.500000000000002220, 15.47927405783633503, -119.5713974700440900 ) ) ;
#13043=CARTESIAN_POINT ( 'NONE',  ( -3.500000000000000888, 19.52072594216371826, -120.7380641367107614 ) ) ;
#13046=CARTESIAN_POINT ( 'NONE',  ( -3.310556943750002645, 15.58864905735837780, -133.7682724695661420 ) ) ;
#13047=CARTESIAN_POINT ( 'NONE',  ( 3.500000000000001332, 17.50000000000001066, -33.46098080242150274 ) ) ;
#13048=DIRECTION ( 'NONE',  ( 0.000000000000000000, 1.000000000000000000, 0.000000000000000000 ) ) ;
#13050=CARTESIAN_POINT ( 'NONE',  ( 3.500000000000001332, 17.50000000000001066, -41.46098080242150985 ) ) ;
#13052=CARTESIAN_POINT ( 'NONE',  ( -3.500000000000001332, 17.50000000000002487, -136.9609808024214885 ) ) ;
#13053=CARTESIAN_POINT ( 'NONE',  ( -3.310556943750000425, 19.41135094264166838, -125.8474391362328078 ) ) ;
#13056=( BOUNDED_CURVE ( )  B_SPLINE_CURVE ( 2, ( #19817, #19605, #6641, #35363, #29600, #26420, #23220, #36187, #7058 ),
 .UNSPECIFIED., .F., .T. ) 
 B_SPLINE_CURVE_WITH_KNOTS ( ( 3, 2, 2, 2, 3 ),
 ( 0.5145833333333332815, 0.5152777777777777235, 0.5166666666666667185, 0.5180555555555556024, 0.5187500000000000444 ),
 .UNSPECIFIED. ) 
 CURVE ( )  GEOMETRIC_REPRESENTATION_ITEM ( )  RATIONAL_B_SPLINE_CURVE ( ( 0.9330127018922194093, 0.9330127018922194093, 1.000000000000000000, 0.8660254037844387076, 1.000000000000000000, 0.8660254037844387076, 1.000000000000000000, 0.9330127018922194093, 0.9330127018922194093 ) ) 
 REPRESENTATION_ITEM ( '' )  );
#13057=CARTESIAN_POINT ( 'NONE',  ( 0.000000000000000000, 21.00000000000002487, -149.5231586289125687 ) ) ;
#13058=CARTESIAN_POINT ( 'NONE',  ( -1.750000000000002220, 14.46891108675448301, -91.79431413575484555 ) ) ;
#13059=DIRECTION ( 'NONE',  ( -0.000000000000000000, 1.259100132267607459E-16, -1.000000000000000000 ) ) ;
#13060=CARTESIAN_POINT ( 'NONE',  ( 3.310556943750001313, 17.50000000000001421, -60.26410580289947916 ) ) ;
#13061=CARTESIAN_POINT ( 'NONE',  ( -3.310556943750000425, 19.41135094264166838, -116.9349391362327850 ) ) ;
#13062=FACE_OUTER_BOUND ( 'NONE', #3827, .T. ) ;
#13063=CARTESIAN_POINT ( 'NONE',  ( 3.500000000000001332, 17.50000000000001066, -30.15473080337743994 ) ) ;
#13064=CARTESIAN_POINT ( 'NONE',  ( -3.500000000000000000, 19.52072594216371826, -121.7380641367107614 ) ) ;
#13066=CARTESIAN_POINT ( 'NONE',  ( 3.310556943749999981, 15.58864905735837425, -135.4349391362327992 ) ) ;
#13070=CARTESIAN_POINT ( 'NONE',  ( 2.340729813953370519E-16, 21.32270188528330834, -71.10160580289947063 ) ) ;
#13072=CARTESIAN_POINT ( 'NONE',  ( -1.655278471874999990, 20.36702641396248836, -66.93077246956613635 ) ) ;
#13073=ORIENTED_EDGE ( 'NONE', *, *, #5673, .F. ) ;
#13074=CARTESIAN_POINT ( 'NONE',  ( -3.310556943750002201, 15.58864905735837247, -83.76827246956614204 ) ) ;
#13079=CARTESIAN_POINT ( 'NONE',  ( -1.394453263437886604E-15, 14.00000000000001421, -69.71098080242150274 ) ) ;
#13080=CARTESIAN_POINT ( 'NONE',  ( -3.310556943750002201, 15.58864905735836714, -48.68077246956615056 ) ) ;
#13081=AXIS2_PLACEMENT_3D ( 'NONE', #5246, #11830, #5667 ) ;
#13083=CARTESIAN_POINT ( 'NONE',  ( 3.310556943749999981, 15.58864905735837070, -104.3474391362328220 ) ) ;
#13089=CARTESIAN_POINT ( 'NONE',  ( -1.655278471874999990, 20.36702641396248836, -55.93077246956613635 ) ) ;
#13090=VERTEX_POINT ( 'NONE', #41971 ) ;
#13093=FACE_OUTER_BOUND ( 'NONE', #37621, .T. ) ;
#13096=CARTESIAN_POINT ( 'NONE',  ( 4.648177544792955347E-16, 21.00000000000002132, -114.2109808024214885 ) ) ;
#13097=ORIENTED_EDGE ( 'NONE', *, *, #31403, .F. ) ;
#13099=CARTESIAN_POINT ( 'NONE',  ( -3.310556943750001313, 17.50000000000002132, -123.7641058028994649 ) ) ;
#13101=CARTESIAN_POINT ( 'NONE',  ( 3.310556943750001313, 19.41135094264165772, -33.26827246956613493 ) ) ;
#13102=CARTESIAN_POINT ( 'NONE',  ( 1.655278471875001101, 20.36702641396248481, -25.18493913623280633 ) ) ;
#13104=CARTESIAN_POINT ( 'NONE',  ( 1.655278471874998436, 14.63297358603754539, -85.51827246956612782 ) ) ;
#13105=CARTESIAN_POINT ( 'NONE',  ( 3.310556943749999981, 15.58864905735837780, -141.3474391362327935 ) ) ;
#13107=CARTESIAN_POINT ( 'NONE',  ( -7.460324959392693302E-14, 21.00000000000002132, -103.2109808024215027 ) ) ;
#13109=CARTESIAN_POINT ( 'NONE',  ( 3.500000000000000000, 15.47927405783633326, -114.2380641367107472 ) ) ;
#13110=( BOUNDED_CURVE ( )  B_SPLINE_CURVE ( 2, ( #37806, #21633, #2286, #34611, #25050, #19498, #19703, #22899, #39058 ),
 .UNSPECIFIED., .F., .T. ) 
 B_SPLINE_CURVE_WITH_KNOTS ( ( 3, 2, 2, 2, 3 ),
 ( 0.08958333333333333426, 0.09027777777777777624, 0.09166666666666666019, 0.09305555555555555802, 0.09375000000000000000 ),
 .UNSPECIFIED. ) 
 CURVE ( )  GEOMETRIC_REPRESENTATION_ITEM ( )  RATIONAL_B_SPLINE_CURVE ( ( 0.9330127018922194093, 0.9330127018922194093, 1.000000000000000000, 0.8660254037844387076, 1.000000000000000000, 0.8660254037844387076, 1.000000000000000000, 0.9330127018922194093, 0.9330127018922194093 ) ) 
 REPRESENTATION_ITEM ( '' )  );
#13112=CARTESIAN_POINT ( 'NONE',  ( 3.310556943750001313, 17.50000000000002487, -134.3516058028994564 ) ) ;
#13113=LINE ( 'NONE', #19078, #31564 ) ;
#13114=CARTESIAN_POINT ( 'NONE',  ( 1.655278471875001101, 20.36702641396249192, -93.09743913623280775 ) ) ;
#13116=CARTESIAN_POINT ( 'NONE',  ( -1.749999999999999778, 20.53108891324555429, -93.12764746908815994 ) ) ;
#13118=CARTESIAN_POINT ( 'NONE',  ( 3.500000000000001776, 19.52072594216370760, -74.07139747004409003 ) ) ;
#13119=EDGE_CURVE ( 'NONE', #22032, #1435, #1805, .T. ) ;
#13120=CARTESIAN_POINT ( 'NONE',  ( -7.022189441860112050E-16, 13.67729811471672186, -60.60160580289945642 ) ) ;
#13123=CARTESIAN_POINT ( 'NONE',  ( -3.500000000000002220, 15.47927405783633503, -129.5713974700441042 ) ) ;
#13124=CARTESIAN_POINT ( 'NONE',  ( -3.310556943750002645, 15.58864905735837247, -82.76827246956615625 ) ) ;
#13126=CARTESIAN_POINT ( 'NONE',  ( -7.022189441860112050E-16, 13.67729811471672896, -113.5141058028994792 ) ) ;
#13127=CARTESIAN_POINT ( 'NONE',  ( -7.022189441860112050E-16, 13.67729811471672186, -80.51410580289947916 ) ) ;
#13129=CARTESIAN_POINT ( 'NONE',  ( -3.310556943750002201, 15.58864905735837425, -100.7682724695661420 ) ) ;
#13131=CARTESIAN_POINT ( 'NONE',  ( 1.750000000000001110, 20.53108891324555785, -103.9880641367107756 ) ) ;
#13134=CYLINDRICAL_SURFACE ( 'NONE', #34908, 3.499999999999999556 ) ;
#13135=CARTESIAN_POINT ( 'NONE',  ( 3.500000000000001332, 17.50000000000001066, -45.46098080242151696 ) ) ;
#13137=CARTESIAN_POINT ( 'NONE',  ( -3.310556943750000425, 19.41135094264166483, -66.84743913623280775 ) ) ;
#13139=CARTESIAN_POINT ( 'NONE',  ( -1.655278471874999990, 20.36702641396249547, -121.9307724695661364 ) ) ;
#13141=VERTEX_POINT ( 'NONE', #2829 ) ;
#13144=CYLINDRICAL_SURFACE ( 'NONE', #9005, 3.499999999999999556 ) ;
#13145=CARTESIAN_POINT ( 'NONE',  ( 3.310556943750001313, 19.41135094264166483, -76.18077246956615056 ) ) ;
#13152=CARTESIAN_POINT ( 'NONE',  ( 3.310556943750001313, 17.50000000000002487, -139.2641058028994792 ) ) ;
#13153=CARTESIAN_POINT ( 'NONE',  ( -0.9378221735089310451, 14.00000000000001066, -51.44938900211595012 ) ) ;
#13154=CARTESIAN_POINT ( 'NONE',  ( -1.750000000000002220, 14.46891108675448656, -110.7943141357548456 ) ) ;
#13155=CARTESIAN_POINT ( 'NONE',  ( 3.310556943750001313, 17.50000000000001066, -44.35160580289947063 ) ) ;
#13156=CARTESIAN_POINT ( 'NONE',  ( -3.310556943750000425, 19.41135094264166838, -102.9349391362327992 ) ) ;
#13157=CARTESIAN_POINT ( 'NONE',  ( 1.655278471875001101, 20.36702641396248481, -31.09743913623280775 ) ) ;
#13158=AXIS2_PLACEMENT_3D ( 'NONE', #32576, #26630, #9635 ) ;
#13159=CARTESIAN_POINT ( 'NONE',  ( 0.9378221735089300459, 21.00000000000001421, -68.94938900211596433 ) ) ;
#13160=CARTESIAN_POINT ( 'NONE',  ( -7.424026671074350129E-16, 13.45854811567263809, -101.7109808024215027 ) ) ;
#13163=CARTESIAN_POINT ( 'NONE',  ( 3.500000000000001776, 19.52072594216371115, -90.07139747004410424 ) ) ;
#13168=CARTESIAN_POINT ( 'NONE',  ( 3.500000000000001776, 19.52072594216370760, -60.37764746908817415 ) ) ;
#13170=CYLINDRICAL_SURFACE ( 'NONE', #6113, 3.499999999999999556 ) ;
#13171=ADVANCED_FACE ( 'NONE', ( #20042 ), #33006, .T. ) ;
#13172=CARTESIAN_POINT ( 'NONE',  ( 2.474675557024783212E-16, 21.54145188432739388, -49.90473080337743284 ) ) ;
#13174=CARTESIAN_POINT ( 'NONE',  ( -3.310556943750000425, 19.41135094264166128, -27.93493913623279568 ) ) ;
#13176=FACE_OUTER_BOUND ( 'NONE', #38714, .T. ) ;
#13181=CARTESIAN_POINT ( 'NONE',  ( -3.310556943750001313, 17.50000000000001776, -82.76410580289947916 ) ) ;
#13183=ORIENTED_EDGE ( 'NONE', *, *, #21816, .T. ) ;
#13185=CARTESIAN_POINT ( 'NONE',  ( 7.367361408496833051E-14, 14.00000000000001776, -108.4047308033774186 ) ) ;
#13186=ORIENTED_EDGE ( 'NONE', *, *, #38141, .T. ) ;
#13188=CARTESIAN_POINT ( 'NONE',  ( -3.310556943750001313, 17.50000000000001776, -88.76410580289947916 ) ) ;
#13190=ORIENTED_EDGE ( 'NONE', *, *, #11550, .F. ) ;
#13198=CARTESIAN_POINT ( 'NONE',  ( 3.310556943750001313, 17.50000000000002487, -131.2641058028994507 ) ) ;
#13204=CARTESIAN_POINT ( 'NONE',  ( -1.655278471874999990, 20.36702641396249547, -118.0182724695661278 ) ) ;
#13205=ORIENTED_EDGE ( 'NONE', *, *, #24174, .F. ) ;
#13207=CARTESIAN_POINT ( 'NONE',  ( 3.500000000000001776, 19.52072594216372181, -132.0713974700441042 ) ) ;
#13208=CARTESIAN_POINT ( 'NONE',  ( 1.655278471874998436, 14.63297358603754361, -71.51827246956612782 ) ) ;
#13209=CARTESIAN_POINT ( 'NONE',  ( 3.500000000000001776, 19.52072594216371826, -119.3776474690881741 ) ) ;
#13211=CARTESIAN_POINT ( 'NONE',  ( 3.310556943750001313, 17.50000000000001776, -100.2641058028994792 ) ) ;
#13216=CARTESIAN_POINT ( 'NONE',  ( 1.750000000000001110, 20.53108891324555074, -73.29431413575483134 ) ) ;
#13218=CARTESIAN_POINT ( 'NONE',  ( -3.310556943750000425, 19.41135094264165772, -38.84743913623281486 ) ) ;
#13219=CARTESIAN_POINT ( 'NONE',  ( 3.310556943750001313, 17.50000000000001776, -97.35160580289945642 ) ) ;
#13221=CARTESIAN_POINT ( 'NONE',  ( -3.500000000000000888, 19.52072594216370760, -64.73806413671077564 ) ) ;
#13223=CARTESIAN_POINT ( 'NONE',  ( -3.310556943750002201, 15.58864905735837780, -116.7682724695661278 ) ) ;
#13229=CARTESIAN_POINT ( 'NONE',  ( -1.655278471874999990, 20.36702641396249192, -97.93077246956613635 ) ) ;
#13233=( BOUNDED_CURVE ( )  B_SPLINE_CURVE ( 2, ( #15365, #37275, #8128, #28313, #41298, #21107, #34079, #4934, #25560 ),
 .UNSPECIFIED., .F., .T. ) 
 B_SPLINE_CURVE_WITH_KNOTS ( ( 3, 2, 2, 2, 3 ),
 ( 0.08541666666666666852, 0.08611111111111111049, 0.08749999999999999445, 0.08888888888888889228, 0.08958333333333333426 ),
 .UNSPECIFIED. ) 
 CURVE ( )  GEOMETRIC_REPRESENTATION_ITEM ( )  RATIONAL_B_SPLINE_CURVE ( ( 0.9330127018922194093, 0.9330127018922194093, 1.000000000000000000, 0.8660254037844387076, 1.000000000000000000, 0.8660254037844387076, 1.000000000000000000, 0.9330127018922194093, 0.9330127018922194093 ) ) 
 REPRESENTATION_ITEM ( '' )  );
#13236=CARTESIAN_POINT ( 'NONE',  ( 0.000000000000000000, 17.50000000000002487, -149.5231586289125687 ) ) ;
#13237=( BOUNDED_CURVE ( )  B_SPLINE_CURVE ( 2, ( #33279, #40301, #4144, #37123, #7976, #23293, #20945, #33917, #17757 ),
 .UNSPECIFIED., .F., .F. ) 
 B_SPLINE_CURVE_WITH_KNOTS ( ( 3, 2, 2, 2, 3 ),
 ( 0.1479166666666666685, 0.1486111111111111105, 0.1499999999999999944, 0.1513888888888888784, 0.1520833333333333481 ),
 .UNSPECIFIED. ) 
 CURVE ( )  GEOMETRIC_REPRESENTATION_ITEM ( )  RATIONAL_B_SPLINE_CURVE ( ( 0.9330127018922194093, 0.9330127018922194093, 1.000000000000000000, 0.8660254037844387076, 1.000000000000000000, 0.8660254037844387076, 1.000000000000000000, 0.9330127018922180770, 0.9330127018922194093 ) ) 
 REPRESENTATION_ITEM ( '' )  );
#13239=ORIENTED_EDGE ( 'NONE', *, *, #18764, .F. ) ;
#13243=CARTESIAN_POINT ( 'NONE',  ( -3.310556943750000425, 19.41135094264166128, -28.84743913623280420 ) ) ;
#13245=CARTESIAN_POINT ( 'NONE',  ( -3.500000000000002220, 15.47927405783633503, -123.5713974700440900 ) ) ;
#13248=CARTESIAN_POINT ( 'NONE',  ( -1.749999999999999778, 20.53108891324556140, -138.8213974700441042 ) ) ;
#13251=CARTESIAN_POINT ( 'NONE',  ( -7.460324959392693302E-14, 21.00000000000001776, -86.21098080242150274 ) ) ;
#13253=CARTESIAN_POINT ( 'NONE',  ( 1.749999999999998224, 14.46891108675448478, -119.3213974700440900 ) ) ;
#13254=DIRECTION ( 'NONE',  ( -0.000000000000000000, 1.259100132267607459E-16, -1.000000000000000000 ) ) ;
#13255=CARTESIAN_POINT ( 'NONE',  ( 1.655278471875001101, 20.36702641396249902, -137.1849391362327992 ) ) ;
#13256=CARTESIAN_POINT ( 'NONE',  ( -3.500000000000001332, 17.50000000000001066, -25.96098080242151340 ) ) ;
#13261=CARTESIAN_POINT ( 'NONE',  ( 0.9378221735089300459, 21.00000000000002132, -118.2556390011600200 ) ) ;
#13263=CARTESIAN_POINT ( 'NONE',  ( 2.474675557024783212E-16, 21.54145188432740810, -141.2109808024214885 ) ) ;
#13264=CARTESIAN_POINT ( 'NONE',  ( 3.310556943750001313, 19.41135094264166838, -117.1807724695661506 ) ) ;
#13269=CARTESIAN_POINT ( 'NONE',  ( -7.424026671074350129E-16, 13.45854811567263631, -92.71098080242150274 ) ) ;
#13271=CARTESIAN_POINT ( 'NONE',  ( -1.655278471875002211, 14.63297358603754184, -52.59743913623281486 ) ) ;
#13272=CARTESIAN_POINT ( 'NONE',  ( 2.340729813953370519E-16, 21.32270188528331900, -114.1016058028994564 ) ) ;
#13273=DIRECTION ( 'NONE',  ( -0.000000000000000000, 1.259100132267607459E-16, -1.000000000000000000 ) ) ;
#13274=CARTESIAN_POINT ( 'NONE',  ( -3.500000000000000888, 19.52072594216370405, -30.73806413671076143 ) ) ;
#13277=CARTESIAN_POINT ( 'NONE',  ( -3.310556943750001313, 17.50000000000002487, -135.8516058028994564 ) ) ;
#13279=CARTESIAN_POINT ( 'NONE',  ( -8.715332896486792803E-15, 21.00000000000002842, -137.9047308033774186 ) ) ;
#13280=FACE_OUTER_BOUND ( 'NONE', #21044, .T. ) ;
#13281=CARTESIAN_POINT ( 'NONE',  ( -1.655278471874999990, 20.36702641396248836, -62.01827246956613493 ) ) ;
#13283=CARTESIAN_POINT ( 'NONE',  ( -3.310556943750001313, 17.50000000000001421, -62.76410580289947205 ) ) ;
#13284=ORIENTED_EDGE ( 'NONE', *, *, #9555, .F. ) ;
#13285=CARTESIAN_POINT ( 'NONE',  ( 3.310556943749999981, 15.58864905735836892, -84.43493913623278502 ) ) ;
#13289=CARTESIAN_POINT ( 'NONE',  ( 3.310556943750001313, 19.41135094264166128, -46.18077246956614346 ) ) ;
#13292=CARTESIAN_POINT ( 'NONE',  ( 2.340729813953370519E-16, 21.32270188528331900, -104.0141058028994649 ) ) ;
#13293=CARTESIAN_POINT ( 'NONE',  ( 4.648177544792955347E-16, 21.00000000000001776, -93.90473080337743284 ) ) ;
#13299=CARTESIAN_POINT ( 'NONE',  ( -3.310556943750001313, 17.50000000000001421, -58.76410580289947916 ) ) ;
#13303=CARTESIAN_POINT ( 'NONE',  ( -1.749999999999999778, 20.53108891324554719, -40.82139747004409713 ) ) ;
#13306=DIRECTION ( 'NONE',  ( 0.000000000000000000, 1.000000000000000000, 0.000000000000000000 ) ) ;
#13309=( BOUNDED_CURVE ( )  B_SPLINE_CURVE ( 2, ( #36705, #27135, #20762, #33734, #21374, #41366, #9027, #31364, #22006 ),
 .UNSPECIFIED., .F., .T. ) 
 B_SPLINE_CURVE_WITH_KNOTS ( ( 3, 2, 2, 2, 3 ),
 ( 0.9895833333333333703, 0.9902777777777778123, 0.9916666666666666963, 0.9930555555555555802, 0.9937500000000000222 ),
 .UNSPECIFIED. ) 
 CURVE ( )  GEOMETRIC_REPRESENTATION_ITEM ( )  RATIONAL_B_SPLINE_CURVE ( ( 0.9330127018922194093, 0.9330127018922194093, 1.000000000000000000, 0.8660254037844387076, 1.000000000000000000, 0.8660254037844387076, 1.000000000000000000, 0.9330127018922194093, 0.9330127018922194093 ) ) 
 REPRESENTATION_ITEM ( '' )  );
#13310=CARTESIAN_POINT ( 'NONE',  ( 3.310556943750001313, 19.41135094264166838, -124.1807724695661364 ) ) ;
#13313=CARTESIAN_POINT ( 'NONE',  ( -1.655278471874999990, 20.36702641396248481, -33.01827246956613493 ) ) ;
#13314=CARTESIAN_POINT ( 'NONE',  ( 3.310556943749999981, 15.58864905735836892, -88.43493913623279923 ) ) ;
#13315=CARTESIAN_POINT ( 'NONE',  ( -3.310556943750001313, 17.50000000000002487, -141.7641058028994792 ) ) ;
#13320=CARTESIAN_POINT ( 'NONE',  ( -3.310556943750002645, 15.58864905735837780, -125.7682724695661278 ) ) ;
#13322=FACE_OUTER_BOUND ( 'NONE', #29706, .T. ) ;
#13323=CARTESIAN_POINT ( 'NONE',  ( 3.310556943750001313, 17.50000000000001776, -93.26410580289947916 ) ) ;
#13324=DIRECTION ( 'NONE',  ( 0.000000000000000000, 1.000000000000000000, 0.000000000000000000 ) ) ;
#13325=CARTESIAN_POINT ( 'NONE',  ( -3.500000000000001332, 17.50000000000002132, -125.9609808024215170 ) ) ;
#13326=CARTESIAN_POINT ( 'NONE',  ( -1.394453263437886604E-15, 14.00000000000002132, -127.7109808024214885 ) ) ;
#13327=CARTESIAN_POINT ( 'NONE',  ( -3.500000000000001332, 17.50000000000001776, -75.65473080337741862 ) ) ;
#13328=CARTESIAN_POINT ( 'NONE',  ( -7.022189441860112050E-16, 13.67729811471672186, -57.60160580289947063 ) ) ;
#13330=FACE_OUTER_BOUND ( 'NONE', #33502, .T. ) ;
#13333=CARTESIAN_POINT ( 'NONE',  ( -1.655278471875002211, 14.63297358603754716, -86.68493913623278502 ) ) ;
#13334=CARTESIAN_POINT ( 'NONE',  ( -3.500000000000002220, 15.47927405783632793, -77.57139747004410424 ) ) ;
#13336=CARTESIAN_POINT ( 'NONE',  ( -3.310556943750001313, 17.50000000000002132, -109.7641058028994649 ) ) ;
#13337=CARTESIAN_POINT ( 'NONE',  ( -7.022189441860112050E-16, 13.67729811471672186, -79.51410580289947916 ) ) ;
#13340=CARTESIAN_POINT ( 'NONE',  ( -1.655278471874999990, 20.36702641396249547, -104.0182724695661278 ) ) ;
#13341=CARTESIAN_POINT ( 'NONE',  ( -1.749999999999999778, 20.53108891324555785, -103.8213974700440900 ) ) ;
#13343=FACE_OUTER_BOUND ( 'NONE', #4204, .T. ) ;
#13345=CARTESIAN_POINT ( 'NONE',  ( 0.9378221735089300459, 21.00000000000001421, -57.94938900211595723 ) ) ;
#13346=DIRECTION ( 'NONE',  ( -0.000000000000000000, 1.259100132267607459E-16, -1.000000000000000000 ) ) ;
#13347=CARTESIAN_POINT ( 'NONE',  ( -3.310556943750002201, 15.58864905735836892, -58.68077246956614346 ) ) ;
#13349=CARTESIAN_POINT ( 'NONE',  ( 3.310556943750001313, 17.50000000000002132, -121.2641058028994792 ) ) ;
#13354=CARTESIAN_POINT ( 'NONE',  ( -0.9378221735089310451, 14.00000000000002132, -103.7556390011600342 ) ) ;
#13356=CARTESIAN_POINT ( 'NONE',  ( -1.655278471875002211, 14.63297358603754539, -73.59743913623280775 ) ) ;
#13361=ADVANCED_FACE ( 'NONE', ( #41586 ), #18195, .T. ) ;
#13362=CARTESIAN_POINT ( 'NONE',  ( -1.655278471874999990, 20.36702641396249902, -139.9307724695661364 ) ) ;
#13363=CARTESIAN_POINT ( 'NONE',  ( -0.9378221735089377065, 21.00000000000001421, -129.1663226036829428 ) ) ;
#13364=( BOUNDED_CURVE ( )  B_SPLINE_CURVE ( 2, ( #26939, #14165, #27141, #27762, #39900, #36712, #40109, #5004, #14593 ),
 .UNSPECIFIED., .F., .T. ) 
 B_SPLINE_CURVE_WITH_KNOTS ( ( 3, 2, 2, 2, 3 ),
 ( 0.9812499999999999556, 0.9819444444444443976, 0.9833333333333332815, 0.9847222222222222765, 0.9854166666666667185 ),
 .UNSPECIFIED. ) 
 CURVE ( )  GEOMETRIC_REPRESENTATION_ITEM ( )  RATIONAL_B_SPLINE_CURVE ( ( 0.9330127018922194093, 0.9330127018922194093, 1.000000000000000000, 0.8660254037844387076, 1.000000000000000000, 0.8660254037844387076, 1.000000000000000000, 0.9330127018922194093, 0.9330127018922194093 ) ) 
 REPRESENTATION_ITEM ( '' )  );
#13365=CARTESIAN_POINT ( 'NONE',  ( 2.340729813953370519E-16, 21.32270188528330479, -36.10160580289946353 ) ) ;
#13366=CARTESIAN_POINT ( 'NONE',  ( -3.310556943750002645, 15.58864905735837425, -104.7682724695661420 ) ) ;
#13367=CARTESIAN_POINT ( 'NONE',  ( -1.655278471875002211, 14.63297358603754006, -26.59743913623280420 ) ) ;
#13369=CARTESIAN_POINT ( 'NONE',  ( -3.500000000000002220, 15.47927405783632970, -102.8776474690881884 ) ) ;
#13371=LINE ( 'NONE', #25937, #26114 ) ;
#13372=CARTESIAN_POINT ( 'NONE',  ( -3.500000000000001332, 17.50000000000001776, -93.65473080337743284 ) ) ;
#13373=CARTESIAN_POINT ( 'NONE',  ( 4.648177544792955347E-16, 21.00000000000001776, -88.90473080337740441 ) ) ;
#13375=EDGE_CURVE ( 'NONE', #12197, #27884, #36584, .T. ) ;
#13377=CARTESIAN_POINT ( 'NONE',  ( -1.750000000000002220, 14.46891108675447768, -51.79431413575484555 ) ) ;
#13378=CARTESIAN_POINT ( 'NONE',  ( -3.500000000000001332, 17.50000000000001066, -30.65473080337742573 ) ) ;
#13380=ADVANCED_FACE ( 'NONE', ( #28388 ), #2023, .T. ) ;
#13381=CARTESIAN_POINT ( 'NONE',  ( -3.500000000000001332, 17.50000000000001066, -44.65473080337743994 ) ) ;
#13383=CARTESIAN_POINT ( 'NONE',  ( 1.655278471874998436, 14.63297358603753651, -25.51827246956613138 ) ) ;
#13385=CARTESIAN_POINT ( 'NONE',  ( -0.9378221735089291577, 21.00000000000001066, -39.86007260463890134 ) ) ;
#13390=CARTESIAN_POINT ( 'NONE',  ( 3.310556943749999981, 15.58864905735836892, -81.34743913623280775 ) ) ;
#13394=CARTESIAN_POINT ( 'NONE',  ( 3.500000000000001332, 19.52072594216371115, -80.37764746908818836 ) ) ;
#13396=CARTESIAN_POINT ( 'NONE',  ( 3.310556943750001313, 19.41135094264166483, -92.18077246956612214 ) ) ;
#13397=ORIENTED_EDGE ( 'NONE', *, *, #28164, .T. ) ;
#13398=VERTEX_POINT ( 'NONE', #34147 ) ;
#13400=FACE_OUTER_BOUND ( 'NONE', #9258, .T. ) ;
#13403=CARTESIAN_POINT ( 'NONE',  ( -7.022189441860112050E-16, 13.67729811471672718, -125.5141058028994934 ) ) ;
#13404=ORIENTED_EDGE ( 'NONE', *, *, #3149, .F. ) ;
#13405=CARTESIAN_POINT ( 'NONE',  ( 3.500000000000001332, 19.52072594216370760, -64.07139747004410424 ) ) ;
#13406=CARTESIAN_POINT ( 'NONE',  ( -3.310556943750002645, 15.58864905735836714, -51.76827246956612072 ) ) ;
#13407=CARTESIAN_POINT ( 'NONE',  ( -3.310556943750002645, 15.58864905735837780, -121.7682724695661278 ) ) ;
#13408=ORIENTED_EDGE ( 'NONE', *, *, #18089, .T. ) ;
#13409=ORIENTED_EDGE ( 'NONE', *, *, #2216, .F. ) ;
#13410=CARTESIAN_POINT ( 'NONE',  ( -3.500000000000000888, 19.52072594216372181, -130.7380641367107614 ) ) ;
#13411=CARTESIAN_POINT ( 'NONE',  ( -1.655278471874999990, 20.36702641396248836, -70.01827246956612782 ) ) ;
#13412=CARTESIAN_POINT ( 'NONE',  ( 1.749999999999998224, 14.46891108675448478, -116.6276474690881741 ) ) ;
#13413=CARTESIAN_POINT ( 'NONE',  ( 2.340729813953370519E-16, 21.32270188528331190, -101.0141058028994792 ) ) ;
#13417=CARTESIAN_POINT ( 'NONE',  ( 2.474675557024783212E-16, 21.54145188432739388, -69.21098080242151696 ) ) ;
#13419=CARTESIAN_POINT ( 'NONE',  ( -3.310556943750001313, 17.50000000000001066, -38.76410580289947916 ) ) ;
#13420=CARTESIAN_POINT ( 'NONE',  ( -1.655278471875002211, 14.63297358603754716, -94.68493913623279923 ) ) ;
#13421=CARTESIAN_POINT ( 'NONE',  ( -7.424026671074350129E-16, 13.45854811567263454, -58.40473080337743284 ) ) ;
#13423=CARTESIAN_POINT ( 'NONE',  ( 1.655278471875001101, 20.36702641396249547, -116.1849391362327850 ) ) ;
#13425=CARTESIAN_POINT ( 'NONE',  ( -0.9378221735089291577, 21.00000000000001421, -61.16632260368297835 ) ) ;
#13428=CARTESIAN_POINT ( 'NONE',  ( 1.749999999999998224, 14.46891108675447946, -79.62764746908817415 ) ) ;
#13429=CARTESIAN_POINT ( 'NONE',  ( -1.394453263437886604E-15, 14.00000000000001776, -107.7109808024215170 ) ) ;
#13430=CARTESIAN_POINT ( 'NONE',  ( -3.310556943750002201, 15.58864905735837425, -99.68077246956613635 ) ) ;
#13433=ORIENTED_EDGE ( 'NONE', *, *, #38327, .T. ) ;
#13434=CARTESIAN_POINT ( 'NONE',  ( -0.9378221735089640188, 20.99999999999999645, -87.86007260463890134 ) ) ;
#13436=DIRECTION ( 'NONE',  ( 0.000000000000000000, 1.000000000000000000, 0.000000000000000000 ) ) ;
#13437=CARTESIAN_POINT ( 'NONE',  ( -0.9378221735089310451, 14.00000000000002309, -112.4493890021159501 ) ) ;
#13443=CARTESIAN_POINT ( 'NONE',  ( -1.655278471875002211, 14.63297358603754006, -30.59743913623280775 ) ) ;
#13445=DIRECTION ( 'NONE',  ( 0.000000000000000000, 1.000000000000000000, 0.000000000000000000 ) ) ;
#13450=CARTESIAN_POINT ( 'NONE',  ( -1.749999999999999778, 20.53108891324554719, -37.82139747004409003 ) ) ;
#13452=ADVANCED_FACE ( 'NONE', ( #9894 ), #36023, .T. ) ;
#13454=CARTESIAN_POINT ( 'NONE',  ( -3.500000000000000888, 19.52072594216371826, -118.7380641367107614 ) ) ;
#13455=CARTESIAN_POINT ( 'NONE',  ( -1.749999999999999778, 20.53108891324555429, -75.12764746908817415 ) ) ;
#13456=CARTESIAN_POINT ( 'NONE',  ( 3.310556943749999981, 15.58864905735837425, -133.4349391362327992 ) ) ;
#13457=CARTESIAN_POINT ( 'NONE',  ( -7.424026671074350129E-16, 13.45854811567263098, -29.71098080242151340 ) ) ;
#13461=CARTESIAN_POINT ( 'NONE',  ( -1.750000000000002220, 14.46891108675448834, -133.7943141357548598 ) ) ;
#13462=CARTESIAN_POINT ( 'NONE',  ( -7.022189441860112050E-16, 13.67729811471672718, -117.5141058028994792 ) ) ;
#13466=CARTESIAN_POINT ( 'NONE',  ( 1.749999999999998224, 14.46891108675448123, -88.62764746908817415 ) ) ;
#13467=AXIS2_PLACEMENT_3D ( 'NONE', #14296, #18686, #39818 ) ;
#13468=( BOUNDED_CURVE ( )  B_SPLINE_CURVE ( 2, ( #3077, #34768, #22011, #9676, #5848, #32212, #25631, #9247, #3282 ),
 .UNSPECIFIED., .F., .F. ) 
 B_SPLINE_CURVE_WITH_KNOTS ( ( 3, 2, 2, 2, 3 ),
 ( 0.4229166666666666630, 0.4236111111111111049, 0.4249999999999999889, 0.4263888888888888729, 0.4270833333333333148 ),
 .UNSPECIFIED. ) 
 CURVE ( )  GEOMETRIC_REPRESENTATION_ITEM ( )  RATIONAL_B_SPLINE_CURVE ( ( 0.9330127018922194093, 0.9330127018922194093, 1.000000000000000000, 0.8660254037844387076, 1.000000000000000000, 0.8660254037844387076, 1.000000000000000000, 0.9330127018922194093, 0.9330127018922194093 ) ) 
 REPRESENTATION_ITEM ( '' )  );
#13470=CARTESIAN_POINT ( 'NONE',  ( -3.310556943750000425, 19.41135094264166128, -55.84743913623280065 ) ) ;
#13471=CARTESIAN_POINT ( 'NONE',  ( 2.340729813953370519E-16, 21.32270188528331900, -113.1016058028994706 ) ) ;
#13472=LINE ( 'NONE', #3903, #26848 ) ;
#13473=CARTESIAN_POINT ( 'NONE',  ( 1.749999999999998224, 14.46891108675447413, -28.32139747004410069 ) ) ;
#13476=CARTESIAN_POINT ( 'NONE',  ( -7.022189441860112050E-16, 13.67729811471672896, -134.6016058028994564 ) ) ;
#13478=CARTESIAN_POINT ( 'NONE',  ( -1.394453263437886604E-15, 14.00000000000001421, -66.40473080337741862 ) ) ;
#13480=CARTESIAN_POINT ( 'NONE',  ( 1.655278471874998436, 14.63297358603754184, -61.51827246956613493 ) ) ;
#13482=CARTESIAN_POINT ( 'NONE',  ( -7.022189441860112050E-16, 13.67729811471671830, -63.51410580289947205 ) ) ;
#13483=ORIENTED_EDGE ( 'NONE', *, *, #16684, .F. ) ;
#13484=CARTESIAN_POINT ( 'NONE',  ( -3.310556943750001313, 17.50000000000001776, -87.85160580289947063 ) ) ;
#13487=FACE_OUTER_BOUND ( 'NONE', #22821, .T. ) ;
#13489=CARTESIAN_POINT ( 'NONE',  ( 1.655278471874998436, 14.63297358603754006, -46.43077246956614346 ) ) ;
#13491=CARTESIAN_POINT ( 'NONE',  ( 3.310556943750001313, 19.41135094264166483, -98.18077246956613635 ) ) ;
#13492=FACE_OUTER_BOUND ( 'NONE', #2256, .T. ) ;
#13493=VERTEX_POINT ( 'NONE', #16272 ) ;
#13495=ORIENTED_EDGE ( 'NONE', *, *, #5094, .F. ) ;
#13497=EDGE_CURVE ( 'NONE', #37838, #37609, #22181, .T. ) ;
#13498=CARTESIAN_POINT ( 'NONE',  ( -1.655278471875002211, 14.63297358603754361, -57.59743913623280065 ) ) ;
#13502=FACE_OUTER_BOUND ( 'NONE', #4235, .T. ) ;
#13503=CARTESIAN_POINT ( 'NONE',  ( 3.500000000000001332, 19.52072594216370405, -31.37764746908818125 ) ) ;
#13507=VERTEX_POINT ( 'NONE', #28805 ) ;
#13509=CARTESIAN_POINT ( 'NONE',  ( 3.500000000000001332, 17.50000000000001066, -43.46098080242151696 ) ) ;
#13510=CARTESIAN_POINT ( 'NONE',  ( 1.655278471874998436, 14.63297358603754006, -44.43077246956614346 ) ) ;
#13512=DIRECTION ( 'NONE',  ( -0.000000000000000000, 1.259100132267607459E-16, -1.000000000000000000 ) ) ;
#13513=CARTESIAN_POINT ( 'NONE',  ( 0.9378221735089300459, 21.00000000000001776, -94.25563900116002003 ) ) ;
#13515=CARTESIAN_POINT ( 'NONE',  ( 1.655278471874998436, 14.63297358603753828, -30.51827246956613493 ) ) ;
#13517=CARTESIAN_POINT ( 'NONE',  ( 1.655278471874998436, 14.63297358603754539, -82.51827246956614204 ) ) ;
#13518=CARTESIAN_POINT ( 'NONE',  ( -3.310556943750002645, 15.58864905735837780, -133.6807724695661648 ) ) ;
#13521=PRODUCT_DEFINITION_CONTEXT ( 'detailed design', #36414, 'design' ) ;
#13522=CARTESIAN_POINT ( 'NONE',  ( -3.310556943750001313, 17.50000000000002132, -128.8516058028994564 ) ) ;
#13523=CARTESIAN_POINT ( 'NONE',  ( 4.648177544792955347E-16, 21.00000000000001066, -42.21098080242150274 ) ) ;
#13524=CARTESIAN_POINT ( 'NONE',  ( 2.340729813953370519E-16, 21.32270188528331190, -86.01410580289946495 ) ) ;
#13526=CARTESIAN_POINT ( 'NONE',  ( 3.500000000000000000, 15.47927405783632437, -65.23806413671076143 ) ) ;
#13527=CARTESIAN_POINT ( 'NONE',  ( 3.500000000000001332, 17.50000000000002132, -126.4609808024215170 ) ) ;
#13528=CARTESIAN_POINT ( 'NONE',  ( 2.474675557024783212E-16, 21.54145188432739744, -74.90473080337743284 ) ) ;
#13529=CARTESIAN_POINT ( 'NONE',  ( 3.310556943749999981, 15.58864905735836537, -61.43493913623279923 ) ) ;
#13531=DIRECTION ( 'NONE',  ( 0.000000000000000000, 1.000000000000000000, 0.000000000000000000 ) ) ;
#13533=CARTESIAN_POINT ( 'NONE',  ( 2.340729813953370519E-16, 21.32270188528331190, -80.10160580289947063 ) ) ;
#13534=CYLINDRICAL_SURFACE ( 'NONE', #2428, 3.499999999999999556 ) ;
#13537=CARTESIAN_POINT ( 'NONE',  ( -1.655278471874999990, 20.36702641396249547, -110.9307724695661506 ) ) ;
#13538=CARTESIAN_POINT ( 'NONE',  ( 3.310556943750001313, 17.50000000000001776, -81.26410580289947916 ) ) ;
#13539=DIRECTION ( 'NONE',  ( -0.000000000000000000, 1.259100132267607459E-16, -1.000000000000000000 ) ) ;
#13540=ORIENTED_EDGE ( 'NONE', *, *, #39886, .F. ) ;
#13541=CARTESIAN_POINT ( 'NONE',  ( -3.310556943750001313, 17.50000000000002132, -103.8516058028994564 ) ) ;
#13542=CARTESIAN_POINT ( 'NONE',  ( -1.750000000000002220, 14.46891108675448478, -103.4880641367107756 ) ) ;
#13545=CARTESIAN_POINT ( 'NONE',  ( -3.500000000000000000, 19.52072594216370405, -38.04431413575484555 ) ) ;
#13547=DIRECTION ( 'NONE',  ( -0.000000000000000000, 1.259100132267607459E-16, -1.000000000000000000 ) ) ;
#13548=CARTESIAN_POINT ( 'NONE',  ( -3.310556943750000425, 19.41135094264166483, -62.84743913623280775 ) ) ;
#13550=CARTESIAN_POINT ( 'NONE',  ( -1.655278471875002211, 14.63297358603755072, -120.5974391362328078 ) ) ;
#13551=CYLINDRICAL_SURFACE ( 'NONE', #29099, 3.499999999999999556 ) ;
#13554=ORIENTED_EDGE ( 'NONE', *, *, #38378, .T. ) ;
#13557=CARTESIAN_POINT ( 'NONE',  ( 4.286263797015737581E-16, 14.00000000000002487, -149.5231586289125687 ) ) ;
#13559=EDGE_CURVE ( 'NONE', #34378, #11163, #28138, .T. ) ;
#13560=CARTESIAN_POINT ( 'NONE',  ( -7.022189441860112050E-16, 13.67729811471672186, -72.51410580289946495 ) ) ;
#13567=CARTESIAN_POINT ( 'NONE',  ( 2.340729813953370519E-16, 21.32270188528332255, -137.0141058028994792 ) ) ;
#13568=VECTOR ( 'NONE', #8789, 1000.000000000000000 ) ;
#13571=CARTESIAN_POINT ( 'NONE',  ( -0.9378221735088960731, 14.00000000000000355, -110.7556390011600342 ) ) ;
#13572=CARTESIAN_POINT ( 'NONE',  ( -3.310556943750000425, 19.41135094264165772, -39.93493913623280633 ) ) ;
#13573=CARTESIAN_POINT ( 'NONE',  ( 3.310556943749999981, 15.58864905735837070, -100.4349391362327992 ) ) ;
#13575=CARTESIAN_POINT ( 'NONE',  ( 1.655278471874998436, 14.63297358603753828, -26.43077246956613990 ) ) ;
#13576=CARTESIAN_POINT ( 'NONE',  ( 3.500000000000000000, 15.47927405783632615, -69.23806413671077564 ) ) ;
#13577=CARTESIAN_POINT ( 'NONE',  ( 3.500000000000001776, 19.52072594216371826, -104.3776474690881741 ) ) ;
#13580=CARTESIAN_POINT ( 'NONE',  ( 3.500000000000001776, 19.52072594216371115, -92.07139747004409003 ) ) ;
#13584=CARTESIAN_POINT ( 'NONE',  ( 3.500000000000000000, 15.47927405783632260, -55.54431413575484555 ) ) ;
#13585=CARTESIAN_POINT ( 'NONE',  ( -1.394453263437886604E-15, 14.00000000000001066, -53.71098080242150985 ) ) ;
#13586=CARTESIAN_POINT ( 'NONE',  ( -3.500000000000000000, 19.52072594216371826, -134.7380641367107614 ) ) ;
#13587=VERTEX_POINT ( 'NONE', #22643 ) ;
#13588=CARTESIAN_POINT ( 'NONE',  ( 3.500000000000000000, 15.47927405783632082, -44.23806413671076143 ) ) ;
#13590=CARTESIAN_POINT ( 'NONE',  ( -3.310556943750000425, 19.41135094264166128, -26.93493913623279212 ) ) ;
#13592=CARTESIAN_POINT ( 'NONE',  ( 7.785697387528201340E-15, 14.00000000000002487, -137.4047308033774470 ) ) ;
#13593=CARTESIAN_POINT ( 'NONE',  ( 4.648177544792955347E-16, 21.00000000000001421, -60.90473080337742573 ) ) ;
#13597=CARTESIAN_POINT ( 'NONE',  ( -3.310556943750001313, 17.50000000000001776, -74.76410580289947916 ) ) ;
#13598=FACE_OUTER_BOUND ( 'NONE', #29334, .T. ) ;
#13601=CARTESIAN_POINT ( 'NONE',  ( -3.500000000000001332, 17.50000000000001776, -97.96098080242150274 ) ) ;
#13605=CARTESIAN_POINT ( 'NONE',  ( 2.340729813953370519E-16, 21.32270188528331190, -88.01410580289947916 ) ) ;
#13606=ORIENTED_EDGE ( 'NONE', *, *, #16082, .T. ) ;
#13613=EDGE_CURVE ( 'NONE', #26292, #16644, #820, .T. ) ;
#13614=CARTESIAN_POINT ( 'NONE',  ( 1.655278471875001101, 20.36702641396249547, -127.0974391362328078 ) ) ;
#13615=VERTEX_POINT ( 'NONE', #39210 ) ;
#13616=CARTESIAN_POINT ( 'NONE',  ( -1.655278471874999990, 20.36702641396248836, -54.01827246956612782 ) ) ;
#13617=CARTESIAN_POINT ( 'NONE',  ( 2.340729813953370519E-16, 21.32270188528331900, -119.1016058028994564 ) ) ;
#13618=ORIENTED_EDGE ( 'NONE', *, *, #7073, .F. ) ;
#13620=CARTESIAN_POINT ( 'NONE',  ( 3.500000000000000000, 15.47927405783633503, -125.2380641367107614 ) ) ;
#13622=CARTESIAN_POINT ( 'NONE',  ( 1.655278471874998436, 14.63297358603753828, -37.43077246956613635 ) ) ;
#13623=CARTESIAN_POINT ( 'NONE',  ( -1.655278471875002211, 14.63297358603754539, -70.68493913623278502 ) ) ;
#13624=CARTESIAN_POINT ( 'NONE',  ( 2.474675557024783212E-16, 21.54145188432740099, -117.2109808024215027 ) ) ;
#13625=CARTESIAN_POINT ( 'NONE',  ( -3.310556943750002645, 15.58864905735837425, -99.68077246956613635 ) ) ;
#13626=LINE ( 'NONE', #35959, #32260 ) ;
#13627=DIRECTION ( 'NONE',  ( -0.000000000000000000, 1.259100132267607459E-16, -1.000000000000000000 ) ) ;
#13629=CARTESIAN_POINT ( 'NONE',  ( -1.750000000000002220, 14.46891108675448123, -70.79431413575483134 ) ) ;
#13630=CARTESIAN_POINT ( 'NONE',  ( 0.9378221735089281585, 14.00000000000002132, -100.6663226036829855 ) ) ;
#13631=CARTESIAN_POINT ( 'NONE',  ( -3.310556943750002645, 15.58864905735836537, -38.68077246956613635 ) ) ;
#13633=CARTESIAN_POINT ( 'NONE',  ( 3.310556943749999981, 15.58864905735836892, -93.43493913623281344 ) ) ;
#13634=CARTESIAN_POINT ( 'NONE',  ( 2.474675557024783212E-16, 21.54145188432739388, -56.90473080337743284 ) ) ;
#13635=CARTESIAN_POINT ( 'NONE',  ( 7.367361408496833051E-14, 14.00000000000001776, -108.7109808024215027 ) ) ;
#13636=CARTESIAN_POINT ( 'NONE',  ( -7.022189441860112050E-16, 13.67729811471672896, -110.6016058028994564 ) ) ;
#13637=CARTESIAN_POINT ( 'NONE',  ( 3.310556943749999981, 15.58864905735836182, -45.43493913623279923 ) ) ;
#13643=CARTESIAN_POINT ( 'NONE',  ( -1.749999999999999778, 20.53108891324554719, -23.82139747004409358 ) ) ;
#13644=EDGE_CURVE ( 'NONE', #29719, #34720, #26540, .T. ) ;
#13645=CARTESIAN_POINT ( 'NONE',  ( 3.310556943750001313, 17.50000000000001776, -94.26410580289947916 ) ) ;
#13646=CARTESIAN_POINT ( 'NONE',  ( -1.749999999999999778, 20.53108891324554719, -36.82139747004409003 ) ) ;
#13649=DIRECTION ( 'NONE',  ( -0.000000000000000000, 1.259100132267607459E-16, -1.000000000000000000 ) ) ;
#13652=CARTESIAN_POINT ( 'NONE',  ( -1.394453263437886604E-15, 14.00000000000002132, -123.4047308033774044 ) ) ;
#13656=CARTESIAN_POINT ( 'NONE',  ( -3.310556943750001313, 17.50000000000001066, -30.76410580289946850 ) ) ;
#13657=ORIENTED_EDGE ( 'NONE', *, *, #38676, .T. ) ;
#13658=CARTESIAN_POINT ( 'NONE',  ( -3.695301148110399846E-14, 21.00000000000002132, -123.9047308033774044 ) ) ;
#13663=EDGE_LOOP ( 'NONE', ( #20927, #7124, #11043, #19774 ) ) ;
#13664=CARTESIAN_POINT ( 'NONE',  ( 0.9378221735089367073, 14.00000000000002487, -135.3600726046389013 ) ) ;
#13665=AXIS2_PLACEMENT_3D ( 'NONE', #37540, #18186, #31155 ) ;
#13669=CARTESIAN_POINT ( 'NONE',  ( 1.750000000000001110, 20.53108891324555074, -68.29431413575484555 ) ) ;
#13671=CARTESIAN_POINT ( 'NONE',  ( -1.655278471874999990, 20.36702641396249902, -137.0182724695661420 ) ) ;
#13672=CARTESIAN_POINT ( 'NONE',  ( -1.750000000000002220, 14.46891108675447590, -27.79431413575483845 ) ) ;
#13673=( BOUNDED_CURVE ( )  B_SPLINE_CURVE ( 2, ( #5237, #24393, #17797, #40553, #8217, #17592, #21191, #5023, #15024 ),
 .UNSPECIFIED., .F., .T. ) 
 B_SPLINE_CURVE_WITH_KNOTS ( ( 3, 2, 2, 2, 3 ),
 ( 0.4895833333333333148, 0.4902777777777777568, 0.4916666666666666408, 0.4930555555555555802, 0.4937500000000000222 ),
 .UNSPECIFIED. ) 
 CURVE ( )  GEOMETRIC_REPRESENTATION_ITEM ( )  RATIONAL_B_SPLINE_CURVE ( ( 0.9330127018922194093, 0.9330127018922194093, 1.000000000000000000, 0.8660254037844387076, 1.000000000000000000, 0.8660254037844387076, 1.000000000000000000, 0.9330127018922194093, 0.9330127018922194093 ) ) 
 REPRESENTATION_ITEM ( '' )  );
#13675=CARTESIAN_POINT ( 'NONE',  ( 2.474675557024783212E-16, 21.54145188432740810, -141.9047308033774186 ) ) ;
#13676=CARTESIAN_POINT ( 'NONE',  ( 1.749999999999998224, 14.46891108675448656, -123.6276474690881741 ) ) ;
#13678=CARTESIAN_POINT ( 'NONE',  ( 3.500000000000001776, 19.52072594216372181, -136.3776474690881741 ) ) ;
#13679=CARTESIAN_POINT ( 'NONE',  ( -1.655278471875002211, 14.63297358603755072, -119.5974391362328078 ) ) ;
#13683=CARTESIAN_POINT ( 'NONE',  ( 3.500000000000000000, 15.47927405783632615, -86.54431413575484555 ) ) ;
#13684=CARTESIAN_POINT ( 'NONE',  ( -1.749999999999999778, 20.53108891324555074, -69.82139747004409003 ) ) ;
#13685=CARTESIAN_POINT ( 'NONE',  ( 1.655278471875001101, 20.36702641396248836, -54.09743913623281486 ) ) ;
#13686=CARTESIAN_POINT ( 'NONE',  ( 1.655278471874998436, 14.63297358603754894, -112.5182724695661420 ) ) ;
#13687=CARTESIAN_POINT ( 'NONE',  ( 4.648177544792955347E-16, 21.00000000000001066, -38.21098080242150985 ) ) ;
#13688=CARTESIAN_POINT ( 'NONE',  ( -3.500000000000001332, 17.50000000000001066, -27.65473080337743639 ) ) ;
#13689=CARTESIAN_POINT ( 'NONE',  ( 0.9378221735089300459, 21.00000000000002132, -116.2556390011600200 ) ) ;
#13691=CARTESIAN_POINT ( 'NONE',  ( 3.310556943750001313, 17.50000000000002132, -128.3516058028994564 ) ) ;
#13695=EDGE_CURVE ( 'NONE', #5825, #9113, #7608, .T. ) ;
#13696=CARTESIAN_POINT ( 'NONE',  ( 2.340729813953370519E-16, 21.32270188528330834, -62.10160580289945642 ) ) ;
#13698=CARTESIAN_POINT ( 'NONE',  ( 3.310556943750001313, 17.50000000000001421, -62.26410580289947205 ) ) ;
#13699=ORIENTED_EDGE ( 'NONE', *, *, #31035, .F. ) ;
#13701=CARTESIAN_POINT ( 'NONE',  ( 3.310556943750001313, 17.50000000000001776, -84.35160580289947063 ) ) ;
#13702=ADVANCED_FACE ( 'NONE', ( #34174 ), #8229, .T. ) ;
#13705=CARTESIAN_POINT ( 'NONE',  ( 4.286263797015737581E-16, 14.00000000000002487, -149.5231586289125687 ) ) ;
#13706=CYLINDRICAL_SURFACE ( 'NONE', #30182, 3.499999999999999556 ) ;
#13708=CARTESIAN_POINT ( 'NONE',  ( 2.340729813953370519E-16, 21.32270188528330834, -44.01410580289947916 ) ) ;
#13710=CARTESIAN_POINT ( 'NONE',  ( -1.655278471874999990, 20.36702641396249192, -97.93077246956613635 ) ) ;
#13712=VERTEX_POINT ( 'NONE', #4831 ) ;
#13716=CARTESIAN_POINT ( 'NONE',  ( -1.655278471874999990, 20.36702641396248836, -53.93077246956613635 ) ) ;
#13717=ORIENTED_EDGE ( 'NONE', *, *, #36588, .T. ) ;
#13720=CARTESIAN_POINT ( 'NONE',  ( -1.394453263437886604E-15, 14.00000000000001421, -76.71098080242148853 ) ) ;
#13721=CARTESIAN_POINT ( 'NONE',  ( 4.648177544792955347E-16, 21.00000000000001776, -96.21098080242150274 ) ) ;
#13725=CARTESIAN_POINT ( 'NONE',  ( -3.500000000000000888, 19.52072594216370405, -46.04431413575483845 ) ) ;
#13726=CARTESIAN_POINT ( 'NONE',  ( -3.310556943750000425, 19.41135094264165772, -42.84743913623280065 ) ) ;
#13727=CARTESIAN_POINT ( 'NONE',  ( 3.500000000000001332, 17.50000000000002132, -108.4609808024215027 ) ) ;
#13728=CARTESIAN_POINT ( 'NONE',  ( -3.500000000000001332, 17.50000000000002487, -133.6547308033774186 ) ) ;
#13730=( BOUNDED_CURVE ( )  B_SPLINE_CURVE ( 2, ( #10954, #4360, #1379, #17127, #33498, #7551, #8174, #4143, #26912 ),
 .UNSPECIFIED., .F., .T. ) 
 B_SPLINE_CURVE_WITH_KNOTS ( ( 3, 2, 2, 2, 3 ),
 ( 0.4145833333333333592, 0.4152777777777778012, 0.4166666666666666852, 0.4180555555555555691, 0.4187500000000000111 ),
 .UNSPECIFIED. ) 
 CURVE ( )  GEOMETRIC_REPRESENTATION_ITEM ( )  RATIONAL_B_SPLINE_CURVE ( ( 0.9330127018922194093, 0.9330127018922220739, 1.000000000000000000, 0.8660254037844387076, 1.000000000000000000, 0.8660254037844387076, 1.000000000000000000, 0.9330127018922194093, 0.9330127018922194093 ) ) 
 REPRESENTATION_ITEM ( '' )  );
#13731=AXIS2_PLACEMENT_3D ( 'NONE', #4386, #1198, #10977 ) ;
#13734=CARTESIAN_POINT ( 'NONE',  ( -1.655278471874999990, 20.36702641396248481, -28.01827246956613138 ) ) ;
#13735=EDGE_CURVE ( 'NONE', #29815, #25124, #40930, .T. ) ;
#13737=CARTESIAN_POINT ( 'NONE',  ( 2.340729813953370519E-16, 21.32270188528331190, -82.10160580289945642 ) ) ;
#13738=CARTESIAN_POINT ( 'NONE',  ( -7.022189441860112050E-16, 13.67729811471672718, -132.5141058028994792 ) ) ;
#13742=CARTESIAN_POINT ( 'NONE',  ( 3.500000000000001332, 19.52072594216371115, -85.37764746908817415 ) ) ;
#13743=CARTESIAN_POINT ( 'NONE',  ( 3.310556943750001313, 17.50000000000002132, -127.3516058028994422 ) ) ;
#13745=CARTESIAN_POINT ( 'NONE',  ( 3.310556943749999981, 15.58864905735836892, -88.34743913623280775 ) ) ;
#13746=DIRECTION ( 'NONE',  ( -0.000000000000000000, 1.259100132267607459E-16, -1.000000000000000000 ) ) ;
#13747=CARTESIAN_POINT ( 'NONE',  ( 3.500000000000000000, 15.47927405783632615, -75.54431413575484555 ) ) ;
#13748=CYLINDRICAL_SURFACE ( 'NONE', #35663, 3.499999999999999556 ) ;
#13749=CARTESIAN_POINT ( 'NONE',  ( -3.500000000000002220, 15.47927405783632615, -76.57139747004409003 ) ) ;
#13750=EDGE_CURVE ( 'NONE', #19314, #1224, #10747, .T. ) ;
#13752=CARTESIAN_POINT ( 'NONE',  ( 1.655278471875001101, 20.36702641396248836, -59.18493913623279212 ) ) ;
#13756=CARTESIAN_POINT ( 'NONE',  ( -1.655278471874999990, 20.36702641396249192, -78.01827246956614204 ) ) ;
#13757=CARTESIAN_POINT ( 'NONE',  ( 3.310556943750001313, 17.50000000000002487, -141.3516058028994564 ) ) ;
#13759=CARTESIAN_POINT ( 'NONE',  ( -1.655278471875002211, 14.63297358603755072, -111.5974391362328078 ) ) ;
#13760=CARTESIAN_POINT ( 'NONE',  ( 3.310556943749999981, 15.58864905735836892, -83.34743913623279354 ) ) ;
#13761=CARTESIAN_POINT ( 'NONE',  ( -1.394453263437886604E-15, 14.00000000000001421, -57.40473080337742573 ) ) ;
#13763=CARTESIAN_POINT ( 'NONE',  ( 3.310556943750001313, 19.41135094264166838, -102.2682724695661278 ) ) ;
#13764=CARTESIAN_POINT ( 'NONE',  ( -1.750000000000002220, 14.46891108675448478, -101.4880641367107756 ) ) ;
#13767=CARTESIAN_POINT ( 'NONE',  ( 0.000000000000000000, 17.50000000000002487, -149.5231586289125687 ) ) ;
#13770=CARTESIAN_POINT ( 'NONE',  ( -1.655278471874999990, 20.36702641396248836, -61.93077246956614346 ) ) ;
#13772=CARTESIAN_POINT ( 'NONE',  ( 2.340729813953370519E-16, 21.32270188528331900, -118.0141058028994792 ) ) ;
#13773=DIRECTION ( 'NONE',  ( -0.000000000000000000, 1.259100132267607459E-16, -1.000000000000000000 ) ) ;
#13779=CARTESIAN_POINT ( 'NONE',  ( 1.655278471874998436, 14.63297358603754184, -66.43077246956613635 ) ) ;
#13781=ORIENTED_EDGE ( 'NONE', *, *, #3274, .T. ) ;
#13782=CARTESIAN_POINT ( 'NONE',  ( 1.749999999999998224, 14.46891108675448123, -83.62764746908818836 ) ) ;
#13785=AXIS2_PLACEMENT_3D ( 'NONE', #12755, #19138, #31473 ) ;
#13786=ORIENTED_EDGE ( 'NONE', *, *, #22675, .F. ) ;
#13788=CARTESIAN_POINT ( 'NONE',  ( -3.310556943750000425, 19.41135094264167549, -136.8474391362328220 ) ) ;
#13789=CARTESIAN_POINT ( 'NONE',  ( 0.000000000000000000, 17.50000000000002487, -149.5231586289125687 ) ) ;
#13790=CARTESIAN_POINT ( 'NONE',  ( -1.655278471874999990, 20.36702641396248481, -44.01827246956613493 ) ) ;
#13791=CARTESIAN_POINT ( 'NONE',  ( -0.9378221735089310451, 14.00000000000002132, -89.44938900211595012 ) ) ;
#13792=CARTESIAN_POINT ( 'NONE',  ( 3.310556943750001313, 17.50000000000001066, -38.35160580289946353 ) ) ;
#13793=CARTESIAN_POINT ( 'NONE',  ( 3.310556943749999981, 15.58864905735837070, -96.43493913623281344 ) ) ;
#13795=CARTESIAN_POINT ( 'NONE',  ( -1.655278471874999990, 20.36702641396248481, -24.93077246956613990 ) ) ;
#13796=CARTESIAN_POINT ( 'NONE',  ( 4.286263797015737581E-16, 14.00000000000002487, -149.5231586289125687 ) ) ;
#13797=CARTESIAN_POINT ( 'NONE',  ( 2.474675557024783212E-16, 21.54145188432739744, -99.21098080242150274 ) ) ;
#13798=CARTESIAN_POINT ( 'NONE',  ( 3.500000000000001332, 19.52072594216371115, -100.0713974700440900 ) ) ;
#13799=DIRECTION ( 'NONE',  ( 0.000000000000000000, 1.000000000000000000, 0.000000000000000000 ) ) ;
#13800=CARTESIAN_POINT ( 'NONE',  ( -1.750000000000002220, 14.46891108675448301, -91.48806413671076143 ) ) ;
#13806=CARTESIAN_POINT ( 'NONE',  ( -3.500000000000001332, 17.50000000000001421, -52.96098080242150985 ) ) ;
#13807=DIRECTION ( 'NONE',  ( -0.000000000000000000, 1.259100132267607459E-16, -1.000000000000000000 ) ) ;
#13810=CARTESIAN_POINT ( 'NONE',  ( -3.500000000000002220, 15.47927405783632260, -43.57139747004409713 ) ) ;
#13811=CARTESIAN_POINT ( 'NONE',  ( -0.9378221735089310451, 14.00000000000002309, -131.7556390011600342 ) ) ;
#13812=CARTESIAN_POINT ( 'NONE',  ( -3.310556943750000425, 19.41135094264166128, -29.93493913623279568 ) ) ;
#13813=CARTESIAN_POINT ( 'NONE',  ( -3.500000000000001332, 17.50000000000001421, -56.96098080242150985 ) ) ;
#13816=CARTESIAN_POINT ( 'NONE',  ( 0.9378221735089281585, 14.00000000000002132, -120.3600726046389013 ) ) ;
#13818=CARTESIAN_POINT ( 'NONE',  ( -1.655278471874999990, 20.36702641396249192, -77.93077246956615056 ) ) ;
#13823=CARTESIAN_POINT ( 'NONE',  ( -1.394453263437886604E-15, 14.00000000000001421, -54.40473080337742573 ) ) ;
#13825=CARTESIAN_POINT ( 'NONE',  ( -0.9378221735089310451, 14.00000000000002132, -87.75563900116003424 ) ) ;
#13826=CARTESIAN_POINT ( 'NONE',  ( -1.655278471874999990, 20.36702641396249192, -89.93077246956613635 ) ) ;
#13827=VERTEX_POINT ( 'NONE', #1641 ) ;
#13832=CARTESIAN_POINT ( 'NONE',  ( 3.310556943749999981, 15.58864905735837425, -125.3474391362328078 ) ) ;
#13834=CARTESIAN_POINT ( 'NONE',  ( -3.310556943750000425, 19.41135094264166128, -51.93493913623279923 ) ) ;
#13835=CARTESIAN_POINT ( 'NONE',  ( -1.655278471874999990, 20.36702641396249547, -115.0182724695661278 ) ) ;
#13837=ORIENTED_EDGE ( 'NONE', *, *, #19931, .F. ) ;
#13838=CARTESIAN_POINT ( 'NONE',  ( -3.500000000000002220, 15.47927405783633503, -126.5713974700440900 ) ) ;
#13839=CARTESIAN_POINT ( 'NONE',  ( 3.310556943749999981, 15.58864905735836182, -41.34743913623280065 ) ) ;
#13841=CARTESIAN_POINT ( 'NONE',  ( -3.310556943750001313, 17.50000000000001421, -65.85160580289945642 ) ) ;
#13842=CARTESIAN_POINT ( 'NONE',  ( 1.750000000000001110, 20.53108891324555785, -119.2943141357548313 ) ) ;
#13843=CARTESIAN_POINT ( 'NONE',  ( 1.655278471874998436, 14.63297358603754716, -104.4307724695661364 ) ) ;
#13845=DIRECTION ( 'NONE',  ( 0.000000000000000000, 1.000000000000000000, 0.000000000000000000 ) ) ;
#13847=CARTESIAN_POINT ( 'NONE',  ( -3.500000000000001332, 17.50000000000001421, -70.96098080242151696 ) ) ;
#13848=CARTESIAN_POINT ( 'NONE',  ( 3.500000000000001332, 19.52072594216371826, -122.3776474690881741 ) ) ;
#13849=CARTESIAN_POINT ( 'NONE',  ( -1.655278471874999990, 20.36702641396248481, -38.93077246956613635 ) ) ;
#13850=CARTESIAN_POINT ( 'NONE',  ( -1.655278471874999990, 20.36702641396249192, -95.01827246956612782 ) ) ;
#13851=( BOUNDED_CURVE ( )  B_SPLINE_CURVE ( 2, ( #10365, #9746, #32689, #22707, #7379, #33108, #26326, #36090, #23340 ),
 .UNSPECIFIED., .F., .T. ) 
 B_SPLINE_CURVE_WITH_KNOTS ( ( 3, 2, 2, 2, 3 ),
 ( 0.3145833333333333259, 0.3152777777777777679, 0.3166666666666666519, 0.3180555555555555358, 0.3187499999999999778 ),
 .UNSPECIFIED. ) 
 CURVE ( )  GEOMETRIC_REPRESENTATION_ITEM ( )  RATIONAL_B_SPLINE_CURVE ( ( 0.9330127018922194093, 0.9330127018922194093, 1.000000000000000000, 0.8660254037844387076, 1.000000000000000000, 0.8660254037844387076, 1.000000000000000000, 0.9330127018922194093, 0.9330127018922194093 ) ) 
 REPRESENTATION_ITEM ( '' )  );
#13852=CARTESIAN_POINT ( 'NONE',  ( -7.424026671074350129E-16, 13.45854811567263454, -60.40473080337742573 ) ) ;
#13854=CARTESIAN_POINT ( 'NONE',  ( -3.310556943750001313, 17.50000000000002132, -111.8516058028994564 ) ) ;
#13855=CARTESIAN_POINT ( 'NONE',  ( 3.310556943750001313, 19.41135094264166128, -45.26827246956613493 ) ) ;
#13861=CARTESIAN_POINT ( 'NONE',  ( -1.655278471875002211, 14.63297358603754716, -92.59743913623280775 ) ) ;
#13862=CARTESIAN_POINT ( 'NONE',  ( 3.500000000000000000, 15.47927405783632082, -39.23806413671076854 ) ) ;
#13864=ORIENTED_EDGE ( 'NONE', *, *, #40868, .F. ) ;
#13866=( BOUNDED_CURVE ( )  B_SPLINE_CURVE ( 2, ( #22383, #35979, #35573, #35362, #36186, #38972, #6436, #3035, #41967 ),
 .UNSPECIFIED., .F., .T. ) 
 B_SPLINE_CURVE_WITH_KNOTS ( ( 3, 2, 2, 2, 3 ),
 ( 0.9520833333333332815, 0.9527777777777777235, 0.9541666666666667185, 0.9555555555555556024, 0.9562500000000000444 ),
 .UNSPECIFIED. ) 
 CURVE ( )  GEOMETRIC_REPRESENTATION_ITEM ( )  RATIONAL_B_SPLINE_CURVE ( ( 0.9330127018922194093, 0.9330127018922194093, 1.000000000000000000, 0.8660254037844387076, 1.000000000000000000, 0.8660254037844387076, 1.000000000000000000, 0.9330127018922194093, 0.9330127018922194093 ) ) 
 REPRESENTATION_ITEM ( '' )  );
#13869=CARTESIAN_POINT ( 'NONE',  ( 1.750000000000001110, 20.53108891324555785, -122.9880641367107614 ) ) ;
#13870=EDGE_LOOP ( 'NONE', ( #40826, #20251, #26075, #36849 ) ) ;
#13873=CARTESIAN_POINT ( 'NONE',  ( -1.655278471874999990, 20.36702641396248481, -30.93077246956614346 ) ) ;
#13874=VERTEX_POINT ( 'NONE', #11416 ) ;
#13876=VECTOR ( 'NONE', #22026, 1000.000000000000000 ) ;
#13883=CARTESIAN_POINT ( 'NONE',  ( 7.785697387528201340E-15, 14.00000000000002487, -137.4047308033774470 ) ) ;
#13884=CARTESIAN_POINT ( 'NONE',  ( -0.9378221735089291577, 21.00000000000002487, -136.1663226036829997 ) ) ;
#13885=CARTESIAN_POINT ( 'NONE',  ( -7.022189441860112050E-16, 13.67729811471672718, -130.6016058028994280 ) ) ;
#13886=CARTESIAN_POINT ( 'NONE',  ( -3.500000000000001332, 17.50000000000001066, -27.96098080242151340 ) ) ;
#13887=ADVANCED_FACE ( 'NONE', ( #34590 ), #21615, .T. ) ;
#13889=CARTESIAN_POINT ( 'NONE',  ( -3.500000000000001332, 17.50000000000002487, -142.6547308033774186 ) ) ;
#13892=CARTESIAN_POINT ( 'NONE',  ( 3.500000000000001776, 19.52072594216372181, -134.3776474690881741 ) ) ;
#13893=CARTESIAN_POINT ( 'NONE',  ( 1.655278471874998436, 14.63297358603754894, -117.4307724695661364 ) ) ;
#13896=CARTESIAN_POINT ( 'NONE',  ( -7.424026671074350129E-16, 13.45854811567263631, -86.71098080242151696 ) ) ;
#13898=CARTESIAN_POINT ( 'NONE',  ( -3.310556943750000425, 19.41135094264166128, -54.84743913623280775 ) ) ;
#13899=CARTESIAN_POINT ( 'NONE',  ( -7.022189441860112050E-16, 13.67729811471672718, -111.6016058028994706 ) ) ;
#13901=CARTESIAN_POINT ( 'NONE',  ( -7.424026671074350129E-16, 13.45854811567263098, -28.40473080337743994 ) ) ;
#13902=CARTESIAN_POINT ( 'NONE',  ( 4.648177544792955347E-16, 21.00000000000002132, -116.2109808024215027 ) ) ;
#13905=CARTESIAN_POINT ( 'NONE',  ( 1.655278471875001101, 20.36702641396249547, -128.1849391362327992 ) ) ;
#13909=CARTESIAN_POINT ( 'NONE',  ( -3.310556943750000425, 19.41135094264166128, -62.93493913623279212 ) ) ;
#13910=EDGE_CURVE ( 'NONE', #22667, #30683, #23565, .T. ) ;
#13912=ORIENTED_EDGE ( 'NONE', *, *, #25876, .F. ) ;
#13913=CARTESIAN_POINT ( 'NONE',  ( -1.655278471875002211, 14.63297358603754716, -81.68493913623279923 ) ) ;
#13919=CARTESIAN_POINT ( 'NONE',  ( -3.310556943750002201, 15.58864905735836714, -47.68077246956614346 ) ) ;
#13921=CARTESIAN_POINT ( 'NONE',  ( -7.022189441860112050E-16, 13.67729811471672541, -101.5141058028994792 ) ) ;
#13923=AXIS2_PLACEMENT_3D ( 'NONE', #34243, #11081, #11684 ) ;
#13926=VERTEX_POINT ( 'NONE', #5877 ) ;
#13928=CARTESIAN_POINT ( 'NONE',  ( 1.655278471875001101, 20.36702641396248836, -54.09743913623281486 ) ) ;
#13929=( BOUNDED_CURVE ( )  B_SPLINE_CURVE ( 2, ( #26675, #14335, #14123, #24133, #20721, #33697, #10510, #942, #33897 ),
 .UNSPECIFIED., .F., .T. ) 
 B_SPLINE_CURVE_WITH_KNOTS ( ( 3, 2, 2, 2, 3 ),
 ( 0.7062500000000000444, 0.7069444444444444864, 0.7083333333333333703, 0.7097222222222222543, 0.7104166666666666963 ),
 .UNSPECIFIED. ) 
 CURVE ( )  GEOMETRIC_REPRESENTATION_ITEM ( )  RATIONAL_B_SPLINE_CURVE ( ( 0.9330127018922194093, 0.9330127018922194093, 1.000000000000000000, 0.8660254037844387076, 1.000000000000000000, 0.8660254037844387076, 1.000000000000000000, 0.9330127018922194093, 0.9330127018922194093 ) ) 
 REPRESENTATION_ITEM ( '' )  );
#13936=LINE ( 'NONE', #968, #4134 ) ;
#13938=ORIENTED_EDGE ( 'NONE', *, *, #3328, .F. ) ;
#13940=CARTESIAN_POINT ( 'NONE',  ( -3.500000000000000888, 19.52072594216370405, -43.04431413575483134 ) ) ;
#13944=CARTESIAN_POINT ( 'NONE',  ( -3.500000000000001332, 17.50000000000002132, -110.6547308033774328 ) ) ;
#13947=CARTESIAN_POINT ( 'NONE',  ( -3.310556943750001313, 17.50000000000001066, -27.85160580289947063 ) ) ;
#13948=CARTESIAN_POINT ( 'NONE',  ( -0.9378221735089310451, 14.00000000000002132, -97.44938900211596433 ) ) ;
#13949=CARTESIAN_POINT ( 'NONE',  ( 1.655278471875001101, 20.36702641396249192, -85.18493913623278502 ) ) ;
#13950=CARTESIAN_POINT ( 'NONE',  ( -1.655278471874999990, 20.36702641396249902, -135.9307724695661364 ) ) ;
#13954=CARTESIAN_POINT ( 'NONE',  ( 3.500000000000000000, 15.47927405783632793, -85.54431413575483134 ) ) ;
#13955=CARTESIAN_POINT ( 'NONE',  ( 3.310556943749999981, 15.58864905735837425, -128.4349391362327992 ) ) ;
#13956=DIRECTION ( 'NONE',  ( -0.000000000000000000, 1.259100132267607459E-16, -1.000000000000000000 ) ) ;
#13957=CARTESIAN_POINT ( 'NONE',  ( 3.310556943750001313, 19.41135094264166483, -86.18077246956613635 ) ) ;
#13958=CARTESIAN_POINT ( 'NONE',  ( 3.500000000000001332, 19.52072594216370405, -24.37764746908817415 ) ) ;
#13960=CARTESIAN_POINT ( 'NONE',  ( 1.750000000000001110, 20.53108891324555074, -66.98806413671076143 ) ) ;
#13961=CARTESIAN_POINT ( 'NONE',  ( -7.424026671074350129E-16, 13.45854811567263454, -72.40473080337743284 ) ) ;
#13962=CARTESIAN_POINT ( 'NONE',  ( -1.655278471875002211, 14.63297358603754184, -53.68493913623280633 ) ) ;
#13964=DIRECTION ( 'NONE',  ( 0.000000000000000000, 1.000000000000000000, 0.000000000000000000 ) ) ;
#13966=CARTESIAN_POINT ( 'NONE',  ( 1.655278471874998436, 14.63297358603754361, -79.51827246956614204 ) ) ;
#13967=CARTESIAN_POINT ( 'NONE',  ( 1.655278471874998436, 14.63297358603755249, -141.5182724695661420 ) ) ;
#13969=CARTESIAN_POINT ( 'NONE',  ( -3.310556943750002201, 15.58864905735837425, -107.6807724695661506 ) ) ;
#13970=CARTESIAN_POINT ( 'NONE',  ( -7.022189441860112050E-16, 13.67729811471672186, -76.51410580289947916 ) ) ;
#13971=DIRECTION ( 'NONE',  ( -0.000000000000000000, 1.259100132267607459E-16, -1.000000000000000000 ) ) ;
#13972=ORIENTED_EDGE ( 'NONE', *, *, #42045, .F. ) ;
#13973=CARTESIAN_POINT ( 'NONE',  ( -7.022189441860112050E-16, 13.67729811471672541, -100.6016058028994706 ) ) ;
#13974=CARTESIAN_POINT ( 'NONE',  ( 1.750000000000001110, 20.53108891324555785, -101.9880641367107756 ) ) ;
#13977=CARTESIAN_POINT ( 'NONE',  ( -1.394453263437886604E-15, 14.00000000000001776, -86.40473080337743284 ) ) ;
#13978=CARTESIAN_POINT ( 'NONE',  ( -3.500000000000000000, 19.52072594216371115, -81.73806413671074722 ) ) ;
#13980=CARTESIAN_POINT ( 'NONE',  ( -1.655278471874999990, 20.36702641396248836, -62.93077246956614346 ) ) ;
#13982=CARTESIAN_POINT ( 'NONE',  ( -1.655278471874999990, 20.36702641396249547, -114.9307724695661364 ) ) ;
#13983=DIRECTION ( 'NONE',  ( -0.000000000000000000, 1.259100132267607459E-16, -1.000000000000000000 ) ) ;
#13986=VERTEX_POINT ( 'NONE', #41403 ) ;
#13988=ADVANCED_FACE ( 'NONE', ( #31610 ), #28625, .T. ) ;
#13993=CARTESIAN_POINT ( 'NONE',  ( 3.310556943750001313, 19.41135094264166128, -70.18077246956613635 ) ) ;
#13994=ORIENTED_EDGE ( 'NONE', *, *, #28841, .F. ) ;
#13996=( BOUNDED_CURVE ( )  B_SPLINE_CURVE ( 2, ( #2340, #9571, #25104, #37858, #2758, #35086, #12542, #15961, #41052 ),
 .UNSPECIFIED., .F., .T. ) 
 B_SPLINE_CURVE_WITH_KNOTS ( ( 3, 2, 2, 2, 3 ),
 ( 0.5479166666666667185, 0.5486111111111111605, 0.5500000000000000444, 0.5513888888888889284, 0.5520833333333333703 ),
 .UNSPECIFIED. ) 
 CURVE ( )  GEOMETRIC_REPRESENTATION_ITEM ( )  RATIONAL_B_SPLINE_CURVE ( ( 0.9330127018922194093, 0.9330127018922194093, 1.000000000000000000, 0.8660254037844387076, 1.000000000000000000, 0.8660254037844387076, 1.000000000000000000, 0.9330127018922194093, 0.9330127018922194093 ) ) 
 REPRESENTATION_ITEM ( '' )  );
#13997=CARTESIAN_POINT ( 'NONE',  ( -0.9378221735089291577, 21.00000000000001776, -87.16632260368298546 ) ) ;
#13998=CARTESIAN_POINT ( 'NONE',  ( 3.500000000000001332, 17.50000000000002132, -112.1547308033774328 ) ) ;
#14003=CARTESIAN_POINT ( 'NONE',  ( 3.310556943750001313, 19.41135094264167549, -136.1807724695661364 ) ) ;
#14007=CARTESIAN_POINT ( 'NONE',  ( -7.022189441860112050E-16, 13.67729811471671653, -43.60160580289947063 ) ) ;
#14008=CARTESIAN_POINT ( 'NONE',  ( 0.9378221735089367073, 14.00000000000002487, -134.6663226036829712 ) ) ;
#14009=CARTESIAN_POINT ( 'NONE',  ( -3.310556943750000425, 19.41135094264165772, -37.93493913623280633 ) ) ;
#14010=CARTESIAN_POINT ( 'NONE',  ( -3.310556943750002645, 15.58864905735837425, -97.76827246956611361 ) ) ;
#14013=CARTESIAN_POINT ( 'NONE',  ( -3.310556943750000425, 19.41135094264167549, -142.9349391362327992 ) ) ;
#14014=DIRECTION ( 'NONE',  ( 0.000000000000000000, 1.000000000000000000, 0.000000000000000000 ) ) ;
#14015=CARTESIAN_POINT ( 'NONE',  ( 1.749999999999998224, 14.46891108675448301, -100.6276474690881741 ) ) ;
#14018=CARTESIAN_POINT ( 'NONE',  ( -7.424026671074350129E-16, 13.45854811567263631, -92.40473080337743284 ) ) ;
#14019=CARTESIAN_POINT ( 'NONE',  ( 3.310556943749999981, 15.58864905735836714, -68.43493913623279923 ) ) ;
#14024=CARTESIAN_POINT ( 'NONE',  ( 3.500000000000000000, 15.47927405783632082, -53.54431413575483845 ) ) ;
#14029=CARTESIAN_POINT ( 'NONE',  ( -1.750000000000002220, 14.46891108675447768, -45.48806413671076143 ) ) ;
#14030=DIRECTION ( 'NONE',  ( -0.000000000000000000, 1.259100132267607459E-16, -1.000000000000000000 ) ) ;
#14031=CARTESIAN_POINT ( 'NONE',  ( 3.310556943749999981, 15.58864905735836182, -28.43493913623279212 ) ) ;
#14032=CARTESIAN_POINT ( 'NONE',  ( 0.000000000000000000, 17.50000000000002487, -149.5231586289125687 ) ) ;
#14035=CARTESIAN_POINT ( 'NONE',  ( -0.9378221735089310451, 14.00000000000002132, -106.7556390011600200 ) ) ;
#14037=CARTESIAN_POINT ( 'NONE',  ( 3.310556943750001313, 19.41135094264166838, -78.18077246956613635 ) ) ;
#14038=CARTESIAN_POINT ( 'NONE',  ( -1.394453263437886604E-15, 14.00000000000002132, -133.7109808024214885 ) ) ;
#14039=ORIENTED_EDGE ( 'NONE', *, *, #20690, .F. ) ;
#14040=DIRECTION ( 'NONE',  ( 0.000000000000000000, 1.000000000000000000, 0.000000000000000000 ) ) ;
#14042=VERTEX_POINT ( 'NONE', #41614 ) ;
#14045=CARTESIAN_POINT ( 'NONE',  ( 1.655278471875001101, 20.36702641396249192, -87.09743913623280775 ) ) ;
#14046=ORIENTED_EDGE ( 'NONE', *, *, #33772, .F. ) ;
#14047=EDGE_LOOP ( 'NONE', ( #5809, #23625, #2191, #37279 ) ) ;
#14049=EDGE_CURVE ( 'NONE', #29511, #8532, #15250, .T. ) ;
#14051=DIRECTION ( 'NONE',  ( 0.000000000000000000, 1.000000000000000000, 0.000000000000000000 ) ) ;
#14052=CARTESIAN_POINT ( 'NONE',  ( -7.022189441860112050E-16, 13.67729811471672718, -126.5141058028994507 ) ) ;
#14053=CARTESIAN_POINT ( 'NONE',  ( -0.9378221735089310451, 14.00000000000002132, -94.75563900116002003 ) ) ;
#14054=CARTESIAN_POINT ( 'NONE',  ( 3.310556943750001313, 19.41135094264166128, -55.26827246956612782 ) ) ;
#14055=CARTESIAN_POINT ( 'NONE',  ( 3.310556943750001313, 19.41135094264166838, -113.2682724695661562 ) ) ;
#14058=CARTESIAN_POINT ( 'NONE',  ( 3.500000000000001776, 19.52072594216371826, -125.0713974700440900 ) ) ;
#14059=CARTESIAN_POINT ( 'NONE',  ( -3.310556943750002645, 15.58864905735836537, -38.68077246956613635 ) ) ;
#14060=CARTESIAN_POINT ( 'NONE',  ( -1.655278471875002211, 14.63297358603754361, -65.68493913623279923 ) ) ;
#14061=CARTESIAN_POINT ( 'NONE',  ( -1.749999999999999778, 20.53108891324555785, -119.1276474690881741 ) ) ;
#14062=CARTESIAN_POINT ( 'NONE',  ( 3.310556943750001313, 19.41135094264166838, -104.1807724695661221 ) ) ;
#14063=CYLINDRICAL_SURFACE ( 'NONE', #5640, 3.499999999999999556 ) ;
#14065=LINE ( 'NONE', #23855, #10972 ) ;
#14067=CARTESIAN_POINT ( 'NONE',  ( 2.474675557024783212E-16, 21.54145188432739388, -72.21098080242151696 ) ) ;
#14068=CARTESIAN_POINT ( 'NONE',  ( 1.749999999999998224, 14.46891108675448301, -100.6276474690881741 ) ) ;
#14069=CARTESIAN_POINT ( 'NONE',  ( 1.655278471875001101, 20.36702641396248481, -37.09743913623281486 ) ) ;
#14070=CARTESIAN_POINT ( 'NONE',  ( -1.655278471875002211, 14.63297358603754716, -91.68493913623279923 ) ) ;
#14071=CARTESIAN_POINT ( 'NONE',  ( 1.749999999999998224, 14.46891108675447768, -59.32139747004409713 ) ) ;
#14073=CARTESIAN_POINT ( 'NONE',  ( 1.655278471874998436, 14.63297358603754894, -110.5182724695661420 ) ) ;
#14074=CARTESIAN_POINT ( 'NONE',  ( -3.310556943750001313, 17.50000000000001066, -43.85160580289947063 ) ) ;
#14080=LINE ( 'NONE', #27053, #5496 ) ;
#14081=CARTESIAN_POINT ( 'NONE',  ( -3.310556943750001313, 17.50000000000001776, -93.76410580289947916 ) ) ;
#14085=CARTESIAN_POINT ( 'NONE',  ( 3.500000000000001332, 17.50000000000001421, -57.46098080242150985 ) ) ;
#14092=CARTESIAN_POINT ( 'NONE',  ( 3.500000000000000000, 15.47927405783633326, -118.2380641367107472 ) ) ;
#14098=CARTESIAN_POINT ( 'NONE',  ( 0.000000000000000000, 17.50000000000002487, -149.5231586289125687 ) ) ;
#14099=LINE ( 'NONE', #28311, #11264 ) ;
#14100=CARTESIAN_POINT ( 'NONE',  ( 3.310556943750001313, 17.50000000000002487, -142.2641058028994792 ) ) ;
#14103=CARTESIAN_POINT ( 'NONE',  ( -3.310556943750000425, 19.41135094264167549, -129.9349391362327992 ) ) ;
#14104=CARTESIAN_POINT ( 'NONE',  ( 3.500000000000001332, 17.50000000000001066, -28.46098080242151340 ) ) ;
#14106=CARTESIAN_POINT ( 'NONE',  ( 3.500000000000001332, 17.50000000000002487, -140.1547308033774186 ) ) ;
#14107=( BOUNDED_CURVE ( )  B_SPLINE_CURVE ( 2, ( #41887, #38680, #9552, #38047, #2739, #8908, #32300, #41670, #22728 ),
 .UNSPECIFIED., .F., .T. ) 
 B_SPLINE_CURVE_WITH_KNOTS ( ( 3, 2, 2, 2, 3 ),
 ( 0.2437499999999999944, 0.2444444444444444364, 0.2458333333333333204, 0.2472222222222222321, 0.2479166666666666741 ),
 .UNSPECIFIED. ) 
 CURVE ( )  GEOMETRIC_REPRESENTATION_ITEM ( )  RATIONAL_B_SPLINE_CURVE ( ( 0.9330127018922194093, 0.9330127018922194093, 1.000000000000000000, 0.8660254037844387076, 1.000000000000000000, 0.8660254037844387076, 1.000000000000000000, 0.9330127018922194093, 0.9330127018922194093 ) ) 
 REPRESENTATION_ITEM ( '' )  );
#14109=CARTESIAN_POINT ( 'NONE',  ( -3.500000000000002220, 15.47927405783633503, -134.8776474690881741 ) ) ;
#14110=CARTESIAN_POINT ( 'NONE',  ( -3.310556943750002645, 15.58864905735837780, -115.6807724695661364 ) ) ;
#14113=CARTESIAN_POINT ( 'NONE',  ( 1.750000000000001110, 20.53108891324555429, -83.29431413575483134 ) ) ;
#14114=CARTESIAN_POINT ( 'NONE',  ( -1.655278471875002211, 14.63297358603754184, -53.59743913623281486 ) ) ;
#14115=CARTESIAN_POINT ( 'NONE',  ( -1.655278471875002211, 14.63297358603755072, -113.6849391362327992 ) ) ;
#14119=CARTESIAN_POINT ( 'NONE',  ( -7.022189441860112050E-16, 13.67729811471672896, -127.6016058028994706 ) ) ;
#14122=CARTESIAN_POINT ( 'NONE',  ( 1.750000000000001110, 20.53108891324556140, -142.9880641367107614 ) ) ;
#14123=CARTESIAN_POINT ( 'NONE',  ( 1.749999999999998224, 14.46891108675447768, -58.62764746908817415 ) ) ;
#14124=CARTESIAN_POINT ( 'NONE',  ( 3.310556943750001313, 19.41135094264166128, -65.26827246956614204 ) ) ;
#14125=ORIENTED_EDGE ( 'NONE', *, *, #19211, .T. ) ;
#14126=CARTESIAN_POINT ( 'NONE',  ( -3.310556943750000425, 19.41135094264166838, -81.93493913623278502 ) ) ;
#14128=CARTESIAN_POINT ( 'NONE',  ( 3.500000000000001332, 17.50000000000001066, -26.15473080337743639 ) ) ;
#14131=CARTESIAN_POINT ( 'NONE',  ( 3.310556943750001313, 17.50000000000001066, -44.26410580289947916 ) ) ;
#14133=CARTESIAN_POINT ( 'NONE',  ( 3.310556943749999981, 15.58864905735837070, -101.3474391362328220 ) ) ;
#14135=ORIENTED_EDGE ( 'NONE', *, *, #8792, .T. ) ;
#14139=CARTESIAN_POINT ( 'NONE',  ( 3.310556943749999981, 15.58864905735836182, -52.34743913623281486 ) ) ;
#14141=ORIENTED_EDGE ( 'NONE', *, *, #24827, .T. ) ;
#14142=DIRECTION ( 'NONE',  ( 0.000000000000000000, 1.000000000000000000, 0.000000000000000000 ) ) ;
#14143=CARTESIAN_POINT ( 'NONE',  ( -3.500000000000001332, 17.50000000000001776, -91.65473080337743284 ) ) ;
#14145=FACE_OUTER_BOUND ( 'NONE', #2204, .T. ) ;
#14148=CARTESIAN_POINT ( 'NONE',  ( -3.500000000000000888, 19.52072594216370405, -42.04431413575483845 ) ) ;
#14151=ADVANCED_FACE ( 'NONE', ( #16914 ), #3310, .F. ) ;
#14153=CARTESIAN_POINT ( 'NONE',  ( -7.022189441860112050E-16, 13.67729811471671475, -28.60160580289947063 ) ) ;
#14154=CARTESIAN_POINT ( 'NONE',  ( -1.394453263437886604E-15, 14.00000000000002132, -122.4047308033774044 ) ) ;
#14155=CARTESIAN_POINT ( 'NONE',  ( 3.310556943750001313, 17.50000000000001776, -83.35160580289947063 ) ) ;
#14156=CARTESIAN_POINT ( 'NONE',  ( 3.310556943749999981, 15.58864905735837425, -132.3474391362328220 ) ) ;
#14159=CARTESIAN_POINT ( 'NONE',  ( -3.500000000000001332, 17.50000000000001776, -75.65473080337741862 ) ) ;
#14160=CARTESIAN_POINT ( 'NONE',  ( -3.310556943750002645, 15.58864905735837780, -127.7682724695661136 ) ) ;
#14162=CARTESIAN_POINT ( 'NONE',  ( 3.310556943749999981, 15.58864905735836892, -86.34743913623279354 ) ) ;
#14163=FACE_OUTER_BOUND ( 'NONE', #8671, .T. ) ;
#14164=CARTESIAN_POINT ( 'NONE',  ( 0.9378221735089281585, 14.00000000000002132, -101.3600726046389013 ) ) ;
#14165=CARTESIAN_POINT ( 'NONE',  ( 0.9378221735089281585, 14.00000000000000711, -25.36007260463891555 ) ) ;
#14166=CARTESIAN_POINT ( 'NONE',  ( -1.749999999999999778, 20.53108891324555074, -71.82139747004409003 ) ) ;
#14167=CARTESIAN_POINT ( 'NONE',  ( 2.340729813953370519E-16, 21.32270188528331190, -56.10160580289947774 ) ) ;
#14172=CARTESIAN_POINT ( 'NONE',  ( -3.310556943750001313, 17.50000000000001776, -78.85160580289945642 ) ) ;
#14173=CARTESIAN_POINT ( 'NONE',  ( 2.340729813953370519E-16, 21.32270188528332255, -140.1016058028994564 ) ) ;
#14175=CARTESIAN_POINT ( 'NONE',  ( -3.310556943750001313, 17.50000000000002132, -107.7641058028994649 ) ) ;
#14176=CARTESIAN_POINT ( 'NONE',  ( -3.310556943750002645, 15.58864905735837070, -76.68077246956615056 ) ) ;
#14177=CARTESIAN_POINT ( 'NONE',  ( -1.749999999999999778, 20.53108891324555429, -101.1276474690881741 ) ) ;
#14178=ORIENTED_EDGE ( 'NONE', *, *, #17883, .F. ) ;
#14179=CARTESIAN_POINT ( 'NONE',  ( -3.310556943750000425, 19.41135094264166838, -96.93493913623279923 ) ) ;
#14180=CARTESIAN_POINT ( 'NONE',  ( -1.750000000000002220, 14.46891108675448478, -99.48806413671077564 ) ) ;
#14182=CARTESIAN_POINT ( 'NONE',  ( -3.500000000000000000, 19.52072594216371115, -85.73806413671076143 ) ) ;
#14184=CARTESIAN_POINT ( 'NONE',  ( -0.9378221735089310451, 14.00000000000001066, -51.75563900116002714 ) ) ;
#14186=CARTESIAN_POINT ( 'NONE',  ( -1.655278471875002211, 14.63297358603754361, -62.59743913623280775 ) ) ;
#14188=CARTESIAN_POINT ( 'NONE',  ( -3.500000000000002220, 15.47927405783633503, -112.8776474690881599 ) ) ;
#14189=CARTESIAN_POINT ( 'NONE',  ( -1.655278471875002211, 14.63297358603755072, -114.5974391362327935 ) ) ;
#14190=CARTESIAN_POINT ( 'NONE',  ( 3.500000000000000000, 15.47927405783632082, -36.54431413575484555 ) ) ;
#14191=ADVANCED_FACE ( 'NONE', ( #16099 ), #10114, .T. ) ;
#14193=ORIENTED_EDGE ( 'NONE', *, *, #24323, .F. ) ;
#14194=ORIENTED_EDGE ( 'NONE', *, *, #32932, .T. ) ;
#14197=CARTESIAN_POINT ( 'NONE',  ( 3.500000000000001332, 19.52072594216370405, -33.37764746908818125 ) ) ;
#14198=CARTESIAN_POINT ( 'NONE',  ( 3.310556943750001313, 19.41135094264166128, -69.18077246956613635 ) ) ;
#14200=ORIENTED_EDGE ( 'NONE', *, *, #1229, .F. ) ;
#14202=CARTESIAN_POINT ( 'NONE',  ( 0.9378221735089281585, 14.00000000000001776, -83.66632260368299967 ) ) ;
#14207=CARTESIAN_POINT ( 'NONE',  ( -7.022189441860112050E-16, 13.67729811471673074, -136.5141058028994792 ) ) ;
#14209=CARTESIAN_POINT ( 'NONE',  ( 3.310556943750001313, 17.50000000000001066, -43.35160580289947063 ) ) ;
#14210=DIRECTION ( 'NONE',  ( -0.000000000000000000, 1.259100132267607459E-16, -1.000000000000000000 ) ) ;
#14211=CARTESIAN_POINT ( 'NONE',  ( 3.310556943749999981, 15.58864905735836182, -38.43493913623279923 ) ) ;
#14212=CARTESIAN_POINT ( 'NONE',  ( 3.310556943750001313, 19.41135094264166483, -99.26827246956612782 ) ) ;
#14215=CARTESIAN_POINT ( 'NONE',  ( -1.655278471874999990, 20.36702641396249902, -142.0182724695661420 ) ) ;
#14217=CARTESIAN_POINT ( 'NONE',  ( 3.500000000000001332, 17.50000000000001776, -97.46098080242150274 ) ) ;
#14218=CARTESIAN_POINT ( 'NONE',  ( 1.750000000000001110, 20.53108891324556140, -132.2943141357548598 ) ) ;
#14219=EDGE_CURVE ( 'NONE', #7389, #5144, #32492, .T. ) ;
#14221=CARTESIAN_POINT ( 'NONE',  ( -1.749999999999999778, 20.53108891324555429, -85.82139747004409003 ) ) ;
#14222=CARTESIAN_POINT ( 'NONE',  ( -1.655278471874999990, 20.36702641396248836, -68.01827246956612782 ) ) ;
#14226=CARTESIAN_POINT ( 'NONE',  ( -0.9378221735089310451, 14.00000000000002309, -119.7556390011600342 ) ) ;
#14227=CARTESIAN_POINT ( 'NONE',  ( 1.750000000000001110, 20.53108891324555074, -51.29431413575484555 ) ) ;
#14229=CARTESIAN_POINT ( 'NONE',  ( -0.9378221735089291577, 21.00000000000001421, -46.86007260463890844 ) ) ;
#14230=CARTESIAN_POINT ( 'NONE',  ( 1.749999999999998224, 14.46891108675448301, -103.6276474690881741 ) ) ;
#14233=CARTESIAN_POINT ( 'NONE',  ( 3.500000000000001776, 19.52072594216371826, -115.0713974700440758 ) ) ;
#14235=CARTESIAN_POINT ( 'NONE',  ( -7.022189441860112050E-16, 13.67729811471671297, -24.60160580289946708 ) ) ;
#14238=CARTESIAN_POINT ( 'NONE',  ( -1.394453263437886604E-15, 14.00000000000001776, -102.4047308033774186 ) ) ;
#14240=CARTESIAN_POINT ( 'NONE',  ( -1.655278471875002211, 14.63297358603754539, -76.59743913623280775 ) ) ;
#14242=CARTESIAN_POINT ( 'NONE',  ( 1.749999999999998224, 14.46891108675448301, -98.62764746908817415 ) ) ;
#14243=( BOUNDED_CURVE ( )  B_SPLINE_CURVE ( 2, ( #29926, #26959, #39921, #17386, #20985, #33960, #36953, #1425, #27164 ),
 .UNSPECIFIED., .F., .T. ) 
 B_SPLINE_CURVE_WITH_KNOTS ( ( 3, 2, 2, 2, 3 ),
 ( 0.6187500000000000222, 0.6194444444444444642, 0.6208333333333333481, 0.6222222222222222321, 0.6229166666666666741 ),
 .UNSPECIFIED. ) 
 CURVE ( )  GEOMETRIC_REPRESENTATION_ITEM ( )  RATIONAL_B_SPLINE_CURVE ( ( 0.9330127018922194093, 0.9330127018922194093, 1.000000000000000000, 0.8660254037844387076, 1.000000000000000000, 0.8660254037844387076, 1.000000000000000000, 0.9330127018922194093, 0.9330127018922194093 ) ) 
 REPRESENTATION_ITEM ( '' )  );
#14244=ADVANCED_FACE ( 'NONE', ( #9488 ), #6509, .T. ) ;
#14246=ORIENTED_EDGE ( 'NONE', *, *, #2669, .T. ) ;
#14247=CARTESIAN_POINT ( 'NONE',  ( -3.500000000000000000, 19.52072594216371826, -120.7380641367107756 ) ) ;
#14248=CARTESIAN_POINT ( 'NONE',  ( -3.310556943750001313, 17.50000000000001776, -85.76410580289947916 ) ) ;
#14249=ORIENTED_EDGE ( 'NONE', *, *, #38769, .F. ) ;
#14250=ORIENTED_EDGE ( 'NONE', *, *, #21469, .T. ) ;
#14254=DIRECTION ( 'NONE',  ( -0.000000000000000000, 1.259100132267607459E-16, -1.000000000000000000 ) ) ;
#14256=CARTESIAN_POINT ( 'NONE',  ( -1.655278471874999990, 20.36702641396249547, -127.9307724695661364 ) ) ;
#14259=CARTESIAN_POINT ( 'NONE',  ( 1.655278471874998436, 14.63297358603754184, -56.51827246956612782 ) ) ;
#14260=CARTESIAN_POINT ( 'NONE',  ( 1.655278471875001101, 20.36702641396249547, -117.1849391362327850 ) ) ;
#14262=CARTESIAN_POINT ( 'NONE',  ( 1.749999999999998224, 14.46891108675448656, -125.3213974700440900 ) ) ;
#14263=EDGE_CURVE ( 'NONE', #5754, #24508, #6912, .T. ) ;
#14264=CARTESIAN_POINT ( 'NONE',  ( 2.340729813953370519E-16, 21.32270188528330479, -39.01410580289947916 ) ) ;
#14265=CARTESIAN_POINT ( 'NONE',  ( -3.310556943750000425, 19.41135094264166128, -68.93493913623279923 ) ) ;
#14266=CARTESIAN_POINT ( 'NONE',  ( 3.500000000000001776, 19.52072594216371826, -114.3776474690881599 ) ) ;
#14268=CARTESIAN_POINT ( 'NONE',  ( -7.022189441860112050E-16, 13.67729811471672541, -96.51410580289946495 ) ) ;
#14269=CARTESIAN_POINT ( 'NONE',  ( -1.394453263437886604E-15, 14.00000000000001421, -66.40473080337741862 ) ) ;
#14272=CARTESIAN_POINT ( 'NONE',  ( 2.474675557024783212E-16, 21.54145188432739388, -70.21098080242150274 ) ) ;
#14274=CARTESIAN_POINT ( 'NONE',  ( 0.9378221735089281585, 14.00000000000002132, -122.6663226036829855 ) ) ;
#14275=CARTESIAN_POINT ( 'NONE',  ( -1.655278471874999990, 20.36702641396248481, -30.93077246956614346 ) ) ;
#14276=CARTESIAN_POINT ( 'NONE',  ( -3.310556943750002645, 15.58864905735837247, -91.76827246956615625 ) ) ;
#14277=CARTESIAN_POINT ( 'NONE',  ( -3.500000000000000888, 19.52072594216370760, -56.73806413671076143 ) ) ;
#14279=CARTESIAN_POINT ( 'NONE',  ( 1.655278471874998436, 14.63297358603754894, -114.5182724695661278 ) ) ;
#14280=CARTESIAN_POINT ( 'NONE',  ( 3.310556943749999981, 15.58864905735836182, -41.43493913623279212 ) ) ;
#14282=CARTESIAN_POINT ( 'NONE',  ( -1.836030130193217234E-14, 21.00000000000002487, -135.2109808024214885 ) ) ;
#14287=CARTESIAN_POINT ( 'NONE',  ( -0.9378221735089291577, 21.00000000000001066, -23.86007260463890844 ) ) ;
#14288=CARTESIAN_POINT ( 'NONE',  ( -3.310556943750001313, 17.50000000000001776, -90.76410580289947916 ) ) ;
#14289=CARTESIAN_POINT ( 'NONE',  ( -3.500000000000001332, 17.50000000000002487, -135.6547308033774186 ) ) ;
#14293=AXIS2_PLACEMENT_3D ( 'NONE', #15464, #2054, #5456 ) ;
#14294=PRODUCT_DEFINITION_SHAPE ( 'NONE', 'NONE',  #6498 ) ;
#14296=CARTESIAN_POINT ( 'NONE',  ( 0.000000000000000000, 17.50000000000002487, -149.5231586289125687 ) ) ;
#14297=ORIENTED_EDGE ( 'NONE', *, *, #3273, .F. ) ;
#14300=VERTEX_POINT ( 'NONE', #29665 ) ;
#14304=VERTEX_POINT ( 'NONE', #529 ) ;
#14306=CARTESIAN_POINT ( 'NONE',  ( -3.500000000000002220, 15.47927405783632437, -53.87764746908817415 ) ) ;
#14308=CARTESIAN_POINT ( 'NONE',  ( -1.655278471875002211, 14.63297358603755427, -140.5974391362327935 ) ) ;
#14309=CARTESIAN_POINT ( 'NONE',  ( 3.500000000000000000, 15.47927405783632615, -68.54431413575484555 ) ) ;
#14310=ADVANCED_FACE ( 'NONE', ( #13502 ), #26489, .T. ) ;
#14312=CARTESIAN_POINT ( 'NONE',  ( 3.310556943750001313, 17.50000000000002132, -129.3516058028994564 ) ) ;
#14313=CARTESIAN_POINT ( 'NONE',  ( 1.655278471874998436, 14.63297358603754184, -56.51827246956612782 ) ) ;
#14314=VERTEX_POINT ( 'NONE', #10532 ) ;
#14316=CARTESIAN_POINT ( 'NONE',  ( 1.749999999999998224, 14.46891108675448834, -139.3213974700441042 ) ) ;
#14317=AXIS2_PLACEMENT_3D ( 'NONE', #19270, #32245, #20745 ) ;
#14319=CARTESIAN_POINT ( 'NONE',  ( 1.749999999999998224, 14.46891108675448656, -133.6276474690881741 ) ) ;
#14320=CARTESIAN_POINT ( 'NONE',  ( -3.310556943750001313, 17.50000000000002132, -112.7641058028994792 ) ) ;
#14323=CARTESIAN_POINT ( 'NONE',  ( -1.749999999999999778, 20.53108891324555429, -87.12764746908817415 ) ) ;
#14325=CARTESIAN_POINT ( 'NONE',  ( 1.655278471875001101, 20.36702641396248836, -50.09743913623280775 ) ) ;
#14326=CARTESIAN_POINT ( 'NONE',  ( 2.340729813953370519E-16, 21.32270188528331900, -106.1016058028994564 ) ) ;
#14328=CARTESIAN_POINT ( 'NONE',  ( -0.9378221735089291577, 21.00000000000001776, -80.16632260368298546 ) ) ;
#14330=CARTESIAN_POINT ( 'NONE',  ( 3.310556943749999981, 15.58864905735837425, -127.4349391362327992 ) ) ;
#14331=EDGE_CURVE ( 'NONE', #11503, #31753, #30880, .T. ) ;
#14334=CARTESIAN_POINT ( 'NONE',  ( 3.500000000000001332, 19.52072594216371826, -124.0713974700440758 ) ) ;
#14335=CARTESIAN_POINT ( 'NONE',  ( 0.9378221735089281585, 14.00000000000001243, -58.66632260368298546 ) ) ;
#14336=CARTESIAN_POINT ( 'NONE',  ( 3.310556943749999981, 15.58864905735836537, -58.43493913623279212 ) ) ;
#14337=EDGE_CURVE ( 'NONE', #31508, #17813, #36851, .T. ) ;
#14340=CARTESIAN_POINT ( 'NONE',  ( -7.022189441860112050E-16, 13.67729811471672186, -80.60160580289945642 ) ) ;
#14345=CARTESIAN_POINT ( 'NONE',  ( 1.655278471875001101, 20.36702641396248481, -40.09743913623281486 ) ) ;
#14346=CARTESIAN_POINT ( 'NONE',  ( 3.310556943750001313, 17.50000000000001776, -100.2641058028994792 ) ) ;
#14352=CARTESIAN_POINT ( 'NONE',  ( -3.310556943750002645, 15.58864905735836714, -53.68077246956612925 ) ) ;
#14355=ORIENTED_EDGE ( 'NONE', *, *, #10100, .F. ) ;
#14357=CARTESIAN_POINT ( 'NONE',  ( -0.9378221735089310451, 14.00000000000002132, -91.44938900211595012 ) ) ;
#14359=( BOUNDED_CURVE ( )  B_SPLINE_CURVE ( 2, ( #454, #13425, #36177, #7048, #20028, #39582, #10457, #23436, #26836 ),
 .UNSPECIFIED., .F., .F. ) 
 B_SPLINE_CURVE_WITH_KNOTS ( ( 3, 2, 2, 2, 3 ),
 ( 0.6854166666666666741, 0.6861111111111111160, 0.6875000000000000000, 0.6888888888888888840, 0.6895833333333333259 ),
 .UNSPECIFIED. ) 
 CURVE ( )  GEOMETRIC_REPRESENTATION_ITEM ( )  RATIONAL_B_SPLINE_CURVE ( ( 0.9330127018922194093, 0.9330127018922194093, 1.000000000000000000, 0.8660254037844387076, 1.000000000000000000, 0.8660254037844387076, 1.000000000000000000, 0.9330127018922194093, 0.9330127018922194093 ) ) 
 REPRESENTATION_ITEM ( '' )  );
#14360=CARTESIAN_POINT ( 'NONE',  ( 4.648177544792955347E-16, 21.00000000000001066, -39.21098080242150985 ) ) ;
#14361=EDGE_LOOP ( 'NONE', ( #28570, #15938, #11822, #26375 ) ) ;
#14363=CARTESIAN_POINT ( 'NONE',  ( -3.500000000000001332, 17.50000000000001066, -42.96098080242151696 ) ) ;
#14364=DIRECTION ( 'NONE',  ( -0.000000000000000000, 1.259100132267607459E-16, -1.000000000000000000 ) ) ;
#14367=CARTESIAN_POINT ( 'NONE',  ( 2.340729813953370519E-16, 21.32270188528330479, -30.10160580289947418 ) ) ;
#14369=CARTESIAN_POINT ( 'NONE',  ( 1.655278471874998436, 14.63297358603755072, -132.4307724695661364 ) ) ;
#14375=CARTESIAN_POINT ( 'NONE',  ( 1.655278471874998436, 14.63297358603754894, -120.5182724695661278 ) ) ;
#14377=CARTESIAN_POINT ( 'NONE',  ( -3.310556943750000425, 19.41135094264166483, -86.84743913623280775 ) ) ;
#14379=FACE_OUTER_BOUND ( 'NONE', #9392, .T. ) ;
#14380=CARTESIAN_POINT ( 'NONE',  ( -3.500000000000001332, 17.50000000000001421, -71.65473080337743284 ) ) ;
#14381=CARTESIAN_POINT ( 'NONE',  ( -3.310556943750000425, 19.41135094264166483, -52.93493913623280633 ) ) ;
#14383=FACE_OUTER_BOUND ( 'NONE', #15394, .T. ) ;
#14385=CARTESIAN_POINT ( 'NONE',  ( -3.310556943750001313, 17.50000000000001776, -79.85160580289945642 ) ) ;
#14386=CARTESIAN_POINT ( 'NONE',  ( 1.655278471875001101, 20.36702641396249902, -140.1849391362327708 ) ) ;
#14388=CARTESIAN_POINT ( 'NONE',  ( -3.310556943750002201, 15.58864905735837425, -101.6807724695661364 ) ) ;
#14389=CARTESIAN_POINT ( 'NONE',  ( 3.310556943750001313, 19.41135094264166483, -76.18077246956615056 ) ) ;
#14390=CARTESIAN_POINT ( 'NONE',  ( -0.9378221735089310451, 14.00000000000002309, -115.4493890021159501 ) ) ;
#14392=CARTESIAN_POINT ( 'NONE',  ( 2.340729813953370519E-16, 21.32270188528331190, -96.10160580289945642 ) ) ;
#14394=CARTESIAN_POINT ( 'NONE',  ( 1.750000000000001110, 20.53108891324555429, -91.29431413575484555 ) ) ;
#14395=DIRECTION ( 'NONE',  ( -0.000000000000000000, 1.259100132267607459E-16, -1.000000000000000000 ) ) ;
#14397=CARTESIAN_POINT ( 'NONE',  ( -1.655278471874999990, 20.36702641396248836, -56.93077246956614346 ) ) ;
#14399=CARTESIAN_POINT ( 'NONE',  ( 1.655278471875001101, 20.36702641396249547, -117.0974391362327935 ) ) ;
#14402=ADVANCED_FACE ( 'NONE', ( #21149 ), #24352, .T. ) ;
#14407=CARTESIAN_POINT ( 'NONE',  ( -1.655278471874999990, 20.36702641396248836, -66.93077246956613635 ) ) ;
#14408=ORIENTED_EDGE ( 'NONE', *, *, #629, .F. ) ;
#14409=ORIENTED_EDGE ( 'NONE', *, *, #40824, .T. ) ;
#14410=CARTESIAN_POINT ( 'NONE',  ( -1.750000000000002220, 14.46891108675448301, -86.79431413575483134 ) ) ;
#14412=CARTESIAN_POINT ( 'NONE',  ( 4.648177544792955347E-16, 21.00000000000001776, -83.21098080242150274 ) ) ;
#14416=CARTESIAN_POINT ( 'NONE',  ( 0.000000000000000000, 17.50000000000002487, -149.5231586289125687 ) ) ;
#14417=CARTESIAN_POINT ( 'NONE',  ( -1.655278471875002211, 14.63297358603755249, -135.5974391362328220 ) ) ;
#14418=CARTESIAN_POINT ( 'NONE',  ( -1.749999999999999778, 20.53108891324555429, -74.82139747004410424 ) ) ;
#14419=CARTESIAN_POINT ( 'NONE',  ( 3.310556943750001313, 19.41135094264166128, -47.26827246956614204 ) ) ;
#14420=LINE ( 'NONE', #18602, #35645 ) ;
#14421=CARTESIAN_POINT ( 'NONE',  ( 1.655278471874998436, 14.63297358603753828, -35.51827246956612782 ) ) ;
#14423=CARTESIAN_POINT ( 'NONE',  ( 3.310556943750001313, 19.41135094264166483, -100.2682724695661278 ) ) ;
#14424=EDGE_CURVE ( 'NONE', #7402, #14839, #13730, .T. ) ;
#14427=ADVANCED_FACE ( 'NONE', ( #39876 ), #23724, .T. ) ;
#14428=CARTESIAN_POINT ( 'NONE',  ( 3.310556943749999981, 15.58864905735837425, -136.4349391362327992 ) ) ;
#14430=CARTESIAN_POINT ( 'NONE',  ( -3.500000000000001332, 17.50000000000001776, -97.96098080242150274 ) ) ;
#14431=CARTESIAN_POINT ( 'NONE',  ( 0.9378221735089300459, 21.00000000000001776, -99.94938900211596433 ) ) ;
#14432=CARTESIAN_POINT ( 'NONE',  ( 1.750000000000001110, 20.53108891324555074, -64.29431413575484555 ) ) ;
#14433=CARTESIAN_POINT ( 'NONE',  ( 1.750000000000001110, 20.53108891324555429, -84.98806413671076143 ) ) ;
#14434=CARTESIAN_POINT ( 'NONE',  ( 3.310556943750001313, 17.50000000000001421, -69.35160580289947063 ) ) ;
#14435=( BOUNDED_CURVE ( )  B_SPLINE_CURVE ( 2, ( #10122, #32866, #19276, #7142, #26500, #39456, #9927, #29247, #26296 ),
 .UNSPECIFIED., .F., .F. ) 
 B_SPLINE_CURVE_WITH_KNOTS ( ( 3, 2, 2, 2, 3 ),
 ( 0.2104166666666666685, 0.2111111111111111105, 0.2124999999999999944, 0.2138888888888888784, 0.2145833333333333481 ),
 .UNSPECIFIED. ) 
 CURVE ( )  GEOMETRIC_REPRESENTATION_ITEM ( )  RATIONAL_B_SPLINE_CURVE ( ( 0.9330127018922194093, 0.9330127018922194093, 1.000000000000000000, 0.8660254037844387076, 1.000000000000000000, 0.8660254037844387076, 1.000000000000000000, 0.9330127018922180770, 0.9330127018922194093 ) ) 
 REPRESENTATION_ITEM ( '' )  );
#14439=LINE ( 'NONE', #37196, #27549 ) ;
#14440=CARTESIAN_POINT ( 'NONE',  ( -1.749999999999999778, 20.53108891324555074, -48.12764746908818125 ) ) ;
#14441=CARTESIAN_POINT ( 'NONE',  ( 1.655278471875001101, 20.36702641396249547, -122.0974391362328078 ) ) ;
#14442=CARTESIAN_POINT ( 'NONE',  ( 0.000000000000000000, 21.00000000000002487, -149.5231586289125687 ) ) ;
#14445=CARTESIAN_POINT ( 'NONE',  ( -3.500000000000000888, 19.52072594216371826, -114.7380641367107472 ) ) ;
#14446=CARTESIAN_POINT ( 'NONE',  ( 3.500000000000001332, 19.52072594216370760, -55.07139747004409713 ) ) ;
#14447=CARTESIAN_POINT ( 'NONE',  ( 0.9378221735089300459, 21.00000000000001776, -75.94938900211593591 ) ) ;
#14448=CARTESIAN_POINT ( 'NONE',  ( 4.648177544792955347E-16, 21.00000000000001421, -60.90473080337742573 ) ) ;
#14451=CARTESIAN_POINT ( 'NONE',  ( -3.310556943750001313, 17.50000000000001776, -75.76410580289946495 ) ) ;
#14452=CARTESIAN_POINT ( 'NONE',  ( -1.394453263437886604E-15, 14.00000000000001776, -96.71098080242150274 ) ) ;
#14454=CARTESIAN_POINT ( 'NONE',  ( 4.648177544792955347E-16, 21.00000000000001066, -26.90473080337742928 ) ) ;
#14457=VECTOR ( 'NONE', #39414, 1000.000000000000000 ) ;
#14458=CARTESIAN_POINT ( 'NONE',  ( -1.750000000000002220, 14.46891108675447946, -63.79431413575484555 ) ) ;
#14459=CARTESIAN_POINT ( 'NONE',  ( -1.655278471875002211, 14.63297358603754716, -85.59743913623279354 ) ) ;
#14461=ORIENTED_EDGE ( 'NONE', *, *, #40184, .F. ) ;
#14465=FACE_OUTER_BOUND ( 'NONE', #21029, .T. ) ;
#14466=ORIENTED_EDGE ( 'NONE', *, *, #3278, .T. ) ;
#14468=CARTESIAN_POINT ( 'NONE',  ( 2.340729813953370519E-16, 21.32270188528330834, -51.10160580289946353 ) ) ;
#14469=CARTESIAN_POINT ( 'NONE',  ( 3.310556943750001313, 19.41135094264166838, -115.2682724695661278 ) ) ;
#14470=ORIENTED_EDGE ( 'NONE', *, *, #39617, .T. ) ;
#14473=CARTESIAN_POINT ( 'NONE',  ( -3.500000000000001332, 17.50000000000002132, -122.6547308033774186 ) ) ;
#14474=ADVANCED_FACE ( 'NONE', ( #4774 ), #17756, .T. ) ;
#14475=CARTESIAN_POINT ( 'NONE',  ( 3.310556943749999981, 15.58864905735836182, -42.34743913623279354 ) ) ;
#14476=CARTESIAN_POINT ( 'NONE',  ( 3.310556943749999981, 15.58864905735836537, -64.43493913623279923 ) ) ;
#14477=CARTESIAN_POINT ( 'NONE',  ( 1.749999999999998224, 14.46891108675448478, -111.6276474690881884 ) ) ;
#14479=CARTESIAN_POINT ( 'NONE',  ( -3.310556943750001313, 17.50000000000001776, -95.76410580289946495 ) ) ;
#14480=CARTESIAN_POINT ( 'NONE',  ( -1.394453263437886604E-15, 14.00000000000001066, -47.40473080337742573 ) ) ;
#14481=CARTESIAN_POINT ( 'NONE',  ( 4.648177544792955347E-16, 21.00000000000001421, -51.90473080337743284 ) ) ;
#14482=FACE_OUTER_BOUND ( 'NONE', #1072, .T. ) ;
#14485=CARTESIAN_POINT ( 'NONE',  ( -1.750000000000002220, 14.46891108675447946, -64.79431413575484555 ) ) ;
#14487=CARTESIAN_POINT ( 'NONE',  ( 3.310556943750001313, 19.41135094264165772, -30.18077246956614701 ) ) ;
#14488=( BOUNDED_CURVE ( )  B_SPLINE_CURVE ( 2, ( #35131, #25151, #41945, #5791, #16206, #25362, #28535, #12588, #35339 ),
 .UNSPECIFIED., .F., .F. ) 
 B_SPLINE_CURVE_WITH_KNOTS ( ( 3, 2, 2, 2, 3 ),
 ( 0.5145833333333332815, 0.5152777777777777235, 0.5166666666666667185, 0.5180555555555556024, 0.5187500000000000444 ),
 .UNSPECIFIED. ) 
 CURVE ( )  GEOMETRIC_REPRESENTATION_ITEM ( )  RATIONAL_B_SPLINE_CURVE ( ( 0.9330127018922194093, 0.9330127018922194093, 1.000000000000000000, 0.8660254037844387076, 1.000000000000000000, 0.8660254037844387076, 1.000000000000000000, 0.9330127018922194093, 0.9330127018922194093 ) ) 
 REPRESENTATION_ITEM ( '' )  );
#14489=CARTESIAN_POINT ( 'NONE',  ( -3.310556943750001313, 17.50000000000001776, -88.85160580289947063 ) ) ;
#14490=CARTESIAN_POINT ( 'NONE',  ( 2.474675557024783212E-16, 21.54145188432739388, -52.90473080337742573 ) ) ;
#14491=FACE_OUTER_BOUND ( 'NONE', #7332, .T. ) ;
#14492=CARTESIAN_POINT ( 'NONE',  ( -1.655278471874999990, 20.36702641396249547, -114.0182724695661278 ) ) ;
#14493=CARTESIAN_POINT ( 'NONE',  ( 1.655278471875001101, 20.36702641396248481, -36.18493913623279923 ) ) ;
#14495=CARTESIAN_POINT ( 'NONE',  ( 1.750000000000001110, 20.53108891324555074, -53.29431413575484555 ) ) ;
#14499=CARTESIAN_POINT ( 'NONE',  ( -0.9378221735089310451, 14.00000000000000888, -23.44938900211595367 ) ) ;
#14500=CARTESIAN_POINT ( 'NONE',  ( -3.310556943750000425, 19.41135094264166838, -92.84743913623279354 ) ) ;
#14503=VERTEX_POINT ( 'NONE', #31554 ) ;
#14505=CARTESIAN_POINT ( 'NONE',  ( 4.648177544792955347E-16, 21.00000000000001066, -33.21098080242150274 ) ) ;
#14506=LINE ( 'NONE', #37258, #8138 ) ;
#14512=CARTESIAN_POINT ( 'NONE',  ( 1.749999999999998224, 14.46891108675448478, -118.3213974700440900 ) ) ;
#14514=VECTOR ( 'NONE', #25795, 1000.000000000000000 ) ;
#14516=CARTESIAN_POINT ( 'NONE',  ( 4.648177544792955347E-16, 21.00000000000001421, -65.21098080242150274 ) ) ;
#14521=CARTESIAN_POINT ( 'NONE',  ( -1.394453263437886604E-15, 14.00000000000001776, -89.71098080242148853 ) ) ;
#14523=CARTESIAN_POINT ( 'NONE',  ( -3.310556943750002645, 15.58864905735837958, -139.6807724695661364 ) ) ;
#14524=CARTESIAN_POINT ( 'NONE',  ( 1.750000000000001110, 20.53108891324554719, -37.98806413671076854 ) ) ;
#14527=CARTESIAN_POINT ( 'NONE',  ( 1.655278471875001101, 20.36702641396249902, -132.1849391362327992 ) ) ;
#14528=CARTESIAN_POINT ( 'NONE',  ( 1.655278471875001101, 20.36702641396248836, -54.18493913623280633 ) ) ;
#14529=ORIENTED_EDGE ( 'NONE', *, *, #6190, .F. ) ;
#14531=CARTESIAN_POINT ( 'NONE',  ( 1.749999999999998224, 14.46891108675448834, -141.3213974700441042 ) ) ;
#14532=EDGE_CURVE ( 'NONE', #11928, #10427, #6144, .T. ) ;
#14534=CARTESIAN_POINT ( 'NONE',  ( -7.424026671074350129E-16, 13.45854811567264164, -127.7109808024214885 ) ) ;
#14535=CARTESIAN_POINT ( 'NONE',  ( -3.310556943750000425, 19.41135094264166838, -110.8474391362328078 ) ) ;
#14537=CYLINDRICAL_SURFACE ( 'NONE', #7543, 3.499999999999999556 ) ;
#14538=CARTESIAN_POINT ( 'NONE',  ( -7.424026671074350129E-16, 13.45854811567263631, -81.71098080242150274 ) ) ;
#14540=CARTESIAN_POINT ( 'NONE',  ( 1.655278471874998436, 14.63297358603754006, -48.43077246956614346 ) ) ;
#14541=CARTESIAN_POINT ( 'NONE',  ( 3.310556943750001313, 17.50000000000002132, -109.3516058028994564 ) ) ;
#14546=CARTESIAN_POINT ( 'NONE',  ( -3.500000000000000000, 19.52072594216371115, -89.04431413575483134 ) ) ;
#14547=CARTESIAN_POINT ( 'NONE',  ( -1.655278471874999990, 20.36702641396249547, -126.0182724695661278 ) ) ;
#14551=CARTESIAN_POINT ( 'NONE',  ( -1.655278471874999990, 20.36702641396248836, -61.01827246956613493 ) ) ;
#14553=CARTESIAN_POINT ( 'NONE',  ( -1.655278471874999990, 20.36702641396249192, -78.01827246956614204 ) ) ;
#14556=CARTESIAN_POINT ( 'NONE',  ( 3.500000000000001332, 17.50000000000001776, -77.15473080337741862 ) ) ;
#14557=CARTESIAN_POINT ( 'NONE',  ( 3.500000000000001332, 19.52072594216370405, -26.07139747004409713 ) ) ;
#14560=CARTESIAN_POINT ( 'NONE',  ( -3.310556943750002201, 15.58864905735836714, -40.68077246956613635 ) ) ;
#14561=CARTESIAN_POINT ( 'NONE',  ( -7.022189441860112050E-16, 13.67729811471672363, -93.51410580289947916 ) ) ;
#14566=CARTESIAN_POINT ( 'NONE',  ( -7.022189441860112050E-16, 13.67729811471671653, -50.51410580289946495 ) ) ;
#14570=CARTESIAN_POINT ( 'NONE',  ( -1.394453263437886604E-15, 14.00000000000001066, -43.71098080242150985 ) ) ;
#14572=AXIS2_PLACEMENT_3D ( 'NONE', #3123, #33083, #19693 ) ;
#14573=LINE ( 'NONE', #23517, #24519 ) ;
#14576=DIRECTION ( 'NONE',  ( -0.000000000000000000, 1.259100132267607459E-16, -1.000000000000000000 ) ) ;
#14577=CARTESIAN_POINT ( 'NONE',  ( 2.474675557024783212E-16, 21.54145188432739033, -38.21098080242150985 ) ) ;
#14580=VECTOR ( 'NONE', #19503, 1000.000000000000000 ) ;
#14582=CARTESIAN_POINT ( 'NONE',  ( 3.310556943750001313, 17.50000000000001066, -23.35160580289946708 ) ) ;
#14584=CARTESIAN_POINT ( 'NONE',  ( -1.655278471875002211, 14.63297358603755249, -127.5974391362328078 ) ) ;
#14587=CARTESIAN_POINT ( 'NONE',  ( -1.394453263437886604E-15, 14.00000000000001066, -38.40473080337743284 ) ) ;
#14588=CARTESIAN_POINT ( 'NONE',  ( 2.340729813953370519E-16, 21.32270188528331900, -125.1016058028994564 ) ) ;
#14589=CARTESIAN_POINT ( 'NONE',  ( 3.500000000000001332, 19.52072594216371826, -141.0713974700441042 ) ) ;
#14590=CARTESIAN_POINT ( 'NONE',  ( 1.749999999999998224, 14.46891108675447413, -37.32139747004409003 ) ) ;
#14591=CARTESIAN_POINT ( 'NONE',  ( 4.648177544792955347E-16, 21.00000000000001776, -102.2109808024215027 ) ) ;
#14593=CARTESIAN_POINT ( 'NONE',  ( 4.648177544792955347E-16, 21.00000000000001066, -24.90473080337743284 ) ) ;
#14594=CARTESIAN_POINT ( 'NONE',  ( -3.500000000000002220, 15.47927405783632615, -68.57139747004410424 ) ) ;
#14595=CARTESIAN_POINT ( 'NONE',  ( -3.310556943750001313, 17.50000000000001421, -54.85160580289946353 ) ) ;
#14598=CARTESIAN_POINT ( 'NONE',  ( -3.310556943750002645, 15.58864905735837070, -76.76827246956612782 ) ) ;
#14600=CARTESIAN_POINT ( 'NONE',  ( 3.310556943750001313, 19.41135094264166838, -101.1807724695661364 ) ) ;
#14601=CARTESIAN_POINT ( 'NONE',  ( 3.310556943750001313, 17.50000000000001776, -76.26410580289946495 ) ) ;
#14602=ORIENTED_EDGE ( 'NONE', *, *, #5137, .F. ) ;
#14603=CARTESIAN_POINT ( 'NONE',  ( 3.310556943750001313, 17.50000000000001776, -95.35160580289945642 ) ) ;
#14604=AXIS2_PLACEMENT_3D ( 'NONE', #36072, #19916, #36501 ) ;
#14607=CARTESIAN_POINT ( 'NONE',  ( -1.394453263437886604E-15, 14.00000000000001066, -26.71098080242150985 ) ) ;
#14608=CARTESIAN_POINT ( 'NONE',  ( 3.500000000000001332, 17.50000000000002132, -117.4609808024215170 ) ) ;
#14609=CARTESIAN_POINT ( 'NONE',  ( 3.310556943750001313, 17.50000000000001421, -55.26410580289947916 ) ) ;
#14611=CARTESIAN_POINT ( 'NONE',  ( -3.310556943750001313, 17.50000000000002132, -108.7641058028994649 ) ) ;
#14612=( BOUNDED_CURVE ( )  B_SPLINE_CURVE ( 2, ( #5838, #31359, #2225, #41155, #12002, #22685, #29685, #29471, #26094 ),
 .UNSPECIFIED., .F., .T. ) 
 B_SPLINE_CURVE_WITH_KNOTS ( ( 3, 2, 2, 2, 3 ),
 ( 0.3520833333333333592, 0.3527777777777778012, 0.3541666666666666852, 0.3555555555555555691, 0.3562500000000000111 ),
 .UNSPECIFIED. ) 
 CURVE ( )  GEOMETRIC_REPRESENTATION_ITEM ( )  RATIONAL_B_SPLINE_CURVE ( ( 0.9330127018922194093, 0.9330127018922220739, 1.000000000000000000, 0.8660254037844387076, 1.000000000000000000, 0.8660254037844387076, 1.000000000000000000, 0.9330127018922194093, 0.9330127018922194093 ) ) 
 REPRESENTATION_ITEM ( '' )  );
#14613=VECTOR ( 'NONE', #32086, 1000.000000000000000 ) ;
#14615=( BOUNDED_CURVE ( )  B_SPLINE_CURVE ( 2, ( #35165, #41770, #6861, #12415, #9224, #38987, #19006, #19423, #31973 ),
 .UNSPECIFIED., .F., .T. ) 
 B_SPLINE_CURVE_WITH_KNOTS ( ( 3, 2, 2, 2, 3 ),
 ( 0.4395833333333333259, 0.4402777777777777679, 0.4416666666666666519, 0.4430555555555555358, 0.4437499999999999778 ),
 .UNSPECIFIED. ) 
 CURVE ( )  GEOMETRIC_REPRESENTATION_ITEM ( )  RATIONAL_B_SPLINE_CURVE ( ( 0.9330127018922194093, 0.9330127018922194093, 1.000000000000000000, 0.8660254037844387076, 1.000000000000000000, 0.8660254037844387076, 1.000000000000000000, 0.9330127018922194093, 0.9330127018922194093 ) ) 
 REPRESENTATION_ITEM ( '' )  );
#14619=CARTESIAN_POINT ( 'NONE',  ( 0.9378221735089300459, 21.00000000000001066, -33.25563900116002714 ) ) ;
#14620=CARTESIAN_POINT ( 'NONE',  ( 3.310556943749999981, 15.58864905735836714, -70.34743913623280775 ) ) ;
#14622=ORIENTED_EDGE ( 'NONE', *, *, #11036, .T. ) ;
#14624=CARTESIAN_POINT ( 'NONE',  ( 3.500000000000001332, 19.52072594216371826, -112.0713974700441184 ) ) ;
#14627=EDGE_CURVE ( 'NONE', #25556, #23073, #32240, .T. ) ;
#14628=ORIENTED_EDGE ( 'NONE', *, *, #35545, .F. ) ;
#14631=CARTESIAN_POINT ( 'NONE',  ( 3.310556943750001313, 19.41135094264167549, -132.1807724695661364 ) ) ;
#14632=CARTESIAN_POINT ( 'NONE',  ( -3.500000000000002220, 15.47927405783633503, -115.8776474690881884 ) ) ;
#14633=EDGE_CURVE ( 'NONE', #632, #34688, #33016, .T. ) ;
#14634=VECTOR ( 'NONE', #13512, 1000.000000000000000 ) ;
#14635=CARTESIAN_POINT ( 'NONE',  ( 3.310556943749999981, 15.58864905735836182, -45.43493913623279212 ) ) ;
#14636=CARTESIAN_POINT ( 'NONE',  ( 3.310556943749999981, 15.58864905735836182, -34.43493913623279923 ) ) ;
#14637=CARTESIAN_POINT ( 'NONE',  ( 3.310556943749999981, 15.58864905735836892, -94.43493913623279923 ) ) ;
#14638=CARTESIAN_POINT ( 'NONE',  ( -3.500000000000000888, 19.52072594216370405, -24.73806413671077209 ) ) ;
#14641=PRODUCT_DEFINITION_FORMATION_WITH_SPECIFIED_SOURCE ( 'ANY', '', #2424, .NOT_KNOWN. ) ;
#14642=CARTESIAN_POINT ( 'NONE',  ( -3.310556943750000425, 19.41135094264167549, -138.9349391362327708 ) ) ;
#14645=CARTESIAN_POINT ( 'NONE',  ( -3.500000000000002220, 15.47927405783632970, -96.87764746908817415 ) ) ;
#14648=CARTESIAN_POINT ( 'NONE',  ( 1.749999999999998224, 14.46891108675448123, -88.32139747004409003 ) ) ;
#14649=CARTESIAN_POINT ( 'NONE',  ( 1.655278471875001101, 20.36702641396248836, -68.18493913623279923 ) ) ;
#14653=DIRECTION ( 'NONE',  ( 0.000000000000000000, 1.000000000000000000, 0.000000000000000000 ) ) ;
#14654=CARTESIAN_POINT ( 'NONE',  ( 3.500000000000000000, 15.47927405783632082, -50.54431413575484555 ) ) ;
#14655=CARTESIAN_POINT ( 'NONE',  ( 3.310556943750001313, 17.50000000000002132, -117.2641058028994792 ) ) ;
#14656=CARTESIAN_POINT ( 'NONE',  ( -3.500000000000001332, 17.50000000000001776, -79.65473080337743284 ) ) ;
#14658=EDGE_LOOP ( 'NONE', ( #33180, #26703, #32628, #27433, #6197, #23233 ) ) ;
#14659=CARTESIAN_POINT ( 'NONE',  ( 1.750000000000001110, 20.53108891324555785, -112.9880641367107614 ) ) ;
#14661=LINE ( 'NONE', #18254, #39675 ) ;
#14662=FACE_OUTER_BOUND ( 'NONE', #14927, .T. ) ;
#14665=CARTESIAN_POINT ( 'NONE',  ( 3.310556943750001313, 17.50000000000001421, -73.26410580289947916 ) ) ;
#14669=CARTESIAN_POINT ( 'NONE',  ( -3.310556943750002201, 15.58864905735836182, -25.68077246956613990 ) ) ;
#14670=CARTESIAN_POINT ( 'NONE',  ( -3.310556943750001313, 17.50000000000001776, -82.76410580289947916 ) ) ;
#14672=ORIENTED_EDGE ( 'NONE', *, *, #41716, .F. ) ;
#14673=ORIENTED_EDGE ( 'NONE', *, *, #37893, .F. ) ;
#14674=VECTOR ( 'NONE', #25763, 1000.000000000000000 ) ;
#14677=ORIENTED_EDGE ( 'NONE', *, *, #17066, .F. ) ;
#14678=CARTESIAN_POINT ( 'NONE',  ( -3.500000000000001332, 17.50000000000002132, -126.6547308033774186 ) ) ;
#14679=CARTESIAN_POINT ( 'NONE',  ( -1.655278471874999990, 20.36702641396248836, -50.01827246956614204 ) ) ;
#14680=CARTESIAN_POINT ( 'NONE',  ( 1.655278471874998436, 14.63297358603754894, -116.5182724695661278 ) ) ;
#14682=( BOUNDED_CURVE ( )  B_SPLINE_CURVE ( 2, ( #41016, #8060, #14861, #17641, #28243, #8676, #21034, #34626, #14448 ),
 .UNSPECIFIED., .F., .T. ) 
 B_SPLINE_CURVE_WITH_KNOTS ( ( 3, 2, 2, 2, 3 ),
 ( 0.6812500000000000222, 0.6819444444444444642, 0.6833333333333333481, 0.6847222222222222321, 0.6854166666666666741 ),
 .UNSPECIFIED. ) 
 CURVE ( )  GEOMETRIC_REPRESENTATION_ITEM ( )  RATIONAL_B_SPLINE_CURVE ( ( 0.9330127018922194093, 0.9330127018922194093, 1.000000000000000000, 0.8660254037844387076, 1.000000000000000000, 0.8660254037844387076, 1.000000000000000000, 0.9330127018922194093, 0.9330127018922194093 ) ) 
 REPRESENTATION_ITEM ( '' )  );
#14683=EDGE_CURVE ( 'NONE', #24198, #36839, #60, .T. ) ;
#14684=CARTESIAN_POINT ( 'NONE',  ( -3.500000000000000888, 19.52072594216371826, -121.7380641367107614 ) ) ;
#14686=CARTESIAN_POINT ( 'NONE',  ( 1.655278471875001101, 20.36702641396248481, -33.09743913623280775 ) ) ;
#14687=CARTESIAN_POINT ( 'NONE',  ( -3.310556943750001313, 17.50000000000001421, -67.85160580289947063 ) ) ;
#14688=CARTESIAN_POINT ( 'NONE',  ( -7.424026671074350129E-16, 13.45854811567263987, -114.7109808024215027 ) ) ;
#14690=CARTESIAN_POINT ( 'NONE',  ( 3.310556943750001313, 19.41135094264166483, -95.18077246956613635 ) ) ;
#14692=CARTESIAN_POINT ( 'NONE',  ( -1.750000000000002220, 14.46891108675447413, -25.79431413575483845 ) ) ;
#14693=CARTESIAN_POINT ( 'NONE',  ( 0.9378221735089281585, 14.00000000000002309, -124.6663226036829855 ) ) ;
#14695=CARTESIAN_POINT ( 'NONE',  ( 3.500000000000001332, 17.50000000000001421, -62.46098080242150274 ) ) ;
#14697=CARTESIAN_POINT ( 'NONE',  ( 1.655278471874998436, 14.63297358603753828, -32.43077246956614346 ) ) ;
#14698=CARTESIAN_POINT ( 'NONE',  ( -7.022189441860112050E-16, 13.67729811471672363, -90.60160580289947063 ) ) ;
#14699=CARTESIAN_POINT ( 'NONE',  ( 1.749999999999998224, 14.46891108675447768, -54.32139747004409713 ) ) ;
#14700=AXIS2_PLACEMENT_3D ( 'NONE', #6514, #3317, #10543 ) ;
#14701=CARTESIAN_POINT ( 'NONE',  ( -3.310556943750000425, 19.41135094264166838, -104.9349391362327992 ) ) ;
#14702=CARTESIAN_POINT ( 'NONE',  ( -7.022189441860112050E-16, 13.67729811471671653, -38.60160580289946353 ) ) ;
#14710=CARTESIAN_POINT ( 'NONE',  ( -1.655278471875002211, 14.63297358603754716, -89.59743913623280775 ) ) ;
#14712=EDGE_CURVE ( 'NONE', #34104, #5189, #6655, .T. ) ;
#14714=ORIENTED_EDGE ( 'NONE', *, *, #15459, .T. ) ;
#14721=ORIENTED_EDGE ( 'NONE', *, *, #14999, .T. ) ;
#14722=CARTESIAN_POINT ( 'NONE',  ( 3.500000000000000000, 15.47927405783632793, -82.23806413671076143 ) ) ;
#14724=EDGE_CURVE ( 'NONE', #39830, #13507, #12830, .T. ) ;
#14729=EDGE_LOOP ( 'NONE', ( #28730, #15171, #7920, #16396 ) ) ;
#14731=CARTESIAN_POINT ( 'NONE',  ( 3.500000000000001332, 19.52072594216371826, -140.0713974700441042 ) ) ;
#14732=CARTESIAN_POINT ( 'NONE',  ( 1.655278471874998436, 14.63297358603755072, -134.4307724695661364 ) ) ;
#14733=CARTESIAN_POINT ( 'NONE',  ( 1.750000000000001110, 20.53108891324555429, -78.29431413575484555 ) ) ;
#14735=CARTESIAN_POINT ( 'NONE',  ( 3.310556943750001313, 17.50000000000002487, -132.3516058028994564 ) ) ;
#14736=CARTESIAN_POINT ( 'NONE',  ( -1.655278471875002211, 14.63297358603754184, -53.68493913623280633 ) ) ;
#14739=CARTESIAN_POINT ( 'NONE',  ( -1.750000000000002220, 14.46891108675449011, -137.4880641367107614 ) ) ;
#14740=( BOUNDED_CURVE ( )  B_SPLINE_CURVE ( 2, ( #31054, #11898, #30849, #27650, #40620, #18082, #8500, #5103, #11479 ),
 .UNSPECIFIED., .F., .F. ) 
 B_SPLINE_CURVE_WITH_KNOTS ( ( 3, 2, 2, 2, 3 ),
 ( 0.1520833333333333481, 0.1527777777777777901, 0.1541666666666666741, 0.1555555555555555580, 0.1562500000000000000 ),
 .UNSPECIFIED. ) 
 CURVE ( )  GEOMETRIC_REPRESENTATION_ITEM ( )  RATIONAL_B_SPLINE_CURVE ( ( 0.9330127018922194093, 0.9330127018922207416, 1.000000000000000000, 0.8660254037844387076, 1.000000000000000000, 0.8660254037844387076, 1.000000000000000000, 0.9330127018922194093, 0.9330127018922194093 ) ) 
 REPRESENTATION_ITEM ( '' )  );
#14743=CARTESIAN_POINT ( 'NONE',  ( -3.500000000000002220, 15.47927405783633503, -130.8776474690881741 ) ) ;
#14744=CARTESIAN_POINT ( 'NONE',  ( 1.655278471875001101, 20.36702641396249547, -110.0974391362328078 ) ) ;
#14748=CARTESIAN_POINT ( 'NONE',  ( -3.500000000000000888, 19.52072594216371115, -79.04431413575483134 ) ) ;
#14750=CARTESIAN_POINT ( 'NONE',  ( 0.9378221735089300459, 21.00000000000001421, -51.25563900116002714 ) ) ;
#14751=CARTESIAN_POINT ( 'NONE',  ( -3.310556943750001313, 17.50000000000001066, -46.76410580289947205 ) ) ;
#14752=CARTESIAN_POINT ( 'NONE',  ( -1.655278471874999990, 20.36702641396249547, -109.0182724695661420 ) ) ;
#14754=CARTESIAN_POINT ( 'NONE',  ( -0.9378221735089291577, 21.00000000000001066, -42.86007260463891555 ) ) ;
#14755=CARTESIAN_POINT ( 'NONE',  ( -3.500000000000002220, 15.47927405783632970, -88.87764746908817415 ) ) ;
#14757=CARTESIAN_POINT ( 'NONE',  ( -1.655278471875002211, 14.63297358603755072, -121.6849391362327992 ) ) ;
#14760=CARTESIAN_POINT ( 'NONE',  ( 0.9378221735089281585, 14.00000000000000888, -27.66632260368298901 ) ) ;
#14761=CARTESIAN_POINT ( 'NONE',  ( -1.394453263437886604E-15, 14.00000000000001421, -71.40473080337743284 ) ) ;
#14762=CARTESIAN_POINT ( 'NONE',  ( 1.655278471874998436, 14.63297358603754184, -60.51827246956613493 ) ) ;
#14763=ORIENTED_EDGE ( 'NONE', *, *, #31836, .F. ) ;
#14764=CARTESIAN_POINT ( 'NONE',  ( 2.340729813953370519E-16, 21.32270188528331190, -81.10160580289945642 ) ) ;
#14767=CARTESIAN_POINT ( 'NONE',  ( 3.500000000000001332, 19.52072594216371115, -99.07139747004409003 ) ) ;
#14769=CARTESIAN_POINT ( 'NONE',  ( -3.310556943750000425, 19.41135094264166128, -39.84743913623281486 ) ) ;
#14775=CARTESIAN_POINT ( 'NONE',  ( 1.655278471875001101, 20.36702641396248481, -46.09743913623280775 ) ) ;
#14777=EDGE_LOOP ( 'NONE', ( #37120, #26741, #22913, #33766 ) ) ;
#14778=CARTESIAN_POINT ( 'NONE',  ( 2.474675557024783212E-16, 21.54145188432739033, -25.21098080242151696 ) ) ;
#14780=CARTESIAN_POINT ( 'NONE',  ( 0.9378221735089300459, 21.00000000000001421, -62.94938900211595723 ) ) ;
#14781=VERTEX_POINT ( 'NONE', #33446 ) ;
#14782=CARTESIAN_POINT ( 'NONE',  ( 1.750000000000001110, 20.53108891324555785, -112.2943141357548456 ) ) ;
#14783=CARTESIAN_POINT ( 'NONE',  ( 3.500000000000001776, 19.52072594216370405, -37.37764746908816704 ) ) ;
#14785=CARTESIAN_POINT ( 'NONE',  ( 3.500000000000001332, 19.52072594216371826, -125.3776474690881599 ) ) ;
#14787=CARTESIAN_POINT ( 'NONE',  ( 3.310556943749999981, 15.58864905735836004, -24.43493913623280633 ) ) ;
#14789=CARTESIAN_POINT ( 'NONE',  ( -3.310556943750000425, 19.41135094264166838, -128.8474391362327935 ) ) ;
#14792=CARTESIAN_POINT ( 'NONE',  ( 3.500000000000001332, 19.52072594216370405, -29.07139747004410069 ) ) ;
#14793=CARTESIAN_POINT ( 'NONE',  ( -3.310556943750002645, 15.58864905735837780, -122.7682724695661278 ) ) ;
#14795=CARTESIAN_POINT ( 'NONE',  ( -7.424026671074350129E-16, 13.45854811567263276, -40.40473080337743994 ) ) ;
#14796=CARTESIAN_POINT ( 'NONE',  ( -0.9378221735089310451, 14.00000000000001066, -49.44938900211594301 ) ) ;
#14798=EDGE_CURVE ( 'NONE', #24198, #6800, #15096, .T. ) ;
#14799=CARTESIAN_POINT ( 'NONE',  ( 3.500000000000001776, 19.52072594216370760, -70.07139747004410424 ) ) ;
#14801=CARTESIAN_POINT ( 'NONE',  ( -3.310556943750000425, 19.41135094264166483, -55.93493913623279923 ) ) ;
#14803=CARTESIAN_POINT ( 'NONE',  ( 0.9378221735089324884, 14.00000000000002665, -137.6663226036829997 ) ) ;
#14804=CARTESIAN_POINT ( 'NONE',  ( -1.655278471875002211, 14.63297358603754539, -73.68493913623279923 ) ) ;
#14806=CARTESIAN_POINT ( 'NONE',  ( 3.310556943749999981, 15.58864905735837070, -103.3474391362328220 ) ) ;
#14807=CARTESIAN_POINT ( 'NONE',  ( -1.655278471875002211, 14.63297358603754539, -75.59743913623280775 ) ) ;
#14808=ORIENTED_EDGE ( 'NONE', *, *, #5668, .F. ) ;
#14809=CARTESIAN_POINT ( 'NONE',  ( -3.310556943750002201, 15.58864905735837425, -98.76827246956612782 ) ) ;
#14811=CARTESIAN_POINT ( 'NONE',  ( -0.9378221735089310451, 14.00000000000001066, -32.75563900116002714 ) ) ;
#14812=CARTESIAN_POINT ( 'NONE',  ( 3.500000000000001332, 19.52072594216370405, -26.37764746908817415 ) ) ;
#14815=CARTESIAN_POINT ( 'NONE',  ( 2.340729813953370519E-16, 21.32270188528331190, -57.01410580289947916 ) ) ;
#14817=CARTESIAN_POINT ( 'NONE',  ( 1.655278471875001101, 20.36702641396249547, -110.0974391362328078 ) ) ;
#14818=VERTEX_POINT ( 'NONE', #14521 ) ;
#14819=VERTEX_POINT ( 'NONE', #4091 ) ;
#14821=ORIENTED_EDGE ( 'NONE', *, *, #7811, .F. ) ;
#14822=DIRECTION ( 'NONE',  ( -0.000000000000000000, 1.259100132267607459E-16, -1.000000000000000000 ) ) ;
#14823=CARTESIAN_POINT ( 'NONE',  ( 2.340729813953370519E-16, 21.32270188528330834, -61.01410580289946495 ) ) ;
#14826=CARTESIAN_POINT ( 'NONE',  ( 4.648177544792955347E-16, 21.00000000000001776, -87.21098080242151696 ) ) ;
#14830=ORIENTED_EDGE ( 'NONE', *, *, #6689, .T. ) ;
#14831=CARTESIAN_POINT ( 'NONE',  ( -3.500000000000002220, 15.47927405783633503, -142.8776474690881741 ) ) ;
#14832=CARTESIAN_POINT ( 'NONE',  ( 2.340729813953370519E-16, 21.32270188528332255, -131.0141058028994507 ) ) ;
#14833=CARTESIAN_POINT ( 'NONE',  ( 1.750000000000001110, 20.53108891324555785, -119.2943141357548313 ) ) ;
#14834=VECTOR ( 'NONE', #1568, 1000.000000000000000 ) ;
#14835=CARTESIAN_POINT ( 'NONE',  ( 3.310556943750001313, 17.50000000000001066, -39.35160580289946353 ) ) ;
#14836=CARTESIAN_POINT ( 'NONE',  ( 3.310556943750001313, 19.41135094264165772, -31.26827246956613493 ) ) ;
#14837=CARTESIAN_POINT ( 'NONE',  ( 1.655278471874998436, 14.63297358603754539, -92.51827246956611361 ) ) ;
#14838=CARTESIAN_POINT ( 'NONE',  ( -3.500000000000001332, 17.50000000000001066, -25.65473080337743284 ) ) ;
#14839=VERTEX_POINT ( 'NONE', #7928 ) ;
#14841=CARTESIAN_POINT ( 'NONE',  ( -3.310556943750000425, 19.41135094264167549, -139.9349391362327992 ) ) ;
#14842=CARTESIAN_POINT ( 'NONE',  ( 3.500000000000001332, 17.50000000000001776, -94.46098080242151696 ) ) ;
#14844=CARTESIAN_POINT ( 'NONE',  ( 3.310556943749999981, 15.58864905735836537, -60.34743913623280065 ) ) ;
#14846=CARTESIAN_POINT ( 'NONE',  ( 3.500000000000000000, 15.47927405783632615, -84.23806413671076143 ) ) ;
#14847=CARTESIAN_POINT ( 'NONE',  ( -3.310556943750002201, 15.58864905735837070, -68.76827246956612782 ) ) ;
#14851=CARTESIAN_POINT ( 'NONE',  ( -1.749999999999999778, 20.53108891324555074, -51.12764746908816704 ) ) ;
#14852=VECTOR ( 'NONE', #34842, 1000.000000000000000 ) ;
#14853=CARTESIAN_POINT ( 'NONE',  ( 3.310556943750001313, 19.41135094264166838, -121.1807724695661506 ) ) ;
#14855=( BOUNDED_CURVE ( )  B_SPLINE_CURVE ( 2, ( #843, #13816, #7007, #29758, #17440, #26798, #10200, #39537, #20409 ),
 .UNSPECIFIED., .F., .T. ) 
 B_SPLINE_CURVE_WITH_KNOTS ( ( 3, 2, 2, 2, 3 ),
 ( 0.1895833333333333259, 0.1902777777777777679, 0.1916666666666666796, 0.1930555555555555636, 0.1937500000000000056 ),
 .UNSPECIFIED. ) 
 CURVE ( )  GEOMETRIC_REPRESENTATION_ITEM ( )  RATIONAL_B_SPLINE_CURVE ( ( 0.9330127018922194093, 0.9330127018922194093, 1.000000000000000000, 0.8660254037844387076, 1.000000000000000000, 0.8660254037844387076, 1.000000000000000000, 0.9330127018922194093, 0.9330127018922194093 ) ) 
 REPRESENTATION_ITEM ( '' )  );
#14858=CARTESIAN_POINT ( 'NONE',  ( 3.500000000000001332, 17.50000000000002132, -115.1547308033774328 ) ) ;
#14860=CARTESIAN_POINT ( 'NONE',  ( -4.648177544792955347E-16, 21.00000000000002487, -143.2109808024214885 ) ) ;
#14861=CARTESIAN_POINT ( 'NONE',  ( 1.749999999999998224, 14.46891108675447768, -61.32139747004409713 ) ) ;
#14862=EDGE_CURVE ( 'NONE', #34834, #11928, #30039, .T. ) ;
#14865=CARTESIAN_POINT ( 'NONE',  ( 2.340729813953370519E-16, 21.32270188528331190, -72.01410580289947916 ) ) ;
#14867=CARTESIAN_POINT ( 'NONE',  ( 3.500000000000001332, 17.50000000000001421, -72.46098080242151696 ) ) ;
#14868=VERTEX_POINT ( 'NONE', #4309 ) ;
#14869=CARTESIAN_POINT ( 'NONE',  ( -1.749999999999999778, 20.53108891324556140, -133.1276474690881741 ) ) ;
#14871=CARTESIAN_POINT ( 'NONE',  ( -3.310556943750002645, 15.58864905735837247, -86.68077246956615056 ) ) ;
#14872=ORIENTED_EDGE ( 'NONE', *, *, #38909, .F. ) ;
#14873=VERTEX_POINT ( 'NONE', #27493 ) ;
#14876=VECTOR ( 'NONE', #33269, 1000.000000000000000 ) ;
#14877=CARTESIAN_POINT ( 'NONE',  ( -7.460324959392693302E-14, 21.00000000000001776, -100.9047308033774186 ) ) ;
#14878=CARTESIAN_POINT ( 'NONE',  ( -3.310556943750000425, 19.41135094264166128, -50.93493913623280633 ) ) ;
#14879=CARTESIAN_POINT ( 'NONE',  ( -7.022189441860112050E-16, 13.67729811471672718, -111.6016058028994706 ) ) ;
#14882=CARTESIAN_POINT ( 'NONE',  ( -3.310556943750000425, 19.41135094264165772, -34.84743913623281486 ) ) ;
#14883=CARTESIAN_POINT ( 'NONE',  ( 1.655278471874998436, 14.63297358603754184, -63.51827246956613493 ) ) ;
#14884=CARTESIAN_POINT ( 'NONE',  ( -3.500000000000002220, 15.47927405783633503, -113.8776474690881741 ) ) ;
#14886=CARTESIAN_POINT ( 'NONE',  ( 1.655278471875001101, 20.36702641396249192, -95.09743913623280775 ) ) ;
#14887=CARTESIAN_POINT ( 'NONE',  ( -1.750000000000002220, 14.46891108675447768, -47.48806413671076143 ) ) ;
#14890=CARTESIAN_POINT ( 'NONE',  ( 3.500000000000000000, 15.47927405783632260, -64.54431413575483134 ) ) ;
#14892=CARTESIAN_POINT ( 'NONE',  ( -1.655278471875002211, 14.63297358603754006, -34.59743913623280775 ) ) ;
#14893=CARTESIAN_POINT ( 'NONE',  ( -7.424026671074350129E-16, 13.45854811567263276, -52.40473080337743284 ) ) ;
#14894=CARTESIAN_POINT ( 'NONE',  ( 0.9378221735089300459, 21.00000000000001776, -92.25563900116003424 ) ) ;
#14895=CARTESIAN_POINT ( 'NONE',  ( -3.310556943750001313, 17.50000000000002132, -109.8516058028994564 ) ) ;
#14896=CARTESIAN_POINT ( 'NONE',  ( -3.310556943750001313, 17.50000000000001066, -37.85160580289946353 ) ) ;
#14902=CARTESIAN_POINT ( 'NONE',  ( 4.648177544792955347E-16, 21.00000000000001421, -48.21098080242150274 ) ) ;
#14904=CARTESIAN_POINT ( 'NONE',  ( 3.310556943750001313, 17.50000000000001776, -85.26410580289947916 ) ) ;
#14907=VECTOR ( 'NONE', #23176, 1000.000000000000000 ) ;
#14910=CARTESIAN_POINT ( 'NONE',  ( 1.750000000000001110, 20.53108891324556140, -132.9880641367107614 ) ) ;
#14913=CARTESIAN_POINT ( 'NONE',  ( -3.500000000000001332, 17.50000000000001066, -30.96098080242150274 ) ) ;
#14917=ADVANCED_FACE ( 'NONE', ( #20894 ), #40248, .T. ) ;
#14918=FACE_OUTER_BOUND ( 'NONE', #16405, .T. ) ;
#14919=EDGE_LOOP ( 'NONE', ( #16699, #1732, #32537, #39987 ) ) ;
#14923=CARTESIAN_POINT ( 'NONE',  ( -1.394453263437886604E-15, 14.00000000000001776, -102.7109808024215027 ) ) ;
#14926=( BOUNDED_CURVE ( )  B_SPLINE_CURVE ( 2, ( #14154, #40314, #37334, #30739, #4581, #40523, #4789, #1393, #17560 ),
 .UNSPECIFIED., .F., .T. ) 
 B_SPLINE_CURVE_WITH_KNOTS ( ( 3, 2, 2, 2, 3 ),
 ( 0.1729166666666666630, 0.1736111111111111049, 0.1749999999999999889, 0.1763888888888889006, 0.1770833333333333426 ),
 .UNSPECIFIED. ) 
 CURVE ( )  GEOMETRIC_REPRESENTATION_ITEM ( )  RATIONAL_B_SPLINE_CURVE ( ( 0.9330127018922194093, 0.9330127018922194093, 1.000000000000000000, 0.8660254037844387076, 1.000000000000000000, 0.8660254037844387076, 1.000000000000000000, 0.9330127018922194093, 0.9330127018922194093 ) ) 
 REPRESENTATION_ITEM ( '' )  );
#14927=EDGE_LOOP ( 'NONE', ( #34222, #13618, #10217, #39590 ) ) ;
#14928=CARTESIAN_POINT ( 'NONE',  ( -1.394453263437886604E-15, 14.00000000000001421, -61.71098080242150985 ) ) ;
#14930=CARTESIAN_POINT ( 'NONE',  ( -3.310556943750002645, 15.58864905735837958, -136.6807724695661364 ) ) ;
#14931=VERTEX_POINT ( 'NONE', #17291 ) ;
#14932=CARTESIAN_POINT ( 'NONE',  ( 0.9378221735089281585, 14.00000000000001243, -54.66632260368298546 ) ) ;
#14933=CARTESIAN_POINT ( 'NONE',  ( -1.655278471875002211, 14.63297358603755249, -124.6849391362327992 ) ) ;
#14934=CARTESIAN_POINT ( 'NONE',  ( 3.310556943749999981, 15.58864905735836537, -54.43493913623280633 ) ) ;
#14937=CARTESIAN_POINT ( 'NONE',  ( 3.500000000000001332, 17.50000000000002487, -138.1547308033774186 ) ) ;
#14938=( LENGTH_UNIT ( ) NAMED_UNIT ( * ) SI_UNIT ( .MILLI., .METRE. ) );
#14940=CARTESIAN_POINT ( 'NONE',  ( -3.310556943750000425, 19.41135094264166483, -83.93493913623278502 ) ) ;
#14941=CARTESIAN_POINT ( 'NONE',  ( 3.500000000000001776, 19.52072594216372181, -130.3776474690881741 ) ) ;
#14942=CARTESIAN_POINT ( 'NONE',  ( 3.310556943749999981, 15.58864905735837247, -110.3474391362327935 ) ) ;
#14947=CARTESIAN_POINT ( 'NONE',  ( 2.474675557024783212E-16, 21.54145188432739744, -79.21098080242150274 ) ) ;
#14949=CARTESIAN_POINT ( 'NONE',  ( -3.310556943750001313, 17.50000000000001421, -49.76410580289947205 ) ) ;
#14950=AXIS2_PLACEMENT_3D ( 'NONE', #16789, #23383, #25944 ) ;
#14952=CARTESIAN_POINT ( 'NONE',  ( 1.655278471875001101, 20.36702641396249547, -109.1849391362327992 ) ) ;
#14954=CARTESIAN_POINT ( 'NONE',  ( -1.394453263437886604E-15, 14.00000000000001421, -79.71098080242148853 ) ) ;
#14955=DIRECTION ( 'NONE',  ( -0.000000000000000000, 1.259100132267607459E-16, -1.000000000000000000 ) ) ;
#14956=CARTESIAN_POINT ( 'NONE',  ( -3.310556943750000425, 19.41135094264166838, -124.9349391362327992 ) ) ;
#14959=CARTESIAN_POINT ( 'NONE',  ( 0.9378221735089281585, 14.00000000000001776, -83.36007260463891555 ) ) ;
#14960=CARTESIAN_POINT ( 'NONE',  ( -3.500000000000000000, 19.52072594216370760, -57.73806413671076143 ) ) ;
#14961=CARTESIAN_POINT ( 'NONE',  ( 3.310556943750001313, 17.50000000000001421, -58.35160580289947063 ) ) ;
#14962=VERTEX_POINT ( 'NONE', #7503 ) ;
#14963=CARTESIAN_POINT ( 'NONE',  ( -7.022189441860112050E-16, 13.67729811471672186, -73.60160580289947063 ) ) ;
#14964=CARTESIAN_POINT ( 'NONE',  ( 3.500000000000000000, 15.47927405783632082, -40.54431413575485266 ) ) ;
#14967=FACE_OUTER_BOUND ( 'NONE', #33010, .T. ) ;
#14970=CARTESIAN_POINT ( 'NONE',  ( -3.310556943750000425, 19.41135094264166128, -37.84743913623281486 ) ) ;
#14971=CARTESIAN_POINT ( 'NONE',  ( -3.500000000000000000, 19.52072594216371115, -93.73806413671076143 ) ) ;
#14972=VERTEX_POINT ( 'NONE', #23891 ) ;
#14973=VECTOR ( 'NONE', #16126, 1000.000000000000000 ) ;
#14974=EDGE_CURVE ( 'NONE', #3824, #19056, #26789, .T. ) ;
#14978=CARTESIAN_POINT ( 'NONE',  ( -1.655278471874999990, 20.36702641396248481, -44.93077246956614346 ) ) ;
#14982=( BOUNDED_CURVE ( )  B_SPLINE_CURVE ( 2, ( #6932, #20120, #10129, #339, #39465, #38845, #6307, #22466, #19907 ),
 .UNSPECIFIED., .F., .T. ) 
 B_SPLINE_CURVE_WITH_KNOTS ( ( 3, 2, 2, 2, 3 ),
 ( 0.7812500000000000000, 0.7819444444444444420, 0.7833333333333333259, 0.7847222222222222099, 0.7854166666666666519 ),
 .UNSPECIFIED. ) 
 CURVE ( )  GEOMETRIC_REPRESENTATION_ITEM ( )  RATIONAL_B_SPLINE_CURVE ( ( 0.9330127018922194093, 0.9330127018922194093, 1.000000000000000000, 0.8660254037844387076, 1.000000000000000000, 0.8660254037844387076, 1.000000000000000000, 0.9330127018922194093, 0.9330127018922194093 ) ) 
 REPRESENTATION_ITEM ( '' )  );
#14983=VECTOR ( 'NONE', #31088, 1000.000000000000000 ) ;
#14984=CARTESIAN_POINT ( 'NONE',  ( 3.500000000000000000, 15.47927405783631727, -23.54431413575484910 ) ) ;
#14986=CARTESIAN_POINT ( 'NONE',  ( 1.750000000000001110, 20.53108891324555429, -97.29431413575484555 ) ) ;
#14988=CARTESIAN_POINT ( 'NONE',  ( -3.500000000000001332, 17.50000000000001066, -38.96098080242150985 ) ) ;
#14989=DIRECTION ( 'NONE',  ( -0.000000000000000000, 1.259100132267607459E-16, -1.000000000000000000 ) ) ;
#14990=CARTESIAN_POINT ( 'NONE',  ( -1.394453263437886604E-15, 14.00000000000001776, -82.71098080242150274 ) ) ;
#14992=CARTESIAN_POINT ( 'NONE',  ( -3.310556943750001313, 17.50000000000001066, -25.85160580289947063 ) ) ;
#14994=CARTESIAN_POINT ( 'NONE',  ( 3.310556943750001313, 17.50000000000002487, -130.2641058028994507 ) ) ;
#14997=EDGE_CURVE ( 'NONE', #26809, #19989, #33615, .T. ) ;
#14998=CARTESIAN_POINT ( 'NONE',  ( 0.000000000000000000, 21.00000000000002487, -149.5231586289125687 ) ) ;
#14999=EDGE_CURVE ( 'NONE', #15387, #9764, #3170, .T. ) ;
#15000=CARTESIAN_POINT ( 'NONE',  ( 2.340729813953370519E-16, 21.32270188528331900, -121.1016058028994706 ) ) ;
#15002=CARTESIAN_POINT ( 'NONE',  ( 3.500000000000000000, 15.47927405783632082, -40.23806413671077564 ) ) ;
#15003=CARTESIAN_POINT ( 'NONE',  ( 3.500000000000000000, 15.47927405783632082, -46.23806413671076143 ) ) ;
#15005=CARTESIAN_POINT ( 'NONE',  ( 3.310556943749999981, 15.58864905735837780, -141.4349391362327708 ) ) ;
#15007=CARTESIAN_POINT ( 'NONE',  ( -1.655278471874999990, 20.36702641396248836, -47.01827246956613493 ) ) ;
#15009=CARTESIAN_POINT ( 'NONE',  ( 4.286263797015737581E-16, 14.00000000000002487, -149.5231586289125687 ) ) ;
#15010=CARTESIAN_POINT ( 'NONE',  ( -7.022189441860112050E-16, 13.67729811471672186, -76.60160580289945642 ) ) ;
#15012=CARTESIAN_POINT ( 'NONE',  ( 3.310556943749999981, 15.58864905735837070, -104.3474391362328220 ) ) ;
#15013=CARTESIAN_POINT ( 'NONE',  ( -3.310556943750002645, 15.58864905735837070, -69.68077246956613635 ) ) ;
#15014=VERTEX_POINT ( 'NONE', #34905 ) ;
#15016=CARTESIAN_POINT ( 'NONE',  ( -3.310556943750001313, 17.50000000000001776, -88.85160580289947063 ) ) ;
#15021=CARTESIAN_POINT ( 'NONE',  ( -3.310556943750001313, 17.50000000000001421, -55.76410580289947916 ) ) ;
#15022=CARTESIAN_POINT ( 'NONE',  ( -3.500000000000002220, 15.47927405783633503, -137.5713974700441042 ) ) ;
#15023=CARTESIAN_POINT ( 'NONE',  ( 3.310556943749999981, 15.58864905735837247, -112.3474391362328078 ) ) ;
#15024=CARTESIAN_POINT ( 'NONE',  ( 4.648177544792955347E-16, 21.00000000000001776, -84.21098080242150274 ) ) ;
#15025=ORIENTED_EDGE ( 'NONE', *, *, #8709, .F. ) ;
#15030=CARTESIAN_POINT ( 'NONE',  ( -3.310556943750001313, 17.50000000000001421, -63.76410580289947205 ) ) ;
#15036=CARTESIAN_POINT ( 'NONE',  ( 4.286263797015737581E-16, 14.00000000000002487, -149.5231586289125687 ) ) ;
#15038=CARTESIAN_POINT ( 'NONE',  ( 0.000000000000000000, 21.00000000000002487, -149.5231586289125687 ) ) ;
#15042=CARTESIAN_POINT ( 'NONE',  ( 2.340729813953370519E-16, 21.32270188528331900, -129.0141058028994507 ) ) ;
#15045=CARTESIAN_POINT ( 'NONE',  ( -3.310556943750000425, 19.41135094264165772, -41.93493913623279212 ) ) ;
#15047=CARTESIAN_POINT ( 'NONE',  ( -3.310556943750002645, 15.58864905735837247, -94.76827246956611361 ) ) ;
#15048=CARTESIAN_POINT ( 'NONE',  ( -3.500000000000001332, 17.50000000000001066, -26.65473080337743639 ) ) ;
#15050=( BOUNDED_CURVE ( )  B_SPLINE_CURVE ( 2, ( #32045, #19494, #38436, #23100, #36068, #19912, #25680, #29059, #2914 ),
 .UNSPECIFIED., .F., .F. ) 
 B_SPLINE_CURVE_WITH_KNOTS ( ( 3, 2, 2, 2, 3 ),
 ( 0.6062499999999999556, 0.6069444444444443976, 0.6083333333333332815, 0.6097222222222222765, 0.6104166666666667185 ),
 .UNSPECIFIED. ) 
 CURVE ( )  GEOMETRIC_REPRESENTATION_ITEM ( )  RATIONAL_B_SPLINE_CURVE ( ( 0.9330127018922194093, 0.9330127018922194093, 1.000000000000000000, 0.8660254037844387076, 1.000000000000000000, 0.8660254037844387076, 1.000000000000000000, 0.9330127018922194093, 0.9330127018922194093 ) ) 
 REPRESENTATION_ITEM ( '' )  );
#15052=CARTESIAN_POINT ( 'NONE',  ( -3.310556943750000425, 19.41135094264167549, -136.9349391362327992 ) ) ;
#15055=CARTESIAN_POINT ( 'NONE',  ( 2.340729813953370519E-16, 21.32270188528330834, -58.01410580289949337 ) ) ;
#15057=CARTESIAN_POINT ( 'NONE',  ( -1.749999999999999778, 20.53108891324555429, -84.82139747004409003 ) ) ;
#15058=CARTESIAN_POINT ( 'NONE',  ( -1.655278471875002211, 14.63297358603754361, -66.68493913623279923 ) ) ;
#15063=CARTESIAN_POINT ( 'NONE',  ( 3.500000000000000000, 15.47927405783632082, -49.54431413575483845 ) ) ;
#15064=CARTESIAN_POINT ( 'NONE',  ( -1.655278471875002211, 14.63297358603755072, -118.5974391362328078 ) ) ;
#15065=DIRECTION ( 'NONE',  ( 0.000000000000000000, 1.000000000000000000, 0.000000000000000000 ) ) ;
#15068=CARTESIAN_POINT ( 'NONE',  ( 3.500000000000001332, 17.50000000000002132, -112.1547308033774328 ) ) ;
#15074=CARTESIAN_POINT ( 'NONE',  ( -7.022189441860112050E-16, 13.67729811471672186, -69.51410580289947916 ) ) ;
#15077=CARTESIAN_POINT ( 'NONE',  ( 1.750000000000001110, 20.53108891324555074, -72.29431413575483134 ) ) ;
#15078=ORIENTED_EDGE ( 'NONE', *, *, #33918, .T. ) ;
#15079=CARTESIAN_POINT ( 'NONE',  ( 3.310556943749999981, 15.58864905735836004, -24.34743913623281486 ) ) ;
#15081=CARTESIAN_POINT ( 'NONE',  ( 1.655278471875001101, 20.36702641396249192, -79.09743913623280775 ) ) ;
#15091=CARTESIAN_POINT ( 'NONE',  ( -1.749999999999999778, 20.53108891324555785, -126.8213974700440900 ) ) ;
#15092=CARTESIAN_POINT ( 'NONE',  ( -3.310556943750001313, 17.50000000000001421, -50.85160580289946353 ) ) ;
#15094=CARTESIAN_POINT ( 'NONE',  ( -3.310556943750002645, 15.58864905735837780, -110.7682724695661420 ) ) ;
#15095=VERTEX_POINT ( 'NONE', #14928 ) ;
#15096=( BOUNDED_CURVE ( )  B_SPLINE_CURVE ( 2, ( #1126, #33867, #17706, #7291, #30674, #14306, #37272, #33227, #27284 ),
 .UNSPECIFIED., .F., .T. ) 
 B_SPLINE_CURVE_WITH_KNOTS ( ( 3, 2, 2, 2, 3 ),
 ( 0.7437500000000000222, 0.7444444444444444642, 0.7458333333333333481, 0.7472222222222222321, 0.7479166666666666741 ),
 .UNSPECIFIED. ) 
 CURVE ( )  GEOMETRIC_REPRESENTATION_ITEM ( )  RATIONAL_B_SPLINE_CURVE ( ( 0.9330127018922194093, 0.9330127018922194093, 1.000000000000000000, 0.8660254037844387076, 1.000000000000000000, 0.8660254037844387076, 1.000000000000000000, 0.9330127018922194093, 0.9330127018922194093 ) ) 
 REPRESENTATION_ITEM ( '' )  );
#15097=CARTESIAN_POINT ( 'NONE',  ( 1.655278471875001101, 20.36702641396248481, -35.09743913623280775 ) ) ;
#15098=CARTESIAN_POINT ( 'NONE',  ( -1.655278471875002211, 14.63297358603754361, -60.68493913623279923 ) ) ;
#15099=CARTESIAN_POINT ( 'NONE',  ( -7.424026671074350129E-16, 13.45854811567263987, -110.7109808024215027 ) ) ;
#15101=CARTESIAN_POINT ( 'NONE',  ( 3.310556943750001313, 17.50000000000001776, -97.26410580289947916 ) ) ;
#15105=CARTESIAN_POINT ( 'NONE',  ( -7.424026671074350129E-16, 13.45854811567263454, -65.71098080242151696 ) ) ;
#15107=CARTESIAN_POINT ( 'NONE',  ( -7.022189441860112050E-16, 13.67729811471671475, -29.51410580289948982 ) ) ;
#15108=CARTESIAN_POINT ( 'NONE',  ( -1.750000000000002220, 14.46891108675447946, -56.48806413671076143 ) ) ;
#15111=CARTESIAN_POINT ( 'NONE',  ( 2.340729813953370519E-16, 21.32270188528331900, -107.1016058028994706 ) ) ;
#15112=CARTESIAN_POINT ( 'NONE',  ( -3.310556943750001313, 17.50000000000001066, -39.85160580289947063 ) ) ;
#15118=CARTESIAN_POINT ( 'NONE',  ( 0.000000000000000000, 17.50000000000002487, -149.5231586289125687 ) ) ;
#15120=CARTESIAN_POINT ( 'NONE',  ( -1.655278471874999990, 20.36702641396249192, -85.93077246956613635 ) ) ;
#15121=CARTESIAN_POINT ( 'NONE',  ( 1.750000000000001110, 20.53108891324555785, -116.9880641367107614 ) ) ;
#15123=CARTESIAN_POINT ( 'NONE',  ( -1.750000000000002220, 14.46891108675447413, -25.48806413671075788 ) ) ;
#15124=VERTEX_POINT ( 'NONE', #38303 ) ;
#15126=ORIENTED_EDGE ( 'NONE', *, *, #14633, .F. ) ;
#15133=VERTEX_POINT ( 'NONE', #34075 ) ;
#15139=CARTESIAN_POINT ( 'NONE',  ( 0.9378221735089300459, 21.00000000000001776, -90.94938900211595012 ) ) ;
#15140=LINE ( 'NONE', #8541, #3788 ) ;
#15141=CARTESIAN_POINT ( 'NONE',  ( 3.310556943750001313, 17.50000000000002487, -139.2641058028994792 ) ) ;
#15144=CARTESIAN_POINT ( 'NONE',  ( -1.394453263437886604E-15, 14.00000000000001421, -63.40473080337742573 ) ) ;
#15145=CARTESIAN_POINT ( 'NONE',  ( 1.655278471874998436, 14.63297358603755072, -123.5182724695661278 ) ) ;
#15146=CARTESIAN_POINT ( 'NONE',  ( -1.655278471875002211, 14.63297358603754361, -57.68493913623279212 ) ) ;
#15147=ORIENTED_EDGE ( 'NONE', *, *, #4080, .T. ) ;
#15150=CARTESIAN_POINT ( 'NONE',  ( -1.750000000000002220, 14.46891108675449011, -136.4880641367107614 ) ) ;
#15152=CARTESIAN_POINT ( 'NONE',  ( -1.655278471874999990, 20.36702641396249192, -75.01827246956612782 ) ) ;
#15153=CARTESIAN_POINT ( 'NONE',  ( -3.500000000000000888, 19.52072594216372181, -130.0443141357548313 ) ) ;
#15154=CARTESIAN_POINT ( 'NONE',  ( -3.310556943750000425, 19.41135094264166838, -111.8474391362328220 ) ) ;
#15158=CARTESIAN_POINT ( 'NONE',  ( 1.750000000000001110, 20.53108891324555429, -81.29431413575484555 ) ) ;
#15159=CARTESIAN_POINT ( 'NONE',  ( -0.9378221735089310451, 14.00000000000001599, -61.75563900116002714 ) ) ;
#15160=CARTESIAN_POINT ( 'NONE',  ( 3.310556943750001313, 19.41135094264166128, -50.18077246956615056 ) ) ;
#15161=CARTESIAN_POINT ( 'NONE',  ( -3.310556943750002645, 15.58864905735837425, -99.76827246956614204 ) ) ;
#15162=CARTESIAN_POINT ( 'NONE',  ( -3.500000000000000000, 19.52072594216371826, -130.0443141357548598 ) ) ;
#15165=CARTESIAN_POINT ( 'NONE',  ( -3.310556943750002201, 15.58864905735837780, -121.7682724695661278 ) ) ;
#15166=CARTESIAN_POINT ( 'NONE',  ( 4.648177544792955347E-16, 21.00000000000001776, -99.21098080242150274 ) ) ;
#15169=CARTESIAN_POINT ( 'NONE',  ( 0.9378221735089300459, 21.00000000000001421, -50.25563900116002714 ) ) ;
#15171=ORIENTED_EDGE ( 'NONE', *, *, #6921, .T. ) ;
#15173=CARTESIAN_POINT ( 'NONE',  ( 1.655278471874998436, 14.63297358603754361, -77.51827246956614204 ) ) ;
#15178=AXIS2_PLACEMENT_3D ( 'NONE', #9299, #26098, #19288 ) ;
#15180=CARTESIAN_POINT ( 'NONE',  ( -1.655278471874999990, 20.36702641396248481, -39.93077246956613635 ) ) ;
#15183=AXIS2_PLACEMENT_3D ( 'NONE', #14032, #29544, #26795 ) ;
#15187=CARTESIAN_POINT ( 'NONE',  ( -1.655278471875002211, 14.63297358603754184, -46.59743913623280775 ) ) ;
#15188=EDGE_CURVE ( 'NONE', #19669, #31096, #9169, .T. ) ;
#15189=ORIENTED_EDGE ( 'NONE', *, *, #8031, .T. ) ;
#15191=CARTESIAN_POINT ( 'NONE',  ( 1.749999999999998224, 14.46891108675447768, -56.32139747004409713 ) ) ;
#15192=CARTESIAN_POINT ( 'NONE',  ( 0.000000000000000000, 17.50000000000002487, -149.5231586289125687 ) ) ;
#15194=CARTESIAN_POINT ( 'NONE',  ( 1.750000000000001110, 20.53108891324555074, -62.98806413671076143 ) ) ;
#15196=FACE_OUTER_BOUND ( 'NONE', #33396, .T. ) ;
#15197=CARTESIAN_POINT ( 'NONE',  ( 1.750000000000001110, 20.53108891324554719, -40.29431413575485266 ) ) ;
#15198=CARTESIAN_POINT ( 'NONE',  ( -1.394453263437886604E-15, 14.00000000000001066, -35.71098080242150985 ) ) ;
#15199=CARTESIAN_POINT ( 'NONE',  ( -0.9378221735089291577, 21.00000000000001421, -64.86007260463891555 ) ) ;
#15201=CARTESIAN_POINT ( 'NONE',  ( 4.286263797015737581E-16, 14.00000000000002487, -149.5231586289125687 ) ) ;
#15203=CARTESIAN_POINT ( 'NONE',  ( 3.310556943750001313, 17.50000000000001066, -25.35160580289946708 ) ) ;
#15205=CARTESIAN_POINT ( 'NONE',  ( 3.310556943749999981, 15.58864905735837425, -128.3474391362328220 ) ) ;
#15209=CARTESIAN_POINT ( 'NONE',  ( -1.750000000000002220, 14.46891108675448123, -76.48806413671076143 ) ) ;
#15210=CARTESIAN_POINT ( 'NONE',  ( 3.310556943749999981, 15.58864905735837247, -121.4349391362327992 ) ) ;
#15212=LINE ( 'NONE', #11386, #41781 ) ;
#15213=CARTESIAN_POINT ( 'NONE',  ( 1.750000000000001110, 20.53108891324554719, -39.98806413671076854 ) ) ;
#15217=CARTESIAN_POINT ( 'NONE',  ( 1.655278471874998436, 14.63297358603755249, -139.5182724695661420 ) ) ;
#15219=CARTESIAN_POINT ( 'NONE',  ( 3.310556943749999981, 15.58864905735836182, -48.43493913623279923 ) ) ;
#15221=CARTESIAN_POINT ( 'NONE',  ( -1.749999999999999778, 20.53108891324555074, -73.12764746908817415 ) ) ;
#15222=CARTESIAN_POINT ( 'NONE',  ( -7.022189441860112050E-16, 13.67729811471672186, -72.60160580289947063 ) ) ;
#15224=CARTESIAN_POINT ( 'NONE',  ( 1.655278471874998436, 14.63297358603754716, -103.4307724695661364 ) ) ;
#15225=CARTESIAN_POINT ( 'NONE',  ( -3.310556943750001313, 17.50000000000001421, -70.76410580289947916 ) ) ;
#15226=ORIENTED_EDGE ( 'NONE', *, *, #21511, .T. ) ;
#15227=ORIENTED_EDGE ( 'NONE', *, *, #14724, .F. ) ;
#15228=CARTESIAN_POINT ( 'NONE',  ( -7.022189441860112050E-16, 13.67729811471672363, -93.60160580289947063 ) ) ;
#15229=( BOUNDED_CURVE ( )  B_SPLINE_CURVE ( 2, ( #19934, #3350, #36303, #35686, #6549, #22918, #152, #4188, #16338 ),
 .UNSPECIFIED., .F., .F. ) 
 B_SPLINE_CURVE_WITH_KNOTS ( ( 3, 2, 2, 2, 3 ),
 ( 0.8229166666666666297, 0.8236111111111110716, 0.8249999999999999556, 0.8263888888888888395, 0.8270833333333332815 ),
 .UNSPECIFIED. ) 
 CURVE ( )  GEOMETRIC_REPRESENTATION_ITEM ( )  RATIONAL_B_SPLINE_CURVE ( ( 0.9330127018922194093, 0.9330127018922194093, 1.000000000000000000, 0.8660254037844387076, 1.000000000000000000, 0.8660254037844387076, 1.000000000000000000, 0.9330127018922194093, 0.9330127018922194093 ) ) 
 REPRESENTATION_ITEM ( '' )  );
#15232=CYLINDRICAL_SURFACE ( 'NONE', #6403, 3.499999999999999556 ) ;
#15233=DIRECTION ( 'NONE',  ( -0.000000000000000000, 1.259100132267607459E-16, -1.000000000000000000 ) ) ;
#15234=CARTESIAN_POINT ( 'NONE',  ( -3.310556943750002201, 15.58864905735836714, -53.68077246956612925 ) ) ;
#15236=CARTESIAN_POINT ( 'NONE',  ( 2.340729813953370519E-16, 21.32270188528331900, -113.0141058028994649 ) ) ;
#15237=CARTESIAN_POINT ( 'NONE',  ( -1.749999999999999778, 20.53108891324555429, -101.8213974700440900 ) ) ;
#15238=( BOUNDED_CURVE ( )  B_SPLINE_CURVE ( 2, ( #23174, #19560, #15973, #16184, #19355, #35525, #22964, #203, #35933 ),
 .UNSPECIFIED., .F., .F. ) 
 B_SPLINE_CURVE_WITH_KNOTS ( ( 3, 2, 2, 2, 3 ),
 ( 0.9062500000000000000, 0.9069444444444444420, 0.9083333333333333259, 0.9097222222222222099, 0.9104166666666666519 ),
 .UNSPECIFIED. ) 
 CURVE ( )  GEOMETRIC_REPRESENTATION_ITEM ( )  RATIONAL_B_SPLINE_CURVE ( ( 0.9330127018922194093, 0.9330127018922194093, 1.000000000000000000, 0.8660254037844387076, 1.000000000000000000, 0.8660254037844387076, 1.000000000000000000, 0.9330127018922194093, 0.9330127018922194093 ) ) 
 REPRESENTATION_ITEM ( '' )  );
#15239=VERTEX_POINT ( 'NONE', #21722 ) ;
#15241=ORIENTED_EDGE ( 'NONE', *, *, #22451, .T. ) ;
#15243=ORIENTED_EDGE ( 'NONE', *, *, #5585, .F. ) ;
#15245=CARTESIAN_POINT ( 'NONE',  ( -1.655278471874999990, 20.36702641396248836, -64.93077246956615056 ) ) ;
#15247=VERTEX_POINT ( 'NONE', #30889 ) ;
#15248=EDGE_CURVE ( 'NONE', #6275, #21152, #33862, .T. ) ;
#15249=EDGE_LOOP ( 'NONE', ( #36967, #19318, #37675, #13433 ) ) ;
#15250=LINE ( 'NONE', #25660, #28015 ) ;
#15251=CARTESIAN_POINT ( 'NONE',  ( -3.500000000000002220, 15.47927405783633503, -142.5713974700441042 ) ) ;
#15252=ADVANCED_FACE ( 'NONE', ( #41087 ), #34696, .T. ) ;
#15254=CARTESIAN_POINT ( 'NONE',  ( 4.286263797015737581E-16, 14.00000000000002487, -149.5231586289125687 ) ) ;
#15258=CARTESIAN_POINT ( 'NONE',  ( 1.655278471874998436, 14.63297358603755072, -131.4307724695661364 ) ) ;
#15260=CARTESIAN_POINT ( 'NONE',  ( -3.310556943750002645, 15.58864905735836714, -42.76827246956613493 ) ) ;
#15261=CARTESIAN_POINT ( 'NONE',  ( -7.022189441860112050E-16, 13.67729811471671475, -31.60160580289945997 ) ) ;
#15262=CARTESIAN_POINT ( 'NONE',  ( 1.655278471875001101, 20.36702641396249192, -94.18493913623279923 ) ) ;
#15263=CARTESIAN_POINT ( 'NONE',  ( 1.749999999999998224, 14.46891108675447235, -23.32139747004409358 ) ) ;
#15264=ORIENTED_EDGE ( 'NONE', *, *, #3781, .T. ) ;
#15266=CARTESIAN_POINT ( 'NONE',  ( -7.022189441860112050E-16, 13.67729811471672896, -139.6016058028994564 ) ) ;
#15269=CARTESIAN_POINT ( 'NONE',  ( 3.500000000000001332, 17.50000000000002487, -136.1547308033774186 ) ) ;
#15271=CARTESIAN_POINT ( 'NONE',  ( 1.749999999999998224, 14.46891108675448123, -82.32139747004410424 ) ) ;
#15272=CARTESIAN_POINT ( 'NONE',  ( -7.022189441860112050E-16, 13.67729811471672186, -66.60160580289945642 ) ) ;
#15274=CARTESIAN_POINT ( 'NONE',  ( -3.500000000000001332, 17.50000000000002487, -136.9609808024214885 ) ) ;
#15275=CARTESIAN_POINT ( 'NONE',  ( -3.500000000000002220, 15.47927405783632970, -90.87764746908817415 ) ) ;
#15276=CARTESIAN_POINT ( 'NONE',  ( 4.648177544792955347E-16, 21.00000000000001421, -60.21098080242150274 ) ) ;
#15278=CARTESIAN_POINT ( 'NONE',  ( 3.310556943750001313, 19.41135094264166838, -118.1807724695661364 ) ) ;
#15280=CARTESIAN_POINT ( 'NONE',  ( 4.286263797015737581E-16, 14.00000000000002487, -149.5231586289125687 ) ) ;
#15283=EDGE_LOOP ( 'NONE', ( #34289, #22969, #16497, #30494 ) ) ;
#15284=CARTESIAN_POINT ( 'NONE',  ( -3.500000000000000888, 19.52072594216371826, -109.7380641367107614 ) ) ;
#15285=CARTESIAN_POINT ( 'NONE',  ( -0.9378221735089291577, 21.00000000000001066, -28.86007260463891200 ) ) ;
#15286=AXIS2_PLACEMENT_3D ( 'NONE', #11373, #18383, #9014 ) ;
#15287=EDGE_CURVE ( 'NONE', #4141, #4881, #39554, .T. ) ;
#15289=CARTESIAN_POINT ( 'NONE',  ( 0.9378221735089300459, 21.00000000000001066, -37.25563900116003424 ) ) ;
#15292=CARTESIAN_POINT ( 'NONE',  ( -1.655278471874999990, 20.36702641396248836, -71.93077246956613635 ) ) ;
#15293=CARTESIAN_POINT ( 'NONE',  ( -1.750000000000002220, 14.46891108675448123, -78.79431413575484555 ) ) ;
#15295=VERTEX_POINT ( 'NONE', #32344 ) ;
#15296=CARTESIAN_POINT ( 'NONE',  ( -3.500000000000001332, 17.50000000000002487, -132.9609808024214885 ) ) ;
#15297=ADVANCED_FACE ( 'NONE', ( #3210 ), #39334, .T. ) ;
#15298=CYLINDRICAL_SURFACE ( 'NONE', #7655, 3.499999999999999556 ) ;
#15299=CARTESIAN_POINT ( 'NONE',  ( 3.310556943750001313, 17.50000000000001776, -81.26410580289947916 ) ) ;
#15300=ORIENTED_EDGE ( 'NONE', *, *, #25593, .T. ) ;
#15303=CARTESIAN_POINT ( 'NONE',  ( -1.750000000000002220, 14.46891108675447768, -48.48806413671076854 ) ) ;
#15304=EDGE_CURVE ( 'NONE', #33952, #18853, #10497, .T. ) ;
#15305=( BOUNDED_CURVE ( )  B_SPLINE_CURVE ( 2, ( #33755, #17382, #24190, #14182, #36948, #10994, #27778, #33956, #27579 ),
 .UNSPECIFIED., .F., .T. ) 
 B_SPLINE_CURVE_WITH_KNOTS ( ( 3, 2, 2, 2, 3 ),
 ( 0.4770833333333333592, 0.4777777777777778012, 0.4791666666666666852, 0.4805555555555555691, 0.4812500000000000111 ),
 .UNSPECIFIED. ) 
 CURVE ( )  GEOMETRIC_REPRESENTATION_ITEM ( )  RATIONAL_B_SPLINE_CURVE ( ( 0.9330127018922194093, 0.9330127018922220739, 1.000000000000000000, 0.8660254037844387076, 1.000000000000000000, 0.8660254037844387076, 1.000000000000000000, 0.9330127018922194093, 0.9330127018922194093 ) ) 
 REPRESENTATION_ITEM ( '' )  );
#15307=DIRECTION ( 'NONE',  ( 0.000000000000000000, 1.000000000000000000, 0.000000000000000000 ) ) ;
#15311=CARTESIAN_POINT ( 'NONE',  ( -3.310556943750000425, 19.41135094264166128, -48.93493913623281344 ) ) ;
#15312=CARTESIAN_POINT ( 'NONE',  ( -3.310556943750001313, 17.50000000000002132, -108.8516058028994564 ) ) ;
#15314=CARTESIAN_POINT ( 'NONE',  ( 3.310556943749999981, 15.58864905735836182, -33.34743913623280775 ) ) ;
#15315=CARTESIAN_POINT ( 'NONE',  ( -3.310556943750000425, 19.41135094264166128, -62.93493913623279212 ) ) ;
#15316=CARTESIAN_POINT ( 'NONE',  ( -1.750000000000002220, 14.46891108675448478, -107.7943141357548456 ) ) ;
#15318=CARTESIAN_POINT ( 'NONE',  ( 1.655278471874998436, 14.63297358603754539, -91.43077246956613635 ) ) ;
#15319=CARTESIAN_POINT ( 'NONE',  ( -1.749999999999999778, 20.53108891324555429, -98.82139747004409003 ) ) ;
#15320=LINE ( 'NONE', #28276, #11204 ) ;
#15323=CARTESIAN_POINT ( 'NONE',  ( 3.500000000000001332, 17.50000000000001421, -66.46098080242150274 ) ) ;
#15325=CARTESIAN_POINT ( 'NONE',  ( 2.340729813953370519E-16, 21.32270188528330479, -28.01410580289947916 ) ) ;
#15326=CARTESIAN_POINT ( 'NONE',  ( 1.749999999999998224, 14.46891108675447768, -55.32139747004409713 ) ) ;
#15328=CARTESIAN_POINT ( 'NONE',  ( -3.310556943750002201, 15.58864905735837425, -105.7682724695661278 ) ) ;
#15330=CARTESIAN_POINT ( 'NONE',  ( -1.655278471874999990, 20.36702641396248481, -33.01827246956613493 ) ) ;
#15335=DIRECTION ( 'NONE',  ( -0.000000000000000000, 1.259100132267607459E-16, -1.000000000000000000 ) ) ;
#15337=CARTESIAN_POINT ( 'NONE',  ( 1.655278471875001101, 20.36702641396249192, -85.09743913623279354 ) ) ;
#15346=ORIENTED_EDGE ( 'NONE', *, *, #40202, .F. ) ;
#15348=CARTESIAN_POINT ( 'NONE',  ( -1.749999999999999778, 20.53108891324554719, -31.12764746908817770 ) ) ;
#15349=ADVANCED_FACE ( 'NONE', ( #13400 ), #25973, .T. ) ;
#15351=CARTESIAN_POINT ( 'NONE',  ( -7.022189441860112050E-16, 13.67729811471672541, -96.51410580289946495 ) ) ;
#15353=VERTEX_POINT ( 'NONE', #38728 ) ;
#15354=LINE ( 'NONE', #25335, #12094 ) ;
#15355=ORIENTED_EDGE ( 'NONE', *, *, #30793, .F. ) ;
#15361=CARTESIAN_POINT ( 'NONE',  ( 0.000000000000000000, 17.50000000000002487, -149.5231586289125687 ) ) ;
#15362=( BOUNDED_CURVE ( )  B_SPLINE_CURVE ( 2, ( #33814, #1278, #33608, #14247, #27225, #40189, #4467, #40811, #39979 ),
 .UNSPECIFIED., .F., .T. ) 
 B_SPLINE_CURVE_WITH_KNOTS ( ( 3, 2, 2, 2, 3 ),
 ( 0.1854166666666666741, 0.1861111111111111160, 0.1875000000000000000, 0.1888888888888888840, 0.1895833333333333259 ),
 .UNSPECIFIED. ) 
 CURVE ( )  GEOMETRIC_REPRESENTATION_ITEM ( )  RATIONAL_B_SPLINE_CURVE ( ( 0.9330127018922194093, 0.9330127018922194093, 1.000000000000000000, 0.8660254037844387076, 1.000000000000000000, 0.8660254037844387076, 1.000000000000000000, 0.9330127018922194093, 0.9330127018922194093 ) ) 
 REPRESENTATION_ITEM ( '' )  );
#15363=DIRECTION ( 'NONE',  ( -0.000000000000000000, 1.259100132267607459E-16, -1.000000000000000000 ) ) ;
#15364=CARTESIAN_POINT ( 'NONE',  ( 3.310556943749999981, 15.58864905735837780, -139.3474391362327935 ) ) ;
#15365=CARTESIAN_POINT ( 'NONE',  ( 4.648177544792955347E-16, 21.00000000000002487, -132.9047308033774186 ) ) ;
#15368=CARTESIAN_POINT ( 'NONE',  ( -3.310556943750001313, 17.50000000000002132, -122.8516058028994564 ) ) ;
#15369=CARTESIAN_POINT ( 'NONE',  ( -3.310556943750002645, 15.58864905735836714, -52.76827246956612782 ) ) ;
#15372=CARTESIAN_POINT ( 'NONE',  ( -1.749999999999999778, 20.53108891324556140, -137.8213974700441042 ) ) ;
#15376=CARTESIAN_POINT ( 'NONE',  ( 1.655278471874998436, 14.63297358603754361, -79.51827246956614204 ) ) ;
#15377=CARTESIAN_POINT ( 'NONE',  ( -1.749999999999999778, 20.53108891324555785, -129.1276474690881741 ) ) ;
#15378=CARTESIAN_POINT ( 'NONE',  ( -3.310556943750000425, 19.41135094264166838, -109.8474391362328078 ) ) ;
#15379=CYLINDRICAL_SURFACE ( 'NONE', #7121, 3.499999999999999556 ) ;
#15382=CARTESIAN_POINT ( 'NONE',  ( -1.749999999999999778, 20.53108891324555429, -81.12764746908818836 ) ) ;
#15383=CARTESIAN_POINT ( 'NONE',  ( -3.500000000000001332, 17.50000000000001421, -61.96098080242150274 ) ) ;
#15384=CARTESIAN_POINT ( 'NONE',  ( 1.655278471874998436, 14.63297358603754006, -40.43077246956613635 ) ) ;
#15385=CARTESIAN_POINT ( 'NONE',  ( -3.310556943750000425, 19.41135094264166483, -98.93493913623279923 ) ) ;
#15386=FACE_OUTER_BOUND ( 'NONE', #19942, .T. ) ;
#15387=VERTEX_POINT ( 'NONE', #22773 ) ;
#15388=CARTESIAN_POINT ( 'NONE',  ( -7.022189441860112050E-16, 13.67729811471672896, -125.6016058028994706 ) ) ;
#15394=EDGE_LOOP ( 'NONE', ( #29290, #32238, #15078, #10018 ) ) ;
#15395=CARTESIAN_POINT ( 'NONE',  ( -3.310556943750001313, 17.50000000000001776, -74.85160580289947063 ) ) ;
#15396=CYLINDRICAL_SURFACE ( 'NONE', #10871, 3.499999999999999556 ) ;
#15398=CARTESIAN_POINT ( 'NONE',  ( -0.9378221735089291577, 21.00000000000001421, -56.16632260368299256 ) ) ;
#15402=CARTESIAN_POINT ( 'NONE',  ( 1.655278471874998436, 14.63297358603753828, -32.43077246956614346 ) ) ;
#15403=DIRECTION ( 'NONE',  ( -0.000000000000000000, 1.259100132267607459E-16, -1.000000000000000000 ) ) ;
#15407=CARTESIAN_POINT ( 'NONE',  ( -3.310556943750001313, 17.50000000000001421, -48.76410580289947205 ) ) ;
#15410=CARTESIAN_POINT ( 'NONE',  ( 0.9378221735089300459, 21.00000000000001421, -55.94938900211595012 ) ) ;
#15411=CARTESIAN_POINT ( 'NONE',  ( -1.750000000000002220, 14.46891108675447413, -24.79431413575484910 ) ) ;
#15415=CARTESIAN_POINT ( 'NONE',  ( 3.500000000000001776, 19.52072594216370405, -41.37764746908817415 ) ) ;
#15417=DIRECTION ( 'NONE',  ( -0.000000000000000000, 1.259100132267607459E-16, -1.000000000000000000 ) ) ;
#15420=CARTESIAN_POINT ( 'NONE',  ( -7.424026671074350129E-16, 13.45854811567264164, -142.7109808024215170 ) ) ;
#15422=CARTESIAN_POINT ( 'NONE',  ( -3.310556943750000425, 19.41135094264166838, -127.8474391362328078 ) ) ;
#15426=CARTESIAN_POINT ( 'NONE',  ( 1.655278471874998436, 14.63297358603754894, -117.5182724695661278 ) ) ;
#15427=CARTESIAN_POINT ( 'NONE',  ( -3.500000000000002220, 15.47927405783632615, -55.57139747004410424 ) ) ;
#15428=CARTESIAN_POINT ( 'NONE',  ( -3.500000000000001332, 17.50000000000001066, -39.65473080337743284 ) ) ;
#15431=CARTESIAN_POINT ( 'NONE',  ( 3.310556943750001313, 17.50000000000002487, -138.3516058028994564 ) ) ;
#15434=EDGE_CURVE ( 'NONE', #24957, #15800, #16606, .T. ) ;
#15435=CARTESIAN_POINT ( 'NONE',  ( 2.340729813953370519E-16, 21.32270188528331190, -51.10160580289946353 ) ) ;
#15437=CARTESIAN_POINT ( 'NONE',  ( 4.648177544792955347E-16, 21.00000000000002132, -114.9047308033774186 ) ) ;
#15438=CARTESIAN_POINT ( 'NONE',  ( -1.655278471874999990, 20.36702641396248836, -74.01827246956612782 ) ) ;
#15440=CARTESIAN_POINT ( 'NONE',  ( 2.340729813953370519E-16, 21.32270188528330834, -68.01410580289947916 ) ) ;
#15442=CARTESIAN_POINT ( 'NONE',  ( 3.310556943750001313, 19.41135094264166838, -91.26827246956612782 ) ) ;
#15446=CARTESIAN_POINT ( 'NONE',  ( 4.286263797015737581E-16, 14.00000000000002487, -149.5231586289125687 ) ) ;
#15447=CARTESIAN_POINT ( 'NONE',  ( -1.655278471874999990, 20.36702641396248836, -50.93077246956613635 ) ) ;
#15449=CARTESIAN_POINT ( 'NONE',  ( -7.022189441860112050E-16, 13.67729811471672718, -113.5141058028994792 ) ) ;
#15450=CARTESIAN_POINT ( 'NONE',  ( 0.9378221735089300459, 21.00000000000001776, -95.94938900211595012 ) ) ;
#15451=VERTEX_POINT ( 'NONE', #427 ) ;
#15452=ORIENTED_EDGE ( 'NONE', *, *, #24416, .F. ) ;
#15454=ORIENTED_EDGE ( 'NONE', *, *, #7921, .F. ) ;
#15456=CARTESIAN_POINT ( 'NONE',  ( -7.022189441860112050E-16, 13.67729811471671830, -63.51410580289947205 ) ) ;
#15459=EDGE_CURVE ( 'NONE', #31863, #18625, #35116, .T. ) ;
#15464=CARTESIAN_POINT ( 'NONE',  ( 0.000000000000000000, 17.50000000000002487, -149.5231586289125687 ) ) ;
#15466=DIRECTION ( 'NONE',  ( -0.000000000000000000, 1.259100132267607459E-16, -1.000000000000000000 ) ) ;
#15467=CARTESIAN_POINT ( 'NONE',  ( 1.655278471875001101, 20.36702641396249547, -129.0974391362328220 ) ) ;
#15469=CARTESIAN_POINT ( 'NONE',  ( 3.310556943750001313, 19.41135094264165772, -38.26827246956612782 ) ) ;
#15470=CARTESIAN_POINT ( 'NONE',  ( 1.655278471874998436, 14.63297358603753828, -27.51827246956613138 ) ) ;
#15471=CARTESIAN_POINT ( 'NONE',  ( 1.655278471875001101, 20.36702641396249192, -91.18493913623279923 ) ) ;
#15472=CARTESIAN_POINT ( 'NONE',  ( 3.500000000000001332, 17.50000000000001066, -25.15473080337743284 ) ) ;
#15475=( BOUNDED_CURVE ( )  B_SPLINE_CURVE ( 2, ( #27075, #40875, #8336, #37689, #40466, #20898, #37894, #30894, #15144 ),
 .UNSPECIFIED., .F., .T. ) 
 B_SPLINE_CURVE_WITH_KNOTS ( ( 3, 2, 2, 2, 3 ),
 ( 0.6604166666666666519, 0.6611111111111110938, 0.6624999999999999778, 0.6638888888888888618, 0.6645833333333333037 ),
 .UNSPECIFIED. ) 
 CURVE ( )  GEOMETRIC_REPRESENTATION_ITEM ( )  RATIONAL_B_SPLINE_CURVE ( ( 0.9330127018922194093, 0.9330127018922194093, 1.000000000000000000, 0.8660254037844387076, 1.000000000000000000, 0.8660254037844387076, 1.000000000000000000, 0.9330127018922194093, 0.9330127018922194093 ) ) 
 REPRESENTATION_ITEM ( '' )  );
#15476=CARTESIAN_POINT ( 'NONE',  ( 2.340729813953370519E-16, 21.32270188528332255, -133.1016058028994564 ) ) ;
#15477=CARTESIAN_POINT ( 'NONE',  ( -0.9378221735089291577, 21.00000000000001776, -84.16632260368299967 ) ) ;
#15481=CARTESIAN_POINT ( 'NONE',  ( -7.424026671074350129E-16, 13.45854811567263454, -78.40473080337743284 ) ) ;
#15482=CARTESIAN_POINT ( 'NONE',  ( 2.340729813953370519E-16, 21.32270188528331190, -67.10160580289947063 ) ) ;
#15485=DIRECTION ( 'NONE',  ( -0.000000000000000000, 1.259100132267607459E-16, -1.000000000000000000 ) ) ;
#15486=CARTESIAN_POINT ( 'NONE',  ( 3.310556943750001313, 17.50000000000001776, -88.35160580289947063 ) ) ;
#15489=CARTESIAN_POINT ( 'NONE',  ( 2.340729813953370519E-16, 21.32270188528331900, -113.0141058028994792 ) ) ;
#15492=ORIENTED_EDGE ( 'NONE', *, *, #6621, .T. ) ;
#15493=ADVANCED_FACE ( 'NONE', ( #14465 ), #26595, .T. ) ;
#15494=CARTESIAN_POINT ( 'NONE',  ( 3.500000000000001776, 19.52072594216371826, -107.0713974700440900 ) ) ;
#15495=DIRECTION ( 'NONE',  ( -0.000000000000000000, 1.259100132267607459E-16, -1.000000000000000000 ) ) ;
#15498=CARTESIAN_POINT ( 'NONE',  ( -0.9378221735089291577, 21.00000000000001066, -32.86007260463891555 ) ) ;
#15500=CARTESIAN_POINT ( 'NONE',  ( -7.022189441860112050E-16, 13.67729811471672186, -70.51410580289947916 ) ) ;
#15502=CARTESIAN_POINT ( 'NONE',  ( -1.394453263437886604E-15, 14.00000000000001066, -46.71098080242149564 ) ) ;
#15503=CARTESIAN_POINT ( 'NONE',  ( 3.500000000000001332, 17.50000000000001421, -69.46098080242150274 ) ) ;
#15505=CARTESIAN_POINT ( 'NONE',  ( 3.310556943750001313, 17.50000000000001066, -24.26410580289947561 ) ) ;
#15506=CARTESIAN_POINT ( 'NONE',  ( -1.394453263437886604E-15, 14.00000000000001066, -31.71098080242150985 ) ) ;
#15507=CARTESIAN_POINT ( 'NONE',  ( -1.655278471874999990, 20.36702641396249192, -81.93077246956615056 ) ) ;
#15508=EDGE_LOOP ( 'NONE', ( #20107, #36624, #4810, #37731 ) ) ;
#15511=CARTESIAN_POINT ( 'NONE',  ( -1.394453263437886604E-15, 14.00000000000001776, -89.40473080337741862 ) ) ;
#15513=CARTESIAN_POINT ( 'NONE',  ( 4.648177544792955347E-16, 21.00000000000001776, -89.90473080337741862 ) ) ;
#15514=CARTESIAN_POINT ( 'NONE',  ( 3.310556943750001313, 19.41135094264165772, -43.26827246956613493 ) ) ;
#15515=CARTESIAN_POINT ( 'NONE',  ( 3.310556943750001313, 19.41135094264166838, -110.2682724695661420 ) ) ;
#15516=VERTEX_POINT ( 'NONE', #1284 ) ;
#15517=CARTESIAN_POINT ( 'NONE',  ( 3.310556943750001313, 19.41135094264165772, -36.18077246956613635 ) ) ;
#15518=CARTESIAN_POINT ( 'NONE',  ( -3.310556943750000425, 19.41135094264166128, -59.93493913623279212 ) ) ;
#15519=CARTESIAN_POINT ( 'NONE',  ( 1.749999999999998224, 14.46891108675448478, -109.6276474690881741 ) ) ;
#15521=CARTESIAN_POINT ( 'NONE',  ( -3.310556943750000425, 19.41135094264166483, -92.84743913623280775 ) ) ;
#15522=CARTESIAN_POINT ( 'NONE',  ( 3.500000000000000000, 15.47927405783632793, -95.23806413671076143 ) ) ;
#15523=EDGE_CURVE ( 'NONE', #19667, #20461, #30201, .T. ) ;
#15524=CARTESIAN_POINT ( 'NONE',  ( -3.500000000000000000, 19.52072594216371826, -108.7380641367107614 ) ) ;
#15527=CARTESIAN_POINT ( 'NONE',  ( 3.500000000000001776, 19.52072594216370760, -59.37764746908817415 ) ) ;
#15528=CYLINDRICAL_SURFACE ( 'NONE', #27126, 3.499999999999999556 ) ;
#15529=CARTESIAN_POINT ( 'NONE',  ( -7.022189441860112050E-16, 13.67729811471671475, -26.51410580289947916 ) ) ;
#15531=CARTESIAN_POINT ( 'NONE',  ( 1.750000000000001110, 20.53108891324555074, -46.98806413671076143 ) ) ;
#15533=CARTESIAN_POINT ( 'NONE',  ( 3.310556943750001313, 17.50000000000002132, -108.3516058028994564 ) ) ;
#15534=CARTESIAN_POINT ( 'NONE',  ( -3.310556943750002201, 15.58864905735836537, -34.76827246956614204 ) ) ;
#15537=CARTESIAN_POINT ( 'NONE',  ( 3.500000000000001332, 19.52072594216370760, -50.07139747004410424 ) ) ;
#15539=CARTESIAN_POINT ( 'NONE',  ( 0.000000000000000000, 17.50000000000002487, -149.5231586289125687 ) ) ;
#15541=CARTESIAN_POINT ( 'NONE',  ( 3.310556943750001313, 19.41135094264166838, -90.18077246956613635 ) ) ;
#15542=ORIENTED_EDGE ( 'NONE', *, *, #37133, .F. ) ;
#15544=EDGE_LOOP ( 'NONE', ( #9487, #2064, #21871, #28102 ) ) ;
#15547=ORIENTED_EDGE ( 'NONE', *, *, #38141, .F. ) ;
#15550=CARTESIAN_POINT ( 'NONE',  ( -3.310556943750001313, 17.50000000000001776, -95.76410580289946495 ) ) ;
#15552=( BOUNDED_CURVE ( )  B_SPLINE_CURVE ( 2, ( #21637, #28438, #18456, #41219, #15274, #32052, #25260, #31839, #41641 ),
 .UNSPECIFIED., .F., .T. ) 
 B_SPLINE_CURVE_WITH_KNOTS ( ( 3, 2, 2, 2, 3 ),
 ( 0.05208333333333333565, 0.05277777777777777762, 0.05416666666666666852, 0.05555555555555555247, 0.05625000000000000139 ),
 .UNSPECIFIED. ) 
 CURVE ( )  GEOMETRIC_REPRESENTATION_ITEM ( )  RATIONAL_B_SPLINE_CURVE ( ( 0.9330127018922192983, 0.9330127018922196314, 1.000000000000000000, 0.8660254037844387076, 1.000000000000000000, 0.8660254037844387076, 1.000000000000000000, 0.9330127018922189652, 0.9330127018922192983 ) ) 
 REPRESENTATION_ITEM ( '' )  );
#15563=CARTESIAN_POINT ( 'NONE',  ( -1.655278471875002211, 14.63297358603755249, -135.5974391362328220 ) ) ;
#15566=ORIENTED_EDGE ( 'NONE', *, *, #22485, .T. ) ;
#15568=CARTESIAN_POINT ( 'NONE',  ( -1.655278471874999990, 20.36702641396249547, -123.0182724695661278 ) ) ;
#15569=CARTESIAN_POINT ( 'NONE',  ( 3.310556943750001313, 17.50000000000001421, -48.35160580289946353 ) ) ;
#15570=VERTEX_POINT ( 'NONE', #20637 ) ;
#15571=CARTESIAN_POINT ( 'NONE',  ( -7.424026671074350129E-16, 13.45854811567264164, -133.4047308033774186 ) ) ;
#15573=CARTESIAN_POINT ( 'NONE',  ( 3.310556943750001313, 19.41135094264166483, -78.26827246956612782 ) ) ;
#15574=CARTESIAN_POINT ( 'NONE',  ( 3.500000000000000000, 15.47927405783632970, -120.5443141357548456 ) ) ;
#15575=CARTESIAN_POINT ( 'NONE',  ( 3.310556943750001313, 19.41135094264166838, -106.1807724695661506 ) ) ;
#15576=EDGE_CURVE ( 'NONE', #10733, #37225, #12095, .T. ) ;
#15579=CARTESIAN_POINT ( 'NONE',  ( -1.749999999999999778, 20.53108891324555429, -77.12764746908817415 ) ) ;
#15582=CARTESIAN_POINT ( 'NONE',  ( -3.310556943750000425, 19.41135094264165772, -43.84743913623280775 ) ) ;
#15583=CARTESIAN_POINT ( 'NONE',  ( -1.655278471875002211, 14.63297358603754894, -102.6849391362327992 ) ) ;
#15584=CARTESIAN_POINT ( 'NONE',  ( -3.500000000000001332, 17.50000000000002132, -113.9609808024215027 ) ) ;
#15585=CARTESIAN_POINT ( 'NONE',  ( 3.500000000000001332, 17.50000000000001421, -66.15473080337743284 ) ) ;
#15587=ORIENTED_EDGE ( 'NONE', *, *, #6449, .F. ) ;
#15588=CARTESIAN_POINT ( 'NONE',  ( 2.340729813953370519E-16, 21.32270188528331900, -121.1016058028994706 ) ) ;
#15590=CARTESIAN_POINT ( 'NONE',  ( -1.749999999999999778, 20.53108891324554719, -28.12764746908817770 ) ) ;
#15593=CARTESIAN_POINT ( 'NONE',  ( 4.648177544792955347E-16, 21.00000000000001421, -71.90473080337743284 ) ) ;
#15597=CARTESIAN_POINT ( 'NONE',  ( -3.310556943750000425, 19.41135094264166483, -72.93493913623279923 ) ) ;
#15599=CYLINDRICAL_SURFACE ( 'NONE', #17653, 3.499999999999999556 ) ;
#15600=CARTESIAN_POINT ( 'NONE',  ( 0.9378221735089300459, 21.00000000000001066, -39.94938900211595723 ) ) ;
#15604=CARTESIAN_POINT ( 'NONE',  ( 3.310556943750001313, 19.41135094264166128, -34.18077246956615056 ) ) ;
#15608=VERTEX_POINT ( 'NONE', #36582 ) ;
#15609=ADVANCED_FACE ( 'NONE', ( #7450 ), #4474, .T. ) ;
#15611=CARTESIAN_POINT ( 'NONE',  ( -3.310556943750002645, 15.58864905735836714, -47.68077246956615056 ) ) ;
#15616=DIRECTION ( 'NONE',  ( -0.000000000000000000, 1.259100132267607459E-16, -1.000000000000000000 ) ) ;
#15621=CARTESIAN_POINT ( 'NONE',  ( -7.424026671074350129E-16, 13.45854811567263098, -32.71098080242150985 ) ) ;
#15623=LINE ( 'NONE', #24988, #35945 ) ;
#15624=VECTOR ( 'NONE', #276, 1000.000000000000000 ) ;
#15625=CARTESIAN_POINT ( 'NONE',  ( 4.648177544792955347E-16, 21.00000000000001776, -92.21098080242150274 ) ) ;
#15627=CARTESIAN_POINT ( 'NONE',  ( 3.500000000000001332, 17.50000000000002487, -140.4609808024215170 ) ) ;
#15629=CARTESIAN_POINT ( 'NONE',  ( -3.310556943750001313, 17.50000000000002132, -122.7641058028994649 ) ) ;
#15633=DIRECTION ( 'NONE',  ( -0.000000000000000000, 1.259100132267607459E-16, -1.000000000000000000 ) ) ;
#15634=CARTESIAN_POINT ( 'NONE',  ( 2.474675557024783212E-16, 21.54145188432739744, -94.21098080242151696 ) ) ;
#15635=CARTESIAN_POINT ( 'NONE',  ( -1.655278471874999990, 20.36702641396249547, -118.0182724695661278 ) ) ;
#15637=CARTESIAN_POINT ( 'NONE',  ( 2.474675557024783212E-16, 21.54145188432739033, -34.90473080337742573 ) ) ;
#15638=FACE_OUTER_BOUND ( 'NONE', #28666, .T. ) ;
#15640=CARTESIAN_POINT ( 'NONE',  ( -3.310556943750002201, 15.58864905735837958, -137.7682724695661420 ) ) ;
#15642=CARTESIAN_POINT ( 'NONE',  ( 1.655278471875001101, 20.36702641396248836, -47.18493913623279923 ) ) ;
#15644=CARTESIAN_POINT ( 'NONE',  ( -1.394453263437886604E-15, 14.00000000000001421, -72.71098080242151696 ) ) ;
#15645=CARTESIAN_POINT ( 'NONE',  ( 1.655278471875001101, 20.36702641396248836, -67.18493913623279923 ) ) ;
#15648=CARTESIAN_POINT ( 'NONE',  ( -3.310556943750000425, 19.41135094264166128, -72.84743913623279354 ) ) ;
#15649=ORIENTED_EDGE ( 'NONE', *, *, #38166, .T. ) ;
#15650=CARTESIAN_POINT ( 'NONE',  ( -3.310556943750002201, 15.58864905735837247, -92.76827246956611361 ) ) ;
#15653=DIRECTION ( 'NONE',  ( 0.000000000000000000, 1.000000000000000000, 0.000000000000000000 ) ) ;
#15654=LINE ( 'NONE', #19464, #17808 ) ;
#15655=CARTESIAN_POINT ( 'NONE',  ( -3.310556943750002201, 15.58864905735836714, -49.68077246956614346 ) ) ;
#15656=EDGE_CURVE ( 'NONE', #6503, #9388, #41195, .T. ) ;
#15657=LINE ( 'NONE', #21397, #34786 ) ;
#15658=CARTESIAN_POINT ( 'NONE',  ( -1.655278471875002211, 14.63297358603754894, -106.5974391362328078 ) ) ;
#15666=CARTESIAN_POINT ( 'NONE',  ( -1.655278471874999990, 20.36702641396248836, -62.93077246956614346 ) ) ;
#15668=ORIENTED_EDGE ( 'NONE', *, *, #12432, .F. ) ;
#15672=CARTESIAN_POINT ( 'NONE',  ( -1.394453263437886604E-15, 14.00000000000002132, -112.7109808024214885 ) ) ;
#15675=CARTESIAN_POINT ( 'NONE',  ( 3.310556943750001313, 19.41135094264166838, -127.1807724695661364 ) ) ;
#15676=VECTOR ( 'NONE', #19254, 1000.000000000000000 ) ;
#15678=CARTESIAN_POINT ( 'NONE',  ( -3.310556943750001313, 17.50000000000001066, -38.85160580289946353 ) ) ;
#15679=CARTESIAN_POINT ( 'NONE',  ( 3.310556943750001313, 19.41135094264165772, -29.26827246956613138 ) ) ;
#15680=CARTESIAN_POINT ( 'NONE',  ( 1.655278471875001101, 20.36702641396249192, -88.18493913623279923 ) ) ;
#15681=CARTESIAN_POINT ( 'NONE',  ( 1.655278471875001101, 20.36702641396249902, -138.0974391362327935 ) ) ;
#15684=VECTOR ( 'NONE', #1594, 1000.000000000000000 ) ;
#15686=CARTESIAN_POINT ( 'NONE',  ( 3.310556943749999981, 15.58864905735837425, -133.4349391362327992 ) ) ;
#15689=CARTESIAN_POINT ( 'NONE',  ( 1.750000000000001110, 20.53108891324556140, -135.9880641367107614 ) ) ;
#15690=CARTESIAN_POINT ( 'NONE',  ( 0.000000000000000000, 17.50000000000002487, -149.5231586289125687 ) ) ;
#15691=CARTESIAN_POINT ( 'NONE',  ( -7.424026671074350129E-16, 13.45854811567263454, -79.40473080337741862 ) ) ;
#15692=CARTESIAN_POINT ( 'NONE',  ( 1.655278471875001101, 20.36702641396248836, -63.18493913623279923 ) ) ;
#15696=CARTESIAN_POINT ( 'NONE',  ( -3.310556943750000425, 19.41135094264166483, -85.93493913623278502 ) ) ;
#15697=CARTESIAN_POINT ( 'NONE',  ( -1.394453263437886604E-15, 14.00000000000001066, -47.71098080242150274 ) ) ;
#15698=CARTESIAN_POINT ( 'NONE',  ( -3.310556943750002201, 15.58864905735837780, -114.6807724695661364 ) ) ;
#15700=VERTEX_POINT ( 'NONE', #37837 ) ;
#15702=CARTESIAN_POINT ( 'NONE',  ( -3.500000000000000888, 19.52072594216371826, -105.7380641367107614 ) ) ;
#15703=CARTESIAN_POINT ( 'NONE',  ( -1.749999999999999778, 20.53108891324554719, -28.82139747004410069 ) ) ;
#15708=CARTESIAN_POINT ( 'NONE',  ( -3.310556943750000425, 19.41135094264166483, -63.84743913623280775 ) ) ;
#15710=AXIS2_PLACEMENT_3D ( 'NONE', #36850, #20889, #10900 ) ;
#15713=ORIENTED_EDGE ( 'NONE', *, *, #11068, .F. ) ;
#15714=CARTESIAN_POINT ( 'NONE',  ( 1.749999999999998224, 14.46891108675448301, -99.62764746908817415 ) ) ;
#15716=CARTESIAN_POINT ( 'NONE',  ( 3.310556943749999981, 15.58864905735836714, -79.34743913623282197 ) ) ;
#15718=EDGE_LOOP ( 'NONE', ( #21614, #6602, #33652, #20851 ) ) ;
#15720=ADVANCED_FACE ( 'NONE', ( #4880 ), #12089, .T. ) ;
#15724=( BOUNDED_CURVE ( )  B_SPLINE_CURVE ( 2, ( #26472, #32632, #3496, #16486, #306, #6898, #19870, #3705, #7326 ),
 .UNSPECIFIED., .F., .T. ) 
 B_SPLINE_CURVE_WITH_KNOTS ( ( 3, 2, 2, 2, 3 ),
 ( 0.3270833333333333370, 0.3277777777777777790, 0.3291666666666666630, 0.3305555555555555469, 0.3312499999999999889 ),
 .UNSPECIFIED. ) 
 CURVE ( )  GEOMETRIC_REPRESENTATION_ITEM ( )  RATIONAL_B_SPLINE_CURVE ( ( 0.9330127018922194093, 0.9330127018922194093, 1.000000000000000000, 0.8660254037844387076, 1.000000000000000000, 0.8660254037844387076, 1.000000000000000000, 0.9330127018922194093, 0.9330127018922194093 ) ) 
 REPRESENTATION_ITEM ( '' )  );
#15725=CARTESIAN_POINT ( 'NONE',  ( -3.310556943750001313, 17.50000000000001066, -45.85160580289945642 ) ) ;
#15726=CARTESIAN_POINT ( 'NONE',  ( -3.310556943750000425, 19.41135094264166838, -107.9349391362327992 ) ) ;
#15727=ORIENTED_EDGE ( 'NONE', *, *, #39727, .T. ) ;
#15728=CARTESIAN_POINT ( 'NONE',  ( -3.310556943750001313, 17.50000000000001066, -30.76410580289946850 ) ) ;
#15729=CARTESIAN_POINT ( 'NONE',  ( -1.655278471875002211, 14.63297358603754361, -59.68493913623279212 ) ) ;
#15730=CARTESIAN_POINT ( 'NONE',  ( -3.500000000000001332, 17.50000000000002132, -106.9609808024215027 ) ) ;
#15732=CARTESIAN_POINT ( 'NONE',  ( -1.749999999999999778, 20.53108891324555429, -94.82139747004409003 ) ) ;
#15733=CYLINDRICAL_SURFACE ( 'NONE', #23429, 3.499999999999999556 ) ;
#15735=EDGE_CURVE ( 'NONE', #16185, #11917, #19199, .T. ) ;
#15737=CARTESIAN_POINT ( 'NONE',  ( 3.500000000000001776, 19.52072594216370760, -61.37764746908818125 ) ) ;
#15738=CARTESIAN_POINT ( 'NONE',  ( -1.394453263437886604E-15, 14.00000000000001066, -46.71098080242149564 ) ) ;
#15739=CARTESIAN_POINT ( 'NONE',  ( -7.022189441860112050E-16, 13.67729811471671297, -24.51410580289947561 ) ) ;
#15742=CARTESIAN_POINT ( 'NONE',  ( -1.749999999999999778, 20.53108891324555074, -49.82139747004410424 ) ) ;
#15744=CARTESIAN_POINT ( 'NONE',  ( 1.655278471875001101, 20.36702641396248481, -31.18493913623279923 ) ) ;
#15751=CARTESIAN_POINT ( 'NONE',  ( 3.310556943749999981, 15.58864905735836714, -80.34743913623279354 ) ) ;
#15752=ORIENTED_EDGE ( 'NONE', *, *, #22775, .F. ) ;
#15755=CARTESIAN_POINT ( 'NONE',  ( -3.500000000000000000, 19.52072594216371826, -124.0443141357548456 ) ) ;
#15756=ORIENTED_EDGE ( 'NONE', *, *, #969, .T. ) ;
#15759=CARTESIAN_POINT ( 'NONE',  ( 3.310556943750001313, 17.50000000000001776, -97.26410580289947916 ) ) ;
#15762=LINE ( 'NONE', #18528, #21132 ) ;
#15764=CARTESIAN_POINT ( 'NONE',  ( 1.749999999999998224, 14.46891108675448834, -139.6276474690881741 ) ) ;
#15769=EDGE_CURVE ( 'NONE', #28471, #4141, #18700, .T. ) ;
#15771=ORIENTED_EDGE ( 'NONE', *, *, #18892, .T. ) ;
#15773=AXIS2_PLACEMENT_3D ( 'NONE', #15872, #25439, #22439 ) ;
#15774=CARTESIAN_POINT ( 'NONE',  ( 0.9378221735089213862, 21.00000000000002487, -129.2556390011600058 ) ) ;
#15775=EDGE_CURVE ( 'NONE', #4672, #39176, #25081, .T. ) ;
#15776=CARTESIAN_POINT ( 'NONE',  ( -1.655278471875002211, 14.63297358603755249, -131.5974391362328220 ) ) ;
#15777=CARTESIAN_POINT ( 'NONE',  ( 0.9378221735089294908, 14.00000000000002665, -141.6663226036829997 ) ) ;
#15779=CARTESIAN_POINT ( 'NONE',  ( 0.9378221735089300459, 21.00000000000001066, -28.25563900116003069 ) ) ;
#15780=CARTESIAN_POINT ( 'NONE',  ( 2.340729813953370519E-16, 21.32270188528331900, -125.1016058028994564 ) ) ;
#15781=CARTESIAN_POINT ( 'NONE',  ( -3.310556943750002645, 15.58864905735836714, -48.76827246956614204 ) ) ;
#15782=VERTEX_POINT ( 'NONE', #8485 ) ;
#15783=CARTESIAN_POINT ( 'NONE',  ( 3.500000000000000000, 15.47927405783633503, -128.2380641367107614 ) ) ;
#15785=CARTESIAN_POINT ( 'NONE',  ( -1.655278471874999990, 20.36702641396249192, -76.01827246956612782 ) ) ;
#15786=CARTESIAN_POINT ( 'NONE',  ( -7.424026671074350129E-16, 13.45854811567263987, -122.7109808024215027 ) ) ;
#15787=CARTESIAN_POINT ( 'NONE',  ( 1.655278471875001101, 20.36702641396249547, -106.0974391362328078 ) ) ;
#15789=CARTESIAN_POINT ( 'NONE',  ( 0.9378221735089630196, 14.00000000000003553, -93.36007260463891555 ) ) ;
#15793=CARTESIAN_POINT ( 'NONE',  ( -1.749999999999999778, 20.53108891324555074, -74.12764746908817415 ) ) ;
#15795=CARTESIAN_POINT ( 'NONE',  ( 3.310556943749999981, 15.58864905735836182, -42.34743913623279354 ) ) ;
#15796=CARTESIAN_POINT ( 'NONE',  ( -7.022189441860112050E-16, 13.67729811471672541, -102.6016058028994706 ) ) ;
#15797=CARTESIAN_POINT ( 'NONE',  ( 0.000000000000000000, 17.50000000000002487, -149.5231586289125687 ) ) ;
#15798=CARTESIAN_POINT ( 'NONE',  ( 3.500000000000000000, 15.47927405783632260, -65.23806413671076143 ) ) ;
#15800=VERTEX_POINT ( 'NONE', #15511 ) ;
#15801=CARTESIAN_POINT ( 'NONE',  ( 3.310556943750001313, 19.41135094264166838, -120.2682724695661278 ) ) ;
#15802=CARTESIAN_POINT ( 'NONE',  ( -3.500000000000001332, 17.50000000000001066, -27.96098080242151340 ) ) ;
#15805=LINE ( 'NONE', #41539, #37750 ) ;
#15811=CARTESIAN_POINT ( 'NONE',  ( -7.022189441860112050E-16, 13.67729811471672186, -76.60160580289945642 ) ) ;
#15813=CARTESIAN_POINT ( 'NONE',  ( 0.9378221735089300459, 21.00000000000001421, -47.94938900211595012 ) ) ;
#15814=CARTESIAN_POINT ( 'NONE',  ( -1.750000000000002220, 14.46891108675448478, -102.4880641367107756 ) ) ;
#15816=ADVANCED_FACE ( 'NONE', ( #30831 ), #31452, .T. ) ;
#15819=CARTESIAN_POINT ( 'NONE',  ( 2.340729813953370519E-16, 21.32270188528330834, -35.01410580289947205 ) ) ;
#15820=CARTESIAN_POINT ( 'NONE',  ( 1.750000000000001110, 20.53108891324555074, -71.98806413671076143 ) ) ;
#15821=AXIS2_PLACEMENT_3D ( 'NONE', #33034, #13059, #32411 ) ;
#15823=ORIENTED_EDGE ( 'NONE', *, *, #41477, .F. ) ;
#15825=EDGE_CURVE ( 'NONE', #14781, #5598, #7521, .T. ) ;
#15829=ORIENTED_EDGE ( 'NONE', *, *, #296, .T. ) ;
#15835=CARTESIAN_POINT ( 'NONE',  ( -7.424026671074350129E-16, 13.45854811567263987, -117.4047308033774328 ) ) ;
#15836=CARTESIAN_POINT ( 'NONE',  ( 4.286263797015737581E-16, 14.00000000000002487, -149.5231586289125687 ) ) ;
#15837=CARTESIAN_POINT ( 'NONE',  ( 3.500000000000001776, 19.52072594216370405, -33.37764746908818125 ) ) ;
#15838=DIRECTION ( 'NONE',  ( -0.000000000000000000, 1.259100132267607459E-16, -1.000000000000000000 ) ) ;
#15840=CARTESIAN_POINT ( 'NONE',  ( 3.500000000000000000, 15.47927405783632970, -106.2380641367107472 ) ) ;
#15842=CARTESIAN_POINT ( 'NONE',  ( 3.500000000000000000, 15.47927405783633503, -138.5443141357548313 ) ) ;
#15843=CARTESIAN_POINT ( 'NONE',  ( 3.500000000000001332, 17.50000000000002132, -120.4609808024215170 ) ) ;
#15844=CARTESIAN_POINT ( 'NONE',  ( 3.310556943749999981, 15.58864905735837247, -122.3474391362328362 ) ) ;
#15848=CARTESIAN_POINT ( 'NONE',  ( -7.424026671074350129E-16, 13.45854811567263631, -89.71098080242150274 ) ) ;
#15849=CARTESIAN_POINT ( 'NONE',  ( -1.394453263437886604E-15, 14.00000000000001066, -40.71098080242150274 ) ) ;
#15850=CARTESIAN_POINT ( 'NONE',  ( -7.022189441860112050E-16, 13.67729811471671830, -58.51410580289947916 ) ) ;
#15851=CARTESIAN_POINT ( 'NONE',  ( 2.340729813953370519E-16, 21.32270188528331900, -116.1016058028994848 ) ) ;
#15852=CARTESIAN_POINT ( 'NONE',  ( 4.648177544792955347E-16, 21.00000000000001421, -53.90473080337743284 ) ) ;
#15853=CARTESIAN_POINT ( 'NONE',  ( 3.500000000000001332, 17.50000000000001066, -33.15473080337742573 ) ) ;
#15856=CARTESIAN_POINT ( 'NONE',  ( -3.310556943750000425, 19.41135094264167549, -138.9349391362327708 ) ) ;
#15857=AXIS2_PLACEMENT_3D ( 'NONE', #15539, #197, #9361 ) ;
#15859=CARTESIAN_POINT ( 'NONE',  ( 7.785697387528201340E-15, 14.00000000000002487, -138.4047308033774470 ) ) ;
#15860=CARTESIAN_POINT ( 'NONE',  ( 2.340729813953370519E-16, 21.32270188528331190, -50.10160580289946353 ) ) ;
#15863=CARTESIAN_POINT ( 'NONE',  ( 1.655278471875001101, 20.36702641396248836, -68.18493913623279923 ) ) ;
#15865=CARTESIAN_POINT ( 'NONE',  ( 3.310556943750001313, 19.41135094264166128, -72.18077246956613635 ) ) ;
#15867=( BOUNDED_CURVE ( )  B_SPLINE_CURVE ( 2, ( #22841, #35810, #19642, #3477, #16468, #23045, #36013, #29417, #26454 ),
 .UNSPECIFIED., .F., .F. ) 
 B_SPLINE_CURVE_WITH_KNOTS ( ( 3, 2, 2, 2, 3 ),
 ( 0.8854166666666666297, 0.8861111111111110716, 0.8874999999999999556, 0.8888888888888888395, 0.8895833333333332815 ),
 .UNSPECIFIED. ) 
 CURVE ( )  GEOMETRIC_REPRESENTATION_ITEM ( )  RATIONAL_B_SPLINE_CURVE ( ( 0.9330127018922194093, 0.9330127018922194093, 1.000000000000000000, 0.8660254037844387076, 1.000000000000000000, 0.8660254037844387076, 1.000000000000000000, 0.9330127018922194093, 0.9330127018922194093 ) ) 
 REPRESENTATION_ITEM ( '' )  );
#15868=CARTESIAN_POINT ( 'NONE',  ( 3.310556943750001313, 19.41135094264166838, -89.26827246956612782 ) ) ;
#15871=CYLINDRICAL_SURFACE ( 'NONE', #33594, 3.499999999999999556 ) ;
#15872=CARTESIAN_POINT ( 'NONE',  ( 0.000000000000000000, 17.50000000000002487, -149.5231586289125687 ) ) ;
#15873=CARTESIAN_POINT ( 'NONE',  ( -1.655278471874999990, 20.36702641396248836, -48.93077246956615056 ) ) ;
#15875=CARTESIAN_POINT ( 'NONE',  ( 3.310556943749999981, 15.58864905735837070, -107.3474391362327935 ) ) ;
#15876=CARTESIAN_POINT ( 'NONE',  ( 3.500000000000000000, 15.47927405783632970, -96.23806413671076143 ) ) ;
#15877=ORIENTED_EDGE ( 'NONE', *, *, #41899, .F. ) ;
#15882=EDGE_CURVE ( 'NONE', #37421, #18226, #11860, .T. ) ;
#15883=CARTESIAN_POINT ( 'NONE',  ( 3.310556943749999981, 15.58864905735836537, -55.34743913623281486 ) ) ;
#15884=ORIENTED_EDGE ( 'NONE', *, *, #40769, .T. ) ;
#15885=ORIENTED_EDGE ( 'NONE', *, *, #28250, .T. ) ;
#15887=CARTESIAN_POINT ( 'NONE',  ( -1.394453263437886604E-15, 14.00000000000001421, -58.71098080242150985 ) ) ;
#15890=CARTESIAN_POINT ( 'NONE',  ( 0.000000000000000000, 17.50000000000002487, -149.5231586289125687 ) ) ;
#15891=ORIENTED_EDGE ( 'NONE', *, *, #17312, .T. ) ;
#15892=CARTESIAN_POINT ( 'NONE',  ( -1.750000000000002220, 14.46891108675447946, -54.79431413575484555 ) ) ;
#15893=CARTESIAN_POINT ( 'NONE',  ( 1.655278471874998436, 14.63297358603755072, -126.4307724695661364 ) ) ;
#15897=CARTESIAN_POINT ( 'NONE',  ( -1.655278471874999990, 20.36702641396248481, -37.01827246956612782 ) ) ;
#15898=CARTESIAN_POINT ( 'NONE',  ( -1.655278471874999990, 20.36702641396248481, -30.01827246956613493 ) ) ;
#15899=CARTESIAN_POINT ( 'NONE',  ( 3.310556943749999981, 15.58864905735836892, -85.43493913623278502 ) ) ;
#15900=CARTESIAN_POINT ( 'NONE',  ( -3.310556943750000425, 19.41135094264167549, -138.8474391362327935 ) ) ;
#15902=CARTESIAN_POINT ( 'NONE',  ( 1.655278471875001101, 20.36702641396249902, -131.1849391362327992 ) ) ;
#15907=CARTESIAN_POINT ( 'NONE',  ( -1.750000000000002220, 14.46891108675448123, -79.48806413671076143 ) ) ;
#15908=CARTESIAN_POINT ( 'NONE',  ( 2.340729813953370519E-16, 21.32270188528331190, -62.10160580289945642 ) ) ;
#15912=CARTESIAN_POINT ( 'NONE',  ( -1.655278471875002211, 14.63297358603754716, -85.68493913623278502 ) ) ;
#15914=CARTESIAN_POINT ( 'NONE',  ( 2.340729813953370519E-16, 21.32270188528331900, -114.0141058028994792 ) ) ;
#15915=CARTESIAN_POINT ( 'NONE',  ( 3.500000000000001332, 19.52072594216370405, -34.37764746908818125 ) ) ;
#15917=ORIENTED_EDGE ( 'NONE', *, *, #33772, .T. ) ;
#15918=CARTESIAN_POINT ( 'NONE',  ( 1.750000000000001110, 20.53108891324555785, -105.9880641367107614 ) ) ;
#15923=CARTESIAN_POINT ( 'NONE',  ( 0.9378221735089281585, 14.00000000000001066, -45.66632260368297835 ) ) ;
#15926=CARTESIAN_POINT ( 'NONE',  ( -3.310556943750002201, 15.58864905735837070, -68.68077246956613635 ) ) ;
#15928=CARTESIAN_POINT ( 'NONE',  ( -7.022189441860112050E-16, 13.67729811471672718, -121.5141058028994792 ) ) ;
#15929=LINE ( 'NONE', #29083, #580 ) ;
#15933=CARTESIAN_POINT ( 'NONE',  ( -3.500000000000001332, 17.50000000000002132, -103.9609808024215027 ) ) ;
#15936=CARTESIAN_POINT ( 'NONE',  ( 1.655278471874998436, 14.63297358603754361, -73.43077246956613635 ) ) ;
#15938=ORIENTED_EDGE ( 'NONE', *, *, #23772, .T. ) ;
#15939=CARTESIAN_POINT ( 'NONE',  ( -0.9378221735089310451, 14.00000000000001066, -53.44938900211595723 ) ) ;
#15940=CARTESIAN_POINT ( 'NONE',  ( -1.655278471875002211, 14.63297358603755427, -140.5974391362327935 ) ) ;
#15942=VECTOR ( 'NONE', #26507, 1000.000000000000114 ) ;
#15944=CARTESIAN_POINT ( 'NONE',  ( -7.022189441860112050E-16, 13.67729811471671653, -44.60160580289947063 ) ) ;
#15945=CARTESIAN_POINT ( 'NONE',  ( -7.022189441860112050E-16, 13.67729811471672541, -104.6016058028994564 ) ) ;
#15946=ORIENTED_EDGE ( 'NONE', *, *, #41458, .T. ) ;
#15947=CARTESIAN_POINT ( 'NONE',  ( -1.655278471874999990, 20.36702641396248481, -28.93077246956614346 ) ) ;
#15948=VECTOR ( 'NONE', #39395, 1000.000000000000000 ) ;
#15950=CARTESIAN_POINT ( 'NONE',  ( 3.500000000000001776, 19.52072594216371826, -105.3776474690881884 ) ) ;
#15953=CARTESIAN_POINT ( 'NONE',  ( 1.749999999999998224, 14.46891108675448301, -96.32139747004409003 ) ) ;
#15954=CARTESIAN_POINT ( 'NONE',  ( 0.9378221735089300459, 21.00000000000001421, -63.25563900116003424 ) ) ;
#15957=CARTESIAN_POINT ( 'NONE',  ( -7.424026671074350129E-16, 13.45854811567263454, -57.71098080242150985 ) ) ;
#15959=CARTESIAN_POINT ( 'NONE',  ( 3.310556943750001313, 19.41135094264165772, -29.18077246956613990 ) ) ;
#15960=CARTESIAN_POINT ( 'NONE',  ( 3.500000000000001776, 19.52072594216370760, -51.07139747004409713 ) ) ;
#15961=CARTESIAN_POINT ( 'NONE',  ( 0.9378221735089300459, 21.00000000000001776, -77.25563900116002003 ) ) ;
#15962=CARTESIAN_POINT ( 'NONE',  ( 3.310556943749999981, 15.58864905735836182, -33.43493913623279923 ) ) ;
#15965=DIRECTION ( 'NONE',  ( -0.000000000000000000, 1.259100132267607459E-16, -1.000000000000000000 ) ) ;
#15970=CARTESIAN_POINT ( 'NONE',  ( -3.310556943750002201, 15.58864905735837247, -81.68077246956613635 ) ) ;
#15971=CARTESIAN_POINT ( 'NONE',  ( -3.500000000000002220, 15.47927405783632082, -25.57139747004409713 ) ) ;
#15973=CARTESIAN_POINT ( 'NONE',  ( 1.749999999999998224, 14.46891108675447413, -34.32139747004410424 ) ) ;
#15974=CARTESIAN_POINT ( 'NONE',  ( 0.9378221735089630196, 14.00000000000003730, -108.3600726046389155 ) ) ;
#15978=CARTESIAN_POINT ( 'NONE',  ( 1.655278471874998436, 14.63297358603754539, -93.43077246956613635 ) ) ;
#15980=ORIENTED_EDGE ( 'NONE', *, *, #23524, .F. ) ;
#15981=CYLINDRICAL_SURFACE ( 'NONE', #17735, 3.499999999999999556 ) ;
#15983=( BOUNDED_CURVE ( )  B_SPLINE_CURVE ( 2, ( #4994, #40721, #24571, #17767, #1602, #36917, #11791, #24363, #33728 ),
 .UNSPECIFIED., .F., .T. ) 
 B_SPLINE_CURVE_WITH_KNOTS ( ( 3, 2, 2, 2, 3 ),
 ( 0.3020833333333333148, 0.3027777777777777568, 0.3041666666666666408, 0.3055555555555555802, 0.3062500000000000222 ),
 .UNSPECIFIED. ) 
 CURVE ( )  GEOMETRIC_REPRESENTATION_ITEM ( )  RATIONAL_B_SPLINE_CURVE ( ( 0.9330127018922194093, 0.9330127018922194093, 1.000000000000000000, 0.8660254037844387076, 1.000000000000000000, 0.8660254037844387076, 1.000000000000000000, 0.9330127018922194093, 0.9330127018922194093 ) ) 
 REPRESENTATION_ITEM ( '' )  );
#15984=AXIS2_PLACEMENT_3D ( 'NONE', #8284, #24252, #24052 ) ;
#15985=( BOUNDED_CURVE ( )  B_SPLINE_CURVE ( 2, ( #4112, #33037, #33690, #30059, #37093, #30485, #36661, #20713, #934 ),
 .UNSPECIFIED., .F., .T. ) 
 B_SPLINE_CURVE_WITH_KNOTS ( ( 3, 2, 2, 2, 3 ),
 ( 0.4104166666666666519, 0.4111111111111110938, 0.4124999999999999778, 0.4138888888888888618, 0.4145833333333333592 ),
 .UNSPECIFIED. ) 
 CURVE ( )  GEOMETRIC_REPRESENTATION_ITEM ( )  RATIONAL_B_SPLINE_CURVE ( ( 0.9330127018922194093, 0.9330127018922194093, 1.000000000000000000, 0.8660254037844387076, 1.000000000000000000, 0.8660254037844387076, 1.000000000000000000, 0.9330127018922167448, 0.9330127018922194093 ) ) 
 REPRESENTATION_ITEM ( '' )  );
#15990=ORIENTED_EDGE ( 'NONE', *, *, #7143, .F. ) ;
#15993=CARTESIAN_POINT ( 'NONE',  ( 4.286263797015737581E-16, 14.00000000000002487, -149.5231586289125687 ) ) ;
#15995=CARTESIAN_POINT ( 'NONE',  ( 2.340729813953370519E-16, 21.32270188528332255, -133.0141058028994792 ) ) ;
#15996=ORIENTED_EDGE ( 'NONE', *, *, #24369, .F. ) ;
#15997=CARTESIAN_POINT ( 'NONE',  ( 3.500000000000001332, 19.52072594216371826, -139.0713974700441042 ) ) ;
#15998=CARTESIAN_POINT ( 'NONE',  ( 3.310556943750001313, 17.50000000000002132, -120.3516058028994706 ) ) ;
#15999=CARTESIAN_POINT ( 'NONE',  ( -3.310556943750001313, 17.50000000000001421, -49.85160580289946353 ) ) ;
#16001=CARTESIAN_POINT ( 'NONE',  ( -3.500000000000001332, 17.50000000000002487, -132.6547308033774186 ) ) ;
#16003=CARTESIAN_POINT ( 'NONE',  ( -3.310556943750000425, 19.41135094264166483, -77.93493913623279923 ) ) ;
#16004=CARTESIAN_POINT ( 'NONE',  ( -1.749999999999999778, 20.53108891324555785, -124.1276474690881599 ) ) ;
#16005=CARTESIAN_POINT ( 'NONE',  ( 2.340729813953370519E-16, 21.32270188528331900, -109.0141058028994792 ) ) ;
#16006=LINE ( 'NONE', #21946, #5085 ) ;
#16009=CARTESIAN_POINT ( 'NONE',  ( 3.500000000000001332, 17.50000000000001776, -77.46098080242150274 ) ) ;
#16012=CARTESIAN_POINT ( 'NONE',  ( -1.655278471875002211, 14.63297358603754184, -43.59743913623280775 ) ) ;
#16013=CARTESIAN_POINT ( 'NONE',  ( -3.310556943750001313, 17.50000000000001776, -100.8516058028994706 ) ) ;
#16014=CARTESIAN_POINT ( 'NONE',  ( 0.9378221735089281585, 14.00000000000001599, -68.36007260463890134 ) ) ;
#16015=CARTESIAN_POINT ( 'NONE',  ( -1.750000000000002220, 14.46891108675447946, -66.48806413671076143 ) ) ;
#16018=CARTESIAN_POINT ( 'NONE',  ( -3.310556943750000425, 19.41135094264166838, -119.9349391362327992 ) ) ;
#16019=CYLINDRICAL_SURFACE ( 'NONE', #33619, 3.499999999999999556 ) ;
#16024=CARTESIAN_POINT ( 'NONE',  ( -1.655278471875002211, 14.63297358603754894, -99.59743913623280775 ) ) ;
#16025=CARTESIAN_POINT ( 'NONE',  ( -3.500000000000000000, 19.52072594216370760, -63.04431413575484555 ) ) ;
#16027=VERTEX_POINT ( 'NONE', #38891 ) ;
#16028=CYLINDRICAL_SURFACE ( 'NONE', #13158, 3.499999999999999556 ) ;
#16030=CARTESIAN_POINT ( 'NONE',  ( 1.749999999999998224, 14.46891108675447590, -48.32139747004410424 ) ) ;
#16031=CARTESIAN_POINT ( 'NONE',  ( 1.750000000000001110, 20.53108891324554719, -39.98806413671076854 ) ) ;
#16036=CARTESIAN_POINT ( 'NONE',  ( -3.310556943750000425, 19.41135094264166128, -36.84743913623281486 ) ) ;
#16041=CARTESIAN_POINT ( 'NONE',  ( -3.500000000000000000, 19.52072594216371115, -100.0443141357548313 ) ) ;
#16044=FACE_OUTER_BOUND ( 'NONE', #2157, .T. ) ;
#16046=CARTESIAN_POINT ( 'NONE',  ( 3.500000000000001332, 19.52072594216371826, -140.3776474690881741 ) ) ;
#16048=CARTESIAN_POINT ( 'NONE',  ( -1.750000000000002220, 14.46891108675448656, -116.4880641367107614 ) ) ;
#16050=CARTESIAN_POINT ( 'NONE',  ( -3.500000000000000888, 19.52072594216370405, -31.04431413575484200 ) ) ;
#16056=CARTESIAN_POINT ( 'NONE',  ( -1.750000000000002220, 14.46891108675449011, -140.7943141357548313 ) ) ;
#16058=CYLINDRICAL_SURFACE ( 'NONE', #32010, 3.499999999999999556 ) ;
#16059=CARTESIAN_POINT ( 'NONE',  ( -3.310556943750001313, 17.50000000000002132, -125.7641058028994792 ) ) ;
#16062=( BOUNDED_CURVE ( )  B_SPLINE_CURVE ( 2, ( #19629, #22622, #35599, #26244, #35385, #16664, #3467, #32808, #3678 ),
 .UNSPECIFIED., .F., .F. ) 
 B_SPLINE_CURVE_WITH_KNOTS ( ( 3, 2, 2, 2, 3 ),
 ( 0.9229166666666667185, 0.9236111111111111605, 0.9250000000000000444, 0.9263888888888889284, 0.9270833333333333703 ),
 .UNSPECIFIED. ) 
 CURVE ( )  GEOMETRIC_REPRESENTATION_ITEM ( )  RATIONAL_B_SPLINE_CURVE ( ( 0.9330127018922194093, 0.9330127018922194093, 1.000000000000000000, 0.8660254037844387076, 1.000000000000000000, 0.8660254037844387076, 1.000000000000000000, 0.9330127018922194093, 0.9330127018922194093 ) ) 
 REPRESENTATION_ITEM ( '' )  );
#16064=CARTESIAN_POINT ( 'NONE',  ( -1.749999999999999778, 20.53108891324555429, -89.12764746908817415 ) ) ;
#16065=CARTESIAN_POINT ( 'NONE',  ( 1.750000000000001110, 20.53108891324554719, -32.98806413671076854 ) ) ;
#16066=CARTESIAN_POINT ( 'NONE',  ( -3.310556943750000425, 19.41135094264166128, -60.84743913623280775 ) ) ;
#16067=CARTESIAN_POINT ( 'NONE',  ( -1.655278471875002211, 14.63297358603755072, -116.6849391362327850 ) ) ;
#16068=CARTESIAN_POINT ( 'NONE',  ( -1.750000000000002220, 14.46891108675447590, -33.48806413671076854 ) ) ;
#16069=CARTESIAN_POINT ( 'NONE',  ( 1.743066579297357930E-14, 14.00000000000002132, -135.7109808024214885 ) ) ;
#16071=CARTESIAN_POINT ( 'NONE',  ( -3.310556943750001313, 17.50000000000002487, -131.8516058028994564 ) ) ;
#16074=CARTESIAN_POINT ( 'NONE',  ( -3.310556943750002201, 15.58864905735836714, -41.76827246956612782 ) ) ;
#16075=CARTESIAN_POINT ( 'NONE',  ( 0.000000000000000000, 17.50000000000002487, -149.5231586289125687 ) ) ;
#16077=CARTESIAN_POINT ( 'NONE',  ( -3.310556943750000425, 19.41135094264166128, -66.93493913623279923 ) ) ;
#16079=CARTESIAN_POINT ( 'NONE',  ( 1.655278471874998436, 14.63297358603754184, -63.43077246956614346 ) ) ;
#16081=CARTESIAN_POINT ( 'NONE',  ( -1.655278471874999990, 20.36702641396249192, -85.01827246956612782 ) ) ;
#16082=EDGE_CURVE ( 'NONE', #632, #13712, #16716, .T. ) ;
#16087=CARTESIAN_POINT ( 'NONE',  ( -1.394453263437886604E-15, 14.00000000000000711, -23.71098080242150985 ) ) ;
#16088=CARTESIAN_POINT ( 'NONE',  ( 3.310556943750001313, 17.50000000000001421, -48.26410580289947205 ) ) ;
#16090=CARTESIAN_POINT ( 'NONE',  ( -3.310556943750000425, 19.41135094264166838, -105.8474391362327935 ) ) ;
#16091=CARTESIAN_POINT ( 'NONE',  ( 4.648177544792955347E-16, 21.00000000000001776, -95.90473080337744705 ) ) ;
#16095=ORIENTED_EDGE ( 'NONE', *, *, #28272, .F. ) ;
#16097=CARTESIAN_POINT ( 'NONE',  ( -3.310556943750002645, 15.58864905735836892, -58.68077246956613635 ) ) ;
#16099=FACE_OUTER_BOUND ( 'NONE', #4364, .T. ) ;
#16102=CARTESIAN_POINT ( 'NONE',  ( -3.500000000000001332, 17.50000000000002487, -140.6547308033774186 ) ) ;
#16103=VERTEX_POINT ( 'NONE', #16565 ) ;
#16104=CARTESIAN_POINT ( 'NONE',  ( -3.500000000000002220, 15.47927405783632082, -38.87764746908817415 ) ) ;
#16105=CARTESIAN_POINT ( 'NONE',  ( -3.310556943750002201, 15.58864905735837780, -124.6807724695661364 ) ) ;
#16106=CARTESIAN_POINT ( 'NONE',  ( 0.9378221735089281585, 14.00000000000001776, -94.66632260368297125 ) ) ;
#16108=CARTESIAN_POINT ( 'NONE',  ( -1.655278471874999990, 20.36702641396248481, -35.01827246956614204 ) ) ;
#16110=CARTESIAN_POINT ( 'NONE',  ( 2.340729813953370519E-16, 21.32270188528330479, -29.10160580289947063 ) ) ;
#16111=CARTESIAN_POINT ( 'NONE',  ( 3.310556943749999981, 15.58864905735836892, -87.43493913623278502 ) ) ;
#16112=CARTESIAN_POINT ( 'NONE',  ( 2.340729813953370519E-16, 21.32270188528332255, -140.0141058028994792 ) ) ;
#16115=CARTESIAN_POINT ( 'NONE',  ( -1.749999999999999778, 20.53108891324554719, -34.82139747004410424 ) ) ;
#16116=( BOUNDED_CURVE ( )  B_SPLINE_CURVE ( 2, ( #11280, #24264, #18283, #28064, #34449, #37234, #14692, #30638, #40211 ),
 .UNSPECIFIED., .F., .T. ) 
 B_SPLINE_CURVE_WITH_KNOTS ( ( 3, 2, 2, 2, 3 ),
 ( 0.9770833333333333037, 0.9777777777777777457, 0.9791666666666666297, 0.9805555555555555136, 0.9812499999999999556 ),
 .UNSPECIFIED. ) 
 CURVE ( )  GEOMETRIC_REPRESENTATION_ITEM ( )  RATIONAL_B_SPLINE_CURVE ( ( 0.9330127018922194093, 0.9330127018922194093, 1.000000000000000000, 0.8660254037844387076, 1.000000000000000000, 0.8660254037844387076, 1.000000000000000000, 0.9330127018922194093, 0.9330127018922194093 ) ) 
 REPRESENTATION_ITEM ( '' )  );
#16117=CARTESIAN_POINT ( 'NONE',  ( 1.655278471875001101, 20.36702641396249902, -135.1849391362327992 ) ) ;
#16122=CARTESIAN_POINT ( 'NONE',  ( -3.500000000000002220, 15.47927405783632793, -81.57139747004410424 ) ) ;
#16123=EDGE_CURVE ( 'NONE', #35835, #34390, #21305, .T. ) ;
#16124=CARTESIAN_POINT ( 'NONE',  ( -1.655278471874999990, 20.36702641396248836, -57.01827246956612782 ) ) ;
#16126=DIRECTION ( 'NONE',  ( -0.000000000000000000, 1.259100132267607459E-16, -1.000000000000000000 ) ) ;
#16128=CARTESIAN_POINT ( 'NONE',  ( 2.340729813953370519E-16, 21.32270188528331190, -86.10160580289948484 ) ) ;
#16129=CARTESIAN_POINT ( 'NONE',  ( -1.394453263437886604E-15, 14.00000000000001421, -77.40473080337740441 ) ) ;
#16130=CARTESIAN_POINT ( 'NONE',  ( 1.655278471875001101, 20.36702641396249547, -115.0974391362327935 ) ) ;
#16131=CARTESIAN_POINT ( 'NONE',  ( -3.310556943750002645, 15.58864905735837070, -78.68077246956613635 ) ) ;
#16134=CARTESIAN_POINT ( 'NONE',  ( -3.500000000000000888, 19.52072594216371826, -107.7380641367107756 ) ) ;
#16142=CARTESIAN_POINT ( 'NONE',  ( 1.655278471874998436, 14.63297358603754361, -68.43077246956613635 ) ) ;
#16144=CARTESIAN_POINT ( 'NONE',  ( 3.310556943749999981, 15.58864905735837247, -122.3474391362328362 ) ) ;
#16145=DIRECTION ( 'NONE',  ( -0.000000000000000000, 1.259100132267607459E-16, -1.000000000000000000 ) ) ;
#16148=LINE ( 'NONE', #35893, #17849 ) ;
#16150=CARTESIAN_POINT ( 'NONE',  ( 1.655278471875001101, 20.36702641396249192, -75.09743913623280775 ) ) ;
#16151=EDGE_LOOP ( 'NONE', ( #23662, #18678, #9331, #16912 ) ) ;
#16155=CARTESIAN_POINT ( 'NONE',  ( 3.310556943750001313, 19.41135094264167549, -143.1807724695661364 ) ) ;
#16156=CARTESIAN_POINT ( 'NONE',  ( -3.500000000000000000, 19.52072594216370760, -51.73806413671076854 ) ) ;
#16157=LINE ( 'NONE', #19325, #36333 ) ;
#16158=CARTESIAN_POINT ( 'NONE',  ( 2.340729813953370519E-16, 21.32270188528330479, -45.10160580289947063 ) ) ;
#16159=CARTESIAN_POINT ( 'NONE',  ( -3.310556943750002645, 15.58864905735837425, -103.7682724695661278 ) ) ;
#16160=CARTESIAN_POINT ( 'NONE',  ( -3.310556943750000425, 19.41135094264165772, -31.84743913623280420 ) ) ;
#16162=CARTESIAN_POINT ( 'NONE',  ( -7.424026671074350129E-16, 13.45854811567263987, -109.7109808024215027 ) ) ;
#16165=CARTESIAN_POINT ( 'NONE',  ( -3.500000000000000888, 19.52072594216371115, -98.73806413671077564 ) ) ;
#16170=CARTESIAN_POINT ( 'NONE',  ( -3.500000000000002220, 15.47927405783632437, -60.87764746908817415 ) ) ;
#16171=CARTESIAN_POINT ( 'NONE',  ( -3.500000000000001332, 17.50000000000001066, -46.96098080242150274 ) ) ;
#16172=CARTESIAN_POINT ( 'NONE',  ( 3.500000000000001776, 19.52072594216370405, -46.07139747004409713 ) ) ;
#16173=CARTESIAN_POINT ( 'NONE',  ( 0.9378221735089281585, 14.00000000000002132, -106.6663226036829855 ) ) ;
#16174=CARTESIAN_POINT ( 'NONE',  ( 1.655278471874998436, 14.63297358603753828, -30.51827246956613493 ) ) ;
#16176=CARTESIAN_POINT ( 'NONE',  ( 4.648177544792955347E-16, 21.00000000000001421, -65.90473080337741862 ) ) ;
#16181=CARTESIAN_POINT ( 'NONE',  ( -3.310556943750002201, 15.58864905735837247, -83.68077246956615056 ) ) ;
#16182=CYLINDRICAL_SURFACE ( 'NONE', #11768, 3.499999999999999556 ) ;
#16183=ORIENTED_EDGE ( 'NONE', *, *, #24192, .T. ) ;
#16184=CARTESIAN_POINT ( 'NONE',  ( 3.500000000000000000, 15.47927405783632082, -34.23806413671076854 ) ) ;
#16185=VERTEX_POINT ( 'NONE', #14923 ) ;
#16188=CARTESIAN_POINT ( 'NONE',  ( -7.022189441860112050E-16, 13.67729811471672363, -90.51410580289946495 ) ) ;
#16190=DIRECTION ( 'NONE',  ( 0.000000000000000000, 1.000000000000000000, 0.000000000000000000 ) ) ;
#16191=ORIENTED_EDGE ( 'NONE', *, *, #24575, .F. ) ;
#16195=FACE_OUTER_BOUND ( 'NONE', #28980, .T. ) ;
#16196=CARTESIAN_POINT ( 'NONE',  ( 1.655278471874998436, 14.63297358603755072, -131.4307724695661364 ) ) ;
#16199=CARTESIAN_POINT ( 'NONE',  ( -1.655278471874999990, 20.36702641396249547, -121.0182724695661278 ) ) ;
#16200=CARTESIAN_POINT ( 'NONE',  ( -1.655278471874999990, 20.36702641396248836, -52.01827246956612782 ) ) ;
#16201=ORIENTED_EDGE ( 'NONE', *, *, #39427, .F. ) ;
#16202=CARTESIAN_POINT ( 'NONE',  ( 2.474675557024783212E-16, 21.54145188432740099, -128.9047308033774470 ) ) ;
#16203=CARTESIAN_POINT ( 'NONE',  ( 1.655278471875001101, 20.36702641396248836, -73.18493913623279923 ) ) ;
#16204=CARTESIAN_POINT ( 'NONE',  ( 3.500000000000001332, 17.50000000000002132, -123.4609808024215027 ) ) ;
#16205=CARTESIAN_POINT ( 'NONE',  ( -3.310556943750001313, 17.50000000000002132, -109.7641058028994649 ) ) ;
#16206=CARTESIAN_POINT ( 'NONE',  ( 3.500000000000001332, 17.50000000000001776, -81.15473080337743284 ) ) ;
#16208=CARTESIAN_POINT ( 'NONE',  ( 1.749999999999998224, 14.46891108675447946, -76.62764746908817415 ) ) ;
#16209=CARTESIAN_POINT ( 'NONE',  ( -1.750000000000002220, 14.46891108675447768, -50.79431413575484555 ) ) ;
#16210=CARTESIAN_POINT ( 'NONE',  ( 1.655278471874998436, 14.63297358603754006, -42.43077246956614346 ) ) ;
#16211=CARTESIAN_POINT ( 'NONE',  ( 3.310556943750001313, 17.50000000000001776, -96.35160580289945642 ) ) ;
#16212=CARTESIAN_POINT ( 'NONE',  ( 0.9378221735089281585, 14.00000000000001599, -73.66632260368299967 ) ) ;
#16213=CARTESIAN_POINT ( 'NONE',  ( -1.750000000000002220, 14.46891108675447946, -62.48806413671076143 ) ) ;
#16214=DIRECTION ( 'NONE',  ( -0.000000000000000000, 1.259100132267607459E-16, -1.000000000000000000 ) ) ;
#16216=CARTESIAN_POINT ( 'NONE',  ( 3.310556943749999981, 15.58864905735837247, -120.4349391362327992 ) ) ;
#16222=CARTESIAN_POINT ( 'NONE',  ( 3.310556943750001313, 19.41135094264166838, -99.18077246956613635 ) ) ;
#16228=EDGE_CURVE ( 'NONE', #25797, #13141, #11512, .T. ) ;
#16229=CARTESIAN_POINT ( 'NONE',  ( 4.648177544792955347E-16, 21.00000000000002132, -127.2109808024214885 ) ) ;
#16230=( BOUNDED_CURVE ( )  B_SPLINE_CURVE ( 2, ( #63, #9433, #32188, #26023, #16656, #6241, #41561, #23026, #35995 ),
 .UNSPECIFIED., .F., .F. ) 
 B_SPLINE_CURVE_WITH_KNOTS ( ( 3, 2, 2, 2, 3 ),
 ( 0.2354166666666666630, 0.2361111111111111049, 0.2374999999999999889, 0.2388888888888889006, 0.2395833333333333426 ),
 .UNSPECIFIED. ) 
 CURVE ( )  GEOMETRIC_REPRESENTATION_ITEM ( )  RATIONAL_B_SPLINE_CURVE ( ( 0.9330127018922194093, 0.9330127018922194093, 1.000000000000000000, 0.8660254037844387076, 1.000000000000000000, 0.8660254037844387076, 1.000000000000000000, 0.9330127018922194093, 0.9330127018922194093 ) ) 
 REPRESENTATION_ITEM ( '' )  );
#16231=CARTESIAN_POINT ( 'NONE',  ( -1.750000000000002220, 14.46891108675448123, -70.79431413575483134 ) ) ;
#16235=CARTESIAN_POINT ( 'NONE',  ( -7.022189441860112050E-16, 13.67729811471671653, -36.51410580289947205 ) ) ;
#16242=CARTESIAN_POINT ( 'NONE',  ( -0.9378221735089310451, 14.00000000000001066, -37.44938900211595012 ) ) ;
#16244=CARTESIAN_POINT ( 'NONE',  ( -0.9378221735089310451, 14.00000000000002309, -119.4493890021159501 ) ) ;
#16245=CARTESIAN_POINT ( 'NONE',  ( -3.500000000000002220, 15.47927405783633503, -119.5713974700440900 ) ) ;
#16247=CARTESIAN_POINT ( 'NONE',  ( 3.310556943749999981, 15.58864905735837425, -135.4349391362327992 ) ) ;
#16248=CARTESIAN_POINT ( 'NONE',  ( 3.500000000000000000, 15.47927405783632082, -34.54431413575484555 ) ) ;
#16251=DIRECTION ( 'NONE',  ( -0.000000000000000000, 1.259100132267607459E-16, -1.000000000000000000 ) ) ;
#16252=VECTOR ( 'NONE', #33352, 1000.000000000000000 ) ;
#16254=CARTESIAN_POINT ( 'NONE',  ( 1.749999999999998224, 14.46891108675448478, -118.6276474690881741 ) ) ;
#16256=CARTESIAN_POINT ( 'NONE',  ( 2.474675557024783212E-16, 21.54145188432740810, -140.2109808024215170 ) ) ;
#16257=CARTESIAN_POINT ( 'NONE',  ( 1.655278471875001101, 20.36702641396249547, -121.0974391362328078 ) ) ;
#16259=EDGE_LOOP ( 'NONE', ( #11151, #22761, #21608, #26962 ) ) ;
#16261=CARTESIAN_POINT ( 'NONE',  ( -3.500000000000001332, 17.50000000000001776, -81.96098080242150274 ) ) ;
#16262=CARTESIAN_POINT ( 'NONE',  ( 1.750000000000001110, 20.53108891324555429, -92.29431413575484555 ) ) ;
#16264=CARTESIAN_POINT ( 'NONE',  ( 3.310556943749999981, 15.58864905735836537, -61.34743913623280775 ) ) ;
#16265=CARTESIAN_POINT ( 'NONE',  ( -1.655278471874999990, 20.36702641396249547, -119.0182724695661278 ) ) ;
#16266=CARTESIAN_POINT ( 'NONE',  ( -3.500000000000000000, 19.52072594216371826, -122.0443141357548456 ) ) ;
#16267=CARTESIAN_POINT ( 'NONE',  ( -3.500000000000001332, 17.50000000000001066, -30.65473080337742573 ) ) ;
#16268=CARTESIAN_POINT ( 'NONE',  ( -1.394453263437886604E-15, 14.00000000000002132, -121.4047308033774328 ) ) ;
#16270=CARTESIAN_POINT ( 'NONE',  ( 3.310556943749999981, 15.58864905735837425, -134.4349391362327992 ) ) ;
#16272=CARTESIAN_POINT ( 'NONE',  ( 4.648177544792955347E-16, 21.00000000000002132, -112.9047308033774186 ) ) ;
#16274=CARTESIAN_POINT ( 'NONE',  ( 2.340729813953370519E-16, 21.32270188528330834, -68.10160580289945642 ) ) ;
#16276=CARTESIAN_POINT ( 'NONE',  ( -1.655278471875002211, 14.63297358603754539, -67.59743913623280775 ) ) ;
#16277=EDGE_LOOP ( 'NONE', ( #30659, #27331, #23041, #40561 ) ) ;
#16279=CARTESIAN_POINT ( 'NONE',  ( -3.310556943750002201, 15.58864905735837247, -85.76827246956612782 ) ) ;
#16282=CARTESIAN_POINT ( 'NONE',  ( 0.000000000000000000, 21.00000000000002487, -149.5231586289125687 ) ) ;
#16283=CARTESIAN_POINT ( 'NONE',  ( 2.340729813953370519E-16, 21.32270188528331190, -51.01410580289947205 ) ) ;
#16285=CARTESIAN_POINT ( 'NONE',  ( -1.655278471875002211, 14.63297358603754894, -105.5974391362328078 ) ) ;
#16286=FACE_OUTER_BOUND ( 'NONE', #35488, .T. ) ;
#16288=EDGE_LOOP ( 'NONE', ( #28823, #6858, #28406, #30351 ) ) ;
#16293=CARTESIAN_POINT ( 'NONE',  ( 3.310556943750001313, 17.50000000000001421, -56.26410580289947916 ) ) ;
#16296=DIRECTION ( 'NONE',  ( 0.000000000000000000, -0.000000000000000000, -1.000000000000000000 ) ) ;
#16297=AXIS2_PLACEMENT_3D ( 'NONE', #40172, #37199, #21027 ) ;
#16300=CARTESIAN_POINT ( 'NONE',  ( 3.500000000000000000, 15.47927405783632082, -47.23806413671076143 ) ) ;
#16301=ORIENTED_EDGE ( 'NONE', *, *, #4527, .F. ) ;
#16302=EDGE_CURVE ( 'NONE', #3414, #30668, #18531, .T. ) ;
#16303=( BOUNDED_CURVE ( )  B_SPLINE_CURVE ( 2, ( #40098, #24164, #23952, #38792, #3065, #5627, #35389, #18809, #31769 ),
 .UNSPECIFIED., .F., .T. ) 
 B_SPLINE_CURVE_WITH_KNOTS ( ( 3, 2, 2, 2, 3 ),
 ( 0.7520833333333333259, 0.7527777777777777679, 0.7541666666666666519, 0.7555555555555555358, 0.7562499999999999778 ),
 .UNSPECIFIED. ) 
 CURVE ( )  GEOMETRIC_REPRESENTATION_ITEM ( )  RATIONAL_B_SPLINE_CURVE ( ( 0.9330127018922194093, 0.9330127018922194093, 1.000000000000000000, 0.8660254037844387076, 1.000000000000000000, 0.8660254037844387076, 1.000000000000000000, 0.9330127018922194093, 0.9330127018922194093 ) ) 
 REPRESENTATION_ITEM ( '' )  );
#16304=CARTESIAN_POINT ( 'NONE',  ( 4.286263797015737581E-16, 14.00000000000002487, -149.5231586289125687 ) ) ;
#16305=CARTESIAN_POINT ( 'NONE',  ( 1.655278471875001101, 20.36702641396249547, -126.0974391362328078 ) ) ;
#16306=LINE ( 'NONE', #3730, #33221 ) ;
#16309=CARTESIAN_POINT ( 'NONE',  ( 3.310556943750001313, 19.41135094264165772, -35.26827246956613493 ) ) ;
#16310=CARTESIAN_POINT ( 'NONE',  ( 1.655278471875001101, 20.36702641396248481, -28.18493913623279568 ) ) ;
#16311=CARTESIAN_POINT ( 'NONE',  ( 1.655278471875001101, 20.36702641396249192, -90.18493913623279923 ) ) ;
#16312=CARTESIAN_POINT ( 'NONE',  ( -3.310556943750001313, 17.50000000000002487, -140.7641058028994792 ) ) ;
#16314=CARTESIAN_POINT ( 'NONE',  ( 3.500000000000001332, 17.50000000000002132, -127.1547308033774186 ) ) ;
#16315=CARTESIAN_POINT ( 'NONE',  ( 4.648177544792955347E-16, 21.00000000000001776, -98.21098080242148853 ) ) ;
#16317=CARTESIAN_POINT ( 'NONE',  ( -3.310556943750000425, 19.41135094264167549, -131.9349391362328277 ) ) ;
#16318=CARTESIAN_POINT ( 'NONE',  ( -1.655278471874999990, 20.36702641396249192, -90.93077246956613635 ) ) ;
#16320=CARTESIAN_POINT ( 'NONE',  ( -3.500000000000002220, 15.47927405783633503, -125.8776474690881599 ) ) ;
#16322=CARTESIAN_POINT ( 'NONE',  ( -1.750000000000002220, 14.46891108675448123, -77.48806413671076143 ) ) ;
#16323=CARTESIAN_POINT ( 'NONE',  ( -1.655278471875002211, 14.63297358603754361, -61.68493913623279923 ) ) ;
#16326=CARTESIAN_POINT ( 'NONE',  ( 4.648177544792955347E-16, 21.00000000000001066, -41.21098080242150274 ) ) ;
#16327=CARTESIAN_POINT ( 'NONE',  ( -3.310556943750002645, 15.58864905735837247, -84.76827246956612782 ) ) ;
#16328=CARTESIAN_POINT ( 'NONE',  ( -3.310556943750002645, 15.58864905735837958, -142.7682724695661420 ) ) ;
#16329=CARTESIAN_POINT ( 'NONE',  ( -3.310556943750000425, 19.41135094264166838, -113.8474391362327935 ) ) ;
#16330=CARTESIAN_POINT ( 'NONE',  ( -3.310556943750000425, 19.41135094264166483, -80.84743913623280775 ) ) ;
#16331=CARTESIAN_POINT ( 'NONE',  ( 1.750000000000001110, 20.53108891324556140, -138.2943141357548313 ) ) ;
#16332=ORIENTED_EDGE ( 'NONE', *, *, #15188, .F. ) ;
#16333=VECTOR ( 'NONE', #12136, 1000.000000000000000 ) ;
#16334=CARTESIAN_POINT ( 'NONE',  ( -1.655278471875002211, 14.63297358603754894, -101.6849391362327992 ) ) ;
#16335=CARTESIAN_POINT ( 'NONE',  ( 3.500000000000001332, 17.50000000000002132, -104.1547308033774186 ) ) ;
#16337=CARTESIAN_POINT ( 'NONE',  ( -1.749999999999999778, 20.53108891324555429, -94.82139747004409003 ) ) ;
#16338=CARTESIAN_POINT ( 'NONE',  ( 4.648177544792955347E-16, 21.00000000000001066, -43.90473080337743284 ) ) ;
#16341=CARTESIAN_POINT ( 'NONE',  ( 3.310556943750001313, 19.41135094264166483, -68.18077246956613635 ) ) ;
#16342=CARTESIAN_POINT ( 'NONE',  ( -0.9378221735089291577, 21.00000000000001066, -30.16632260368299612 ) ) ;
#16343=CARTESIAN_POINT ( 'NONE',  ( -3.310556943750002645, 15.58864905735837780, -121.6807724695661364 ) ) ;
#16346=ORIENTED_EDGE ( 'NONE', *, *, #31920, .T. ) ;
#16348=CARTESIAN_POINT ( 'NONE',  ( 0.9378221735089300459, 21.00000000000001776, -99.25563900116003424 ) ) ;
#16350=CARTESIAN_POINT ( 'NONE',  ( -3.310556943750002645, 15.58864905735837070, -75.68077246956613635 ) ) ;
#16351=ORIENTED_EDGE ( 'NONE', *, *, #15434, .T. ) ;
#16353=AXIS2_PLACEMENT_3D ( 'NONE', #35621, #23265, #22851 ) ;
#16355=ADVANCED_FACE ( 'NONE', ( #41083 ), #1744, .T. ) ;
#16356=CARTESIAN_POINT ( 'NONE',  ( -1.655278471874999990, 20.36702641396249902, -140.9307724695661364 ) ) ;
#16357=CARTESIAN_POINT ( 'NONE',  ( -0.9378221735089291577, 21.00000000000001421, -51.86007260463890844 ) ) ;
#16358=( BOUNDED_CURVE ( )  B_SPLINE_CURVE ( 2, ( #5177, #14760, #21340, #24331, #1973, #27716, #1360, #23916, #30704 ),
 .UNSPECIFIED., .F., .T. ) 
 B_SPLINE_CURVE_WITH_KNOTS ( ( 3, 2, 2, 2, 3 ),
 ( 0.9645833333333333481, 0.9652777777777777901, 0.9666666666666666741, 0.9680555555555555580, 0.9687500000000000000 ),
 .UNSPECIFIED. ) 
 CURVE ( )  GEOMETRIC_REPRESENTATION_ITEM ( )  RATIONAL_B_SPLINE_CURVE ( ( 0.9330127018922194093, 0.9330127018922194093, 1.000000000000000000, 0.8660254037844387076, 1.000000000000000000, 0.8660254037844387076, 1.000000000000000000, 0.9330127018922194093, 0.9330127018922194093 ) ) 
 REPRESENTATION_ITEM ( '' )  );
#16359=VECTOR ( 'NONE', #18593, 1000.000000000000000 ) ;
#16360=CARTESIAN_POINT ( 'NONE',  ( 0.9378221735089300459, 21.00000000000001066, -40.94938900211595723 ) ) ;
#16361=CARTESIAN_POINT ( 'NONE',  ( -1.655278471874999990, 20.36702641396248481, -44.01827246956613493 ) ) ;
#16362=CARTESIAN_POINT ( 'NONE',  ( -7.022189441860112050E-16, 13.67729811471672541, -101.6016058028994706 ) ) ;
#16363=CARTESIAN_POINT ( 'NONE',  ( -3.310556943750001313, 17.50000000000001066, -27.76410580289947916 ) ) ;
#16365=CARTESIAN_POINT ( 'NONE',  ( -3.500000000000002220, 15.47927405783632970, -100.8776474690881599 ) ) ;
#16368=CARTESIAN_POINT ( 'NONE',  ( -1.749999999999999778, 20.53108891324555429, -88.82139747004410424 ) ) ;
#16370=CARTESIAN_POINT ( 'NONE',  ( -3.695301148110399846E-14, 21.00000000000002132, -124.2109808024214885 ) ) ;
#16373=CARTESIAN_POINT ( 'NONE',  ( 2.474675557024783212E-16, 21.54145188432739388, -59.21098080242150985 ) ) ;
#16374=AXIS2_PLACEMENT_3D ( 'NONE', #722, #33474, #30282 ) ;
#16376=CARTESIAN_POINT ( 'NONE',  ( 4.648177544792955347E-16, 21.00000000000001066, -25.21098080242150985 ) ) ;
#16377=CARTESIAN_POINT ( 'NONE',  ( -3.500000000000000888, 19.52072594216370760, -47.73806413671076143 ) ) ;
#16379=CARTESIAN_POINT ( 'NONE',  ( -7.022189441860112050E-16, 13.67729811471671653, -26.60160580289946708 ) ) ;
#16381=CARTESIAN_POINT ( 'NONE',  ( -1.394453263437886604E-15, 14.00000000000001421, -75.40473080337740441 ) ) ;
#16386=CARTESIAN_POINT ( 'NONE',  ( -1.655278471874999990, 20.36702641396249192, -84.93077246956613635 ) ) ;
#16387=CARTESIAN_POINT ( 'NONE',  ( 0.9378221735089300459, 21.00000000000001421, -52.25563900116002714 ) ) ;
#16390=CARTESIAN_POINT ( 'NONE',  ( 4.648177544792955347E-16, 21.00000000000002132, -105.2109808024215027 ) ) ;
#16391=VERTEX_POINT ( 'NONE', #37679 ) ;
#16392=CARTESIAN_POINT ( 'NONE',  ( -1.394453263437886604E-15, 14.00000000000001776, -87.71098080242151696 ) ) ;
#16393=CARTESIAN_POINT ( 'NONE',  ( 2.340729813953370519E-16, 21.32270188528331190, -91.01410580289947916 ) ) ;
#16396=ORIENTED_EDGE ( 'NONE', *, *, #41780, .F. ) ;
#16399=CARTESIAN_POINT ( 'NONE',  ( -0.9378221735089310451, 14.00000000000002132, -84.44938900211595012 ) ) ;
#16402=CARTESIAN_POINT ( 'NONE',  ( -1.394453263437886604E-15, 14.00000000000001776, -88.40473080337740441 ) ) ;
#16403=CARTESIAN_POINT ( 'NONE',  ( 3.310556943750001313, 17.50000000000001066, -23.26410580289947561 ) ) ;
#16404=CARTESIAN_POINT ( 'NONE',  ( 3.310556943750001313, 17.50000000000002487, -133.2641058028994507 ) ) ;
#16405=EDGE_LOOP ( 'NONE', ( #20584, #39344, #3613, #4572 ) ) ;
#16406=ORIENTED_EDGE ( 'NONE', *, *, #22724, .F. ) ;
#16407=CARTESIAN_POINT ( 'NONE',  ( 3.500000000000000000, 15.47927405783632615, -73.23806413671077564 ) ) ;
#16408=CARTESIAN_POINT ( 'NONE',  ( 3.310556943750001313, 17.50000000000002132, -119.3516058028994706 ) ) ;
#16409=VERTEX_POINT ( 'NONE', #34690 ) ;
#16410=EDGE_LOOP ( 'NONE', ( #35074, #19949, #41250, #7773 ) ) ;
#16411=CARTESIAN_POINT ( 'NONE',  ( 1.750000000000001110, 20.53108891324556140, -129.9880641367107614 ) ) ;
#16413=CARTESIAN_POINT ( 'NONE',  ( 1.655278471874998436, 14.63297358603754361, -74.51827246956612782 ) ) ;
#16414=CARTESIAN_POINT ( 'NONE',  ( -3.500000000000001332, 17.50000000000002132, -120.9609808024215170 ) ) ;
#16415=CARTESIAN_POINT ( 'NONE',  ( 1.655278471874998436, 14.63297358603754716, -101.4307724695661364 ) ) ;
#16419=CARTESIAN_POINT ( 'NONE',  ( 3.500000000000000000, 15.47927405783632437, -73.54431413575484555 ) ) ;
#16420=CARTESIAN_POINT ( 'NONE',  ( 1.750000000000001110, 20.53108891324555785, -125.9880641367107614 ) ) ;
#16421=CARTESIAN_POINT ( 'NONE',  ( -3.310556943750002645, 15.58864905735836537, -37.68077246956613635 ) ) ;
#16422=CARTESIAN_POINT ( 'NONE',  ( -1.655278471875002211, 14.63297358603754894, -98.68493913623279923 ) ) ;
#16423=CARTESIAN_POINT ( 'NONE',  ( -3.500000000000000888, 19.52072594216370760, -63.73806413671076143 ) ) ;
#16425=CARTESIAN_POINT ( 'NONE',  ( -3.310556943750001313, 17.50000000000002132, -117.8516058028994706 ) ) ;
#16426=CARTESIAN_POINT ( 'NONE',  ( -8.715332896486792803E-15, 21.00000000000002842, -136.9047308033774470 ) ) ;
#16431=CARTESIAN_POINT ( 'NONE',  ( -3.310556943750000425, 19.41135094264166838, -96.84743913623282197 ) ) ;
#16440=CARTESIAN_POINT ( 'NONE',  ( -3.310556943750002201, 15.58864905735836537, -26.68077246956613635 ) ) ;
#16442=CARTESIAN_POINT ( 'NONE',  ( -3.500000000000000000, 19.52072594216371826, -123.7380641367107614 ) ) ;
#16446=CARTESIAN_POINT ( 'NONE',  ( -0.9378221735089291577, 21.00000000000001421, -58.16632260368298546 ) ) ;
#16447=VERTEX_POINT ( 'NONE', #14516 ) ;
#16448=CARTESIAN_POINT ( 'NONE',  ( 4.648177544792955347E-16, 21.00000000000001066, -37.90473080337743284 ) ) ;
#16450=CARTESIAN_POINT ( 'NONE',  ( -1.394453263437886604E-15, 14.00000000000001776, -81.71098080242150274 ) ) ;
#16451=CARTESIAN_POINT ( 'NONE',  ( -7.424026671074350129E-16, 13.45854811567263987, -119.4047308033774328 ) ) ;
#16454=CARTESIAN_POINT ( 'NONE',  ( -1.655278471874999990, 20.36702641396249902, -133.0182724695661420 ) ) ;
#16455=CARTESIAN_POINT ( 'NONE',  ( 3.500000000000000000, 15.47927405783632082, -32.54431413575484555 ) ) ;
#16459=CARTESIAN_POINT ( 'NONE',  ( -1.750000000000002220, 14.46891108675447946, -65.48806413671076143 ) ) ;
#16461=CARTESIAN_POINT ( 'NONE',  ( 2.474675557024783212E-16, 21.54145188432740810, -137.2109808024214885 ) ) ;
#16462=CARTESIAN_POINT ( 'NONE',  ( -3.310556943750000425, 19.41135094264166838, -120.8474391362327935 ) ) ;
#16465=DIRECTION ( 'NONE',  ( -0.000000000000000000, 1.259100132267607459E-16, -1.000000000000000000 ) ) ;
#16466=CARTESIAN_POINT ( 'NONE',  ( 1.750000000000001110, 20.53108891324555429, -93.29431413575484555 ) ) ;
#16467=( BOUNDED_CURVE ( )  B_SPLINE_CURVE ( 2, ( #6916, #33069, #39237, #26080, #16917, #19480, #26494, #38834, #13096 ),
 .UNSPECIFIED., .F., .T. ) 
 B_SPLINE_CURVE_WITH_KNOTS ( ( 3, 2, 2, 2, 3 ),
 ( 0.2395833333333333426, 0.2402777777777777846, 0.2416666666666666685, 0.2430555555555555525, 0.2437499999999999944 ),
 .UNSPECIFIED. ) 
 CURVE ( )  GEOMETRIC_REPRESENTATION_ITEM ( )  RATIONAL_B_SPLINE_CURVE ( ( 0.9330127018922194093, 0.9330127018922194093, 1.000000000000000000, 0.8660254037844387076, 1.000000000000000000, 0.8660254037844387076, 1.000000000000000000, 0.9330127018922194093, 0.9330127018922194093 ) ) 
 REPRESENTATION_ITEM ( '' )  );
#16468=CARTESIAN_POINT ( 'NONE',  ( -3.500000000000001332, 17.50000000000001066, -36.96098080242150985 ) ) ;
#16469=CARTESIAN_POINT ( 'NONE',  ( 1.655278471875001101, 20.36702641396248836, -51.09743913623280775 ) ) ;
#16470=CARTESIAN_POINT ( 'NONE',  ( 3.310556943749999981, 15.58864905735837247, -112.4349391362327992 ) ) ;
#16471=CARTESIAN_POINT ( 'NONE',  ( 0.000000000000000000, 17.50000000000002487, -149.5231586289125687 ) ) ;
#16472=CARTESIAN_POINT ( 'NONE',  ( 3.500000000000000000, 15.47927405783632082, -33.23806413671076854 ) ) ;
#16475=CARTESIAN_POINT ( 'NONE',  ( 3.310556943750001313, 19.41135094264167549, -132.2682724695661420 ) ) ;
#16477=CARTESIAN_POINT ( 'NONE',  ( 3.500000000000001332, 19.52072594216371826, -138.0713974700441042 ) ) ;
#16479=CARTESIAN_POINT ( 'NONE',  ( -7.022189441860112050E-16, 13.67729811471671830, -62.60160580289946353 ) ) ;
#16481=CARTESIAN_POINT ( 'NONE',  ( 2.340729813953370519E-16, 21.32270188528330834, -63.01410580289947205 ) ) ;
#16483=CARTESIAN_POINT ( 'NONE',  ( 3.310556943749999981, 15.58864905735836892, -86.43493913623278502 ) ) ;
#16486=CARTESIAN_POINT ( 'NONE',  ( -3.500000000000000000, 19.52072594216371826, -103.7380641367107756 ) ) ;
#16488=CARTESIAN_POINT ( 'NONE',  ( -1.655278471875002211, 14.63297358603754184, -42.59743913623280065 ) ) ;
#16489=EDGE_CURVE ( 'NONE', #34385, #18226, #21098, .T. ) ;
#16492=CARTESIAN_POINT ( 'NONE',  ( 3.310556943750001313, 17.50000000000002132, -105.2641058028994649 ) ) ;
#16494=VERTEX_POINT ( 'NONE', #9378 ) ;
#16497=ORIENTED_EDGE ( 'NONE', *, *, #25985, .T. ) ;
#16499=CARTESIAN_POINT ( 'NONE',  ( 1.655278471874998436, 14.63297358603754184, -59.43077246956614346 ) ) ;
#16500=EDGE_LOOP ( 'NONE', ( #11633, #31656, #25755, #32791 ) ) ;
#16501=ORIENTED_EDGE ( 'NONE', *, *, #15825, .F. ) ;
#16502=CARTESIAN_POINT ( 'NONE',  ( 0.9378221735089281585, 14.00000000000001599, -76.66632260368297125 ) ) ;
#16503=CARTESIAN_POINT ( 'NONE',  ( 3.500000000000001332, 17.50000000000001421, -55.46098080242150985 ) ) ;
#16506=CARTESIAN_POINT ( 'NONE',  ( 3.500000000000001332, 17.50000000000001421, -47.15473080337742573 ) ) ;
#16508=CARTESIAN_POINT ( 'NONE',  ( 0.9378221735089300459, 21.00000000000001066, -34.94938900211595012 ) ) ;
#16509=CARTESIAN_POINT ( 'NONE',  ( -7.022189441860112050E-16, 13.67729811471672896, -124.5141058028994507 ) ) ;
#16510=EDGE_CURVE ( 'NONE', #12464, #20461, #23811, .T. ) ;
#16511=CARTESIAN_POINT ( 'NONE',  ( 1.749999999999998224, 14.46891108675448656, -125.6276474690881599 ) ) ;
#16514=CARTESIAN_POINT ( 'NONE',  ( 2.340729813953370519E-16, 21.32270188528330479, -37.10160580289946353 ) ) ;
#16516=AXIS2_PLACEMENT_3D ( 'NONE', #30225, #27462, #20869 ) ;
#16517=CARTESIAN_POINT ( 'NONE',  ( -1.655278471875002211, 14.63297358603754716, -87.68493913623279923 ) ) ;
#16518=CARTESIAN_POINT ( 'NONE',  ( -3.310556943750000425, 19.41135094264167549, -141.8474391362327935 ) ) ;
#16524=CARTESIAN_POINT ( 'NONE',  ( 1.655278471875001101, 20.36702641396249547, -128.1849391362327992 ) ) ;
#16525=DIRECTION ( 'NONE',  ( -0.000000000000000000, 1.259100132267607459E-16, -1.000000000000000000 ) ) ;
#16526=CARTESIAN_POINT ( 'NONE',  ( 3.310556943750001313, 19.41135094264166483, -91.18077246956613635 ) ) ;
#16529=CARTESIAN_POINT ( 'NONE',  ( -1.749999999999999778, 20.53108891324555429, -76.82139747004410424 ) ) ;
#16530=CARTESIAN_POINT ( 'NONE',  ( 3.310556943750001313, 19.41135094264166483, -60.26827246956613493 ) ) ;
#16533=DIRECTION ( 'NONE',  ( -0.000000000000000000, 1.259100132267607459E-16, -1.000000000000000000 ) ) ;
#16534=CARTESIAN_POINT ( 'NONE',  ( 2.340729813953370519E-16, 21.32270188528331190, -85.10160580289947063 ) ) ;
#16535=FACE_OUTER_BOUND ( 'NONE', #41559, .T. ) ;
#16537=CARTESIAN_POINT ( 'NONE',  ( 3.310556943750001313, 17.50000000000002132, -111.2641058028994649 ) ) ;
#16538=CARTESIAN_POINT ( 'NONE',  ( -7.022189441860112050E-16, 13.67729811471672363, -81.51410580289946495 ) ) ;
#16540=ORIENTED_EDGE ( 'NONE', *, *, #34938, .F. ) ;
#16541=CARTESIAN_POINT ( 'NONE',  ( -7.022189441860112050E-16, 13.67729811471672541, -103.6016058028994564 ) ) ;
#16542=CARTESIAN_POINT ( 'NONE',  ( -3.500000000000001332, 17.50000000000001776, -100.6547308033774328 ) ) ;
#16548=CARTESIAN_POINT ( 'NONE',  ( 3.310556943750001313, 19.41135094264166483, -64.18077246956615056 ) ) ;
#16549=CARTESIAN_POINT ( 'NONE',  ( -1.750000000000002220, 14.46891108675447590, -29.79431413575483845 ) ) ;
#16550=CARTESIAN_POINT ( 'NONE',  ( -3.310556943750001313, 17.50000000000002132, -121.7641058028994792 ) ) ;
#16552=EDGE_CURVE ( 'NONE', #6557, #27019, #37951, .T. ) ;
#16554=VECTOR ( 'NONE', #13971, 1000.000000000000000 ) ;
#16555=ORIENTED_EDGE ( 'NONE', *, *, #1436, .F. ) ;
#16558=CARTESIAN_POINT ( 'NONE',  ( -1.655278471875002211, 14.63297358603754539, -75.59743913623280775 ) ) ;
#16564=CARTESIAN_POINT ( 'NONE',  ( 2.340729813953370519E-16, 21.32270188528332255, -141.0141058028994792 ) ) ;
#16565=CARTESIAN_POINT ( 'NONE',  ( -1.394453263437886604E-15, 14.00000000000001421, -57.71098080242150274 ) ) ;
#16566=CARTESIAN_POINT ( 'NONE',  ( 1.045839947578414805E-15, 14.00000000000002665, -141.7109808024215170 ) ) ;
#16567=CARTESIAN_POINT ( 'NONE',  ( -1.655278471875002211, 14.63297358603754006, -36.68493913623279923 ) ) ;
#16568=CARTESIAN_POINT ( 'NONE',  ( 1.655278471874998436, 14.63297358603754716, -106.5182724695661278 ) ) ;
#16570=CARTESIAN_POINT ( 'NONE',  ( -3.310556943750001313, 17.50000000000001066, -26.76410580289947916 ) ) ;
#16573=CARTESIAN_POINT ( 'NONE',  ( -3.500000000000000888, 19.52072594216371115, -100.0443141357548456 ) ) ;
#16577=CARTESIAN_POINT ( 'NONE',  ( -1.749999999999999778, 20.53108891324555429, -90.82139747004410424 ) ) ;
#16581=CARTESIAN_POINT ( 'NONE',  ( -7.424026671074350129E-16, 13.45854811567263276, -53.71098080242150274 ) ) ;
#16582=CARTESIAN_POINT ( 'NONE',  ( -1.750000000000002220, 14.46891108675447768, -46.48806413671076143 ) ) ;
#16583=CARTESIAN_POINT ( 'NONE',  ( -3.500000000000002220, 15.47927405783633503, -134.5713974700441042 ) ) ;
#16584=CARTESIAN_POINT ( 'NONE',  ( 2.474675557024783212E-16, 21.54145188432739033, -41.90473080337743284 ) ) ;
#16586=CARTESIAN_POINT ( 'NONE',  ( 1.655278471875001101, 20.36702641396248481, -27.18493913623279568 ) ) ;
#16592=CARTESIAN_POINT ( 'NONE',  ( 4.648177544792955347E-16, 21.00000000000001776, -101.9047308033774186 ) ) ;
#16594=CARTESIAN_POINT ( 'NONE',  ( -3.310556943750002201, 15.58864905735837070, -80.68077246956613635 ) ) ;
#16595=CARTESIAN_POINT ( 'NONE',  ( -1.975475456537005874E-15, 21.00000000000002487, -141.9047308033773902 ) ) ;
#16597=CARTESIAN_POINT ( 'NONE',  ( -1.749999999999999778, 20.53108891324554719, -35.82139747004409003 ) ) ;
#16598=ADVANCED_FACE ( 'NONE', ( #22554 ), #7398, .T. ) ;
#16600=ORIENTED_EDGE ( 'NONE', *, *, #4389, .F. ) ;
#16602=CARTESIAN_POINT ( 'NONE',  ( 1.655278471875001101, 20.36702641396249192, -89.09743913623280775 ) ) ;
#16604=ORIENTED_EDGE ( 'NONE', *, *, #21945, .T. ) ;
#16606=LINE ( 'NONE', #26383, #12446 ) ;
#16607=CARTESIAN_POINT ( 'NONE',  ( -3.310556943750000425, 19.41135094264167549, -129.8474391362328220 ) ) ;
#16611=CARTESIAN_POINT ( 'NONE',  ( -1.655278471875002211, 14.63297358603755072, -120.6849391362327992 ) ) ;
#16614=CARTESIAN_POINT ( 'NONE',  ( -1.750000000000002220, 14.46891108675448834, -129.4880641367107614 ) ) ;
#16615=CARTESIAN_POINT ( 'NONE',  ( -7.022189441860112050E-16, 13.67729811471672186, -70.60160580289947063 ) ) ;
#16616=CARTESIAN_POINT ( 'NONE',  ( -3.500000000000000888, 19.52072594216371826, -120.0443141357548313 ) ) ;
#16617=ADVANCED_FACE ( 'NONE', ( #6392 ), #41712, .T. ) ;
#16618=CARTESIAN_POINT ( 'NONE',  ( -1.655278471875002211, 14.63297358603754894, -103.5974391362328220 ) ) ;
#16620=CARTESIAN_POINT ( 'NONE',  ( 1.750000000000001110, 20.53108891324555785, -105.2943141357548313 ) ) ;
#16622=CARTESIAN_POINT ( 'NONE',  ( -3.500000000000002220, 15.47927405783632615, -69.87764746908815994 ) ) ;
#16624=CARTESIAN_POINT ( 'NONE',  ( 1.655278471874998436, 14.63297358603753828, -39.43077246956613635 ) ) ;
#16625=CARTESIAN_POINT ( 'NONE',  ( -3.310556943750002645, 15.58864905735837425, -97.76827246956611361 ) ) ;
#16627=CARTESIAN_POINT ( 'NONE',  ( -3.500000000000001332, 17.50000000000001421, -57.65473080337743284 ) ) ;
#16629=CARTESIAN_POINT ( 'NONE',  ( -7.022189441860112050E-16, 13.67729811471672896, -115.6016058028994706 ) ) ;
#16631=ADVANCED_FACE ( 'NONE', ( #6450 ), #28982, .T. ) ;
#16636=CARTESIAN_POINT ( 'NONE',  ( -7.022189441860112050E-16, 13.67729811471672541, -96.51410580289946495 ) ) ;
#16637=CARTESIAN_POINT ( 'NONE',  ( -1.394453263437886604E-15, 14.00000000000001066, -49.71098080242150274 ) ) ;
#16640=LINE ( 'NONE', #3242, #21995 ) ;
#16641=CARTESIAN_POINT ( 'NONE',  ( -0.9378221735089291577, 21.00000000000002132, -127.1663226036829855 ) ) ;
#16642=VECTOR ( 'NONE', #34608, 1000.000000000000114 ) ;
#16643=CARTESIAN_POINT ( 'NONE',  ( -3.500000000000001332, 17.50000000000002132, -112.6547308033774328 ) ) ;
#16644=VERTEX_POINT ( 'NONE', #38357 ) ;
#16648=CARTESIAN_POINT ( 'NONE',  ( 3.310556943750001313, 19.41135094264166128, -30.18077246956614701 ) ) ;
#16649=EDGE_LOOP ( 'NONE', ( #14529, #37985, #39700, #23336 ) ) ;
#16654=EDGE_LOOP ( 'NONE', ( #26906, #10119, #21408, #19878 ) ) ;
#16656=CARTESIAN_POINT ( 'NONE',  ( -3.500000000000001332, 17.50000000000002132, -114.9609808024215027 ) ) ;
#16657=CARTESIAN_POINT ( 'NONE',  ( 0.9378221735089279365, 21.00000000000002842, -140.2556390011600342 ) ) ;
#16658=CARTESIAN_POINT ( 'NONE',  ( -7.424026671074350129E-16, 13.45854811567263987, -120.4047308033774328 ) ) ;
#16660=CARTESIAN_POINT ( 'NONE',  ( -3.310556943750000425, 19.41135094264167549, -132.9349391362327992 ) ) ;
#16661=CARTESIAN_POINT ( 'NONE',  ( 3.500000000000001776, 19.52072594216370405, -29.37764746908817770 ) ) ;
#16664=CARTESIAN_POINT ( 'NONE',  ( 3.500000000000001332, 19.52072594216370405, -32.37764746908818125 ) ) ;
#16666=CARTESIAN_POINT ( 'NONE',  ( 1.749999999999998224, 14.46891108675447413, -37.32139747004409003 ) ) ;
#16668=CARTESIAN_POINT ( 'NONE',  ( 3.500000000000001776, 19.52072594216372181, -133.3776474690881457 ) ) ;
#16669=CARTESIAN_POINT ( 'NONE',  ( -3.310556943750002645, 15.58864905735837780, -120.6807724695661506 ) ) ;
#16674=FACE_OUTER_BOUND ( 'NONE', #34728, .T. ) ;
#16675=CARTESIAN_POINT ( 'NONE',  ( -3.500000000000001332, 17.50000000000001776, -88.96098080242151696 ) ) ;
#16677=CARTESIAN_POINT ( 'NONE',  ( -3.310556943750002645, 15.58864905735836714, -51.68077246956613635 ) ) ;
#16678=CARTESIAN_POINT ( 'NONE',  ( -1.655278471875002211, 14.63297358603755072, -111.6849391362327992 ) ) ;
#16680=CARTESIAN_POINT ( 'NONE',  ( -3.500000000000000888, 19.52072594216370405, -28.73806413671075788 ) ) ;
#16683=CARTESIAN_POINT ( 'NONE',  ( 3.310556943750001313, 17.50000000000002487, -131.3516058028994564 ) ) ;
#16684=EDGE_CURVE ( 'NONE', #33169, #37838, #29749, .T. ) ;
#16688=CARTESIAN_POINT ( 'NONE',  ( -7.022189441860112050E-16, 13.67729811471671830, -61.60160580289946353 ) ) ;
#16690=CARTESIAN_POINT ( 'NONE',  ( -1.655278471874999990, 20.36702641396248836, -64.93077246956615056 ) ) ;
#16691=VERTEX_POINT ( 'NONE', #41767 ) ;
#16692=CARTESIAN_POINT ( 'NONE',  ( -1.655278471875002211, 14.63297358603754716, -87.68493913623279923 ) ) ;
#16694=CARTESIAN_POINT ( 'NONE',  ( -3.500000000000002220, 15.47927405783632082, -39.87764746908817415 ) ) ;
#16696=CARTESIAN_POINT ( 'NONE',  ( 1.655278471875001101, 20.36702641396248481, -46.09743913623280775 ) ) ;
#16699=ORIENTED_EDGE ( 'NONE', *, *, #15775, .F. ) ;
#16703=CARTESIAN_POINT ( 'NONE',  ( -3.310556943750001313, 17.50000000000001421, -55.76410580289947916 ) ) ;
#16704=VERTEX_POINT ( 'NONE', #266 ) ;
#16705=ORIENTED_EDGE ( 'NONE', *, *, #11116, .F. ) ;
#16709=CARTESIAN_POINT ( 'NONE',  ( 1.749999999999998224, 14.46891108675447590, -47.32139747004410424 ) ) ;
#16711=CARTESIAN_POINT ( 'NONE',  ( -1.750000000000002220, 14.46891108675447768, -41.79431413575483845 ) ) ;
#16712=CARTESIAN_POINT ( 'NONE',  ( -3.310556943750000425, 19.41135094264165772, -43.84743913623280775 ) ) ;
#16713=CARTESIAN_POINT ( 'NONE',  ( 4.648177544792955347E-16, 21.00000000000002487, -139.2109808024214885 ) ) ;
#16714=CARTESIAN_POINT ( 'NONE',  ( 0.9378221735089281585, 14.00000000000000711, -23.66632260368298901 ) ) ;
#16715=DIRECTION ( 'NONE',  ( -0.000000000000000000, 1.259100132267607459E-16, -1.000000000000000000 ) ) ;
#16716=( BOUNDED_CURVE ( )  B_SPLINE_CURVE ( 2, ( #3165, #13363, #6983, #29518, #36109, #26344, #19957, #23141, #39292 ),
 .UNSPECIFIED., .F., .T. ) 
 B_SPLINE_CURVE_WITH_KNOTS ( ( 3, 2, 2, 2, 3 ),
 ( 0.1187500000000000083, 0.1194444444444444503, 0.1208333333333333343, 0.1222222222222222182, 0.1229166666666666741 ),
 .UNSPECIFIED. ) 
 CURVE ( )  GEOMETRIC_REPRESENTATION_ITEM ( )  RATIONAL_B_SPLINE_CURVE ( ( 0.9330127018922194093, 0.9330127018922200755, 1.000000000000000000, 0.8660254037844387076, 1.000000000000000000, 0.8660254037844387076, 1.000000000000000000, 0.9330127018922187432, 0.9330127018922194093 ) ) 
 REPRESENTATION_ITEM ( '' )  );
#16718=CARTESIAN_POINT ( 'NONE',  ( 1.655278471874998436, 14.63297358603753828, -32.51827246956613493 ) ) ;
#16719=CARTESIAN_POINT ( 'NONE',  ( -1.655278471875002211, 14.63297358603753828, -23.68493913623280633 ) ) ;
#16720=CARTESIAN_POINT ( 'NONE',  ( -3.310556943750001313, 17.50000000000001776, -83.85160580289947063 ) ) ;
#16721=CARTESIAN_POINT ( 'NONE',  ( 2.340729813953370519E-16, 21.32270188528332255, -136.0141058028994792 ) ) ;
#16725=CARTESIAN_POINT ( 'NONE',  ( 1.655278471874998436, 14.63297358603755072, -129.5182724695661136 ) ) ;
#16728=CARTESIAN_POINT ( 'NONE',  ( 2.340729813953370519E-16, 21.32270188528331190, -90.01410580289947916 ) ) ;
#16729=CARTESIAN_POINT ( 'NONE',  ( 7.367361408496833051E-14, 14.00000000000001776, -95.40473080337743284 ) ) ;
#16730=DIRECTION ( 'NONE',  ( 0.000000000000000000, 1.000000000000000000, 0.000000000000000000 ) ) ;
#16732=CARTESIAN_POINT ( 'NONE',  ( 1.750000000000001110, 20.53108891324555074, -73.98806413671076143 ) ) ;
#16733=CARTESIAN_POINT ( 'NONE',  ( 2.340729813953370519E-16, 21.32270188528331190, -59.10160580289947063 ) ) ;
#16735=DIRECTION ( 'NONE',  ( -0.000000000000000000, 1.259100132267607459E-16, -1.000000000000000000 ) ) ;
#16737=CARTESIAN_POINT ( 'NONE',  ( -1.655278471874999990, 20.36702641396249192, -82.01827246956614204 ) ) ;
#16738=CARTESIAN_POINT ( 'NONE',  ( -3.500000000000001332, 17.50000000000001421, -59.96098080242151696 ) ) ;
#16740=CARTESIAN_POINT ( 'NONE',  ( -7.022189441860112050E-16, 13.67729811471672541, -107.5141058028994507 ) ) ;
#16741=CARTESIAN_POINT ( 'NONE',  ( 3.310556943750001313, 17.50000000000001776, -78.26410580289946495 ) ) ;
#16744=CARTESIAN_POINT ( 'NONE',  ( -3.310556943750000425, 19.41135094264166838, -99.93493913623279923 ) ) ;
#16745=CARTESIAN_POINT ( 'NONE',  ( 3.500000000000000000, 15.47927405783632793, -104.2380641367107614 ) ) ;
#16748=CARTESIAN_POINT ( 'NONE',  ( -1.749999999999999778, 20.53108891324554719, -38.12764746908817415 ) ) ;
#16751=CARTESIAN_POINT ( 'NONE',  ( -7.022189441860112050E-16, 13.67729811471672186, -62.51410580289947205 ) ) ;
#16752=CARTESIAN_POINT ( 'NONE',  ( -3.500000000000001332, 17.50000000000001066, -29.96098080242151696 ) ) ;
#16754=CARTESIAN_POINT ( 'NONE',  ( 3.310556943750001313, 19.41135094264166838, -121.1807724695661506 ) ) ;
#16755=FACE_OUTER_BOUND ( 'NONE', #5499, .T. ) ;
#16757=ORIENTED_EDGE ( 'NONE', *, *, #391, .F. ) ;
#16758=EDGE_CURVE ( 'NONE', #11063, #31496, #3410, .T. ) ;
#16761=CARTESIAN_POINT ( 'NONE',  ( 0.9378221735089300459, 21.00000000000002487, -130.9493890021159359 ) ) ;
#16762=FACE_OUTER_BOUND ( 'NONE', #36043, .T. ) ;
#16763=CARTESIAN_POINT ( 'NONE',  ( 3.310556943749999981, 15.58864905735836714, -75.34743913623280775 ) ) ;
#16765=EDGE_LOOP ( 'NONE', ( #20009, #16351, #14466, #17451 ) ) ;
#16770=CARTESIAN_POINT ( 'NONE',  ( -3.310556943750002201, 15.58864905735837958, -137.6807724695661364 ) ) ;
#16773=CARTESIAN_POINT ( 'NONE',  ( -3.310556943750001313, 17.50000000000001066, -35.85160580289946353 ) ) ;
#16774=CARTESIAN_POINT ( 'NONE',  ( -3.310556943750001313, 17.50000000000002132, -105.8516058028994564 ) ) ;
#16777=EDGE_CURVE ( 'NONE', #34104, #16103, #7778, .T. ) ;
#16778=CARTESIAN_POINT ( 'NONE',  ( 3.310556943750001313, 17.50000000000001066, -23.26410580289947561 ) ) ;
#16779=CARTESIAN_POINT ( 'NONE',  ( 3.500000000000001332, 17.50000000000001421, -69.15473080337743284 ) ) ;
#16780=CARTESIAN_POINT ( 'NONE',  ( -3.500000000000001332, 17.50000000000001776, -99.96098080242150274 ) ) ;
#16782=CARTESIAN_POINT ( 'NONE',  ( -3.500000000000001332, 17.50000000000002132, -118.9609808024215170 ) ) ;
#16783=CARTESIAN_POINT ( 'NONE',  ( 3.500000000000001776, 19.52072594216371115, -91.07139747004409003 ) ) ;
#16787=CARTESIAN_POINT ( 'NONE',  ( 2.474675557024783212E-16, 21.54145188432739388, -52.21098080242150274 ) ) ;
#16789=CARTESIAN_POINT ( 'NONE',  ( 0.000000000000000000, 17.50000000000002487, -149.5231586289125687 ) ) ;
#16790=CARTESIAN_POINT ( 'NONE',  ( -7.424026671074350129E-16, 13.45854811567263276, -45.40473080337742573 ) ) ;
#16792=CARTESIAN_POINT ( 'NONE',  ( 3.310556943750001313, 19.41135094264166128, -27.26827246956613138 ) ) ;
#16794=CARTESIAN_POINT ( 'NONE',  ( -3.500000000000001332, 17.50000000000001066, -39.65473080337743284 ) ) ;
#16798=CARTESIAN_POINT ( 'NONE',  ( -3.310556943750001313, 17.50000000000001776, -78.76410580289946495 ) ) ;
#16799=CARTESIAN_POINT ( 'NONE',  ( -0.9378221735089299349, 14.00000000000002487, -141.4493890021159643 ) ) ;
#16802=CARTESIAN_POINT ( 'NONE',  ( 0.9378221735089281585, 14.00000000000000888, -27.36007260463891555 ) ) ;
#16806=CARTESIAN_POINT ( 'NONE',  ( 3.310556943750001313, 17.50000000000001776, -89.26410580289947916 ) ) ;
#16807=ORIENTED_EDGE ( 'NONE', *, *, #23062, .F. ) ;
#16808=VERTEX_POINT ( 'NONE', #20588 ) ;
#16811=CARTESIAN_POINT ( 'NONE',  ( 3.500000000000000000, 15.47927405783633326, -115.5443141357548313 ) ) ;
#16812=CARTESIAN_POINT ( 'NONE',  ( -1.655278471874999990, 20.36702641396249547, -126.9307724695661364 ) ) ;
#16813=ORIENTED_EDGE ( 'NONE', *, *, #5608, .T. ) ;
#16814=CARTESIAN_POINT ( 'NONE',  ( -1.750000000000002220, 14.46891108675447590, -31.48806413671076498 ) ) ;
#16815=CARTESIAN_POINT ( 'NONE',  ( 3.310556943750001313, 19.41135094264166128, -53.26827246956612072 ) ) ;
#16816=CARTESIAN_POINT ( 'NONE',  ( -7.022189441860112050E-16, 13.67729811471672718, -121.6016058028994706 ) ) ;
#16820=CARTESIAN_POINT ( 'NONE',  ( 2.474675557024783212E-16, 21.54145188432740099, -123.9047308033774186 ) ) ;
#16822=CARTESIAN_POINT ( 'NONE',  ( -3.310556943750000425, 19.41135094264165772, -37.84743913623281486 ) ) ;
#16823=CARTESIAN_POINT ( 'NONE',  ( -3.310556943750002645, 15.58864905735837070, -72.76827246956612782 ) ) ;
#16824=CARTESIAN_POINT ( 'NONE',  ( -1.750000000000002220, 14.46891108675448656, -115.7943141357548313 ) ) ;
#16825=CARTESIAN_POINT ( 'NONE',  ( -3.310556943750000425, 19.41135094264166483, -101.8474391362328078 ) ) ;
#16829=CARTESIAN_POINT ( 'NONE',  ( -1.749999999999999778, 20.53108891324555074, -72.12764746908817415 ) ) ;
#16830=CARTESIAN_POINT ( 'NONE',  ( 0.000000000000000000, 17.50000000000002487, -149.5231586289125687 ) ) ;
#16831=CARTESIAN_POINT ( 'NONE',  ( -3.310556943750002645, 15.58864905735836537, -39.68077246956613635 ) ) ;
#16832=CARTESIAN_POINT ( 'NONE',  ( 3.310556943750001313, 17.50000000000001776, -95.35160580289945642 ) ) ;
#16833=( BOUNDED_CURVE ( )  B_SPLINE_CURVE ( 2, ( #35329, #17, #35541, #38941, #3005, #15997, #41935, #9819, #12782 ),
 .UNSPECIFIED., .F., .F. ) 
 B_SPLINE_CURVE_WITH_KNOTS ( ( 3, 2, 2, 2, 3 ),
 ( 0.03125000000000000000, 0.03194444444444444198, 0.03333333333333333287, 0.03472222222222222376, 0.03541666666666666574 ),
 .UNSPECIFIED. ) 
 CURVE ( )  GEOMETRIC_REPRESENTATION_ITEM ( )  RATIONAL_B_SPLINE_CURVE ( ( 0.9330127018922194093, 0.9330127018922195203, 1.000000000000000000, 0.8660254037844387076, 1.000000000000000000, 0.8660254037844387076, 1.000000000000000000, 0.9330127018922194093, 0.9330127018922194093 ) ) 
 REPRESENTATION_ITEM ( '' )  );
#16834=CARTESIAN_POINT ( 'NONE',  ( 1.749999999999998224, 14.46891108675447768, -61.32139747004409713 ) ) ;
#16836=CARTESIAN_POINT ( 'NONE',  ( 1.655278471874998436, 14.63297358603754894, -112.5182724695661420 ) ) ;
#16837=CARTESIAN_POINT ( 'NONE',  ( -1.655278471874999990, 20.36702641396248481, -45.01827246956613493 ) ) ;
#16839=CARTESIAN_POINT ( 'NONE',  ( -3.500000000000002220, 15.47927405783632615, -62.57139747004410424 ) ) ;
#16843=CARTESIAN_POINT ( 'NONE',  ( 0.9378221735089300459, 21.00000000000002132, -107.2556390011600342 ) ) ;
#16844=CARTESIAN_POINT ( 'NONE',  ( -7.022189441860112050E-16, 13.67729811471672541, -100.5141058028994792 ) ) ;
#16846=ORIENTED_EDGE ( 'NONE', *, *, #425, .F. ) ;
#16850=CARTESIAN_POINT ( 'NONE',  ( 0.9378221735089281585, 14.00000000000002309, -123.3600726046389155 ) ) ;
#16851=ORIENTED_EDGE ( 'NONE', *, *, #2433, .F. ) ;
#16852=CARTESIAN_POINT ( 'NONE',  ( 0.000000000000000000, 17.50000000000002487, -149.5231586289125687 ) ) ;
#16856=CARTESIAN_POINT ( 'NONE',  ( 3.310556943749999981, 15.58864905735836182, -28.34743913623280420 ) ) ;
#16858=DIRECTION ( 'NONE',  ( -0.000000000000000000, 1.259100132267607459E-16, -1.000000000000000000 ) ) ;
#16864=ORIENTED_EDGE ( 'NONE', *, *, #42020, .T. ) ;
#16865=CARTESIAN_POINT ( 'NONE',  ( -1.655278471875002211, 14.63297358603755427, -142.5974391362327935 ) ) ;
#16869=CARTESIAN_POINT ( 'NONE',  ( -1.655278471874999990, 20.36702641396249902, -135.0182724695661420 ) ) ;
#16870=CARTESIAN_POINT ( 'NONE',  ( -3.500000000000001332, 17.50000000000001066, -28.96098080242151696 ) ) ;
#16872=CARTESIAN_POINT ( 'NONE',  ( 3.500000000000001776, 19.52072594216372181, -140.0713974700441042 ) ) ;
#16875=CARTESIAN_POINT ( 'NONE',  ( 3.500000000000001776, 19.52072594216372181, -131.3776474690881741 ) ) ;
#16876=CARTESIAN_POINT ( 'NONE',  ( -3.310556943750001313, 17.50000000000002132, -117.7641058028994792 ) ) ;
#16880=CARTESIAN_POINT ( 'NONE',  ( 1.749999999999998224, 14.46891108675448123, -84.62764746908817415 ) ) ;
#16881=AXIS2_PLACEMENT_3D ( 'NONE', #36627, #10681, #1528 ) ;
#16882=CARTESIAN_POINT ( 'NONE',  ( -3.500000000000002220, 15.47927405783632793, -69.57139747004409003 ) ) ;
#16883=CARTESIAN_POINT ( 'NONE',  ( -3.310556943750001313, 17.50000000000001421, -52.76410580289947205 ) ) ;
#16884=CARTESIAN_POINT ( 'NONE',  ( 1.655278471875001101, 20.36702641396249547, -110.1849391362327992 ) ) ;
#16886=CARTESIAN_POINT ( 'NONE',  ( 3.500000000000001332, 17.50000000000001066, -29.15473080337743639 ) ) ;
#16889=CARTESIAN_POINT ( 'NONE',  ( 1.655278471874998436, 14.63297358603755072, -133.5182724695661420 ) ) ;
#16892=CARTESIAN_POINT ( 'NONE',  ( 3.310556943750001313, 19.41135094264166128, -62.26827246956614204 ) ) ;
#16894=CARTESIAN_POINT ( 'NONE',  ( -7.022189441860112050E-16, 13.67729811471671830, -61.51410580289946495 ) ) ;
#16896=CARTESIAN_POINT ( 'NONE',  ( -3.310556943750001313, 17.50000000000001776, -86.85160580289947063 ) ) ;
#16901=CARTESIAN_POINT ( 'NONE',  ( -1.655278471874999990, 20.36702641396248481, -44.93077246956614346 ) ) ;
#16903=CARTESIAN_POINT ( 'NONE',  ( -1.655278471874999990, 20.36702641396249192, -99.93077246956613635 ) ) ;
#16905=ORIENTED_EDGE ( 'NONE', *, *, #12642, .T. ) ;
#16907=VERTEX_POINT ( 'NONE', #38418 ) ;
#16909=CARTESIAN_POINT ( 'NONE',  ( 3.310556943750001313, 19.41135094264166128, -50.18077246956615056 ) ) ;
#16910=( BOUNDED_CURVE ( )  B_SPLINE_CURVE ( 2, ( #40490, #8156, #4756, #17527, #26889, #23704, #11345, #10933, #4119 ),
 .UNSPECIFIED., .F., .F. ) 
 B_SPLINE_CURVE_WITH_KNOTS ( ( 3, 2, 2, 2, 3 ),
 ( 0.4729166666666666519, 0.4736111111111110938, 0.4749999999999999778, 0.4763888888888888618, 0.4770833333333333592 ),
 .UNSPECIFIED. ) 
 CURVE ( )  GEOMETRIC_REPRESENTATION_ITEM ( )  RATIONAL_B_SPLINE_CURVE ( ( 0.9330127018922194093, 0.9330127018922194093, 1.000000000000000000, 0.8660254037844387076, 1.000000000000000000, 0.8660254037844387076, 1.000000000000000000, 0.9330127018922167448, 0.9330127018922194093 ) ) 
 REPRESENTATION_ITEM ( '' )  );
#16912=ORIENTED_EDGE ( 'NONE', *, *, #34732, .F. ) ;
#16914=FACE_OUTER_BOUND ( 'NONE', #24246, .T. ) ;
#16915=CARTESIAN_POINT ( 'NONE',  ( -3.500000000000000000, 19.52072594216371115, -91.73806413671076143 ) ) ;
#16917=CARTESIAN_POINT ( 'NONE',  ( 3.500000000000001332, 17.50000000000002132, -114.4609808024215027 ) ) ;
#16920=CARTESIAN_POINT ( 'NONE',  ( -1.750000000000002220, 14.46891108675447768, -42.79431413575483845 ) ) ;
#16921=CARTESIAN_POINT ( 'NONE',  ( 3.310556943749999981, 15.58864905735836182, -43.34743913623280775 ) ) ;
#16922=CARTESIAN_POINT ( 'NONE',  ( 0.9378221735089281585, 14.00000000000000888, -35.36007260463890844 ) ) ;
#16923=CARTESIAN_POINT ( 'NONE',  ( -0.9378221735089291577, 21.00000000000002487, -133.8600726046389013 ) ) ;
#16925=CARTESIAN_POINT ( 'NONE',  ( 3.310556943750001313, 19.41135094264165772, -28.26827246956613493 ) ) ;
#16926=CARTESIAN_POINT ( 'NONE',  ( -1.394453263437886604E-15, 14.00000000000001776, -97.40473080337741862 ) ) ;
#16927=CARTESIAN_POINT ( 'NONE',  ( -1.655278471874999990, 20.36702641396249192, -80.01827246956614204 ) ) ;
#16928=CARTESIAN_POINT ( 'NONE',  ( 3.310556943749999981, 15.58864905735837425, -134.3474391362328220 ) ) ;
#16933=CARTESIAN_POINT ( 'NONE',  ( 3.310556943749999981, 15.58864905735837425, -125.4349391362327992 ) ) ;
#16934=CARTESIAN_POINT ( 'NONE',  ( 1.655278471875001101, 20.36702641396249192, -84.09743913623279354 ) ) ;
#16935=CYLINDRICAL_SURFACE ( 'NONE', #4970, 3.499999999999999556 ) ;
#16936=CARTESIAN_POINT ( 'NONE',  ( -1.394453263437886604E-15, 14.00000000000001421, -75.71098080242151696 ) ) ;
#16937=CARTESIAN_POINT ( 'NONE',  ( 4.648177544792955347E-16, 21.00000000000002132, -111.2109808024214885 ) ) ;
#16938=CARTESIAN_POINT ( 'NONE',  ( -3.500000000000000888, 19.52072594216370760, -73.73806413671074722 ) ) ;
#16939=CARTESIAN_POINT ( 'NONE',  ( 3.310556943750001313, 17.50000000000001421, -57.35160580289947063 ) ) ;
#16942=CARTESIAN_POINT ( 'NONE',  ( 4.648177544792955347E-16, 21.00000000000002487, -129.9047308033774186 ) ) ;
#16943=CARTESIAN_POINT ( 'NONE',  ( -3.310556943750000425, 19.41135094264166483, -80.93493913623279923 ) ) ;
#16944=CARTESIAN_POINT ( 'NONE',  ( -1.655278471875002211, 14.63297358603755427, -139.6849391362327708 ) ) ;
#16947=CARTESIAN_POINT ( 'NONE',  ( 3.310556943750001313, 17.50000000000002132, -109.2641058028994649 ) ) ;
#16948=CARTESIAN_POINT ( 'NONE',  ( 2.340729813953370519E-16, 21.32270188528331190, -79.01410580289947916 ) ) ;
#16949=CARTESIAN_POINT ( 'NONE',  ( 3.500000000000000000, 15.47927405783633503, -138.5443141357548598 ) ) ;
#16951=CARTESIAN_POINT ( 'NONE',  ( 3.310556943750001313, 19.41135094264166838, -104.2682724695661278 ) ) ;
#16952=CARTESIAN_POINT ( 'NONE',  ( 3.500000000000001776, 19.52072594216371826, -105.0713974700441042 ) ) ;
#16954=CARTESIAN_POINT ( 'NONE',  ( 4.648177544792955347E-16, 21.00000000000001776, -94.90473080337743284 ) ) ;
#16955=CARTESIAN_POINT ( 'NONE',  ( -3.500000000000001332, 17.50000000000001066, -37.96098080242150985 ) ) ;
#16958=CARTESIAN_POINT ( 'NONE',  ( -7.022189441860112050E-16, 13.67729811471672186, -59.51410580289948626 ) ) ;
#16960=CARTESIAN_POINT ( 'NONE',  ( -3.310556943750002645, 15.58864905735837780, -113.6807724695661364 ) ) ;
#16961=CARTESIAN_POINT ( 'NONE',  ( 3.369928719974892676E-15, 14.00000000000002309, -140.7109808024215170 ) ) ;
#16964=ORIENTED_EDGE ( 'NONE', *, *, #3721, .F. ) ;
#16968=CARTESIAN_POINT ( 'NONE',  ( 1.749999999999998224, 14.46891108675448656, -128.3213974700441042 ) ) ;
#16969=CARTESIAN_POINT ( 'NONE',  ( -3.310556943750001313, 17.50000000000001421, -66.76410580289947916 ) ) ;
#16972=( BOUNDED_CURVE ( )  B_SPLINE_CURVE ( 2, ( #40689, #20503, #4960, #33473, #11545, #14334, #7746, #24537, #4335 ),
 .UNSPECIFIED., .F., .F. ) 
 B_SPLINE_CURVE_WITH_KNOTS ( ( 3, 2, 2, 2, 3 ),
 ( 0.1562500000000000000, 0.1569444444444444420, 0.1583333333333333259, 0.1597222222222222099, 0.1604166666666666796 ),
 .UNSPECIFIED. ) 
 CURVE ( )  GEOMETRIC_REPRESENTATION_ITEM ( )  RATIONAL_B_SPLINE_CURVE ( ( 0.9330127018922194093, 0.9330127018922194093, 1.000000000000000000, 0.8660254037844387076, 1.000000000000000000, 0.8660254037844387076, 1.000000000000000000, 0.9330127018922180770, 0.9330127018922194093 ) ) 
 REPRESENTATION_ITEM ( '' )  );
#16973=CARTESIAN_POINT ( 'NONE',  ( 4.648177544792955347E-16, 21.00000000000002132, -111.9047308033774186 ) ) ;
#16975=ORIENTED_EDGE ( 'NONE', *, *, #22321, .F. ) ;
#16976=CARTESIAN_POINT ( 'NONE',  ( -3.310556943750001313, 17.50000000000002487, -137.7641058028994792 ) ) ;
#16979=CARTESIAN_POINT ( 'NONE',  ( 1.655278471874998436, 14.63297358603754006, -47.51827246956613493 ) ) ;
#16980=CARTESIAN_POINT ( 'NONE',  ( -3.500000000000001332, 17.50000000000001776, -89.65473080337743284 ) ) ;
#16981=CARTESIAN_POINT ( 'NONE',  ( -1.655278471875002211, 14.63297358603754184, -40.68493913623279212 ) ) ;
#16982=CARTESIAN_POINT ( 'NONE',  ( -1.655278471874999990, 20.36702641396249192, -97.01827246956612782 ) ) ;
#16984=AXIS2_PLACEMENT_3D ( 'NONE', #39753, #38908, #36126 ) ;
#16986=CARTESIAN_POINT ( 'NONE',  ( 3.310556943750001313, 19.41135094264165772, -24.18077246956613990 ) ) ;
#16987=FACE_OUTER_BOUND ( 'NONE', #5765, .T. ) ;
#16988=CARTESIAN_POINT ( 'NONE',  ( 3.500000000000001332, 17.50000000000001776, -99.46098080242150274 ) ) ;
#16989=CARTESIAN_POINT ( 'NONE',  ( 3.500000000000001332, 19.52072594216371826, -124.3776474690881599 ) ) ;
#16991=CARTESIAN_POINT ( 'NONE',  ( 1.750000000000001110, 20.53108891324555429, -92.98806413671076143 ) ) ;
#16995=CARTESIAN_POINT ( 'NONE',  ( 3.500000000000001332, 19.52072594216370760, -68.07139747004409003 ) ) ;
#16996=CARTESIAN_POINT ( 'NONE',  ( 1.749999999999998224, 14.46891108675447590, -53.62764746908817415 ) ) ;
#16997=DIRECTION ( 'NONE',  ( 0.000000000000000000, 1.000000000000000000, 0.000000000000000000 ) ) ;
#16998=CARTESIAN_POINT ( 'NONE',  ( -0.9378221735089221633, 14.00000000000001599, -134.4493890021159359 ) ) ;
#16999=ORIENTED_EDGE ( 'NONE', *, *, #24575, .T. ) ;
#17000=CARTESIAN_POINT ( 'NONE',  ( 3.500000000000001776, 19.52072594216370405, -45.07139747004409713 ) ) ;
#17002=CARTESIAN_POINT ( 'NONE',  ( -3.310556943750002201, 15.58864905735836537, -29.76827246956613493 ) ) ;
#17003=CARTESIAN_POINT ( 'NONE',  ( -1.750000000000002220, 14.46891108675447590, -39.48806413671076854 ) ) ;
#17006=CARTESIAN_POINT ( 'NONE',  ( -3.500000000000000000, 19.52072594216371826, -107.0443141357548456 ) ) ;
#17008=CARTESIAN_POINT ( 'NONE',  ( 3.310556943749999981, 15.58864905735836714, -76.34743913623280775 ) ) ;
#17012=CARTESIAN_POINT ( 'NONE',  ( -1.749999999999999778, 20.53108891324555429, -98.12764746908817415 ) ) ;
#17013=CARTESIAN_POINT ( 'NONE',  ( 4.286263797015737581E-16, 14.00000000000002487, -149.5231586289125687 ) ) ;
#17014=VERTEX_POINT ( 'NONE', #5672 ) ;
#17015=CARTESIAN_POINT ( 'NONE',  ( -3.500000000000001332, 17.50000000000001776, -87.96098080242151696 ) ) ;
#17016=CARTESIAN_POINT ( 'NONE',  ( 2.340729813953370519E-16, 21.32270188528331190, -92.01410580289947916 ) ) ;
#17017=EDGE_CURVE ( 'NONE', #3780, #38312, #31194, .T. ) ;
#17018=ORIENTED_EDGE ( 'NONE', *, *, #37020, .T. ) ;
#17019=ORIENTED_EDGE ( 'NONE', *, *, #17284, .F. ) ;
#17023=CARTESIAN_POINT ( 'NONE',  ( 4.286263797015737581E-16, 14.00000000000002487, -149.5231586289125687 ) ) ;
#17024=CARTESIAN_POINT ( 'NONE',  ( 1.655278471874998436, 14.63297358603755072, -127.4307724695661364 ) ) ;
#17026=CARTESIAN_POINT ( 'NONE',  ( 1.655278471875001101, 20.36702641396248836, -52.18493913623279923 ) ) ;
#17027=CARTESIAN_POINT ( 'NONE',  ( -3.310556943750001313, 17.50000000000002132, -113.8516058028994706 ) ) ;
#17028=ORIENTED_EDGE ( 'NONE', *, *, #33137, .F. ) ;
#17031=CARTESIAN_POINT ( 'NONE',  ( 3.500000000000001776, 19.52072594216371826, -127.0713974700440900 ) ) ;
#17032=VECTOR ( 'NONE', #12809, 1000.000000000000000 ) ;
#17033=ADVANCED_FACE ( 'NONE', ( #32031 ), #2269, .T. ) ;
#17034=CARTESIAN_POINT ( 'NONE',  ( 2.340729813953370519E-16, 21.32270188528330479, -38.01410580289947916 ) ) ;
#17035=CARTESIAN_POINT ( 'NONE',  ( 3.310556943750001313, 19.41135094264166128, -71.26827246956612782 ) ) ;
#17036=CARTESIAN_POINT ( 'NONE',  ( -7.424026671074350129E-16, 13.45854811567263987, -115.7109808024215027 ) ) ;
#17037=CARTESIAN_POINT ( 'NONE',  ( -1.655278471875002211, 14.63297358603754894, -102.5974391362328220 ) ) ;
#17039=DIRECTION ( 'NONE',  ( 0.000000000000000000, 1.000000000000000000, 0.000000000000000000 ) ) ;
#17041=CARTESIAN_POINT ( 'NONE',  ( -3.500000000000000888, 19.52072594216370760, -69.04431413575484555 ) ) ;
#17042=FACE_OUTER_BOUND ( 'NONE', #34638, .T. ) ;
#17043=CARTESIAN_POINT ( 'NONE',  ( -1.655278471874999990, 20.36702641396248481, -37.93077246956613635 ) ) ;
#17044=CARTESIAN_POINT ( 'NONE',  ( 3.310556943749999981, 15.58864905735837070, -98.43493913623279923 ) ) ;
#17045=CARTESIAN_POINT ( 'NONE',  ( -7.424026671074350129E-16, 13.45854811567263454, -59.40473080337743994 ) ) ;
#17047=CARTESIAN_POINT ( 'NONE',  ( 2.340729813953370519E-16, 21.32270188528331900, -112.1016058028994706 ) ) ;
#17048=CARTESIAN_POINT ( 'NONE',  ( 1.655278471874998436, 14.63297358603754006, -41.51827246956612782 ) ) ;
#17050=CARTESIAN_POINT ( 'NONE',  ( 1.749999999999998224, 14.46891108675448656, -127.6276474690881741 ) ) ;
#17054=CARTESIAN_POINT ( 'NONE',  ( 2.340729813953370519E-16, 21.32270188528331190, -93.01410580289947916 ) ) ;
#17055=CARTESIAN_POINT ( 'NONE',  ( 3.500000000000001332, 19.52072594216370760, -62.37764746908818125 ) ) ;
#17057=EDGE_LOOP ( 'NONE', ( #13912, #21875, #11399, #18844 ) ) ;
#17061=ORIENTED_EDGE ( 'NONE', *, *, #30679, .T. ) ;
#17064=CARTESIAN_POINT ( 'NONE',  ( 1.655278471874998436, 14.63297358603753828, -30.43077246956614346 ) ) ;
#17066=EDGE_CURVE ( 'NONE', #15239, #18479, #41617, .T. ) ;
#17067=ORIENTED_EDGE ( 'NONE', *, *, #27748, .T. ) ;
#17073=ORIENTED_EDGE ( 'NONE', *, *, #14331, .F. ) ;
#17076=CARTESIAN_POINT ( 'NONE',  ( 0.9378221735089324884, 14.00000000000002665, -137.3600726046389582 ) ) ;
#17077=CARTESIAN_POINT ( 'NONE',  ( 3.602337597214540226E-14, 14.00000000000002132, -116.7109808024215170 ) ) ;
#17078=CARTESIAN_POINT ( 'NONE',  ( -0.9378221735089310451, 14.00000000000001599, -74.75563900116003424 ) ) ;
#17079=CARTESIAN_POINT ( 'NONE',  ( -7.022189441860112050E-16, 13.67729811471672718, -127.6016058028994706 ) ) ;
#17080=CARTESIAN_POINT ( 'NONE',  ( 1.750000000000001110, 20.53108891324554719, -28.29431413575483845 ) ) ;
#17083=CARTESIAN_POINT ( 'NONE',  ( -1.750000000000002220, 14.46891108675449011, -140.4880641367107614 ) ) ;
#17085=CARTESIAN_POINT ( 'NONE',  ( 0.9378221735089281585, 14.00000000000002309, -123.6663226036829855 ) ) ;
#17087=CARTESIAN_POINT ( 'NONE',  ( -7.424026671074350129E-16, 13.45854811567264164, -134.7109808024214885 ) ) ;
#17088=CARTESIAN_POINT ( 'NONE',  ( 3.310556943749999981, 15.58864905735837247, -118.3474391362328078 ) ) ;
#17091=CARTESIAN_POINT ( 'NONE',  ( -3.500000000000002220, 15.47927405783632793, -83.87764746908818836 ) ) ;
#17094=CARTESIAN_POINT ( 'NONE',  ( -3.310556943750000425, 19.41135094264166128, -53.84743913623281486 ) ) ;
#17095=CARTESIAN_POINT ( 'NONE',  ( -1.655278471874999990, 20.36702641396249547, -111.0182724695661420 ) ) ;
#17097=CARTESIAN_POINT ( 'NONE',  ( 1.749999999999998224, 14.46891108675447413, -29.32139747004410069 ) ) ;
#17098=CARTESIAN_POINT ( 'NONE',  ( 1.750000000000001110, 20.53108891324555785, -116.2943141357548313 ) ) ;
#17100=EDGE_CURVE ( 'NONE', #10733, #2733, #41200, .T. ) ;
#17101=CARTESIAN_POINT ( 'NONE',  ( 1.655278471874998436, 14.63297358603755072, -126.5182724695661278 ) ) ;
#17103=CARTESIAN_POINT ( 'NONE',  ( -1.394453263437886604E-15, 14.00000000000001066, -29.71098080242150985 ) ) ;
#17105=CARTESIAN_POINT ( 'NONE',  ( -7.022189441860112050E-16, 13.67729811471671830, -63.60160580289946353 ) ) ;
#17107=VERTEX_POINT ( 'NONE', #8646 ) ;
#17109=CARTESIAN_POINT ( 'NONE',  ( -1.655278471875002211, 14.63297358603754716, -82.68493913623278502 ) ) ;
#17115=CARTESIAN_POINT ( 'NONE',  ( -3.310556943750001313, 17.50000000000001066, -42.76410580289947916 ) ) ;
#17117=CARTESIAN_POINT ( 'NONE',  ( -7.022189441860112050E-16, 13.67729811471672541, -99.51410580289946495 ) ) ;
#17118=CARTESIAN_POINT ( 'NONE',  ( 1.749999999999998224, 14.46891108675447590, -42.32139747004409713 ) ) ;
#17124=CARTESIAN_POINT ( 'NONE',  ( -1.655278471875002211, 14.63297358603754184, -52.59743913623281486 ) ) ;
#17125=ORIENTED_EDGE ( 'NONE', *, *, #1843, .F. ) ;
#17127=CARTESIAN_POINT ( 'NONE',  ( 3.500000000000000000, 15.47927405783632793, -93.54431413575484555 ) ) ;
#17131=ORIENTED_EDGE ( 'NONE', *, *, #40157, .T. ) ;
#17133=CARTESIAN_POINT ( 'NONE',  ( 3.500000000000000000, 15.47927405783632082, -46.54431413575484555 ) ) ;
#17134=CARTESIAN_POINT ( 'NONE',  ( 0.9378221735089300459, 21.00000000000002132, -108.2556390011600342 ) ) ;
#17135=CARTESIAN_POINT ( 'NONE',  ( 3.500000000000001332, 17.50000000000002132, -125.4609808024215170 ) ) ;
#17138=CARTESIAN_POINT ( 'NONE',  ( -3.310556943750001313, 17.50000000000001066, -31.85160580289945997 ) ) ;
#17140=CARTESIAN_POINT ( 'NONE',  ( -1.655278471874999990, 20.36702641396249192, -83.01827246956614204 ) ) ;
#17141=CARTESIAN_POINT ( 'NONE',  ( -3.310556943750002645, 15.58864905735837780, -132.6807724695661364 ) ) ;
#17145=CARTESIAN_POINT ( 'NONE',  ( -3.310556943750001313, 17.50000000000002132, -125.8516058028994706 ) ) ;
#17147=CARTESIAN_POINT ( 'NONE',  ( 1.655278471875001101, 20.36702641396249192, -87.09743913623280775 ) ) ;
#17150=FACE_OUTER_BOUND ( 'NONE', #37878, .T. ) ;
#17151=CARTESIAN_POINT ( 'NONE',  ( -1.655278471874999990, 20.36702641396249902, -142.0182724695661420 ) ) ;
#17152=CARTESIAN_POINT ( 'NONE',  ( 3.500000000000000000, 15.47927405783632437, -73.23806413671076143 ) ) ;
#17154=CARTESIAN_POINT ( 'NONE',  ( -1.655278471874999990, 20.36702641396248836, -54.01827246956612782 ) ) ;
#17157=CARTESIAN_POINT ( 'NONE',  ( -3.500000000000002220, 15.47927405783633326, -98.87764746908815994 ) ) ;
#17159=CARTESIAN_POINT ( 'NONE',  ( 1.655278471875001101, 20.36702641396249192, -79.18493913623279923 ) ) ;
#17160=EDGE_CURVE ( 'NONE', #39717, #15516, #6084, .T. ) ;
#17161=CARTESIAN_POINT ( 'NONE',  ( -1.655278471874999990, 20.36702641396249902, -139.0182724695661420 ) ) ;
#17163=CARTESIAN_POINT ( 'NONE',  ( 3.310556943750001313, 19.41135094264166838, -110.1807724695661506 ) ) ;
#17164=CARTESIAN_POINT ( 'NONE',  ( 3.310556943750001313, 19.41135094264166128, -73.18077246956615056 ) ) ;
#17166=ORIENTED_EDGE ( 'NONE', *, *, #19787, .T. ) ;
#17167=CARTESIAN_POINT ( 'NONE',  ( 1.655278471874998436, 14.63297358603754716, -103.5182724695661278 ) ) ;
#17168=CARTESIAN_POINT ( 'NONE',  ( -1.749999999999999778, 20.53108891324555429, -100.8213974700440900 ) ) ;
#17170=CARTESIAN_POINT ( 'NONE',  ( 0.000000000000000000, 17.50000000000002487, -149.5231586289125687 ) ) ;
#17174=CARTESIAN_POINT ( 'NONE',  ( -3.310556943750002201, 15.58864905735836892, -59.68077246956614346 ) ) ;
#17175=( BOUNDED_CURVE ( )  B_SPLINE_CURVE ( 2, ( #28922, #39123, #9368, #205, #41919, #3606, #35734, #32331, #10002 ),
 .UNSPECIFIED., .F., .F. ) 
 B_SPLINE_CURVE_WITH_KNOTS ( ( 3, 2, 2, 2, 3 ),
 ( 0.4645833333333333481, 0.4652777777777777901, 0.4666666666666666741, 0.4680555555555555580, 0.4687500000000000000 ),
 .UNSPECIFIED. ) 
 CURVE ( )  GEOMETRIC_REPRESENTATION_ITEM ( )  RATIONAL_B_SPLINE_CURVE ( ( 0.9330127018922194093, 0.9330127018922194093, 1.000000000000000000, 0.8660254037844387076, 1.000000000000000000, 0.8660254037844387076, 1.000000000000000000, 0.9330127018922194093, 0.9330127018922194093 ) ) 
 REPRESENTATION_ITEM ( '' )  );
#17177=CARTESIAN_POINT ( 'NONE',  ( -3.310556943750000425, 19.41135094264166838, -115.8474391362327935 ) ) ;
#17178=CARTESIAN_POINT ( 'NONE',  ( -0.9378221735089136146, 14.00000000000001066, -117.7556390011600200 ) ) ;
#17181=ORIENTED_EDGE ( 'NONE', *, *, #27945, .F. ) ;
#17183=LINE ( 'NONE', #26757, #10384 ) ;
#17184=CARTESIAN_POINT ( 'NONE',  ( 3.310556943750001313, 19.41135094264166128, -68.18077246956613635 ) ) ;
#17186=ORIENTED_EDGE ( 'NONE', *, *, #8800, .T. ) ;
#17194=CARTESIAN_POINT ( 'NONE',  ( 3.310556943750001313, 19.41135094264167549, -135.1807724695661364 ) ) ;
#17195=CARTESIAN_POINT ( 'NONE',  ( 4.648177544792955347E-16, 21.00000000000002487, -131.9047308033774186 ) ) ;
#17196=CARTESIAN_POINT ( 'NONE',  ( -1.655278471874999990, 20.36702641396248481, -43.01827246956613493 ) ) ;
#17197=CARTESIAN_POINT ( 'NONE',  ( -3.500000000000002220, 15.47927405783633503, -110.8776474690881741 ) ) ;
#17198=CARTESIAN_POINT ( 'NONE',  ( -3.310556943750002645, 15.58864905735836537, -37.76827246956612782 ) ) ;
#17199=CARTESIAN_POINT ( 'NONE',  ( -3.310556943750000425, 19.41135094264166483, -100.9349391362328134 ) ) ;
#17201=CARTESIAN_POINT ( 'NONE',  ( -1.655278471874999990, 20.36702641396248481, -25.93077246956613990 ) ) ;
#17203=CARTESIAN_POINT ( 'NONE',  ( -3.500000000000002220, 15.47927405783632970, -103.8776474690881599 ) ) ;
#17204=CARTESIAN_POINT ( 'NONE',  ( 0.9378221735089128375, 21.00000000000003553, -124.2556390011600200 ) ) ;
#17205=CYLINDRICAL_SURFACE ( 'NONE', #24089, 3.499999999999999556 ) ;
#17206=CARTESIAN_POINT ( 'NONE',  ( -3.500000000000000888, 19.52072594216371115, -91.73806413671076143 ) ) ;
#17211=DIRECTION ( 'NONE',  ( -0.000000000000000000, 1.259100132267607459E-16, -1.000000000000000000 ) ) ;
#17212=CARTESIAN_POINT ( 'NONE',  ( 2.474675557024783212E-16, 21.54145188432739388, -53.21098080242150985 ) ) ;
#17216=ORIENTED_EDGE ( 'NONE', *, *, #32184, .F. ) ;
#17217=CARTESIAN_POINT ( 'NONE',  ( 3.500000000000001776, 19.52072594216370405, -42.07139747004409713 ) ) ;
#17219=CARTESIAN_POINT ( 'NONE',  ( -3.310556943750000425, 19.41135094264166128, -28.93493913623279568 ) ) ;
#17220=CARTESIAN_POINT ( 'NONE',  ( -0.9378221735089291577, 21.00000000000001776, -80.86007260463891555 ) ) ;
#17222=VECTOR ( 'NONE', #12652, 1000.000000000000000 ) ;
#17223=ADVANCED_FACE ( 'NONE', ( #2897 ), #2687, .T. ) ;
#17225=CARTESIAN_POINT ( 'NONE',  ( -3.500000000000000000, 19.52072594216370405, -33.73806413671076854 ) ) ;
#17227=CARTESIAN_POINT ( 'NONE',  ( 1.655278471875001101, 20.36702641396249192, -77.09743913623280775 ) ) ;
#17229=VERTEX_POINT ( 'NONE', #15672 ) ;
#17230=LINE ( 'NONE', #4246, #34267 ) ;
#17231=( BOUNDED_CURVE ( )  B_SPLINE_CURVE ( 2, ( #32727, #16173, #10624, #35511, #19344, #38911, #22952, #613, #39533 ),
 .UNSPECIFIED., .F., .T. ) 
 B_SPLINE_CURVE_WITH_KNOTS ( ( 3, 2, 2, 2, 3 ),
 ( 0.3062500000000000222, 0.3069444444444444642, 0.3083333333333333481, 0.3097222222222222321, 0.3104166666666666741 ),
 .UNSPECIFIED. ) 
 CURVE ( )  GEOMETRIC_REPRESENTATION_ITEM ( )  RATIONAL_B_SPLINE_CURVE ( ( 0.9330127018922194093, 0.9330127018922194093, 1.000000000000000000, 0.8660254037844387076, 1.000000000000000000, 0.8660254037844387076, 1.000000000000000000, 0.9330127018922194093, 0.9330127018922194093 ) ) 
 REPRESENTATION_ITEM ( '' )  );
#17232=CARTESIAN_POINT ( 'NONE',  ( -1.749999999999999778, 20.53108891324555074, -54.82139747004409713 ) ) ;
#17233=ORIENTED_EDGE ( 'NONE', *, *, #10968, .F. ) ;
#17235=CARTESIAN_POINT ( 'NONE',  ( 1.655278471874998436, 14.63297358603754539, -85.43077246956613635 ) ) ;
#17241=CARTESIAN_POINT ( 'NONE',  ( 3.310556943750001313, 17.50000000000002132, -125.2641058028994792 ) ) ;
#17244=CARTESIAN_POINT ( 'NONE',  ( -7.022189441860112050E-16, 13.67729811471671830, -54.60160580289946353 ) ) ;
#17245=CARTESIAN_POINT ( 'NONE',  ( 1.655278471874998436, 14.63297358603754894, -112.5182724695661420 ) ) ;
#17247=ORIENTED_EDGE ( 'NONE', *, *, #12848, .T. ) ;
#17248=CARTESIAN_POINT ( 'NONE',  ( -3.500000000000000888, 19.52072594216371826, -126.7380641367107614 ) ) ;
#17249=CARTESIAN_POINT ( 'NONE',  ( 1.655278471874998436, 14.63297358603754006, -41.43077246956614346 ) ) ;
#17250=CARTESIAN_POINT ( 'NONE',  ( -3.310556943750001313, 17.50000000000001421, -66.85160580289947063 ) ) ;
#17251=CARTESIAN_POINT ( 'NONE',  ( -1.750000000000002220, 14.46891108675448656, -117.7943141357548313 ) ) ;
#17252=CARTESIAN_POINT ( 'NONE',  ( -3.310556943750000425, 19.41135094264166838, -102.8474391362328220 ) ) ;
#17253=CARTESIAN_POINT ( 'NONE',  ( 4.648177544792955347E-16, 21.00000000000001421, -47.90473080337742573 ) ) ;
#17256=CARTESIAN_POINT ( 'NONE',  ( -0.9378221735089310451, 14.00000000000001599, -70.44938900211595012 ) ) ;
#17258=CARTESIAN_POINT ( 'NONE',  ( 2.474675557024783212E-16, 21.54145188432739388, -67.21098080242150274 ) ) ;
#17259=CARTESIAN_POINT ( 'NONE',  ( 4.286263797015737581E-16, 14.00000000000002487, -149.5231586289125687 ) ) ;
#17260=CARTESIAN_POINT ( 'NONE',  ( -3.310556943750001313, 17.50000000000001066, -35.76410580289947205 ) ) ;
#17261=CARTESIAN_POINT ( 'NONE',  ( -3.310556943750000425, 19.41135094264166483, -92.93493913623281344 ) ) ;
#17262=CARTESIAN_POINT ( 'NONE',  ( 2.474675557024783212E-16, 21.54145188432739388, -59.90473080337743994 ) ) ;
#17263=CARTESIAN_POINT ( 'NONE',  ( 3.310556943750001313, 19.41135094264166838, -111.2682724695661420 ) ) ;
#17264=CARTESIAN_POINT ( 'NONE',  ( -1.655278471875002211, 14.63297358603754184, -45.68493913623279923 ) ) ;
#17266=CARTESIAN_POINT ( 'NONE',  ( 4.648177544792955347E-16, 21.00000000000001776, -86.90473080337743284 ) ) ;
#17271=CARTESIAN_POINT ( 'NONE',  ( -1.655278471874999990, 20.36702641396249192, -93.93077246956613635 ) ) ;
#17272=CARTESIAN_POINT ( 'NONE',  ( 0.9378221735089281585, 14.00000000000001243, -62.66632260368298546 ) ) ;
#17275=CARTESIAN_POINT ( 'NONE',  ( -1.394453263437886604E-15, 14.00000000000001421, -57.71098080242150274 ) ) ;
#17278=CARTESIAN_POINT ( 'NONE',  ( 3.500000000000001332, 19.52072594216370405, -46.37764746908818125 ) ) ;
#17282=CARTESIAN_POINT ( 'NONE',  ( -1.655278471875002211, 14.63297358603754006, -29.59743913623280775 ) ) ;
#17284=EDGE_CURVE ( 'NONE', #3213, #7495, #5249, .T. ) ;
#17285=CARTESIAN_POINT ( 'NONE',  ( -3.500000000000000000, 19.52072594216371115, -78.73806413671076143 ) ) ;
#17286=ADVANCED_FACE ( 'NONE', ( #25870 ), #29043, .T. ) ;
#17291=CARTESIAN_POINT ( 'NONE',  ( 4.648177544792955347E-16, 21.00000000000001421, -57.21098080242150274 ) ) ;
#17293=CARTESIAN_POINT ( 'NONE',  ( -7.022189441860112050E-16, 13.67729811471672896, -141.5141058028994792 ) ) ;
#17294=CARTESIAN_POINT ( 'NONE',  ( 3.500000000000001332, 19.52072594216370760, -68.37764746908817415 ) ) ;
#17296=CARTESIAN_POINT ( 'NONE',  ( 2.340729813953370519E-16, 21.32270188528332255, -130.1016058028994280 ) ) ;
#17297=CARTESIAN_POINT ( 'NONE',  ( -3.500000000000002220, 15.47927405783632082, -29.87764746908818125 ) ) ;
#17300=CARTESIAN_POINT ( 'NONE',  ( -1.750000000000002220, 14.46891108675449011, -142.4880641367107614 ) ) ;
#17302=CARTESIAN_POINT ( 'NONE',  ( 2.474675557024783212E-16, 21.54145188432740810, -136.2109808024214885 ) ) ;
#17303=EDGE_CURVE ( 'NONE', #7031, #19419, #22880, .T. ) ;
#17304=CARTESIAN_POINT ( 'NONE',  ( -3.310556943750001313, 17.50000000000002132, -115.7641058028994792 ) ) ;
#17308=CARTESIAN_POINT ( 'NONE',  ( -3.500000000000000888, 19.52072594216371115, -88.04431413575483134 ) ) ;
#17311=CARTESIAN_POINT ( 'NONE',  ( 1.655278471875001101, 20.36702641396248836, -55.09743913623281486 ) ) ;
#17312=EDGE_CURVE ( 'NONE', #24647, #36594, #16467, .T. ) ;
#17313=CARTESIAN_POINT ( 'NONE',  ( 3.310556943750001313, 19.41135094264166838, -110.2682724695661420 ) ) ;
#17317=CARTESIAN_POINT ( 'NONE',  ( 3.310556943750001313, 19.41135094264166838, -127.2682724695661278 ) ) ;
#17321=CARTESIAN_POINT ( 'NONE',  ( 4.648177544792955347E-16, 21.00000000000001066, -29.21098080242150985 ) ) ;
#17322=CARTESIAN_POINT ( 'NONE',  ( -7.022189441860112050E-16, 13.67729811471671830, -64.60160580289945642 ) ) ;
#17324=CARTESIAN_POINT ( 'NONE',  ( 3.310556943750001313, 19.41135094264166838, -79.26827246956614204 ) ) ;
#17329=CARTESIAN_POINT ( 'NONE',  ( -3.310556943750001313, 17.50000000000001066, -44.76410580289947916 ) ) ;
#17330=CARTESIAN_POINT ( 'NONE',  ( 1.655278471875001101, 20.36702641396249192, -99.09743913623280775 ) ) ;
#17333=ORIENTED_EDGE ( 'NONE', *, *, #37303, .T. ) ;
#17337=CARTESIAN_POINT ( 'NONE',  ( -1.655278471875002211, 14.63297358603754361, -54.59743913623281486 ) ) ;
#17338=ORIENTED_EDGE ( 'NONE', *, *, #27687, .T. ) ;
#17340=DIRECTION ( 'NONE',  ( -0.000000000000000000, 1.259100132267607459E-16, -1.000000000000000000 ) ) ;
#17343=( BOUNDED_CURVE ( )  B_SPLINE_CURVE ( 2, ( #25159, #7949, #17726, #27515, #40483, #7215, #2598, #25784, #6212 ),
 .UNSPECIFIED., .F., .T. ) 
 B_SPLINE_CURVE_WITH_KNOTS ( ( 3, 2, 2, 2, 3 ),
 ( 0.5020833333333333259, 0.5027777777777777679, 0.5041666666666666519, 0.5055555555555555358, 0.5062499999999999778 ),
 .UNSPECIFIED. ) 
 CURVE ( )  GEOMETRIC_REPRESENTATION_ITEM ( )  RATIONAL_B_SPLINE_CURVE ( ( 0.9330127018922194093, 0.9330127018922194093, 1.000000000000000000, 0.8660254037844387076, 1.000000000000000000, 0.8660254037844387076, 1.000000000000000000, 0.9330127018922194093, 0.9330127018922194093 ) ) 
 REPRESENTATION_ITEM ( '' )  );
#17347=EDGE_LOOP ( 'NONE', ( #26761, #40197, #10373, #24980 ) ) ;
#17348=CARTESIAN_POINT ( 'NONE',  ( 3.500000000000001776, 19.52072594216370405, -42.37764746908817415 ) ) ;
#17349=CARTESIAN_POINT ( 'NONE',  ( 0.000000000000000000, 21.00000000000002487, -149.5231586289125687 ) ) ;
#17350=CARTESIAN_POINT ( 'NONE',  ( -0.9378221735089291577, 21.00000000000002132, -110.8600726046389013 ) ) ;
#17352=CARTESIAN_POINT ( 'NONE',  ( 2.340729813953370519E-16, 21.32270188528330479, -27.10160580289947063 ) ) ;
#17354=CARTESIAN_POINT ( 'NONE',  ( 1.655278471875001101, 20.36702641396249192, -82.18493913623278502 ) ) ;
#17355=CARTESIAN_POINT ( 'NONE',  ( -3.310556943750002645, 15.58864905735837780, -135.6807724695661364 ) ) ;
#17358=EDGE_CURVE ( 'NONE', #25161, #6975, #20828, .T. ) ;
#17359=CARTESIAN_POINT ( 'NONE',  ( -1.750000000000002220, 14.46891108675447590, -38.48806413671076854 ) ) ;
#17361=CARTESIAN_POINT ( 'NONE',  ( -3.310556943750002645, 15.58864905735837780, -128.7682724695661136 ) ) ;
#17362=CARTESIAN_POINT ( 'NONE',  ( -1.394453263437886604E-15, 14.00000000000001066, -42.71098080242150274 ) ) ;
#17363=CARTESIAN_POINT ( 'NONE',  ( 3.310556943750001313, 17.50000000000001776, -85.26410580289947916 ) ) ;
#17364=DIRECTION ( 'NONE',  ( 0.000000000000000000, 1.000000000000000000, 0.000000000000000000 ) ) ;
#17365=CYLINDRICAL_SURFACE ( 'NONE', #13731, 3.499999999999999556 ) ;
#17366=CARTESIAN_POINT ( 'NONE',  ( 3.500000000000001332, 17.50000000000001776, -89.15473080337743284 ) ) ;
#17367=CARTESIAN_POINT ( 'NONE',  ( 3.500000000000001776, 19.52072594216370760, -72.07139747004409003 ) ) ;
#17368=CARTESIAN_POINT ( 'NONE',  ( -1.655278471875002211, 14.63297358603754184, -51.68493913623279923 ) ) ;
#17370=CYLINDRICAL_SURFACE ( 'NONE', #39390, 3.499999999999999556 ) ;
#17371=CARTESIAN_POINT ( 'NONE',  ( -0.9378221735089291577, 21.00000000000001421, -49.16632260368299256 ) ) ;
#17372=CARTESIAN_POINT ( 'NONE',  ( 1.655278471874998436, 14.63297358603754361, -80.51827246956614204 ) ) ;
#17373=CARTESIAN_POINT ( 'NONE',  ( 3.310556943749999981, 15.58864905735837780, -141.4349391362327992 ) ) ;
#17375=CARTESIAN_POINT ( 'NONE',  ( 1.655278471875001101, 20.36702641396249547, -107.0974391362328078 ) ) ;
#17376=CARTESIAN_POINT ( 'NONE',  ( 1.655278471875001101, 20.36702641396249192, -78.09743913623280775 ) ) ;
#17378=CARTESIAN_POINT ( 'NONE',  ( -1.655278471874999990, 20.36702641396249192, -97.01827246956612782 ) ) ;
#17379=CARTESIAN_POINT ( 'NONE',  ( -3.500000000000001332, 17.50000000000001776, -99.65473080337743284 ) ) ;
#17380=AXIS2_PLACEMENT_3D ( 'NONE', #27205, #33360, #4229 ) ;
#17382=CARTESIAN_POINT ( 'NONE',  ( -0.9378221735089640188, 20.99999999999999645, -85.86007260463891555 ) ) ;
#17383=CARTESIAN_POINT ( 'NONE',  ( -0.9378221735089310451, 14.00000000000002132, -81.44938900211595012 ) ) ;
#17385=CARTESIAN_POINT ( 'NONE',  ( -3.310556943750001313, 17.50000000000001421, -59.76410580289947916 ) ) ;
#17386=CARTESIAN_POINT ( 'NONE',  ( -3.500000000000000000, 19.52072594216370760, -68.73806413671077564 ) ) ;
#17387=CARTESIAN_POINT ( 'NONE',  ( -1.655278471875002211, 14.63297358603755072, -116.5974391362327935 ) ) ;
#17388=CARTESIAN_POINT ( 'NONE',  ( 0.9378221735089281585, 14.00000000000000888, -36.66632260368297835 ) ) ;
#17391=ORIENTED_EDGE ( 'NONE', *, *, #25616, .F. ) ;
#17395=AXIS2_PLACEMENT_3D ( 'NONE', #31129, #40906, #24339 ) ;
#17396=CARTESIAN_POINT ( 'NONE',  ( 3.310556943750001313, 17.50000000000001421, -70.26410580289947916 ) ) ;
#17397=ORIENTED_EDGE ( 'NONE', *, *, #484, .T. ) ;
#17398=ORIENTED_EDGE ( 'NONE', *, *, #13695, .T. ) ;
#17400=EDGE_CURVE ( 'NONE', #26191, #8532, #688, .T. ) ;
#17401=DIRECTION ( 'NONE',  ( 0.000000000000000000, 1.000000000000000000, 0.000000000000000000 ) ) ;
#17407=CARTESIAN_POINT ( 'NONE',  ( 3.310556943750001313, 19.41135094264167549, -138.1807724695661364 ) ) ;
#17409=AXIS2_PLACEMENT_3D ( 'NONE', #14416, #30366, #7614 ) ;
#17410=CARTESIAN_POINT ( 'NONE',  ( 1.655278471874998436, 14.63297358603754006, -44.51827246956613493 ) ) ;
#17411=DIRECTION ( 'NONE',  ( 0.000000000000000000, 1.000000000000000000, 0.000000000000000000 ) ) ;
#17412=CARTESIAN_POINT ( 'NONE',  ( -3.310556943750002645, 15.58864905735836537, -38.76827246956612782 ) ) ;
#17413=ADVANCED_FACE ( 'NONE', ( #9491 ), #35435, .T. ) ;
#17414=CARTESIAN_POINT ( 'NONE',  ( 3.310556943750001313, 17.50000000000001776, -97.35160580289945642 ) ) ;
#17415=EDGE_CURVE ( 'NONE', #23990, #21195, #750, .T. ) ;
#17417=CARTESIAN_POINT ( 'NONE',  ( 3.310556943750001313, 19.41135094264167549, -142.2682724695661420 ) ) ;
#17418=CARTESIAN_POINT ( 'NONE',  ( 0.000000000000000000, 17.50000000000002487, -149.5231586289125687 ) ) ;
#17419=CARTESIAN_POINT ( 'NONE',  ( -1.750000000000002220, 14.46891108675448478, -97.79431413575484555 ) ) ;
#17420=CARTESIAN_POINT ( 'NONE',  ( 4.648177544792955347E-16, 21.00000000000002487, -132.2109808024214885 ) ) ;
#17422=CARTESIAN_POINT ( 'NONE',  ( 3.500000000000001332, 17.50000000000001776, -85.15473080337743284 ) ) ;
#17423=CARTESIAN_POINT ( 'NONE',  ( 1.655278471874998436, 14.63297358603754184, -67.51827246956612782 ) ) ;
#17424=( BOUNDED_CURVE ( )  B_SPLINE_CURVE ( 2, ( #25740, #35516, #19348, #32322, #3190, #28491, #12971, #35726, #9793 ),
 .UNSPECIFIED., .F., .T. ) 
 B_SPLINE_CURVE_WITH_KNOTS ( ( 3, 2, 2, 2, 3 ),
 ( 0.1854166666666666741, 0.1861111111111111160, 0.1875000000000000000, 0.1888888888888888840, 0.1895833333333333259 ),
 .UNSPECIFIED. ) 
 CURVE ( )  GEOMETRIC_REPRESENTATION_ITEM ( )  RATIONAL_B_SPLINE_CURVE ( ( 0.9330127018922194093, 0.9330127018922194093, 1.000000000000000000, 0.8660254037844387076, 1.000000000000000000, 0.8660254037844387076, 1.000000000000000000, 0.9330127018922194093, 0.9330127018922194093 ) ) 
 REPRESENTATION_ITEM ( '' )  );
#17428=CARTESIAN_POINT ( 'NONE',  ( 4.648177544792955347E-16, 21.00000000000002132, -120.2109808024215170 ) ) ;
#17429=CARTESIAN_POINT ( 'NONE',  ( -3.500000000000000888, 19.52072594216370760, -52.04431413575484555 ) ) ;
#17430=CARTESIAN_POINT ( 'NONE',  ( 4.648177544792955347E-16, 21.00000000000001421, -46.90473080337742573 ) ) ;
#17434=CARTESIAN_POINT ( 'NONE',  ( 3.500000000000000000, 15.47927405783632082, -45.23806413671076143 ) ) ;
#17435=CARTESIAN_POINT ( 'NONE',  ( 3.500000000000000000, 15.47927405783632437, -55.23806413671077564 ) ) ;
#17436=CARTESIAN_POINT ( 'NONE',  ( -3.310556943750002201, 15.58864905735836182, -23.76827246956612782 ) ) ;
#17437=CARTESIAN_POINT ( 'NONE',  ( 3.500000000000001332, 17.50000000000001776, -76.15473080337741862 ) ) ;
#17440=CARTESIAN_POINT ( 'NONE',  ( 3.500000000000001332, 17.50000000000002132, -120.1547308033774328 ) ) ;
#17442=CARTESIAN_POINT ( 'NONE',  ( 3.310556943749999981, 15.58864905735836714, -77.34743913623279354 ) ) ;
#17443=CARTESIAN_POINT ( 'NONE',  ( 4.648177544792955347E-16, 21.00000000000001776, -97.21098080242148853 ) ) ;
#17444=ORIENTED_EDGE ( 'NONE', *, *, #31399, .F. ) ;
#17445=CARTESIAN_POINT ( 'NONE',  ( 4.648177544792955347E-16, 21.00000000000001421, -74.21098080242151696 ) ) ;
#17447=VERTEX_POINT ( 'NONE', #20315 ) ;
#17448=EDGE_CURVE ( 'NONE', #2623, #30409, #27121, .T. ) ;
#17449=CARTESIAN_POINT ( 'NONE',  ( 4.648177544792955347E-16, 21.00000000000001421, -63.90473080337742573 ) ) ;
#17450=CARTESIAN_POINT ( 'NONE',  ( 3.310556943749999981, 15.58864905735836892, -84.34743913623280775 ) ) ;
#17451=ORIENTED_EDGE ( 'NONE', *, *, #15769, .F. ) ;
#17455=CARTESIAN_POINT ( 'NONE',  ( -3.500000000000001332, 17.50000000000001421, -58.96098080242151696 ) ) ;
#17456=CARTESIAN_POINT ( 'NONE',  ( -7.022189441860112050E-16, 13.67729811471672718, -128.5141058028994792 ) ) ;
#17457=CARTESIAN_POINT ( 'NONE',  ( -1.394453263437886604E-15, 14.00000000000001776, -94.71098080242150274 ) ) ;
#17458=CARTESIAN_POINT ( 'NONE',  ( -3.310556943750002645, 15.58864905735836892, -56.76827246956612782 ) ) ;
#17459=ADVANCED_FACE ( 'NONE', ( #14145 ), #33920, .T. ) ;
#17460=CARTESIAN_POINT ( 'NONE',  ( -7.022189441860112050E-16, 13.67729811471672718, -114.6016058028994564 ) ) ;
#17462=CARTESIAN_POINT ( 'NONE',  ( -1.749999999999999778, 20.53108891324555785, -126.8213974700440900 ) ) ;
#17463=CARTESIAN_POINT ( 'NONE',  ( -3.310556943750001313, 17.50000000000001066, -37.76410580289947205 ) ) ;
#17464=CARTESIAN_POINT ( 'NONE',  ( 1.655278471874998436, 14.63297358603754184, -65.51827246956614204 ) ) ;
#17465=CARTESIAN_POINT ( 'NONE',  ( -7.424026671074350129E-16, 13.45854811567263987, -119.7109808024215027 ) ) ;
#17466=CARTESIAN_POINT ( 'NONE',  ( -3.310556943750002645, 15.58864905735837247, -94.68077246956613635 ) ) ;
#17467=CARTESIAN_POINT ( 'NONE',  ( 0.000000000000000000, 17.50000000000002487, -149.5231586289125687 ) ) ;
#17469=CARTESIAN_POINT ( 'NONE',  ( -1.394453263437886604E-15, 14.00000000000001776, -83.71098080242150274 ) ) ;
#17471=CARTESIAN_POINT ( 'NONE',  ( -1.750000000000002220, 14.46891108675448123, -71.79431413575483134 ) ) ;
#17472=CARTESIAN_POINT ( 'NONE',  ( -0.9378221735089291577, 21.00000000000001066, -44.16632260368298546 ) ) ;
#17473=CARTESIAN_POINT ( 'NONE',  ( 3.310556943749999981, 15.58864905735836182, -32.34743913623280775 ) ) ;
#17474=( BOUNDED_CURVE ( )  B_SPLINE_CURVE ( 2, ( #8504, #21894, #37855, #5526, #18500, #31470, #8299, #21278, #34873 ),
 .UNSPECIFIED., .F., .T. ) 
 B_SPLINE_CURVE_WITH_KNOTS ( ( 3, 2, 2, 2, 3 ),
 ( 0.5937500000000000000, 0.5944444444444444420, 0.5958333333333333259, 0.5972222222222222099, 0.5979166666666666519 ),
 .UNSPECIFIED. ) 
 CURVE ( )  GEOMETRIC_REPRESENTATION_ITEM ( )  RATIONAL_B_SPLINE_CURVE ( ( 0.9330127018922194093, 0.9330127018922194093, 1.000000000000000000, 0.8660254037844387076, 1.000000000000000000, 0.8660254037844387076, 1.000000000000000000, 0.9330127018922194093, 0.9330127018922194093 ) ) 
 REPRESENTATION_ITEM ( '' )  );
#17475=CARTESIAN_POINT ( 'NONE',  ( -7.022189441860112050E-16, 13.67729811471672363, -91.60160580289947063 ) ) ;
#17476=CARTESIAN_POINT ( 'NONE',  ( -1.749999999999999778, 20.53108891324555074, -60.82139747004409713 ) ) ;
#17477=CARTESIAN_POINT ( 'NONE',  ( 3.310556943750001313, 19.41135094264166838, -114.2682724695661278 ) ) ;
#17478=CARTESIAN_POINT ( 'NONE',  ( 2.340729813953370519E-16, 21.32270188528330834, -42.10160580289947063 ) ) ;
#17484=CARTESIAN_POINT ( 'NONE',  ( 1.655278471874998436, 14.63297358603754539, -91.43077246956613635 ) ) ;
#17490=CARTESIAN_POINT ( 'NONE',  ( -0.9378221735089310451, 14.00000000000001599, -78.75563900116003424 ) ) ;
#17491=ORIENTED_EDGE ( 'NONE', *, *, #10829, .T. ) ;
#17495=ORIENTED_EDGE ( 'NONE', *, *, #13559, .F. ) ;
#17496=CARTESIAN_POINT ( 'NONE',  ( 4.648177544792955347E-16, 21.00000000000002132, -110.2109808024215170 ) ) ;
#17501=CARTESIAN_POINT ( 'NONE',  ( -0.9378221735089310451, 14.00000000000001066, -27.44938900211595012 ) ) ;
#17503=CARTESIAN_POINT ( 'NONE',  ( 3.500000000000001332, 19.52072594216371826, -137.0713974700441042 ) ) ;
#17504=CARTESIAN_POINT ( 'NONE',  ( -1.750000000000002220, 14.46891108675448123, -80.79431413575484555 ) ) ;
#17506=CARTESIAN_POINT ( 'NONE',  ( -3.310556943750000425, 19.41135094264167549, -131.9349391362328277 ) ) ;
#17507=CARTESIAN_POINT ( 'NONE',  ( 3.310556943750001313, 17.50000000000001421, -55.35160580289947063 ) ) ;
#17509=CARTESIAN_POINT ( 'NONE',  ( 1.749999999999998224, 14.46891108675448834, -140.3213974700441042 ) ) ;
#17511=CARTESIAN_POINT ( 'NONE',  ( -3.500000000000000888, 19.52072594216372181, -134.0443141357548598 ) ) ;
#17512=CARTESIAN_POINT ( 'NONE',  ( 3.310556943750001313, 17.50000000000002132, -120.2641058028994792 ) ) ;
#17514=DIRECTION ( 'NONE',  ( -0.000000000000000000, 1.259100132267607459E-16, -1.000000000000000000 ) ) ;
#17515=CARTESIAN_POINT ( 'NONE',  ( -1.749999999999999778, 20.53108891324555429, -88.12764746908817415 ) ) ;
#17517=CARTESIAN_POINT ( 'NONE',  ( -3.310556943750002645, 15.58864905735836714, -49.68077246956614346 ) ) ;
#17518=CARTESIAN_POINT ( 'NONE',  ( 3.310556943750001313, 17.50000000000002132, -105.3516058028994564 ) ) ;
#17519=EDGE_CURVE ( 'NONE', #36364, #34720, #14573, .T. ) ;
#17520=CARTESIAN_POINT ( 'NONE',  ( 1.749999999999998224, 14.46891108675448478, -111.3213974700441042 ) ) ;
#17521=CARTESIAN_POINT ( 'NONE',  ( 0.000000000000000000, 17.50000000000002487, -149.5231586289125687 ) ) ;
#17523=CARTESIAN_POINT ( 'NONE',  ( 1.655278471874998436, 14.63297358603755072, -128.5182724695661136 ) ) ;
#17526=CARTESIAN_POINT ( 'NONE',  ( 0.000000000000000000, 21.00000000000002487, -149.5231586289125687 ) ) ;
#17527=CARTESIAN_POINT ( 'NONE',  ( 3.500000000000000000, 15.47927405783632793, -86.23806413671077564 ) ) ;
#17528=CARTESIAN_POINT ( 'NONE',  ( 3.310556943749999981, 15.58864905735836537, -60.43493913623279212 ) ) ;
#17530=CARTESIAN_POINT ( 'NONE',  ( 3.310556943750001313, 17.50000000000001776, -80.35160580289945642 ) ) ;
#17532=CARTESIAN_POINT ( 'NONE',  ( 0.9378221735089300459, 21.00000000000001066, -25.94938900211595367 ) ) ;
#17535=CARTESIAN_POINT ( 'NONE',  ( 1.655278471875001101, 20.36702641396248481, -37.09743913623281486 ) ) ;
#17536=CARTESIAN_POINT ( 'NONE',  ( 1.655278471874998436, 14.63297358603754716, -101.4307724695661364 ) ) ;
#17540=ORIENTED_EDGE ( 'NONE', *, *, #7847, .T. ) ;
#17542=CARTESIAN_POINT ( 'NONE',  ( -1.655278471874999990, 20.36702641396248836, -50.93077246956613635 ) ) ;
#17543=EDGE_CURVE ( 'NONE', #29770, #9807, #13936, .T. ) ;
#17544=EDGE_LOOP ( 'NONE', ( #33049, #25329, #10990, #34730 ) ) ;
#17545=ORIENTED_EDGE ( 'NONE', *, *, #32630, .T. ) ;
#17546=CARTESIAN_POINT ( 'NONE',  ( -1.750000000000002220, 14.46891108675448478, -98.48806413671076143 ) ) ;
#17551=VERTEX_POINT ( 'NONE', #27548 ) ;
#17553=CARTESIAN_POINT ( 'NONE',  ( 1.749999999999998224, 14.46891108675447590, -46.62764746908818125 ) ) ;
#17554=CARTESIAN_POINT ( 'NONE',  ( -1.394453263437886604E-15, 14.00000000000001776, -97.40473080337741862 ) ) ;
#17559=CARTESIAN_POINT ( 'NONE',  ( -3.310556943750000425, 19.41135094264165772, -28.93493913623279568 ) ) ;
#17560=CARTESIAN_POINT ( 'NONE',  ( 4.648177544792955347E-16, 21.00000000000002132, -121.9047308033774044 ) ) ;
#17561=CARTESIAN_POINT ( 'NONE',  ( 1.655278471874998436, 14.63297358603754539, -84.51827246956612782 ) ) ;
#17562=CARTESIAN_POINT ( 'NONE',  ( 1.655278471875001101, 20.36702641396249902, -136.0974391362328220 ) ) ;
#17567=CARTESIAN_POINT ( 'NONE',  ( 2.340729813953370519E-16, 21.32270188528331900, -120.1016058028994706 ) ) ;
#17570=CARTESIAN_POINT ( 'NONE',  ( 1.655278471874998436, 14.63297358603754539, -84.43077246956613635 ) ) ;
#17571=CARTESIAN_POINT ( 'NONE',  ( 1.749999999999998224, 14.46891108675447590, -46.32139747004410424 ) ) ;
#17573=LINE ( 'NONE', #33303, #38362 ) ;
#17574=CARTESIAN_POINT ( 'NONE',  ( -1.655278471874999990, 20.36702641396248836, -56.01827246956612782 ) ) ;
#17577=CARTESIAN_POINT ( 'NONE',  ( 1.743066579297357930E-14, 14.00000000000002132, -129.4047308033774186 ) ) ;
#17578=CARTESIAN_POINT ( 'NONE',  ( 3.310556943750001313, 17.50000000000001776, -79.35160580289945642 ) ) ;
#17579=CARTESIAN_POINT ( 'NONE',  ( -7.022189441860112050E-16, 13.67729811471672896, -140.6016058028994564 ) ) ;
#17581=CARTESIAN_POINT ( 'NONE',  ( 1.655278471875001101, 20.36702641396249547, -102.0974391362328220 ) ) ;
#17582=CARTESIAN_POINT ( 'NONE',  ( 3.310556943750001313, 19.41135094264166483, -77.18077246956613635 ) ) ;
#17583=CARTESIAN_POINT ( 'NONE',  ( 4.648177544792955347E-16, 21.00000000000002132, -115.9047308033774328 ) ) ;
#17584=VERTEX_POINT ( 'NONE', #14360 ) ;
#17585=CARTESIAN_POINT ( 'NONE',  ( 1.655278471874998436, 14.63297358603754716, -98.51827246956612782 ) ) ;
#17587=CARTESIAN_POINT ( 'NONE',  ( -1.750000000000002220, 14.46891108675448301, -86.48806413671076143 ) ) ;
#17588=CARTESIAN_POINT ( 'NONE',  ( 3.500000000000001332, 17.50000000000001421, -51.15473080337743284 ) ) ;
#17589=CARTESIAN_POINT ( 'NONE',  ( 0.000000000000000000, 21.00000000000002487, -149.5231586289125687 ) ) ;
#17590=CARTESIAN_POINT ( 'NONE',  ( -1.655278471875002211, 14.63297358603754361, -59.59743913623280775 ) ) ;
#17591=CARTESIAN_POINT ( 'NONE',  ( 3.310556943749999981, 15.58864905735837247, -118.3474391362328078 ) ) ;
#17592=CARTESIAN_POINT ( 'NONE',  ( 3.500000000000001332, 19.52072594216371115, -84.37764746908818836 ) ) ;
#17594=( BOUNDED_CURVE ( )  B_SPLINE_CURVE ( 2, ( #16566, #15777, #28726, #23142, #3003, #41721, #10389, #815, #7197 ),
 .UNSPECIFIED., .F., .T. ) 
 B_SPLINE_CURVE_WITH_KNOTS ( ( 3, 2, 2, 2, 3 ),
 ( 0.01458333333333333356, 0.01527777777777777728, 0.01666666666666666644, 0.01805555555555555386, 0.01874999999999999931 ),
 .UNSPECIFIED. ) 
 CURVE ( )  GEOMETRIC_REPRESENTATION_ITEM ( )  RATIONAL_B_SPLINE_CURVE ( ( 0.9330127018922192983, 0.9330127018922194093, 1.000000000000000000, 0.8660254037844387076, 1.000000000000000000, 0.8660254037844387076, 1.000000000000000000, 0.9330127018922194093, 0.9330127018922194093 ) ) 
 REPRESENTATION_ITEM ( '' )  );
#17597=( BOUNDED_CURVE ( )  B_SPLINE_CURVE ( 2, ( #37452, #5321, #21489, #21286, #34461, #11695, #14495, #2130, #24483 ),
 .UNSPECIFIED., .F., .F. ) 
 B_SPLINE_CURVE_WITH_KNOTS ( ( 3, 2, 2, 2, 3 ),
 ( 0.7479166666666666741, 0.7486111111111111160, 0.7500000000000000000, 0.7513888888888888840, 0.7520833333333333259 ),
 .UNSPECIFIED. ) 
 CURVE ( )  GEOMETRIC_REPRESENTATION_ITEM ( )  RATIONAL_B_SPLINE_CURVE ( ( 0.9330127018922194093, 0.9330127018922194093, 1.000000000000000000, 0.8660254037844387076, 1.000000000000000000, 0.8660254037844387076, 1.000000000000000000, 0.9330127018922194093, 0.9330127018922194093 ) ) 
 REPRESENTATION_ITEM ( '' )  );
#17602=CARTESIAN_POINT ( 'NONE',  ( 3.310556943750001313, 17.50000000000001421, -69.26410580289947916 ) ) ;
#17604=ORIENTED_EDGE ( 'NONE', *, *, #34190, .T. ) ;
#17605=ADVANCED_FACE ( 'NONE', ( #23727 ), #11173, .T. ) ;
#17606=VERTEX_POINT ( 'NONE', #40513 ) ;
#17613=CARTESIAN_POINT ( 'NONE',  ( 1.655278471874998436, 14.63297358603755072, -134.4307724695661364 ) ) ;
#17614=CARTESIAN_POINT ( 'NONE',  ( -1.749999999999999778, 20.53108891324556140, -131.8213974700441042 ) ) ;
#17615=CARTESIAN_POINT ( 'NONE',  ( 1.655278471874998436, 14.63297358603754006, -46.51827246956613493 ) ) ;
#17617=CARTESIAN_POINT ( 'NONE',  ( 1.655278471875001101, 20.36702641396248481, -31.18493913623279923 ) ) ;
#17618=CARTESIAN_POINT ( 'NONE',  ( -3.310556943750001313, 17.50000000000001776, -98.85160580289947063 ) ) ;
#17620=CARTESIAN_POINT ( 'NONE',  ( -7.022189441860112050E-16, 13.67729811471671297, -23.51410580289947561 ) ) ;
#17621=CARTESIAN_POINT ( 'NONE',  ( -1.394453263437886604E-15, 14.00000000000002132, -121.7109808024215170 ) ) ;
#17622=CARTESIAN_POINT ( 'NONE',  ( -3.500000000000000888, 19.52072594216371115, -94.04431413575484555 ) ) ;
#17623=CARTESIAN_POINT ( 'NONE',  ( 0.9378221735089281585, 14.00000000000002309, -132.6663226036829712 ) ) ;
#17625=CARTESIAN_POINT ( 'NONE',  ( -3.500000000000001332, 17.50000000000001776, -85.65473080337743284 ) ) ;
#17626=CARTESIAN_POINT ( 'NONE',  ( 3.310556943750001313, 19.41135094264166483, -70.26827246956612782 ) ) ;
#17630=DIRECTION ( 'NONE',  ( 0.000000000000000000, 1.000000000000000000, 0.000000000000000000 ) ) ;
#17631=CARTESIAN_POINT ( 'NONE',  ( -1.749999999999999778, 20.53108891324555074, -47.12764746908818125 ) ) ;
#17632=CARTESIAN_POINT ( 'NONE',  ( -3.310556943750001313, 17.50000000000002132, -120.7641058028994792 ) ) ;
#17636=VECTOR ( 'NONE', #5983, 1000.000000000000000 ) ;
#17637=CARTESIAN_POINT ( 'NONE',  ( -1.750000000000002220, 14.46891108675448656, -114.4880641367107614 ) ) ;
#17640=CARTESIAN_POINT ( 'NONE',  ( -3.500000000000002220, 15.47927405783632970, -83.57139747004410424 ) ) ;
#17641=CARTESIAN_POINT ( 'NONE',  ( 3.500000000000000000, 15.47927405783632437, -61.23806413671076143 ) ) ;
#17644=CARTESIAN_POINT ( 'NONE',  ( -3.310556943750002201, 15.58864905735837070, -78.68077246956613635 ) ) ;
#17645=CARTESIAN_POINT ( 'NONE',  ( 4.648177544792955347E-16, 21.00000000000001776, -98.21098080242148853 ) ) ;
#17646=CARTESIAN_POINT ( 'NONE',  ( -0.9378221735089310451, 14.00000000000001599, -54.44938900211595723 ) ) ;
#17648=EDGE_CURVE ( 'NONE', #29085, #38828, #4623, .T. ) ;
#17649=CARTESIAN_POINT ( 'NONE',  ( -1.749999999999999778, 20.53108891324555074, -64.12764746908817415 ) ) ;
#17650=CARTESIAN_POINT ( 'NONE',  ( 2.340729813953370519E-16, 21.32270188528331190, -83.01410580289946495 ) ) ;
#17651=ORIENTED_EDGE ( 'NONE', *, *, #36562, .T. ) ;
#17652=ORIENTED_EDGE ( 'NONE', *, *, #6590, .T. ) ;
#17653=AXIS2_PLACEMENT_3D ( 'NONE', #40904, #2614, #41126 ) ;
#17656=CARTESIAN_POINT ( 'NONE',  ( -0.9378221735089310451, 14.00000000000001599, -58.75563900116003424 ) ) ;
#17659=DIRECTION ( 'NONE',  ( 0.000000000000000000, 1.000000000000000000, 0.000000000000000000 ) ) ;
#17660=CARTESIAN_POINT ( 'NONE',  ( -1.655278471874999990, 20.36702641396248836, -52.01827246956612782 ) ) ;
#17661=CARTESIAN_POINT ( 'NONE',  ( 3.310556943749999981, 15.58864905735837247, -115.4349391362327850 ) ) ;
#17662=ORIENTED_EDGE ( 'NONE', *, *, #9679, .F. ) ;
#17663=( BOUNDED_CURVE ( )  B_SPLINE_CURVE ( 2, ( #40732, #11588, #40532, #30961, #1817, #2234, #8197, #34143, #30749 ),
 .UNSPECIFIED., .F., .F. ) 
 B_SPLINE_CURVE_WITH_KNOTS ( ( 3, 2, 2, 2, 3 ),
 ( 0.1062499999999999972, 0.1069444444444444392, 0.1083333333333333370, 0.1097222222222222210, 0.1104166666666666630 ),
 .UNSPECIFIED. ) 
 CURVE ( )  GEOMETRIC_REPRESENTATION_ITEM ( )  RATIONAL_B_SPLINE_CURVE ( ( 0.9330127018922194093, 0.9330127018922194093, 1.000000000000000000, 0.8660254037844387076, 1.000000000000000000, 0.8660254037844387076, 1.000000000000000000, 0.9330127018922194093, 0.9330127018922194093 ) ) 
 REPRESENTATION_ITEM ( '' )  );
#17664=CARTESIAN_POINT ( 'NONE',  ( -3.500000000000001332, 17.50000000000002132, -123.6547308033774186 ) ) ;
#17665=CARTESIAN_POINT ( 'NONE',  ( 2.340729813953370519E-16, 21.32270188528330479, -42.01410580289947916 ) ) ;
#17666=CARTESIAN_POINT ( 'NONE',  ( -1.655278471875002211, 14.63297358603754361, -64.68493913623279923 ) ) ;
#17667=CARTESIAN_POINT ( 'NONE',  ( -1.750000000000002220, 14.46891108675448656, -113.7943141357548456 ) ) ;
#17669=CARTESIAN_POINT ( 'NONE',  ( 2.340729813953370519E-16, 21.32270188528331190, -98.01410580289947916 ) ) ;
#17670=DIRECTION ( 'NONE',  ( -0.000000000000000000, 1.259100132267607459E-16, -1.000000000000000000 ) ) ;
#17672=CARTESIAN_POINT ( 'NONE',  ( 4.286263797015737581E-16, 14.00000000000002487, -149.5231586289125687 ) ) ;
#17674=CARTESIAN_POINT ( 'NONE',  ( -1.749999999999999778, 20.53108891324555074, -65.12764746908818836 ) ) ;
#17675=VECTOR ( 'NONE', #20288, 1000.000000000000000 ) ;
#17676=DIRECTION ( 'NONE',  ( 0.000000000000000000, 1.000000000000000000, 0.000000000000000000 ) ) ;
#17677=CARTESIAN_POINT ( 'NONE',  ( -7.022189441860112050E-16, 13.67729811471671475, -30.51410580289946495 ) ) ;
#17678=CARTESIAN_POINT ( 'NONE',  ( 3.310556943750001313, 17.50000000000001776, -90.35160580289947063 ) ) ;
#17679=CARTESIAN_POINT ( 'NONE',  ( 3.500000000000000000, 15.47927405783632082, -53.23806413671076854 ) ) ;
#17680=CARTESIAN_POINT ( 'NONE',  ( 3.310556943750001313, 17.50000000000002132, -113.3516058028994564 ) ) ;
#17681=CARTESIAN_POINT ( 'NONE',  ( 1.655278471875001101, 20.36702641396248481, -40.18493913623280633 ) ) ;
#17683=DIRECTION ( 'NONE',  ( 0.000000000000000000, 1.000000000000000000, 0.000000000000000000 ) ) ;
#17687=CARTESIAN_POINT ( 'NONE',  ( -1.394453263437886604E-15, 14.00000000000001421, -61.71098080242150985 ) ) ;
#17688=CARTESIAN_POINT ( 'NONE',  ( -3.310556943750000425, 19.41135094264166838, -93.84743913623282197 ) ) ;
#17689=CARTESIAN_POINT ( 'NONE',  ( 1.749999999999998224, 14.46891108675448478, -117.3213974700440900 ) ) ;
#17691=EDGE_LOOP ( 'NONE', ( #32449, #38812, #36681, #12829 ) ) ;
#17692=CYLINDRICAL_SURFACE ( 'NONE', #31497, 3.499999999999999556 ) ;
#17695=CYLINDRICAL_SURFACE ( 'NONE', #16881, 3.499999999999999556 ) ;
#17696=VERTEX_POINT ( 'NONE', #36479 ) ;
#17697=EDGE_CURVE ( 'NONE', #14819, #22244, #18946, .T. ) ;
#17700=CARTESIAN_POINT ( 'NONE',  ( -1.394453263437886604E-15, 14.00000000000002132, -118.4047308033774328 ) ) ;
#17706=CARTESIAN_POINT ( 'NONE',  ( -1.749999999999999778, 20.53108891324555074, -54.12764746908817415 ) ) ;
#17708=CARTESIAN_POINT ( 'NONE',  ( 0.000000000000000000, 17.50000000000002487, -149.5231586289125687 ) ) ;
#17710=CARTESIAN_POINT ( 'NONE',  ( 1.655278471874998436, 14.63297358603755072, -130.5182724695661136 ) ) ;
#17711=CARTESIAN_POINT ( 'NONE',  ( 1.655278471874998436, 14.63297358603754184, -54.51827246956612782 ) ) ;
#17712=ORIENTED_EDGE ( 'NONE', *, *, #8959, .T. ) ;
#17714=CARTESIAN_POINT ( 'NONE',  ( -1.749999999999999778, 20.53108891324556140, -141.8213974700441042 ) ) ;
#17715=( BOUNDED_CURVE ( )  B_SPLINE_CURVE ( 2, ( #4800, #4387, #21171, #40328, #11190, #24175, #37144, #7997, #17985, #4169, #34144, #17778, #1614, #27566, #40534, #11389, #17151, #37344, #19031, #34770, #18616, #5850, #18401, #15005, #32000, #11802, #21801, #6053, #24797, #25209, #31580, #2235, #9033, #40948, #41584, #21380, #2866, #34359, #37760, #37966, #12012, #9249, #25004, #2447, #5424, #27969, #15217, #28179, #12439, #25423, #38387, #28384, #41165, #15856, #22220, #21588, #31372, #2652, #28803, #5639, #15431, #8401, #34986, #5217, #18820, #41800, #41372, #15640, #12221, #8827, #8615, #34562, #38171, #35187, #18192, #22013, #12654, #37547, #31780, #31161, #2021, #28597, #295, #22426, #9459, #3284, #3907, #36230, #25840, #23262, #13277, #22641, #29854, #6480, #3485, #13066, #6268, #9892, #38805, #12860, #19650, #504, #32417, #7103, #19242, #13476, #26048, #16270, #32215, #6679, #720, #9678, #39011, #22848, #29211, #35403, #25633, #26260, #16889, #39208, #26462, #10089, #23052, #36021, #3080, #20078, #19451, #35818, #33041, #86, #6884, #35617, #32619, #16475, #38594, #29424, #19859, #39416, #16071, #29013, #32826, #3695, #10293, #42009, #16683, #29640, #4332, #37297, #27519, #39853, #7529, #20919, #8152, #40061, #7743, #10507, #20717, #1151, #24328, #27094, #33470, #33893, #4544, #10929, #33251, #939, #20500, #11341, #26672, #23913, #17938, #34098, #33693, #21127, #30916, #36881, #23700, #4752, #17523, #4956, #13691, #39633, #13905, #23488, #30488, #10713, #36451, #36664, #1357, #14119, #7314, #14330, #26886, #17317, #27310, #40276, #11145, #24129, #37097, #20285, #4116, #30278, #17101, #7953, #30063, #17729, #30700, #1569, #14547, #40487, #1774, #2399, #35142, #15388, #18774, #27922, #18561, #31531, #28337, #24534, #25374, #14956, #5590, #31324, #8984, #34931, #21749, #34721, #40896, #8569, #38334, #37917, #31117, #18350, #41322, #28547, #25162, #9196, #41116, #24958, #34513, #24747, #21336, #22172, #18146, #28130, #12389, #1970, #12171, #8776, #21544, #38127, #5174, #5802, #27713, #6004, #40686, #11751, #2183, #15165, #14757, #31734, #11964, #2602, #5372, #18980, #37500, #15588, #21957, #41535, #8356, #11542, #34310, #37713, #3233, #16216, #22588, #15801, #31947, #32566, #23208, #16018, #39360, #3433, #36175, #29160, #12601, #26408, #9410, #3025, #35769, #19397, #39156, #22998, #9839, #22798, #28960, #38754, #10239, #25997, #19190, #32369, #6629, #19593, #6832, #22374, #16425, #29588, #240, #12804, #35352, #7046, #6216, #38, #452, #32162, #29372, #13018, #9624, #13223, #41956, #25788, #35563, #38962, #6426, #26209, #13423, #2818, #3640, #10037, #35968, #19805, #32774, #16629, #28749, #41745, #25582, #38543, #10879, #10668, #1513, #36398, #20025, #1101, #883, #7264, #14279, #37041, #32989, #17477, #29798, #1306, #14492, #27046, #27259, #23864, #33416, #39579, #20237, #26833, #17680, #33198, #4062, #27463, #40220, #30010, #11091, #36612, #23649, #36828, #16836, #3857, #39804, #40429, #30648, #17047, #11288, #7689, #13854, #24273, #7476, #20450, #4281, #37243, #26619, #17263, #20662, #7901, #30226, #33641, #4495, #30437, #663, #13636, #14073, #40008, #10454, #24075, #20870, #33840, #4700, #23432, #14895, #2549, #2127, #37449, #24691, #24900, #34878, #31475, #31680, #5318, #31264, #40840, #18505, #25105, #21690, #1915, #12328, #4904, #15533, #11692, #30858, #5532, #24480, #21898, #27864, #8304, #8510, #37652, #21486, #18721, #28487, #5745, #34458, #15111, #18093, #27659, #18291, #28073, #38069, #41480, #8927, #40630, #25312, #2341, #21283, #8097, #41053, #31063, #34253, #15328, #21075, #34048, #28282, #17885, #41267, #1720, #11905, #12111, #37859, #14701, #8717, #5113, #11489, #34664, #26112, #9954, #20350, #16951, #6743, #3970, #13340, #29491, #13541, #35087, #22116, #16541, #17167, #7375, #39070, #29918, #10149, #10575, #7173, #23337, #362, #22914, #33317, #3346, #35878, #789, #26322, #13763, #3546, #4184, #18922, #26742, #39269, #23118, #16334, #38274, #10361, #19717, #9140, #39702, #30128, #32685, #36085, #5948, #1005, #13129, #6954, #13973, #19929, #26529, #32894, #3759, #36298, #148, #23554, #16744, #29707, #570, #39487, #31890, #29275, #36514, #20143, #33103, #36945, #4400, #33753, #4606, #1830, #14809, #27775, #17789, #17585, #8413, #40745, #26952, #8008, #7807, #1212, #21181, #11601, #39914, #24385, #36726, #8209, #21390, #33953, #34157, #30762, #40341, #17378, #14179, #30550, #24595, #10776, #40123, #34370, #5015, #20782, #17996, #1419, #14392, #1624, #23759, #7588, #27368, #5228, #37560, #27156, #18204, #14603, #23978, #31172, #11203, #4812, #10991, #2033, #33539, #24187, #30973, #37157, #20564, #20979, #30339, #27577, #40544, #11400, #37354, #21598, #38181, #32223, #15228, #28397, #41383, #5651, #25015, #41176, #11812, #9046, #12022, #22435, #15650, #6276, #12232, #37770, #9469, #34572, #28189, #18831, #2456, #22229, #6063, #34996, #5859, #37976, #31791, #12451, #38397, #18626, #15442, #2663, #28608, #32011, #5435, #41594, #12664, #25434, #8836, #18413, #21813, #34781, #24809, #22023, #31590, #35414, #9259, #35198, #19042, #8625, #38604, #25220, #2876, #19252, #15868, #28813, #2247, #41810, #25643, #15016, #27979, #40960, #31382, #6688, #3494, #19867, #26470, #26680, #304, #26269, #35826, #13484, #20086, #16692, #39017, #7323, #42019, #10515, #23061, #19658, #25850, #512, #19459, #16896, #9901, #3292, #29023, #32427, #16483, #32629, #3089, #39426, #29862, #12870, #23496, #39216, #16279, #26059, #39642, #728, #3916, #22651, #33050, #10302, #29220, #16081, #23271, #36459, #29434, #10097, #38814, #36030, #13285, #13701, #6895, #22856, #32834, #3703, #29648, #36238, #13074, #95, #9688, #20293, #7111, #35626, #6489, #1158, #40493, #7751, #23921, #7960, #30071, #17109, #10937, #11549, #1781, #33478, #30923, #20928, #30286, #37508, #14126, #11152, #20725, #13913, #39860, #27102, #37305, #33701, #8159, #40070, #14764, #26893, #21134, #4552, #36888, #10721, #14340, #8363, #4341, #17530, #30495, #1365, #947, #27319, #40283, #24136, #33259, #27526, #4964, #23708, #24542, #37106, #17324, #33900, #27723, #17945, #34107, #36672, #40693, #11350, #7536, #4124, #4759, #17737, #30711, #1576, #20509, #14553, #24335, #31956, #34731, #41125, #5599, #15173, #21758, #41544, #31332, #18360, #18153, #28758, #8577, #34522, #2826, #12397, #15811, #38552, #18571, #2192, #25383, #31539, #41754, #12610, #22182, #1979, #38343, #28556, #2408, #35151, #31742, #5810, #24967, #5381, #25592, #27931, #21551, #15395, #28347, #34941, #38135, #21966, #21344, #34317, #41332, #12180, #28139, #5181, #18784, #11973, #31125, #9206, #14963, #37926, #8786, #40903, #2613, #6014, #25172, #8993, #15597, #18990, #11759, #24756, #37722, #11240, #37601, #7850, #30802, #1252, #20820, #36989, #11642, #4850, #11435, #37395, #30592, #1662, #40789, #8251, #8456, #24222, #37192, #4647, #24427, #31013, #27612, #33792, #18241, #10817, #21435, #33996, #17626, #36767, #21227, #30382, #18037, #39953, #34408, #1460, #24638, #5268, #27817, #14434, #21020, #24017, #33583, #27409, #40379, #1867, #14847, #31213, #17828, #8046, #14019, #26990, #23803, #14649, #40580, #14222, #34198, #7630, #20604, #5058, #4444, #17423, #27201, #40166, #11033, #35037, #15482, #21635, #31422, #8878, #41855, #15058, #15272, #25684, #22268, #12060, #9303, #18668, #34825, #18872, #41002, #28023, #21849, #22475, #12706, #2288, #38645, #31837, #25052, #6317, #38014, #22066, #28231, #9513, #8663, #5692, #6103, #31631, #19083, #2496, #35456, #24851, #32050, #28436, #41425, #34613, #25258, #19292, #12274, #38225, #9087, #5898, #2706, #15692, #11852, #28648, #41638, #2074, #12491, #37808, #25477, #5477, #18454, #38441, #35241, #2919, #15908, #28855, #23326, #10138, #23106, #16323, #36074, #29695, #13529, #35866, #32673, #6942, #19918, #7161, #22693, #32883, #29907, #559, #13120, #9733, #26730, #6534, #16530, #777, #19500, #3748, #12913, #26517, #32471, #3959, #26102, #3335, #3535, #6731, #29265, #13752, #16733, #137, #36504, #39060, #39476, #19705, #25891, #29480, #9944, #22902, #26311, #10350, #36287, #20131, #7365, #10564, #39258, #350, #13328, #32267, #33092, #16939, #3133, #39691, #23544, #16124, #29064, #42058, #38856, #35670, #4390, #37147, #7999, #33943, #994, #1822, #14167, #17574, #14801, #27144, #20970, #7578, #40111, #1201, #17988, #11193, #17781, #1616, #23967, #20771, #5007, #14595, #27766, #30538, #1407, #10980, #30752, #37346, #4802, #36934, #24587, #17154, #40736, #40330, #7796, #13962, #27569, #36714, #34149, #33741, #11592, #4171, #20552, #4595, #14381, #20338, #40536, #30965, #30118, #37551, #27357, #33528, #24177, #33305, #26941, #21173, #39902, #8200, #11392, #17368, #24377, #10765, #23747, #30329, #2450, #5220, #15435, #37968, #19034, #21803, #28181, #34773, #2238, #8829, #28600, #18404, #5426, #18196, #15860, #37762, #12657, #28806, #28389, #32003, #25636, #5642, #31374, #41587, #18618, #2869, #41803, #9252, #31164, #8405, #21383, #22223, #25006, #41375, #15219, #27971, #8617, #41168, #34362, #35190, #6056, #40951, #25426, #2656, #24800, #2024, #31582, #12014, #21590, #15642, #38390, #15007, #5853, #11804, #31784, #34564, #12224, #25212, #38174, #12443, #9038, #22016, #34989, #18823, #25843, #9682, #20663, #17264, #6483, #4282, #13637, #29799, #13855, #35407, #22429, #16837, #40009, #19246, #30227, #1102, #10455, #10880, #7477, #23650, #664, #22644, #7690, #3083, #35620, #14074, #26620, #27047, #3858, #33642, #32217, #23865, #4063, #7265, #38808, #38597, #10669, #20026, #9462, #36829, #4496, #32990, #39580, #6271, #33199, #23434, #17478, #39805, #30438, #36399, #16074, #1307, #20238, #17048, #14280, #30011, #26834, #884, #36613, #20451, #29016, #33417, #42012, #12863, #30859, #27660, #1916, #31064, #2128, #17681, #18094, #24901, #37653, #15112, #40841, #21076, #31476, #24076, #34665, #5114, #1721, #7902, #24692, #1514, #41055, #34049, #27464, #40631, #14702, #4905, #11092, #5533, #17886, #11490, #28075, #11906, #37860, #14896, #24481, #8718, #21691, #11289, #37450, #34459, #18506, #8305, #21284, #37042, #34254, #27865, #2343, #11693, #8511, #5319, #21487, #18292, #4701, #14493, #31265, #27260, #40221, #20871, #33841, #30649, #40430, #24274, #37244, #8098, #25313, #35513, #12543, #9790, #35723, #25948, #15534, #12968, #32107, #12329, #19550, #38275, #35298, #2759, #38070, #41689, #28488, #2550, #9356, #22322, #28911, #2972, #15962, #32522, #6162, #25529, #41481, #15330, #41908, #9141, #28283, #6373, #38912, #22117, #35089, #12112, #19139, #5950, #22748, #12756, #6585, #38493, #8928, #41268, #18923, #25737, #25106, #31891, #38702, #15744, #28696, #9572, #21899, #22530, #19345, #32319, #3187, #16174, #29114, #42113, #34879, #5746, #18723, #31682, #13812, #20405, #17002, #39314, #7642, #192, #10831, #23388, #7001, #26160, #838, #19762, #17219, #10194, #3593, #3811, #19980, #23164, #14031, #39965, #39757, #30183, #36129, #20616, #13174, #23816, #36351, #32944, #39112, #26794, #32728, #1056, #16792, #16586, #29753, #614, #13590, #27003, #36782, #3391, #16379, #29323, #9991, #39534, #29542, #26363, #22953, #35921, #4238, #6787, #33369, #10626, #407, #13383, #26574, #10411, #7222, #23604, #20195, #33154, #4019, #29965, #36565, #7430, #14235, #30394, #1267, #11047, #27214, #40177, #33595, #4455, #24029, #37001, #17436, #7862, #41525, #38742, #5994, #22162 ),
 .UNSPECIFIED., .F., .T. ) 
 B_SPLINE_CURVE_WITH_KNOTS ( ( 3, 2, 2, 2, 2, 2, 2, 2, 2, 2, 2, 2, 2, 2, 2, 2, 2, 2, 2, 2, 2, 2, 2, 2, 2, 2, 2, 2, 2, 2, 2, 2, 2, 2, 2, 2, 2, 2, 2, 2, 2, 2, 2, 2, 2, 2, 2, 2, 2, 2, 2, 2, 2, 2, 2, 2, 2, 2, 2, 2, 2, 2, 2, 2, 2, 2, 2, 2, 2, 2, 2, 2, 2, 2, 2, 2, 2, 2, 2, 2, 2, 2, 2, 2, 2, 2, 2, 2, 2, 2, 2, 2, 2, 2, 2, 2, 2, 2, 2, 2, 2, 2, 2, 2, 2, 2, 2, 2, 2, 2, 2, 2, 2, 2, 2, 2, 2, 2, 2, 2, 2, 2, 2, 2, 2, 2, 2, 2, 2, 2, 2, 2, 2, 2, 2, 2, 2, 2, 2, 2, 2, 2, 2, 2, 2, 2, 2, 2, 2, 2, 2, 2, 2, 2, 2, 2, 2, 2, 2, 2, 2, 2, 2, 2, 2, 2, 2, 2, 2, 2, 2, 2, 2, 2, 2, 2, 2, 2, 2, 2, 2, 2, 2, 2, 2, 2, 2, 2, 2, 2, 2, 2, 2, 2, 2, 2, 2, 2, 2, 2, 2, 2, 2, 2, 2, 2, 2, 2, 2, 2, 2, 2, 2, 2, 2, 2, 2, 2, 2, 2, 2, 2, 2, 2, 2, 2, 2, 2, 2, 2, 2, 2, 2, 2, 2, 2, 2, 2, 2, 2, 2, 2, 2, 2, 2, 2, 2, 2, 2, 2, 2, 2, 2, 2, 2, 2, 2, 2, 2, 2, 2, 2, 2, 2, 2, 2, 2, 2, 2, 2, 2, 2, 2, 2, 2, 2, 2, 2, 2, 2, 2, 2, 2, 2, 2, 2, 2, 2, 2, 2, 2, 2, 2, 2, 2, 2, 2, 2, 2, 2, 2, 2, 2, 2, 2, 2, 2, 2, 2, 2, 2, 2, 2, 2, 2, 2, 2, 2, 2, 2, 2, 2, 2, 2, 2, 2, 2, 2, 2, 2, 2, 2, 2, 2, 2, 2, 2, 2, 2, 2, 2, 2, 2, 2, 2, 2, 2, 2, 2, 2, 2, 2, 2, 2, 2, 2, 2, 2, 2, 2, 2, 2, 2, 2, 2, 2, 2, 2, 2, 2, 2, 2, 2, 2, 2, 2, 2, 2, 2, 2, 2, 2, 2, 2, 2, 2, 2, 2, 2, 2, 2, 2, 2, 2, 2, 2, 2, 2, 2, 2, 2, 2, 2, 2, 2, 2, 2, 2, 2, 2, 2, 2, 2, 2, 2, 2, 2, 2, 2, 2, 2, 2, 2, 2, 2, 2, 2, 2, 2, 2, 2, 2, 2, 2, 2, 2, 2, 2, 2, 2, 2, 2, 2, 2, 2, 2, 2, 2, 2, 2, 2, 2, 2, 2, 2, 2, 2, 2, 2, 2, 2, 2, 2, 2, 2, 2, 2, 2, 2, 2, 2, 2, 2, 2, 2, 2, 2, 2, 2, 2, 2, 2, 2, 2, 2, 2, 2, 2, 2, 2, 2, 2, 2, 2, 2, 2, 2, 2, 2, 2, 2, 2, 2, 2, 2, 2, 2, 2, 2, 2, 2, 2, 2, 2, 2, 2, 2, 2, 2, 2, 2, 2, 2, 2, 2, 2, 2, 2, 2, 2, 2, 2, 2, 2, 2, 2, 2, 2, 2, 2, 2, 2, 2, 2, 2, 2, 2, 2, 2, 2, 2, 2, 2, 2, 2, 2, 2, 2, 2, 2, 2, 2, 2, 2, 2, 2, 2, 2, 2, 2, 2, 2, 2, 2, 2, 2, 2, 2, 2, 2, 2, 2, 2, 2, 2, 2, 2, 2, 2, 2, 2, 2, 2, 2, 2, 2, 2, 2, 2, 2, 2, 2, 2, 2, 2, 2, 2, 2, 2, 2, 2, 2, 2, 2, 2, 2, 2, 2, 2, 2, 2, 2, 2, 2, 2, 2, 2, 2, 2, 2, 2, 2, 2, 2, 2, 2, 2, 2, 2, 2, 2, 2, 2, 2, 2, 2, 2, 2, 2, 2, 2, 2, 2, 2, 2, 2, 2, 2, 2, 2, 2, 2, 2, 2, 2, 2, 2, 2, 2, 2, 2, 2, 2, 2, 2, 2, 2, 2, 2, 2, 2, 2, 2, 2, 2, 2, 2, 2, 2, 2, 2, 2, 2, 2, 2, 2, 2, 2, 2, 2, 2, 2, 2, 2, 2, 2, 2, 2, 2, 2, 2, 2, 2, 2, 2, 2, 2, 2, 2, 2, 3 ),
 ( 0.000000000000000000, 0.001388888888888888942, 0.002777777777777777884, 0.004166666666666666609, 0.005555555555555555768, 0.006944444444444444059, 0.008333333333333333218, 0.009722222222222222376, 0.01111111111111111154, 0.01250000000000000069, 0.01388888888888888812, 0.01527777777777777728, 0.01666666666666666644, 0.01805555555555555386, 0.01944444444444444475, 0.02083333333333333218, 0.02222222222222222307, 0.02361111111111111049, 0.02500000000000000139, 0.02638888888888888881, 0.02777777777777777624, 0.02916666666666666713, 0.03055555555555555455, 0.03194444444444444198, 0.03333333333333333287, 0.03472222222222222376, 0.03611111111111110772, 0.03749999999999999861, 0.03888888888888888951, 0.04027777777777778040, 0.04166666666666666435, 0.04305555555555555525, 0.04444444444444444614, 0.04583333333333333010, 0.04722222222222222099, 0.04861111111111111188, 0.05000000000000000278, 0.05138888888888888673, 0.05277777777777777762, 0.05416666666666666852, 0.05555555555555555247, 0.05694444444444444337, 0.05833333333333333426, 0.05972222222222222515, 0.06111111111111110911, 0.06250000000000000000, 0.06388888888888888395, 0.06527777777777778179, 0.06666666666666666574, 0.06805555555555554970, 0.06944444444444444753, 0.07083333333333333148, 0.07222222222222221544, 0.07361111111111111327, 0.07499999999999999722, 0.07638888888888889506, 0.07777777777777777901, 0.07916666666666666297, 0.08055555555555556080, 0.08194444444444444475, 0.08333333333333332871, 0.08472222222222222654, 0.08611111111111111049, 0.08749999999999999445, 0.08888888888888889228, 0.09027777777777777624, 0.09166666666666666019, 0.09305555555555555802, 0.09444444444444444198, 0.09583333333333333981, 0.09722222222222222376, 0.09861111111111110772, 0.1000000000000000056, 0.1013888888888888895, 0.1027777777777777735, 0.1041666666666666713, 0.1055555555555555552, 0.1069444444444444392, 0.1083333333333333370, 0.1097222222222222210, 0.1111111111111111049, 0.1125000000000000028, 0.1138888888888888867, 0.1152777777777777846, 0.1166666666666666685, 0.1180555555555555525, 0.1194444444444444503, 0.1208333333333333343, 0.1222222222222222182, 0.1236111111111111160, 0.1250000000000000000, 0.1263888888888888840, 0.1277777777777777679, 0.1291666666666666796, 0.1305555555555555636, 0.1319444444444444475, 0.1333333333333333315, 0.1347222222222222154, 0.1361111111111110994, 0.1375000000000000111, 0.1388888888888888951, 0.1402777777777777790, 0.1416666666666666630, 0.1430555555555555469, 0.1444444444444444309, 0.1458333333333333426, 0.1472222222222222265, 0.1486111111111111105, 0.1499999999999999944, 0.1513888888888888784, 0.1527777777777777901, 0.1541666666666666741, 0.1555555555555555580, 0.1569444444444444420, 0.1583333333333333259, 0.1597222222222222099, 0.1611111111111111216, 0.1625000000000000056, 0.1638888888888888895, 0.1652777777777777735, 0.1666666666666666574, 0.1680555555555555691, 0.1694444444444444531, 0.1708333333333333370, 0.1722222222222222210, 0.1736111111111111049, 0.1749999999999999889, 0.1763888888888889006, 0.1777777777777777846, 0.1791666666666666685, 0.1805555555555555525, 0.1819444444444444364, 0.1833333333333333204, 0.1847222222222222321, 0.1861111111111111160, 0.1875000000000000000, 0.1888888888888888840, 0.1902777777777777679, 0.1916666666666666796, 0.1930555555555555636, 0.1944444444444444475, 0.1958333333333333315, 0.1972222222222222154, 0.1986111111111110994, 0.2000000000000000111, 0.2013888888888888951, 0.2027777777777777790, 0.2041666666666666630, 0.2055555555555555469, 0.2069444444444444309, 0.2083333333333333426, 0.2097222222222222265, 0.2111111111111111105, 0.2124999999999999944, 0.2138888888888888784, 0.2152777777777777901, 0.2166666666666666741, 0.2180555555555555580, 0.2194444444444444420, 0.2208333333333333259, 0.2222222222222222099, 0.2236111111111111216, 0.2250000000000000056, 0.2263888888888888895, 0.2277777777777777735, 0.2291666666666666574, 0.2305555555555555691, 0.2319444444444444531, 0.2333333333333333370, 0.2347222222222222210, 0.2361111111111111049, 0.2374999999999999889, 0.2388888888888889006, 0.2402777777777777846, 0.2416666666666666685, 0.2430555555555555525, 0.2444444444444444364, 0.2458333333333333204, 0.2472222222222222321, 0.2486111111111111160, 0.2500000000000000000, 0.2513888888888888840, 0.2527777777777777679, 0.2541666666666666519, 0.2555555555555555358, 0.2569444444444444198, 0.2583333333333333592, 0.2597222222222222432, 0.2611111111111111271, 0.2625000000000000111, 0.2638888888888888951, 0.2652777777777777790, 0.2666666666666666630, 0.2680555555555555469, 0.2694444444444444309, 0.2708333333333333148, 0.2722222222222221988, 0.2736111111111111382, 0.2750000000000000222, 0.2763888888888889062, 0.2777777777777777901, 0.2791666666666666741, 0.2805555555555555580, 0.2819444444444444420, 0.2833333333333333259, 0.2847222222222222099, 0.2861111111111110938, 0.2874999999999999778, 0.2888888888888888618, 0.2902777777777778012, 0.2916666666666666852, 0.2930555555555555691, 0.2944444444444444531, 0.2958333333333333370, 0.2972222222222222210, 0.2986111111111111049, 0.2999999999999999889, 0.3013888888888888729, 0.3027777777777777568, 0.3041666666666666408, 0.3055555555555555802, 0.3069444444444444642, 0.3083333333333333481, 0.3097222222222222321, 0.3111111111111111160, 0.3125000000000000000, 0.3138888888888888840, 0.3152777777777777679, 0.3166666666666666519, 0.3180555555555555358, 0.3194444444444444198, 0.3208333333333333592, 0.3222222222222222432, 0.3236111111111111271, 0.3250000000000000111, 0.3263888888888888951, 0.3277777777777777790, 0.3291666666666666630, 0.3305555555555555469, 0.3319444444444444309, 0.3333333333333333148, 0.3347222222222221988, 0.3361111111111111382, 0.3375000000000000222, 0.3388888888888889062, 0.3402777777777777901, 0.3416666666666666741, 0.3430555555555555580, 0.3444444444444444420, 0.3458333333333333259, 0.3472222222222222099, 0.3486111111111110938, 0.3499999999999999778, 0.3513888888888888618, 0.3527777777777778012, 0.3541666666666666852, 0.3555555555555555691, 0.3569444444444444531, 0.3583333333333333370, 0.3597222222222222210, 0.3611111111111111049, 0.3624999999999999889, 0.3638888888888888729, 0.3652777777777777568, 0.3666666666666666408, 0.3680555555555555802, 0.3694444444444444642, 0.3708333333333333481, 0.3722222222222222321, 0.3736111111111111160, 0.3750000000000000000, 0.3763888888888888840, 0.3777777777777777679, 0.3791666666666666519, 0.3805555555555555358, 0.3819444444444444198, 0.3833333333333333592, 0.3847222222222222432, 0.3861111111111111271, 0.3875000000000000111, 0.3888888888888888951, 0.3902777777777777790, 0.3916666666666666630, 0.3930555555555555469, 0.3944444444444444309, 0.3958333333333333148, 0.3972222222222221988, 0.3986111111111111382, 0.4000000000000000222, 0.4013888888888889062, 0.4027777777777777901, 0.4041666666666666741, 0.4055555555555555580, 0.4069444444444444420, 0.4083333333333333259, 0.4097222222222222099, 0.4111111111111110938, 0.4124999999999999778, 0.4138888888888888618, 0.4152777777777778012, 0.4166666666666666852, 0.4180555555555555691, 0.4194444444444444531, 0.4208333333333333370, 0.4222222222222222210, 0.4236111111111111049, 0.4249999999999999889, 0.4263888888888888729, 0.4277777777777777568, 0.4291666666666666408, 0.4305555555555555802, 0.4319444444444444642, 0.4333333333333333481, 0.4347222222222222321, 0.4361111111111111160, 0.4375000000000000000, 0.4388888888888888840, 0.4402777777777777679, 0.4416666666666666519, 0.4430555555555555358, 0.4444444444444444198, 0.4458333333333333592, 0.4472222222222222432, 0.4486111111111111271, 0.4500000000000000111, 0.4513888888888888951, 0.4527777777777777790, 0.4541666666666666630, 0.4555555555555555469, 0.4569444444444444309, 0.4583333333333333148, 0.4597222222222221988, 0.4611111111111111382, 0.4625000000000000222, 0.4638888888888889062, 0.4652777777777777901, 0.4666666666666666741, 0.4680555555555555580, 0.4694444444444444420, 0.4708333333333333259, 0.4722222222222222099, 0.4736111111111110938, 0.4749999999999999778, 0.4763888888888888618, 0.4777777777777778012, 0.4791666666666666852, 0.4805555555555555691, 0.4819444444444444531, 0.4833333333333333370, 0.4847222222222222210, 0.4861111111111111049, 0.4874999999999999889, 0.4888888888888888729, 0.4902777777777777568, 0.4916666666666666408, 0.4930555555555555802, 0.4944444444444444642, 0.4958333333333333481, 0.4972222222222222321, 0.4986111111111111160, 0.5000000000000000000, 0.5013888888888888840, 0.5027777777777777679, 0.5041666666666666519, 0.5055555555555555358, 0.5069444444444444198, 0.5083333333333333037, 0.5097222222222221877, 0.5111111111111110716, 0.5124999999999999556, 0.5138888888888888395, 0.5152777777777777235, 0.5166666666666667185, 0.5180555555555556024, 0.5194444444444444864, 0.5208333333333333703, 0.5222222222222222543, 0.5236111111111111382, 0.5250000000000000222, 0.5263888888888889062, 0.5277777777777777901, 0.5291666666666666741, 0.5305555555555555580, 0.5319444444444444420, 0.5333333333333333259, 0.5347222222222222099, 0.5361111111111110938, 0.5374999999999999778, 0.5388888888888888618, 0.5402777777777777457, 0.5416666666666666297, 0.5430555555555555136, 0.5444444444444443976, 0.5458333333333332815, 0.5472222222222222765, 0.5486111111111111605, 0.5500000000000000444, 0.5513888888888889284, 0.5527777777777778123, 0.5541666666666666963, 0.5555555555555555802, 0.5569444444444444642, 0.5583333333333333481, 0.5597222222222222321, 0.5611111111111111160, 0.5625000000000000000, 0.5638888888888888840, 0.5652777777777777679, 0.5666666666666666519, 0.5680555555555555358, 0.5694444444444444198, 0.5708333333333333037, 0.5722222222222221877, 0.5736111111111110716, 0.5749999999999999556, 0.5763888888888888395, 0.5777777777777777235, 0.5791666666666667185, 0.5805555555555556024, 0.5819444444444444864, 0.5833333333333333703, 0.5847222222222222543, 0.5861111111111111382, 0.5875000000000000222, 0.5888888888888889062, 0.5902777777777777901, 0.5916666666666666741, 0.5930555555555555580, 0.5944444444444444420, 0.5958333333333333259, 0.5972222222222222099, 0.5986111111111110938, 0.5999999999999999778, 0.6013888888888888618, 0.6027777777777777457, 0.6041666666666666297, 0.6055555555555555136, 0.6069444444444443976, 0.6083333333333332815, 0.6097222222222222765, 0.6111111111111111605, 0.6125000000000000444, 0.6138888888888889284, 0.6152777777777778123, 0.6166666666666666963, 0.6180555555555555802, 0.6194444444444444642, 0.6208333333333333481, 0.6222222222222222321, 0.6236111111111111160, 0.6250000000000000000, 0.6263888888888888840, 0.6277777777777777679, 0.6291666666666666519, 0.6305555555555555358, 0.6319444444444444198, 0.6333333333333333037, 0.6347222222222221877, 0.6361111111111110716, 0.6374999999999999556, 0.6388888888888888395, 0.6402777777777777235, 0.6416666666666667185, 0.6430555555555556024, 0.6444444444444444864, 0.6458333333333333703, 0.6472222222222222543, 0.6486111111111111382, 0.6500000000000000222, 0.6513888888888889062, 0.6527777777777777901, 0.6541666666666666741, 0.6555555555555555580, 0.6569444444444444420, 0.6583333333333333259, 0.6597222222222222099, 0.6611111111111110938, 0.6624999999999999778, 0.6638888888888888618, 0.6652777777777777457, 0.6666666666666666297, 0.6680555555555555136, 0.6694444444444443976, 0.6708333333333332815, 0.6722222222222222765, 0.6736111111111111605, 0.6750000000000000444, 0.6763888888888889284, 0.6777777777777778123, 0.6791666666666666963, 0.6805555555555555802, 0.6819444444444444642, 0.6833333333333333481, 0.6847222222222222321, 0.6861111111111111160, 0.6875000000000000000, 0.6888888888888888840, 0.6902777777777777679, 0.6916666666666666519, 0.6930555555555555358, 0.6944444444444444198, 0.6958333333333333037, 0.6972222222222221877, 0.6986111111111110716, 0.6999999999999999556, 0.7013888888888888395, 0.7027777777777777235, 0.7041666666666667185, 0.7055555555555556024, 0.7069444444444444864, 0.7083333333333333703, 0.7097222222222222543, 0.7111111111111111382, 0.7125000000000000222, 0.7138888888888889062, 0.7152777777777777901, 0.7166666666666666741, 0.7180555555555555580, 0.7194444444444444420, 0.7208333333333333259, 0.7222222222222222099, 0.7236111111111110938, 0.7249999999999999778, 0.7263888888888888618, 0.7277777777777777457, 0.7291666666666666297, 0.7305555555555555136, 0.7319444444444443976, 0.7333333333333332815, 0.7347222222222222765, 0.7361111111111111605, 0.7375000000000000444, 0.7388888888888889284, 0.7402777777777778123, 0.7416666666666666963, 0.7430555555555555802, 0.7444444444444444642, 0.7458333333333333481, 0.7472222222222222321, 0.7486111111111111160, 0.7500000000000000000, 0.7513888888888888840, 0.7527777777777777679, 0.7541666666666666519, 0.7555555555555555358, 0.7569444444444444198, 0.7583333333333333037, 0.7597222222222221877, 0.7611111111111110716, 0.7624999999999999556, 0.7638888888888888395, 0.7652777777777777235, 0.7666666666666667185, 0.7680555555555556024, 0.7694444444444444864, 0.7708333333333333703, 0.7722222222222222543, 0.7736111111111111382, 0.7750000000000000222, 0.7763888888888889062, 0.7777777777777777901, 0.7791666666666666741, 0.7805555555555555580, 0.7819444444444444420, 0.7833333333333333259, 0.7847222222222222099, 0.7861111111111110938, 0.7874999999999999778, 0.7888888888888888618, 0.7902777777777777457, 0.7916666666666666297, 0.7930555555555555136, 0.7944444444444443976, 0.7958333333333332815, 0.7972222222222222765, 0.7986111111111111605, 0.8000000000000000444, 0.8013888888888889284, 0.8027777777777778123, 0.8041666666666666963, 0.8055555555555555802, 0.8069444444444444642, 0.8083333333333333481, 0.8097222222222222321, 0.8111111111111111160, 0.8125000000000000000, 0.8138888888888888840, 0.8152777777777777679, 0.8166666666666666519, 0.8180555555555555358, 0.8194444444444444198, 0.8208333333333333037, 0.8222222222222221877, 0.8236111111111110716, 0.8249999999999999556, 0.8263888888888888395, 0.8277777777777777235, 0.8291666666666667185, 0.8305555555555556024, 0.8319444444444444864, 0.8333333333333333703, 0.8347222222222222543, 0.8361111111111111382, 0.8375000000000000222, 0.8388888888888889062, 0.8402777777777777901, 0.8416666666666666741, 0.8430555555555555580, 0.8444444444444444420, 0.8458333333333333259, 0.8472222222222222099, 0.8486111111111110938, 0.8499999999999999778, 0.8513888888888888618, 0.8527777777777777457, 0.8541666666666666297, 0.8555555555555555136, 0.8569444444444443976, 0.8583333333333332815, 0.8597222222222222765, 0.8611111111111111605, 0.8625000000000000444, 0.8638888888888889284, 0.8652777777777778123, 0.8666666666666666963, 0.8680555555555555802, 0.8694444444444444642, 0.8708333333333333481, 0.8722222222222222321, 0.8736111111111111160, 0.8750000000000000000, 0.8763888888888888840, 0.8777777777777777679, 0.8791666666666666519, 0.8805555555555555358, 0.8819444444444444198, 0.8833333333333333037, 0.8847222222222221877, 0.8861111111111110716, 0.8874999999999999556, 0.8888888888888888395, 0.8902777777777777235, 0.8916666666666667185, 0.8930555555555556024, 0.8944444444444444864, 0.8958333333333333703, 0.8972222222222222543, 0.8986111111111111382, 0.9000000000000000222, 0.9013888888888889062, 0.9027777777777777901, 0.9041666666666666741, 0.9055555555555555580, 0.9069444444444444420, 0.9083333333333333259, 0.9097222222222222099, 0.9111111111111110938, 0.9124999999999999778, 0.9138888888888888618, 0.9152777777777777457, 0.9166666666666666297, 0.9180555555555555136, 0.9194444444444443976, 0.9208333333333332815, 0.9222222222222222765, 0.9236111111111111605, 0.9250000000000000444, 0.9263888888888889284, 0.9277777777777778123, 0.9291666666666666963, 0.9305555555555555802, 0.9319444444444444642, 0.9333333333333333481, 0.9347222222222222321, 0.9361111111111111160, 0.9375000000000000000, 0.9388888888888888840, 0.9402777777777777679, 0.9416666666666666519, 0.9430555555555555358, 0.9444444444444444198, 0.9458333333333333037, 0.9472222222222221877, 0.9486111111111110716, 0.9499999999999999556, 0.9513888888888888395, 0.9527777777777777235, 0.9541666666666667185, 0.9555555555555556024, 0.9569444444444444864, 0.9583333333333333703, 0.9597222222222222543, 0.9611111111111111382, 0.9625000000000000222, 0.9638888888888889062, 0.9652777777777777901, 0.9666666666666666741, 0.9680555555555555580, 0.9694444444444444420, 0.9708333333333333259, 0.9722222222222222099, 0.9736111111111110938, 0.9749999999999999778, 0.9763888888888888618, 0.9777777777777777457, 0.9791666666666666297, 0.9805555555555555136, 0.9819444444444443976, 0.9833333333333332815, 0.9847222222222222765, 0.9861111111111111605, 0.9875000000000000444, 0.9888888888888889284, 0.9902777777777778123, 0.9916666666666666963, 0.9930555555555555802, 0.9944444444444444642, 0.9958333333333333481, 0.9972222222222222321, 0.9986111111111111160, 1.000000000000000000 ),
 .UNSPECIFIED. ) 
 CURVE ( )  GEOMETRIC_REPRESENTATION_ITEM ( )  RATIONAL_B_SPLINE_CURVE ( ( 1.000000000000000000, 0.8660254037844387076, 1.000000000000000000, 0.8660254037844387076, 1.000000000000000000, 0.8660254037844387076, 1.000000000000000000, 0.8660254037844387076, 1.000000000000000000, 0.8660254037844387076, 1.000000000000000000, 0.8660254037844387076, 1.000000000000000000, 0.8660254037844387076, 1.000000000000000000, 0.8660254037844387076, 1.000000000000000000, 0.8660254037844387076, 1.000000000000000000, 0.8660254037844387076, 1.000000000000000000, 0.8660254037844387076, 1.000000000000000000, 0.8660254037844387076, 1.000000000000000000, 0.8660254037844387076, 1.000000000000000000, 0.8660254037844387076, 1.000000000000000000, 0.8660254037844387076, 1.000000000000000000, 0.8660254037844387076, 1.000000000000000000, 0.8660254037844387076, 1.000000000000000000, 0.8660254037844387076, 1.000000000000000000, 0.8660254037844387076, 1.000000000000000000, 0.8660254037844387076, 1.000000000000000000, 0.8660254037844387076, 1.000000000000000000, 0.8660254037844387076, 1.000000000000000000, 0.8660254037844387076, 1.000000000000000000, 0.8660254037844387076, 1.000000000000000000, 0.8660254037844387076, 1.000000000000000000, 0.8660254037844387076, 1.000000000000000000, 0.8660254037844387076, 1.000000000000000000, 0.8660254037844387076, 1.000000000000000000, 0.8660254037844387076, 1.000000000000000000, 0.8660254037844387076, 1.000000000000000000, 0.8660254037844387076, 1.000000000000000000, 0.8660254037844387076, 1.000000000000000000, 0.8660254037844387076, 1.000000000000000000, 0.8660254037844387076, 1.000000000000000000, 0.8660254037844387076, 1.000000000000000000, 0.8660254037844387076, 1.000000000000000000, 0.8660254037844387076, 1.000000000000000000, 0.8660254037844387076, 1.000000000000000000, 0.8660254037844387076, 1.000000000000000000, 0.8660254037844387076, 1.000000000000000000, 0.8660254037844387076, 1.000000000000000000, 0.8660254037844387076, 1.000000000000000000, 0.8660254037844387076, 1.000000000000000000, 0.8660254037844387076, 1.000000000000000000, 0.8660254037844387076, 1.000000000000000000, 0.8660254037844387076, 1.000000000000000000, 0.8660254037844387076, 1.000000000000000000, 0.8660254037844387076, 1.000000000000000000, 0.8660254037844387076, 1.000000000000000000, 0.8660254037844387076, 1.000000000000000000, 0.8660254037844387076, 1.000000000000000000, 0.8660254037844387076, 1.000000000000000000, 0.8660254037844387076, 1.000000000000000000, 0.8660254037844387076, 1.000000000000000000, 0.8660254037844387076, 1.000000000000000000, 0.8660254037844387076, 1.000000000000000000, 0.8660254037844387076, 1.000000000000000000, 0.8660254037844387076, 1.000000000000000000, 0.8660254037844387076, 1.000000000000000000, 0.8660254037844387076, 1.000000000000000000, 0.8660254037844387076, 1.000000000000000000, 0.8660254037844387076, 1.000000000000000000, 0.8660254037844387076, 1.000000000000000000, 0.8660254037844387076, 1.000000000000000000, 0.8660254037844387076, 1.000000000000000000, 0.8660254037844387076, 1.000000000000000000, 0.8660254037844387076, 1.000000000000000000, 0.8660254037844387076, 1.000000000000000000, 0.8660254037844387076, 1.000000000000000000, 0.8660254037844387076, 1.000000000000000000, 0.8660254037844387076, 1.000000000000000000, 0.8660254037844387076, 1.000000000000000000, 0.8660254037844387076, 1.000000000000000000, 0.8660254037844387076, 1.000000000000000000, 0.8660254037844387076, 1.000000000000000000, 0.8660254037844387076, 1.000000000000000000, 0.8660254037844387076, 1.000000000000000000, 0.8660254037844387076, 1.000000000000000000, 0.8660254037844387076, 1.000000000000000000, 0.8660254037844387076, 1.000000000000000000, 0.8660254037844387076, 1.000000000000000000, 0.8660254037844387076, 1.000000000000000000, 0.8660254037844387076, 1.000000000000000000, 0.8660254037844387076, 1.000000000000000000, 0.8660254037844387076, 1.000000000000000000, 0.8660254037844387076, 1.000000000000000000, 0.8660254037844387076, 1.000000000000000000, 0.8660254037844387076, 1.000000000000000000, 0.8660254037844387076, 1.000000000000000000, 0.8660254037844387076, 1.000000000000000000, 0.8660254037844387076, 1.000000000000000000, 0.8660254037844387076, 1.000000000000000000, 0.8660254037844387076, 1.000000000000000000, 0.8660254037844387076, 1.000000000000000000, 0.8660254037844387076, 1.000000000000000000, 0.8660254037844387076, 1.000000000000000000, 0.8660254037844387076, 1.000000000000000000, 0.8660254037844387076, 1.000000000000000000, 0.8660254037844387076, 1.000000000000000000, 0.8660254037844387076, 1.000000000000000000, 0.8660254037844387076, 1.000000000000000000, 0.8660254037844387076, 1.000000000000000000, 0.8660254037844387076, 1.000000000000000000, 0.8660254037844387076, 1.000000000000000000, 0.8660254037844387076, 1.000000000000000000, 0.8660254037844387076, 1.000000000000000000, 0.8660254037844387076, 1.000000000000000000, 0.8660254037844387076, 1.000000000000000000, 0.8660254037844387076, 1.000000000000000000, 0.8660254037844387076, 1.000000000000000000, 0.8660254037844387076, 1.000000000000000000, 0.8660254037844387076, 1.000000000000000000, 0.8660254037844387076, 1.000000000000000000, 0.8660254037844387076, 1.000000000000000000, 0.8660254037844387076, 1.000000000000000000, 0.8660254037844387076, 1.000000000000000000, 0.8660254037844387076, 1.000000000000000000, 0.8660254037844387076, 1.000000000000000000, 0.8660254037844387076, 1.000000000000000000, 0.8660254037844387076, 1.000000000000000000, 0.8660254037844387076, 1.000000000000000000, 0.8660254037844387076, 1.000000000000000000, 0.8660254037844387076, 1.000000000000000000, 0.8660254037844387076, 1.000000000000000000, 0.8660254037844387076, 1.000000000000000000, 0.8660254037844387076, 1.000000000000000000, 0.8660254037844387076, 1.000000000000000000, 0.8660254037844387076, 1.000000000000000000, 0.8660254037844387076, 1.000000000000000000, 0.8660254037844387076, 1.000000000000000000, 0.8660254037844387076, 1.000000000000000000, 0.8660254037844387076, 1.000000000000000000, 0.8660254037844387076, 1.000000000000000000, 0.8660254037844387076, 1.000000000000000000, 0.8660254037844387076, 1.000000000000000000, 0.8660254037844387076, 1.000000000000000000, 0.8660254037844387076, 1.000000000000000000, 0.8660254037844387076, 1.000000000000000000, 0.8660254037844387076, 1.000000000000000000, 0.8660254037844387076, 1.000000000000000000, 0.8660254037844387076, 1.000000000000000000, 0.8660254037844387076, 1.000000000000000000, 0.8660254037844387076, 1.000000000000000000, 0.8660254037844387076, 1.000000000000000000, 0.8660254037844387076, 1.000000000000000000, 0.8660254037844387076, 1.000000000000000000, 0.8660254037844387076, 1.000000000000000000, 0.8660254037844387076, 1.000000000000000000, 0.8660254037844387076, 1.000000000000000000, 0.8660254037844387076, 1.000000000000000000, 0.8660254037844387076, 1.000000000000000000, 0.8660254037844387076, 1.000000000000000000, 0.8660254037844387076, 1.000000000000000000, 0.8660254037844387076, 1.000000000000000000, 0.8660254037844387076, 1.000000000000000000, 0.8660254037844387076, 1.000000000000000000, 0.8660254037844387076, 1.000000000000000000, 0.8660254037844387076, 1.000000000000000000, 0.8660254037844387076, 1.000000000000000000, 0.8660254037844387076, 1.000000000000000000, 0.8660254037844387076, 1.000000000000000000, 0.8660254037844387076, 1.000000000000000000, 0.8660254037844387076, 1.000000000000000000, 0.8660254037844387076, 1.000000000000000000, 0.8660254037844387076, 1.000000000000000000, 0.8660254037844387076, 1.000000000000000000, 0.8660254037844387076, 1.000000000000000000, 0.8660254037844387076, 1.000000000000000000, 0.8660254037844387076, 1.000000000000000000, 0.8660254037844387076, 1.000000000000000000, 0.8660254037844387076, 1.000000000000000000, 0.8660254037844387076, 1.000000000000000000, 0.8660254037844387076, 1.000000000000000000, 0.8660254037844387076, 1.000000000000000000, 0.8660254037844387076, 1.000000000000000000, 0.8660254037844387076, 1.000000000000000000, 0.8660254037844387076, 1.000000000000000000, 0.8660254037844387076, 1.000000000000000000, 0.8660254037844387076, 1.000000000000000000, 0.8660254037844387076, 1.000000000000000000, 0.8660254037844387076, 1.000000000000000000, 0.8660254037844387076, 1.000000000000000000, 0.8660254037844387076, 1.000000000000000000, 0.8660254037844387076, 1.000000000000000000, 0.8660254037844387076, 1.000000000000000000, 0.8660254037844387076, 1.000000000000000000, 0.8660254037844387076, 1.000000000000000000, 0.8660254037844387076, 1.000000000000000000, 0.8660254037844387076, 1.000000000000000000, 0.8660254037844387076, 1.000000000000000000, 0.8660254037844387076, 1.000000000000000000, 0.8660254037844387076, 1.000000000000000000, 0.8660254037844387076, 1.000000000000000000, 0.8660254037844387076, 1.000000000000000000, 0.8660254037844387076, 1.000000000000000000, 0.8660254037844387076, 1.000000000000000000, 0.8660254037844387076, 1.000000000000000000, 0.8660254037844387076, 1.000000000000000000, 0.8660254037844387076, 1.000000000000000000, 0.8660254037844387076, 1.000000000000000000, 0.8660254037844387076, 1.000000000000000000, 0.8660254037844387076, 1.000000000000000000, 0.8660254037844387076, 1.000000000000000000, 0.8660254037844387076, 1.000000000000000000, 0.8660254037844387076, 1.000000000000000000, 0.8660254037844387076, 1.000000000000000000, 0.8660254037844387076, 1.000000000000000000, 0.8660254037844387076, 1.000000000000000000, 0.8660254037844387076, 1.000000000000000000, 0.8660254037844387076, 1.000000000000000000, 0.8660254037844387076, 1.000000000000000000, 0.8660254037844387076, 1.000000000000000000, 0.8660254037844387076, 1.000000000000000000, 0.8660254037844387076, 1.000000000000000000, 0.8660254037844387076, 1.000000000000000000, 0.8660254037844387076, 1.000000000000000000, 0.8660254037844387076, 1.000000000000000000, 0.8660254037844387076, 1.000000000000000000, 0.8660254037844387076, 1.000000000000000000, 0.8660254037844387076, 1.000000000000000000, 0.8660254037844387076, 1.000000000000000000, 0.8660254037844387076, 1.000000000000000000, 0.8660254037844387076, 1.000000000000000000, 0.8660254037844387076, 1.000000000000000000, 0.8660254037844387076, 1.000000000000000000, 0.8660254037844387076, 1.000000000000000000, 0.8660254037844387076, 1.000000000000000000, 0.8660254037844387076, 1.000000000000000000, 0.8660254037844387076, 1.000000000000000000, 0.8660254037844387076, 1.000000000000000000, 0.8660254037844387076, 1.000000000000000000, 0.8660254037844387076, 1.000000000000000000, 0.8660254037844387076, 1.000000000000000000, 0.8660254037844387076, 1.000000000000000000, 0.8660254037844387076, 1.000000000000000000, 0.8660254037844387076, 1.000000000000000000, 0.8660254037844387076, 1.000000000000000000, 0.8660254037844387076, 1.000000000000000000, 0.8660254037844387076, 1.000000000000000000, 0.8660254037844387076, 1.000000000000000000, 0.8660254037844387076, 1.000000000000000000, 0.8660254037844387076, 1.000000000000000000, 0.8660254037844387076, 1.000000000000000000, 0.8660254037844387076, 1.000000000000000000, 0.8660254037844387076, 1.000000000000000000, 0.8660254037844387076, 1.000000000000000000, 0.8660254037844387076, 1.000000000000000000, 0.8660254037844387076, 1.000000000000000000, 0.8660254037844387076, 1.000000000000000000, 0.8660254037844387076, 1.000000000000000000, 0.8660254037844387076, 1.000000000000000000, 0.8660254037844387076, 1.000000000000000000, 0.8660254037844387076, 1.000000000000000000, 0.8660254037844387076, 1.000000000000000000, 0.8660254037844387076, 1.000000000000000000, 0.8660254037844387076, 1.000000000000000000, 0.8660254037844387076, 1.000000000000000000, 0.8660254037844387076, 1.000000000000000000, 0.8660254037844387076, 1.000000000000000000, 0.8660254037844387076, 1.000000000000000000, 0.8660254037844387076, 1.000000000000000000, 0.8660254037844387076, 1.000000000000000000, 0.8660254037844387076, 1.000000000000000000, 0.8660254037844387076, 1.000000000000000000, 0.8660254037844387076, 1.000000000000000000, 0.8660254037844387076, 1.000000000000000000, 0.8660254037844387076, 1.000000000000000000, 0.8660254037844387076, 1.000000000000000000, 0.8660254037844387076, 1.000000000000000000, 0.8660254037844387076, 1.000000000000000000, 0.8660254037844387076, 1.000000000000000000, 0.8660254037844387076, 1.000000000000000000, 0.8660254037844387076, 1.000000000000000000, 0.8660254037844387076, 1.000000000000000000, 0.8660254037844387076, 1.000000000000000000, 0.8660254037844387076, 1.000000000000000000, 0.8660254037844387076, 1.000000000000000000, 0.8660254037844387076, 1.000000000000000000, 0.8660254037844387076, 1.000000000000000000, 0.8660254037844387076, 1.000000000000000000, 0.8660254037844387076, 1.000000000000000000, 0.8660254037844387076, 1.000000000000000000, 0.8660254037844387076, 1.000000000000000000, 0.8660254037844387076, 1.000000000000000000, 0.8660254037844387076, 1.000000000000000000, 0.8660254037844387076, 1.000000000000000000, 0.8660254037844387076, 1.000000000000000000, 0.8660254037844387076, 1.000000000000000000, 0.8660254037844387076, 1.000000000000000000, 0.8660254037844387076, 1.000000000000000000, 0.8660254037844387076, 1.000000000000000000, 0.8660254037844387076, 1.000000000000000000, 0.8660254037844387076, 1.000000000000000000, 0.8660254037844387076, 1.000000000000000000, 0.8660254037844387076, 1.000000000000000000, 0.8660254037844387076, 1.000000000000000000, 0.8660254037844387076, 1.000000000000000000, 0.8660254037844387076, 1.000000000000000000, 0.8660254037844387076, 1.000000000000000000, 0.8660254037844387076, 1.000000000000000000, 0.8660254037844387076, 1.000000000000000000, 0.8660254037844387076, 1.000000000000000000, 0.8660254037844387076, 1.000000000000000000, 0.8660254037844387076, 1.000000000000000000, 0.8660254037844387076, 1.000000000000000000, 0.8660254037844387076, 1.000000000000000000, 0.8660254037844387076, 1.000000000000000000, 0.8660254037844387076, 1.000000000000000000, 0.8660254037844387076, 1.000000000000000000, 0.8660254037844387076, 1.000000000000000000, 0.8660254037844387076, 1.000000000000000000, 0.8660254037844387076, 1.000000000000000000, 0.8660254037844387076, 1.000000000000000000, 0.8660254037844387076, 1.000000000000000000, 0.8660254037844387076, 1.000000000000000000, 0.8660254037844387076, 1.000000000000000000, 0.8660254037844387076, 1.000000000000000000, 0.8660254037844387076, 1.000000000000000000, 0.8660254037844387076, 1.000000000000000000, 0.8660254037844387076, 1.000000000000000000, 0.8660254037844387076, 1.000000000000000000, 0.8660254037844387076, 1.000000000000000000, 0.8660254037844387076, 1.000000000000000000, 0.8660254037844387076, 1.000000000000000000, 0.8660254037844387076, 1.000000000000000000, 0.8660254037844387076, 1.000000000000000000, 0.8660254037844387076, 1.000000000000000000, 0.8660254037844387076, 1.000000000000000000, 0.8660254037844387076, 1.000000000000000000, 0.8660254037844387076, 1.000000000000000000, 0.8660254037844387076, 1.000000000000000000, 0.8660254037844387076, 1.000000000000000000, 0.8660254037844387076, 1.000000000000000000, 0.8660254037844387076, 1.000000000000000000, 0.8660254037844387076, 1.000000000000000000, 0.8660254037844387076, 1.000000000000000000, 0.8660254037844387076, 1.000000000000000000, 0.8660254037844387076, 1.000000000000000000, 0.8660254037844387076, 1.000000000000000000, 0.8660254037844387076, 1.000000000000000000, 0.8660254037844387076, 1.000000000000000000, 0.8660254037844387076, 1.000000000000000000, 0.8660254037844387076, 1.000000000000000000, 0.8660254037844387076, 1.000000000000000000, 0.8660254037844387076, 1.000000000000000000, 0.8660254037844387076, 1.000000000000000000, 0.8660254037844387076, 1.000000000000000000, 0.8660254037844387076, 1.000000000000000000, 0.8660254037844387076, 1.000000000000000000, 0.8660254037844387076, 1.000000000000000000, 0.8660254037844387076, 1.000000000000000000, 0.8660254037844387076, 1.000000000000000000, 0.8660254037844387076, 1.000000000000000000, 0.8660254037844387076, 1.000000000000000000, 0.8660254037844387076, 1.000000000000000000, 0.8660254037844387076, 1.000000000000000000, 0.8660254037844387076, 1.000000000000000000, 0.8660254037844387076, 1.000000000000000000, 0.8660254037844387076, 1.000000000000000000, 0.8660254037844387076, 1.000000000000000000, 0.8660254037844387076, 1.000000000000000000, 0.8660254037844387076, 1.000000000000000000, 0.8660254037844387076, 1.000000000000000000, 0.8660254037844387076, 1.000000000000000000, 0.8660254037844387076, 1.000000000000000000, 0.8660254037844387076, 1.000000000000000000, 0.8660254037844387076, 1.000000000000000000, 0.8660254037844387076, 1.000000000000000000, 0.8660254037844387076, 1.000000000000000000, 0.8660254037844387076, 1.000000000000000000, 0.8660254037844387076, 1.000000000000000000, 0.8660254037844387076, 1.000000000000000000, 0.8660254037844387076, 1.000000000000000000, 0.8660254037844387076, 1.000000000000000000, 0.8660254037844387076, 1.000000000000000000, 0.8660254037844387076, 1.000000000000000000, 0.8660254037844387076, 1.000000000000000000, 0.8660254037844387076, 1.000000000000000000, 0.8660254037844387076, 1.000000000000000000, 0.8660254037844387076, 1.000000000000000000, 0.8660254037844387076, 1.000000000000000000, 0.8660254037844387076, 1.000000000000000000, 0.8660254037844387076, 1.000000000000000000, 0.8660254037844387076, 1.000000000000000000, 0.8660254037844387076, 1.000000000000000000, 0.8660254037844387076, 1.000000000000000000, 0.8660254037844387076, 1.000000000000000000, 0.8660254037844387076, 1.000000000000000000, 0.8660254037844387076, 1.000000000000000000, 0.8660254037844387076, 1.000000000000000000, 0.8660254037844387076, 1.000000000000000000, 0.8660254037844387076, 1.000000000000000000, 0.8660254037844387076, 1.000000000000000000, 0.8660254037844387076, 1.000000000000000000, 0.8660254037844387076, 1.000000000000000000, 0.8660254037844387076, 1.000000000000000000, 0.8660254037844387076, 1.000000000000000000, 0.8660254037844387076, 1.000000000000000000, 0.8660254037844387076, 1.000000000000000000, 0.8660254037844387076, 1.000000000000000000, 0.8660254037844387076, 1.000000000000000000, 0.8660254037844387076, 1.000000000000000000, 0.8660254037844387076, 1.000000000000000000, 0.8660254037844387076, 1.000000000000000000, 0.8660254037844387076, 1.000000000000000000, 0.8660254037844387076, 1.000000000000000000, 0.8660254037844387076, 1.000000000000000000, 0.8660254037844387076, 1.000000000000000000, 0.8660254037844387076, 1.000000000000000000, 0.8660254037844387076, 1.000000000000000000, 0.8660254037844387076, 1.000000000000000000, 0.8660254037844387076, 1.000000000000000000, 0.8660254037844387076, 1.000000000000000000, 0.8660254037844387076, 1.000000000000000000, 0.8660254037844387076, 1.000000000000000000, 0.8660254037844387076, 1.000000000000000000, 0.8660254037844387076, 1.000000000000000000, 0.8660254037844387076, 1.000000000000000000, 0.8660254037844387076, 1.000000000000000000, 0.8660254037844387076, 1.000000000000000000, 0.8660254037844387076, 1.000000000000000000, 0.8660254037844387076, 1.000000000000000000, 0.8660254037844387076, 1.000000000000000000, 0.8660254037844387076, 1.000000000000000000, 0.8660254037844387076, 1.000000000000000000, 0.8660254037844387076, 1.000000000000000000, 0.8660254037844387076, 1.000000000000000000, 0.8660254037844387076, 1.000000000000000000, 0.8660254037844387076, 1.000000000000000000, 0.8660254037844387076, 1.000000000000000000, 0.8660254037844387076, 1.000000000000000000, 0.8660254037844387076, 1.000000000000000000, 0.8660254037844387076, 1.000000000000000000, 0.8660254037844387076, 1.000000000000000000, 0.8660254037844387076, 1.000000000000000000, 0.8660254037844387076, 1.000000000000000000, 0.8660254037844387076, 1.000000000000000000, 0.8660254037844387076, 1.000000000000000000, 0.8660254037844387076, 1.000000000000000000, 0.8660254037844387076, 1.000000000000000000, 0.8660254037844387076, 1.000000000000000000, 0.8660254037844387076, 1.000000000000000000, 0.8660254037844387076, 1.000000000000000000, 0.8660254037844387076, 1.000000000000000000, 0.8660254037844387076, 1.000000000000000000, 0.8660254037844387076, 1.000000000000000000, 0.8660254037844387076, 1.000000000000000000, 0.8660254037844387076, 1.000000000000000000, 0.8660254037844387076, 1.000000000000000000, 0.8660254037844387076, 1.000000000000000000, 0.8660254037844387076, 1.000000000000000000, 0.8660254037844387076, 1.000000000000000000, 0.8660254037844387076, 1.000000000000000000, 0.8660254037844387076, 1.000000000000000000, 0.8660254037844387076, 1.000000000000000000, 0.8660254037844387076, 1.000000000000000000, 0.8660254037844387076, 1.000000000000000000, 0.8660254037844387076, 1.000000000000000000, 0.8660254037844387076, 1.000000000000000000, 0.8660254037844387076, 1.000000000000000000, 0.8660254037844387076, 1.000000000000000000, 0.8660254037844387076, 1.000000000000000000, 0.8660254037844387076, 1.000000000000000000, 0.8660254037844387076, 1.000000000000000000, 0.8660254037844387076, 1.000000000000000000, 0.8660254037844387076, 1.000000000000000000, 0.8660254037844387076, 1.000000000000000000, 0.8660254037844387076, 1.000000000000000000, 0.8660254037844387076, 1.000000000000000000, 0.8660254037844387076, 1.000000000000000000, 0.8660254037844387076, 1.000000000000000000, 0.8660254037844387076, 1.000000000000000000, 0.8660254037844387076, 1.000000000000000000, 0.8660254037844387076, 1.000000000000000000, 0.8660254037844387076, 1.000000000000000000, 0.8660254037844387076, 1.000000000000000000, 0.8660254037844387076, 1.000000000000000000, 0.8660254037844387076, 1.000000000000000000, 0.8660254037844387076, 1.000000000000000000, 0.8660254037844387076, 1.000000000000000000, 0.8660254037844387076, 1.000000000000000000, 0.8660254037844387076, 1.000000000000000000, 0.8660254037844387076, 1.000000000000000000, 0.8660254037844387076, 1.000000000000000000, 0.8660254037844387076, 1.000000000000000000, 0.8660254037844387076, 1.000000000000000000, 0.8660254037844387076, 1.000000000000000000, 0.8660254037844387076, 1.000000000000000000, 0.8660254037844387076, 1.000000000000000000, 0.8660254037844387076, 1.000000000000000000, 0.8660254037844387076, 1.000000000000000000, 0.8660254037844387076, 1.000000000000000000, 0.8660254037844387076, 1.000000000000000000, 0.8660254037844387076, 1.000000000000000000, 0.8660254037844387076, 1.000000000000000000, 0.8660254037844387076, 1.000000000000000000, 0.8660254037844387076, 1.000000000000000000, 0.8660254037844387076, 1.000000000000000000, 0.8660254037844387076, 1.000000000000000000, 0.8660254037844387076, 1.000000000000000000, 0.8660254037844387076, 1.000000000000000000, 0.8660254037844387076, 1.000000000000000000, 0.8660254037844387076, 1.000000000000000000, 0.8660254037844387076, 1.000000000000000000, 0.8660254037844387076, 1.000000000000000000, 0.8660254037844387076, 1.000000000000000000, 0.8660254037844387076, 1.000000000000000000, 0.8660254037844387076, 1.000000000000000000, 0.8660254037844387076, 1.000000000000000000, 0.8660254037844387076, 1.000000000000000000, 0.8660254037844387076, 1.000000000000000000, 0.8660254037844387076, 1.000000000000000000, 0.8660254037844387076, 1.000000000000000000, 0.8660254037844387076, 1.000000000000000000, 0.8660254037844387076, 1.000000000000000000, 0.8660254037844387076, 1.000000000000000000, 0.8660254037844387076, 1.000000000000000000, 0.8660254037844387076, 1.000000000000000000, 0.8660254037844387076, 1.000000000000000000, 0.8660254037844387076, 1.000000000000000000, 0.8660254037844387076, 1.000000000000000000, 0.8660254037844387076, 1.000000000000000000, 0.8660254037844387076, 1.000000000000000000, 0.8660254037844387076, 1.000000000000000000, 0.8660254037844387076, 1.000000000000000000, 0.8660254037844387076, 1.000000000000000000, 0.8660254037844387076, 1.000000000000000000, 0.8660254037844387076, 1.000000000000000000, 0.8660254037844387076, 1.000000000000000000, 0.8660254037844387076, 1.000000000000000000, 0.8660254037844387076, 1.000000000000000000, 0.8660254037844387076, 1.000000000000000000, 0.8660254037844387076, 1.000000000000000000, 0.8660254037844387076, 1.000000000000000000, 0.8660254037844387076, 1.000000000000000000, 0.8660254037844387076, 1.000000000000000000, 0.8660254037844387076, 1.000000000000000000, 0.8660254037844387076, 1.000000000000000000, 0.8660254037844387076, 1.000000000000000000, 0.8660254037844387076, 1.000000000000000000, 0.8660254037844387076, 1.000000000000000000, 0.8660254037844387076, 1.000000000000000000, 0.8660254037844387076, 1.000000000000000000, 0.8660254037844387076, 1.000000000000000000, 0.8660254037844387076, 1.000000000000000000, 0.8660254037844387076, 1.000000000000000000, 0.8660254037844387076, 1.000000000000000000, 0.8660254037844387076, 1.000000000000000000, 0.8660254037844387076, 1.000000000000000000, 0.8660254037844387076, 1.000000000000000000, 0.8660254037844387076, 1.000000000000000000, 0.8660254037844387076, 1.000000000000000000, 0.8660254037844387076, 1.000000000000000000, 0.8660254037844387076, 1.000000000000000000, 0.8660254037844387076, 1.000000000000000000, 0.8660254037844387076, 1.000000000000000000, 0.8660254037844387076, 1.000000000000000000, 0.8660254037844387076, 1.000000000000000000, 0.8660254037844387076, 1.000000000000000000, 0.8660254037844387076, 1.000000000000000000, 0.8660254037844387076, 1.000000000000000000, 0.8660254037844387076, 1.000000000000000000, 0.8660254037844387076, 1.000000000000000000, 0.8660254037844387076, 1.000000000000000000, 0.8660254037844387076, 1.000000000000000000, 0.8660254037844387076, 1.000000000000000000, 0.8660254037844387076, 1.000000000000000000, 0.8660254037844387076, 1.000000000000000000, 0.8660254037844387076, 1.000000000000000000, 0.8660254037844387076, 1.000000000000000000, 0.8660254037844387076, 1.000000000000000000, 0.8660254037844387076, 1.000000000000000000, 0.8660254037844387076, 1.000000000000000000, 0.8660254037844387076, 1.000000000000000000, 0.8660254037844387076, 1.000000000000000000, 0.8660254037844387076, 1.000000000000000000, 0.8660254037844387076, 1.000000000000000000, 0.8660254037844387076, 1.000000000000000000, 0.8660254037844387076, 1.000000000000000000, 0.8660254037844387076, 1.000000000000000000, 0.8660254037844387076, 1.000000000000000000, 0.8660254037844387076, 1.000000000000000000, 0.8660254037844387076, 1.000000000000000000, 0.8660254037844387076, 1.000000000000000000, 0.8660254037844387076, 1.000000000000000000, 0.8660254037844387076, 1.000000000000000000, 0.8660254037844387076, 1.000000000000000000, 0.8660254037844387076, 1.000000000000000000, 0.8660254037844387076, 1.000000000000000000, 0.8660254037844387076, 1.000000000000000000, 0.8660254037844387076, 1.000000000000000000, 0.8660254037844387076, 1.000000000000000000, 0.8660254037844387076, 1.000000000000000000, 0.8660254037844387076, 1.000000000000000000, 0.8660254037844387076, 1.000000000000000000, 0.8660254037844387076, 1.000000000000000000, 0.8660254037844387076, 1.000000000000000000, 0.8660254037844387076, 1.000000000000000000, 0.8660254037844387076, 1.000000000000000000, 0.8660254037844387076, 1.000000000000000000, 0.8660254037844387076, 1.000000000000000000, 0.8660254037844387076, 1.000000000000000000, 0.8660254037844387076, 1.000000000000000000, 0.8660254037844387076, 1.000000000000000000, 0.8660254037844387076, 1.000000000000000000, 0.8660254037844387076, 1.000000000000000000, 0.8660254037844387076, 1.000000000000000000, 0.8660254037844387076, 1.000000000000000000, 0.8660254037844387076, 1.000000000000000000, 0.8660254037844387076, 1.000000000000000000, 0.8660254037844387076, 1.000000000000000000, 0.8660254037844387076, 1.000000000000000000, 0.8660254037844387076, 1.000000000000000000, 0.8660254037844387076, 1.000000000000000000, 0.8660254037844387076, 1.000000000000000000, 0.8660254037844387076, 1.000000000000000000, 0.8660254037844387076, 1.000000000000000000, 0.8660254037844387076, 1.000000000000000000, 0.8660254037844387076, 1.000000000000000000, 0.8660254037844387076, 1.000000000000000000, 0.8660254037844387076, 1.000000000000000000, 0.8660254037844387076, 1.000000000000000000, 0.8660254037844387076, 1.000000000000000000, 0.8660254037844387076, 1.000000000000000000, 0.8660254037844387076, 1.000000000000000000, 0.8660254037844387076, 1.000000000000000000, 0.8660254037844387076, 1.000000000000000000, 0.8660254037844387076, 1.000000000000000000, 0.8660254037844387076, 1.000000000000000000, 0.8660254037844387076, 1.000000000000000000, 0.8660254037844387076, 1.000000000000000000, 0.8660254037844387076, 1.000000000000000000, 0.8660254037844387076, 1.000000000000000000, 0.8660254037844387076, 1.000000000000000000, 0.8660254037844387076, 1.000000000000000000, 0.8660254037844387076, 1.000000000000000000, 0.8660254037844387076, 1.000000000000000000, 0.8660254037844387076, 1.000000000000000000, 0.8660254037844387076, 1.000000000000000000, 0.8660254037844387076, 1.000000000000000000, 0.8660254037844387076, 1.000000000000000000, 0.8660254037844387076, 1.000000000000000000, 0.8660254037844387076, 1.000000000000000000, 0.8660254037844387076, 1.000000000000000000, 0.8660254037844387076, 1.000000000000000000, 0.8660254037844387076, 1.000000000000000000, 0.8660254037844387076, 1.000000000000000000, 0.8660254037844387076, 1.000000000000000000, 0.8660254037844387076, 1.000000000000000000, 0.8660254037844387076, 1.000000000000000000, 0.8660254037844387076, 1.000000000000000000, 0.8660254037844387076, 1.000000000000000000, 0.8660254037844387076, 1.000000000000000000, 0.8660254037844387076, 1.000000000000000000, 0.8660254037844387076, 1.000000000000000000, 0.8660254037844387076, 1.000000000000000000, 0.8660254037844387076, 1.000000000000000000, 0.8660254037844387076, 1.000000000000000000, 0.8660254037844387076, 1.000000000000000000, 0.8660254037844387076, 1.000000000000000000, 0.8660254037844387076, 1.000000000000000000, 0.8660254037844387076, 1.000000000000000000, 0.8660254037844387076, 1.000000000000000000, 0.8660254037844387076, 1.000000000000000000, 0.8660254037844387076, 1.000000000000000000, 0.8660254037844387076, 1.000000000000000000, 0.8660254037844387076, 1.000000000000000000, 0.8660254037844387076, 1.000000000000000000, 0.8660254037844387076, 1.000000000000000000, 0.8660254037844387076, 1.000000000000000000, 0.8660254037844387076, 1.000000000000000000, 0.8660254037844387076, 1.000000000000000000, 0.8660254037844387076, 1.000000000000000000, 0.8660254037844387076, 1.000000000000000000, 0.8660254037844387076, 1.000000000000000000, 0.8660254037844387076, 1.000000000000000000, 0.8660254037844387076, 1.000000000000000000, 0.8660254037844387076, 1.000000000000000000, 0.8660254037844387076, 1.000000000000000000, 0.8660254037844387076, 1.000000000000000000, 0.8660254037844387076, 1.000000000000000000, 0.8660254037844387076, 1.000000000000000000, 0.8660254037844387076, 1.000000000000000000, 0.8660254037844387076, 1.000000000000000000, 0.8660254037844387076, 1.000000000000000000, 0.8660254037844387076, 1.000000000000000000, 0.8660254037844387076, 1.000000000000000000, 0.8660254037844387076, 1.000000000000000000, 0.8660254037844387076, 1.000000000000000000, 0.8660254037844387076, 1.000000000000000000, 0.8660254037844387076, 1.000000000000000000, 0.8660254037844387076, 1.000000000000000000, 0.8660254037844387076, 1.000000000000000000, 0.8660254037844387076, 1.000000000000000000, 0.8660254037844387076, 1.000000000000000000, 0.8660254037844387076, 1.000000000000000000, 0.8660254037844387076, 1.000000000000000000, 0.8660254037844387076, 1.000000000000000000, 0.8660254037844387076, 1.000000000000000000, 0.8660254037844387076, 1.000000000000000000, 0.8660254037844387076, 1.000000000000000000, 0.8660254037844387076, 1.000000000000000000, 0.8660254037844387076, 1.000000000000000000, 0.8660254037844387076, 1.000000000000000000, 0.8660254037844387076, 1.000000000000000000, 0.8660254037844387076, 1.000000000000000000, 0.8660254037844387076, 1.000000000000000000, 0.8660254037844387076, 1.000000000000000000, 0.8660254037844387076, 1.000000000000000000, 0.8660254037844387076, 1.000000000000000000, 0.8660254037844387076, 1.000000000000000000, 0.8660254037844387076, 1.000000000000000000, 0.8660254037844387076, 1.000000000000000000, 0.8660254037844387076, 1.000000000000000000, 0.8660254037844387076, 1.000000000000000000, 0.8660254037844387076, 1.000000000000000000, 0.8660254037844387076, 1.000000000000000000, 0.8660254037844387076, 1.000000000000000000, 0.8660254037844387076, 1.000000000000000000, 0.8660254037844387076, 1.000000000000000000 ) ) 
 REPRESENTATION_ITEM ( '' )  );
#17716=CARTESIAN_POINT ( 'NONE',  ( 3.500000000000001332, 19.52072594216371826, -123.3776474690881884 ) ) ;
#17718=CARTESIAN_POINT ( 'NONE',  ( -3.500000000000000888, 19.52072594216371826, -129.0443141357548598 ) ) ;
#17719=CARTESIAN_POINT ( 'NONE',  ( 1.655278471874998436, 14.63297358603754894, -113.4307724695661364 ) ) ;
#17721=CARTESIAN_POINT ( 'NONE',  ( 3.500000000000001332, 17.50000000000002132, -128.4609808024215170 ) ) ;
#17722=CARTESIAN_POINT ( 'NONE',  ( -3.500000000000002220, 15.47927405783632793, -86.87764746908815994 ) ) ;
#17724=CARTESIAN_POINT ( 'NONE',  ( -1.655278471875002211, 14.63297358603754184, -48.59743913623280775 ) ) ;
#17725=CARTESIAN_POINT ( 'NONE',  ( 1.655278471875001101, 20.36702641396249547, -107.1849391362327992 ) ) ;
#17726=CARTESIAN_POINT ( 'NONE',  ( -1.749999999999999778, 20.53108891324555429, -83.12764746908818836 ) ) ;
#17727=CARTESIAN_POINT ( 'NONE',  ( -0.9378221735089291577, 21.00000000000001776, -99.86007260463890134 ) ) ;
#17729=CARTESIAN_POINT ( 'NONE',  ( 3.310556943750001313, 19.41135094264166838, -126.2682724695661278 ) ) ;
#17732=DIRECTION ( 'NONE',  ( 0.000000000000000000, 1.000000000000000000, 0.000000000000000000 ) ) ;
#17734=CARTESIAN_POINT ( 'NONE',  ( -1.655278471874999990, 20.36702641396248836, -59.01827246956613493 ) ) ;
#17735=AXIS2_PLACEMENT_3D ( 'NONE', #11927, #35108, #28508 ) ;
#17736=ORIENTED_EDGE ( 'NONE', *, *, #28286, .T. ) ;
#17737=CARTESIAN_POINT ( 'NONE',  ( 3.310556943750001313, 17.50000000000001776, -78.35160580289945642 ) ) ;
#17739=CARTESIAN_POINT ( 'NONE',  ( 0.9378221735089281585, 14.00000000000000888, -30.36007260463890844 ) ) ;
#17742=EDGE_CURVE ( 'NONE', #8887, #33952, #5620, .T. ) ;
#17744=CARTESIAN_POINT ( 'NONE',  ( 2.340729813953370519E-16, 21.32270188528330834, -42.01410580289947916 ) ) ;
#17745=CARTESIAN_POINT ( 'NONE',  ( 1.655278471875001101, 20.36702641396249192, -97.09743913623280775 ) ) ;
#17752=CARTESIAN_POINT ( 'NONE',  ( 3.310556943750001313, 17.50000000000001421, -55.26410580289947916 ) ) ;
#17754=EDGE_CURVE ( 'NONE', #4034, #22548, #1560, .T. ) ;
#17756=CYLINDRICAL_SURFACE ( 'NONE', #10387, 3.499999999999999556 ) ;
#17757=CARTESIAN_POINT ( 'NONE',  ( -3.695301148110399846E-14, 21.00000000000002132, -124.9047308033774186 ) ) ;
#17760=ORIENTED_EDGE ( 'NONE', *, *, #39727, .F. ) ;
#17762=CARTESIAN_POINT ( 'NONE',  ( 3.500000000000001776, 19.52072594216370405, -40.37764746908817415 ) ) ;
#17763=DIRECTION ( 'NONE',  ( -0.000000000000000000, 1.259100132267607459E-16, -1.000000000000000000 ) ) ;
#17766=CARTESIAN_POINT ( 'NONE',  ( -1.655278471874999990, 20.36702641396248481, -31.01827246956613493 ) ) ;
#17767=CARTESIAN_POINT ( 'NONE',  ( -3.500000000000000000, 19.52072594216371826, -106.7380641367107614 ) ) ;
#17768=CARTESIAN_POINT ( 'NONE',  ( 2.340729813953370519E-16, 21.32270188528332255, -131.0141058028994792 ) ) ;
#17773=CARTESIAN_POINT ( 'NONE',  ( -3.310556943750001313, 17.50000000000002132, -122.8516058028994564 ) ) ;
#17774=CARTESIAN_POINT ( 'NONE',  ( 1.750000000000001110, 20.53108891324554719, -42.29431413575483845 ) ) ;
#17775=CARTESIAN_POINT ( 'NONE',  ( 2.340729813953370519E-16, 21.32270188528331190, -84.01410580289947916 ) ) ;
#17776=CARTESIAN_POINT ( 'NONE',  ( 4.648177544792955347E-16, 21.00000000000001421, -49.90473080337742573 ) ) ;
#17777=CARTESIAN_POINT ( 'NONE',  ( 4.648177544792955347E-16, 21.00000000000001066, -23.90473080337742928 ) ) ;
#17778=CARTESIAN_POINT ( 'NONE',  ( 3.310556943749999981, 15.58864905735837780, -142.4349391362327992 ) ) ;
#17779=CARTESIAN_POINT ( 'NONE',  ( -3.500000000000001332, 17.50000000000001421, -69.65473080337743284 ) ) ;
#17781=CARTESIAN_POINT ( 'NONE',  ( 3.310556943750001313, 19.41135094264166483, -55.26827246956612782 ) ) ;
#17784=CARTESIAN_POINT ( 'NONE',  ( 1.655278471874998436, 14.63297358603754361, -76.51827246956612782 ) ) ;
#17786=CARTESIAN_POINT ( 'NONE',  ( 3.310556943749999981, 15.58864905735837070, -106.3474391362328078 ) ) ;
#17787=CARTESIAN_POINT ( 'NONE',  ( 1.655278471874998436, 14.63297358603754361, -75.43077246956613635 ) ) ;
#17789=CARTESIAN_POINT ( 'NONE',  ( -7.022189441860112050E-16, 13.67729811471672541, -98.60160580289947063 ) ) ;
#17791=CARTESIAN_POINT ( 'NONE',  ( 4.648177544792955347E-16, 21.00000000000001776, -91.21098080242150274 ) ) ;
#17792=CARTESIAN_POINT ( 'NONE',  ( 0.9378221735089300459, 21.00000000000001421, -50.94938900211594301 ) ) ;
#17793=CARTESIAN_POINT ( 'NONE',  ( 4.648177544792955347E-16, 21.00000000000002132, -117.2109808024215170 ) ) ;
#17794=CARTESIAN_POINT ( 'NONE',  ( -3.310556943750002201, 15.58864905735836892, -55.68077246956614346 ) ) ;
#17795=CARTESIAN_POINT ( 'NONE',  ( -0.9378221735089291577, 21.00000000000002132, -113.1663226036829712 ) ) ;
#17796=CARTESIAN_POINT ( 'NONE',  ( -1.655278471874999990, 20.36702641396249547, -117.9307724695661364 ) ) ;
#17797=CARTESIAN_POINT ( 'NONE',  ( 1.749999999999998224, 14.46891108675448123, -84.62764746908817415 ) ) ;
#17798=ORIENTED_EDGE ( 'NONE', *, *, #20638, .F. ) ;
#17801=ORIENTED_EDGE ( 'NONE', *, *, #20482, .T. ) ;
#17803=CARTESIAN_POINT ( 'NONE',  ( 1.655278471874998436, 14.63297358603754361, -70.43077246956613635 ) ) ;
#17807=CARTESIAN_POINT ( 'NONE',  ( -1.749999999999999778, 20.53108891324556140, -131.1276474690881741 ) ) ;
#17808=VECTOR ( 'NONE', #6067, 1000.000000000000000 ) ;
#17813=VERTEX_POINT ( 'NONE', #2002 ) ;
#17815=CARTESIAN_POINT ( 'NONE',  ( 3.310556943750001313, 19.41135094264166838, -128.1807724695661364 ) ) ;
#17817=CARTESIAN_POINT ( 'NONE',  ( -1.655278471875002211, 14.63297358603754006, -30.68493913623279568 ) ) ;
#17818=CARTESIAN_POINT ( 'NONE',  ( 3.310556943750001313, 17.50000000000001776, -91.35160580289947063 ) ) ;
#17819=CARTESIAN_POINT ( 'NONE',  ( 3.500000000000000000, 15.47927405783631727, -25.23806413671076143 ) ) ;
#17820=EDGE_CURVE ( 'NONE', #38292, #104, #30622, .T. ) ;
#17823=CARTESIAN_POINT ( 'NONE',  ( 1.655278471875001101, 20.36702641396249902, -139.1849391362327708 ) ) ;
#17825=CARTESIAN_POINT ( 'NONE',  ( -3.500000000000001332, 17.50000000000001776, -96.96098080242150274 ) ) ;
#17827=CARTESIAN_POINT ( 'NONE',  ( -3.500000000000000888, 19.52072594216371115, -86.73806413671076143 ) ) ;
#17828=CARTESIAN_POINT ( 'NONE',  ( -7.022189441860112050E-16, 13.67729811471672186, -68.60160580289947063 ) ) ;
#17830=CARTESIAN_POINT ( 'NONE',  ( 0.9378221735089281585, 14.00000000000001776, -84.36007260463890134 ) ) ;
#17832=FACE_OUTER_BOUND ( 'NONE', #37010, .T. ) ;
#17833=CARTESIAN_POINT ( 'NONE',  ( -1.750000000000002220, 14.46891108675447768, -49.79431413575484555 ) ) ;
#17834=CARTESIAN_POINT ( 'NONE',  ( -3.310556943750001313, 17.50000000000002132, -118.7641058028994792 ) ) ;
#17836=( BOUNDED_CURVE ( )  B_SPLINE_CURVE ( 2, ( #17949, #1784, #31745, #38137, #22185, #8996, #18576, #30926, #18364 ),
 .UNSPECIFIED., .F., .F. ) 
 B_SPLINE_CURVE_WITH_KNOTS ( ( 3, 2, 2, 2, 3 ),
 ( 0.02708333333333333426, 0.02777777777777777624, 0.02916666666666666713, 0.03055555555555555455, 0.03125000000000000000 ),
 .UNSPECIFIED. ) 
 CURVE ( )  GEOMETRIC_REPRESENTATION_ITEM ( )  RATIONAL_B_SPLINE_CURVE ( ( 0.9330127018922194093, 0.9330127018922195203, 1.000000000000000000, 0.8660254037844387076, 1.000000000000000000, 0.8660254037844387076, 1.000000000000000000, 0.9330127018922191873, 0.9330127018922194093 ) ) 
 REPRESENTATION_ITEM ( '' )  );
#17837=CARTESIAN_POINT ( 'NONE',  ( 0.9378221735088952959, 21.00000000000004263, -103.2556390011600058 ) ) ;
#17838=EDGE_LOOP ( 'NONE', ( #20158, #22930, #12296, #23416 ) ) ;
#17839=EDGE_CURVE ( 'NONE', #21111, #13493, #21920, .T. ) ;
#17840=CARTESIAN_POINT ( 'NONE',  ( -1.750000000000002220, 14.46891108675448656, -113.4880641367107614 ) ) ;
#17842=CARTESIAN_POINT ( 'NONE',  ( -1.749999999999999778, 20.53108891324555429, -83.82139747004410424 ) ) ;
#17846=CARTESIAN_POINT ( 'NONE',  ( -1.655278471874999990, 20.36702641396248836, -73.93077246956613635 ) ) ;
#17848=CARTESIAN_POINT ( 'NONE',  ( -8.715332896486792803E-15, 21.00000000000002842, -136.9047308033774186 ) ) ;
#17849=VECTOR ( 'NONE', #26336, 1000.000000000000000 ) ;
#17853=CARTESIAN_POINT ( 'NONE',  ( 2.340729813953370519E-16, 21.32270188528331190, -84.01410580289947916 ) ) ;
#17855=EDGE_LOOP ( 'NONE', ( #8362, #38396, #5565, #5457 ) ) ;
#17859=CARTESIAN_POINT ( 'NONE',  ( 0.9378221735089281585, 14.00000000000002132, -102.6663226036829855 ) ) ;
#17860=EDGE_CURVE ( 'NONE', #39932, #34588, #2926, .T. ) ;
#17861=EDGE_CURVE ( 'NONE', #6296, #12051, #41020, .T. ) ;
#17864=CARTESIAN_POINT ( 'NONE',  ( 1.655278471875001101, 20.36702641396248836, -50.18493913623279923 ) ) ;
#17865=CARTESIAN_POINT ( 'NONE',  ( 1.655278471875001101, 20.36702641396249547, -116.1849391362327850 ) ) ;
#17867=CARTESIAN_POINT ( 'NONE',  ( 3.500000000000000000, 15.47927405783632970, -122.2380641367107614 ) ) ;
#17868=CARTESIAN_POINT ( 'NONE',  ( -3.310556943750001313, 17.50000000000001066, -32.76410580289947205 ) ) ;
#17869=CARTESIAN_POINT ( 'NONE',  ( -3.310556943750002645, 15.58864905735836892, -65.76827246956611361 ) ) ;
#17870=CARTESIAN_POINT ( 'NONE',  ( 3.500000000000001332, 17.50000000000002132, -112.4609808024215027 ) ) ;
#17872=CARTESIAN_POINT ( 'NONE',  ( 1.655278471875001101, 20.36702641396249192, -99.09743913623280775 ) ) ;
#17877=AXIS2_PLACEMENT_3D ( 'NONE', #8693, #41245, #11267 ) ;
#17879=CARTESIAN_POINT ( 'NONE',  ( 1.750000000000001110, 20.53108891324555074, -63.29431413575484555 ) ) ;
#17880=FACE_OUTER_BOUND ( 'NONE', #21468, .T. ) ;
#17881=CARTESIAN_POINT ( 'NONE',  ( 1.655278471874998436, 14.63297358603753828, -33.43077246956615056 ) ) ;
#17882=CARTESIAN_POINT ( 'NONE',  ( 2.340729813953370519E-16, 21.32270188528331190, -91.10160580289947063 ) ) ;
#17883=EDGE_CURVE ( 'NONE', #20991, #23881, #29401, .T. ) ;
#17884=CARTESIAN_POINT ( 'NONE',  ( 1.750000000000001110, 20.53108891324555074, -53.98806413671076854 ) ) ;
#17885=CARTESIAN_POINT ( 'NONE',  ( 3.310556943749999981, 15.58864905735837070, -105.4349391362328134 ) ) ;
#17886=CARTESIAN_POINT ( 'NONE',  ( 3.310556943750001313, 19.41135094264166128, -38.26827246956612782 ) ) ;
#17888=CARTESIAN_POINT ( 'NONE',  ( 0.9378221735089213862, 21.00000000000003197, -135.2556390011599774 ) ) ;
#17894=CARTESIAN_POINT ( 'NONE',  ( 2.340729813953370519E-16, 21.32270188528331190, -87.01410580289947916 ) ) ;
#17898=CARTESIAN_POINT ( 'NONE',  ( -0.9378221735089291577, 21.00000000000001421, -50.86007260463890844 ) ) ;
#17904=ORIENTED_EDGE ( 'NONE', *, *, #17742, .T. ) ;
#17910=( BOUNDED_CURVE ( )  B_SPLINE_CURVE ( 2, ( #12026, #21817, #31386, #21395, #14608, #8212, #25019, #37563, #17793 ),
 .UNSPECIFIED., .F., .T. ) 
 B_SPLINE_CURVE_WITH_KNOTS ( ( 3, 2, 2, 2, 3 ),
 ( 0.2145833333333333481, 0.2152777777777777901, 0.2166666666666666741, 0.2180555555555555580, 0.2187500000000000000 ),
 .UNSPECIFIED. ) 
 CURVE ( )  GEOMETRIC_REPRESENTATION_ITEM ( )  RATIONAL_B_SPLINE_CURVE ( ( 0.9330127018922194093, 0.9330127018922207416, 1.000000000000000000, 0.8660254037844387076, 1.000000000000000000, 0.8660254037844387076, 1.000000000000000000, 0.9330127018922194093, 0.9330127018922194093 ) ) 
 REPRESENTATION_ITEM ( '' )  );
#17911=ORIENTED_EDGE ( 'NONE', *, *, #24525, .T. ) ;
#17914=CARTESIAN_POINT ( 'NONE',  ( 3.310556943749999981, 15.58864905735837425, -134.3474391362328220 ) ) ;
#17916=CARTESIAN_POINT ( 'NONE',  ( 3.500000000000001332, 17.50000000000001776, -78.46098080242150274 ) ) ;
#17918=CARTESIAN_POINT ( 'NONE',  ( -1.655278471875002211, 14.63297358603755249, -128.6849391362327992 ) ) ;
#17919=CARTESIAN_POINT ( 'NONE',  ( -1.655278471874999990, 20.36702641396248836, -56.01827246956612782 ) ) ;
#17922=CARTESIAN_POINT ( 'NONE',  ( -3.500000000000001332, 17.50000000000002487, -135.6547308033774186 ) ) ;
#17925=CARTESIAN_POINT ( 'NONE',  ( 3.500000000000001776, 19.52072594216371826, -126.3776474690881599 ) ) ;
#17926=CARTESIAN_POINT ( 'NONE',  ( 1.655278471875001101, 20.36702641396249547, -114.0974391362327935 ) ) ;
#17931=CARTESIAN_POINT ( 'NONE',  ( -3.500000000000000888, 19.52072594216371115, -82.04431413575483134 ) ) ;
#17932=DIRECTION ( 'NONE',  ( -0.000000000000000000, 1.259100132267607459E-16, -1.000000000000000000 ) ) ;
#17933=CARTESIAN_POINT ( 'NONE',  ( -7.022189441860112050E-16, 13.67729811471671653, -49.51410580289947205 ) ) ;
#17934=CARTESIAN_POINT ( 'NONE',  ( -7.022189441860112050E-16, 13.67729811471672541, -104.6016058028994564 ) ) ;
#17936=AXIS2_PLACEMENT_3D ( 'NONE', #20675, #39591, #20462 ) ;
#17938=CARTESIAN_POINT ( 'NONE',  ( 1.655278471875001101, 20.36702641396249547, -129.1849391362327992 ) ) ;
#17941=CARTESIAN_POINT ( 'NONE',  ( -1.749999999999999778, 20.53108891324555785, -117.1276474690881741 ) ) ;
#17942=CARTESIAN_POINT ( 'NONE',  ( -3.500000000000001332, 17.50000000000001421, -71.65473080337743284 ) ) ;
#17943=CARTESIAN_POINT ( 'NONE',  ( 3.310556943749999981, 15.58864905735836537, -59.43493913623279923 ) ) ;
#17944=ORIENTED_EDGE ( 'NONE', *, *, #5439, .F. ) ;
#17945=CARTESIAN_POINT ( 'NONE',  ( -1.655278471874999990, 20.36702641396249192, -79.01827246956614204 ) ) ;
#17947=STYLED_ITEM('',(#42159),#38463);
#17949=CARTESIAN_POINT ( 'NONE',  ( -4.299564228933483745E-15, 21.00000000000002842, -139.9047308033774186 ) ) ;
#17953=CARTESIAN_POINT ( 'NONE',  ( 3.310556943750001313, 19.41135094264166128, -39.18077246956613635 ) ) ;
#17958=CARTESIAN_POINT ( 'NONE',  ( -7.022189441860112050E-16, 13.67729811471671653, -46.51410580289946495 ) ) ;
#17959=ORIENTED_EDGE ( 'NONE', *, *, #7204, .T. ) ;
#17961=DIRECTION ( 'NONE',  ( 0.000000000000000000, 1.000000000000000000, 0.000000000000000000 ) ) ;
#17962=CARTESIAN_POINT ( 'NONE',  ( -3.500000000000000888, 19.52072594216370405, -25.04431413575484910 ) ) ;
#17965=CARTESIAN_POINT ( 'NONE',  ( 3.500000000000001332, 17.50000000000002132, -113.1547308033774328 ) ) ;
#17966=ORIENTED_EDGE ( 'NONE', *, *, #14683, .T. ) ;
#17967=CARTESIAN_POINT ( 'NONE',  ( -1.394453263437886604E-15, 14.00000000000001776, -89.71098080242148853 ) ) ;
#17968=CARTESIAN_POINT ( 'NONE',  ( -3.500000000000000888, 19.52072594216370405, -37.04431413575484555 ) ) ;
#17973=CARTESIAN_POINT ( 'NONE',  ( 2.340729813953370519E-16, 21.32270188528330479, -25.10160580289946708 ) ) ;
#17975=CARTESIAN_POINT ( 'NONE',  ( 3.310556943750001313, 19.41135094264166838, -127.1807724695661364 ) ) ;
#17976=EDGE_CURVE ( 'NONE', #31346, #23575, #24671, .T. ) ;
#17979=CARTESIAN_POINT ( 'NONE',  ( 3.500000000000000000, 15.47927405783632082, -29.23806413671076143 ) ) ;
#17980=CARTESIAN_POINT ( 'NONE',  ( 1.655278471874998436, 14.63297358603754894, -122.5182724695661278 ) ) ;
#17981=CARTESIAN_POINT ( 'NONE',  ( 1.750000000000001110, 20.53108891324556140, -140.9880641367107614 ) ) ;
#17982=CARTESIAN_POINT ( 'NONE',  ( -3.500000000000001332, 17.50000000000001066, -40.65473080337743284 ) ) ;
#17985=CARTESIAN_POINT ( 'NONE',  ( -1.655278471875002211, 14.63297358603755427, -142.6849391362327992 ) ) ;
#17986=CARTESIAN_POINT ( 'NONE',  ( 2.474675557024783212E-16, 21.54145188432739388, -69.90473080337743284 ) ) ;
#17988=CARTESIAN_POINT ( 'NONE',  ( 3.310556943749999981, 15.58864905735836537, -55.43493913623281344 ) ) ;
#17991=CARTESIAN_POINT ( 'NONE',  ( -1.655278471874999990, 20.36702641396249192, -75.01827246956612782 ) ) ;
#17993=CARTESIAN_POINT ( 'NONE',  ( 1.655278471875001101, 20.36702641396249547, -105.0974391362328078 ) ) ;
#17994=CARTESIAN_POINT ( 'NONE',  ( -3.310556943750001313, 17.50000000000001776, -76.76410580289946495 ) ) ;
#17995=VERTEX_POINT ( 'NONE', #3461 ) ;
#17996=CARTESIAN_POINT ( 'NONE',  ( 3.310556943750001313, 19.41135094264166838, -96.26827246956612782 ) ) ;
#17998=CARTESIAN_POINT ( 'NONE',  ( -0.9378221735089291577, 21.00000000000001776, -86.86007260463891555 ) ) ;
#17999=CARTESIAN_POINT ( 'NONE',  ( -1.394453263437886604E-15, 14.00000000000001066, -37.71098080242150985 ) ) ;
#18001=CARTESIAN_POINT ( 'NONE',  ( -3.310556943750000425, 19.41135094264166483, -57.84743913623280065 ) ) ;
#18003=CARTESIAN_POINT ( 'NONE',  ( -3.310556943750001313, 17.50000000000002132, -110.7641058028994649 ) ) ;
#18004=VECTOR ( 'NONE', #25084, 1000.000000000000000 ) ;
#18006=VERTEX_POINT ( 'NONE', #3260 ) ;
#18010=CARTESIAN_POINT ( 'NONE',  ( 3.310556943750001313, 17.50000000000001421, -61.26410580289946495 ) ) ;
#18011=VERTEX_POINT ( 'NONE', #16450 ) ;
#18012=ORIENTED_EDGE ( 'NONE', *, *, #39865, .T. ) ;
#18018=CARTESIAN_POINT ( 'NONE',  ( -3.500000000000001332, 17.50000000000002487, -142.9609808024215170 ) ) ;
#18019=CARTESIAN_POINT ( 'NONE',  ( 3.310556943750001313, 17.50000000000002487, -131.2641058028994507 ) ) ;
#18020=CARTESIAN_POINT ( 'NONE',  ( 3.500000000000001332, 17.50000000000002132, -119.4609808024215170 ) ) ;
#18021=VECTOR ( 'NONE', #2219, 1000.000000000000000 ) ;
#18022=CARTESIAN_POINT ( 'NONE',  ( -1.655278471875002211, 14.63297358603754006, -37.68493913623280633 ) ) ;
#18023=CARTESIAN_POINT ( 'NONE',  ( -1.655278471874999990, 20.36702641396248481, -35.01827246956614204 ) ) ;
#18024=CARTESIAN_POINT ( 'NONE',  ( 1.655278471874998436, 14.63297358603754539, -91.51827246956612782 ) ) ;
#18025=CARTESIAN_POINT ( 'NONE',  ( 2.474675557024783212E-16, 21.54145188432739033, -24.90473080337743284 ) ) ;
#18027=( BOUNDED_CURVE ( )  B_SPLINE_CURVE ( 2, ( #8633, #21606, #15237, #41185, #12030, #8843, #38191, #9478, #19050 ),
 .UNSPECIFIED., .F., .T. ) 
 B_SPLINE_CURVE_WITH_KNOTS ( ( 3, 2, 2, 2, 3 ),
 ( 0.3437500000000000000, 0.3444444444444444420, 0.3458333333333333259, 0.3472222222222222099, 0.3479166666666666519 ),
 .UNSPECIFIED. ) 
 CURVE ( )  GEOMETRIC_REPRESENTATION_ITEM ( )  RATIONAL_B_SPLINE_CURVE ( ( 0.9330127018922194093, 0.9330127018922194093, 1.000000000000000000, 0.8660254037844387076, 1.000000000000000000, 0.8660254037844387076, 1.000000000000000000, 0.9330127018922194093, 0.9330127018922194093 ) ) 
 REPRESENTATION_ITEM ( '' )  );
#18030=CARTESIAN_POINT ( 'NONE',  ( -3.310556943750001313, 17.50000000000002487, -140.8516058028994564 ) ) ;
#18031=VECTOR ( 'NONE', #29185, 1000.000000000000000 ) ;
#18033=CARTESIAN_POINT ( 'NONE',  ( 3.500000000000001776, 19.52072594216371115, -95.37764746908815994 ) ) ;
#18035=CARTESIAN_POINT ( 'NONE',  ( -1.394453263437886604E-15, 14.00000000000001421, -61.40473080337742573 ) ) ;
#18036=CARTESIAN_POINT ( 'NONE',  ( 1.749999999999998224, 14.46891108675448123, -87.32139747004409003 ) ) ;
#18037=CARTESIAN_POINT ( 'NONE',  ( -3.310556943750000425, 19.41135094264166483, -69.93493913623279923 ) ) ;
#18039=CARTESIAN_POINT ( 'NONE',  ( -1.394453263437886604E-15, 14.00000000000002132, -111.4047308033774186 ) ) ;
#18042=DIRECTION ( 'NONE',  ( -0.000000000000000000, 1.259100132267607459E-16, -1.000000000000000000 ) ) ;
#18043=CARTESIAN_POINT ( 'NONE',  ( -3.500000000000001332, 17.50000000000001421, -47.96098080242150274 ) ) ;
#18044=CARTESIAN_POINT ( 'NONE',  ( -1.655278471875002211, 14.63297358603755072, -119.5974391362328078 ) ) ;
#18046=CARTESIAN_POINT ( 'NONE',  ( 1.749999999999998224, 14.46891108675448301, -95.62764746908817415 ) ) ;
#18049=CARTESIAN_POINT ( 'NONE',  ( 2.474675557024783212E-16, 21.54145188432740099, -111.9047308033774186 ) ) ;
#18051=DIRECTION ( 'NONE',  ( 0.000000000000000000, 1.000000000000000000, 0.000000000000000000 ) ) ;
#18052=DIRECTION ( 'NONE',  ( 0.000000000000000000, 1.000000000000000000, 0.000000000000000000 ) ) ;
#18055=CARTESIAN_POINT ( 'NONE',  ( -1.655278471875002211, 14.63297358603754539, -70.59743913623280775 ) ) ;
#18056=CARTESIAN_POINT ( 'NONE',  ( 3.500000000000000000, 15.47927405783633326, -116.2380641367107614 ) ) ;
#18057=CARTESIAN_POINT ( 'NONE',  ( 3.500000000000001332, 19.52072594216370760, -69.37764746908817415 ) ) ;
#18058=ORIENTED_EDGE ( 'NONE', *, *, #6396, .F. ) ;
#18059=CARTESIAN_POINT ( 'NONE',  ( -1.749999999999999778, 20.53108891324555785, -104.1276474690881741 ) ) ;
#18061=CARTESIAN_POINT ( 'NONE',  ( 3.310556943750001313, 17.50000000000001776, -83.26410580289947916 ) ) ;
#18062=ADVANCED_FACE ( 'NONE', ( #9435 ), #35795, .T. ) ;
#18064=ORIENTED_EDGE ( 'NONE', *, *, #39167, .T. ) ;
#18065=AXIS2_PLACEMENT_3D ( 'NONE', #6189, #9170, #3000 ) ;
#18067=ADVANCED_FACE ( 'NONE', ( #35380 ), #12629, .T. ) ;
#18069=CARTESIAN_POINT ( 'NONE',  ( 0.000000000000000000, 17.50000000000002487, -149.5231586289125687 ) ) ;
#18071=CARTESIAN_POINT ( 'NONE',  ( 0.000000000000000000, 20.99999999999998934, 153.5815388724490163 ) ) ;
#18072=CARTESIAN_POINT ( 'NONE',  ( 1.655278471874998436, 14.63297358603754006, -48.51827246956613493 ) ) ;
#18073=CARTESIAN_POINT ( 'NONE',  ( -3.310556943750000425, 19.41135094264166838, -108.9349391362327992 ) ) ;
#18075=( BOUNDED_CURVE ( )  B_SPLINE_CURVE ( 2, ( #14238, #27217, #22958, #35927, #32733, #3599, #19985, #619, #16592 ),
 .UNSPECIFIED., .F., .F. ) 
 B_SPLINE_CURVE_WITH_KNOTS ( ( 3, 2, 2, 2, 3 ),
 ( 0.3395833333333333481, 0.3402777777777777901, 0.3416666666666666741, 0.3430555555555555580, 0.3437500000000000000 ),
 .UNSPECIFIED. ) 
 CURVE ( )  GEOMETRIC_REPRESENTATION_ITEM ( )  RATIONAL_B_SPLINE_CURVE ( ( 0.9330127018922194093, 0.9330127018922194093, 1.000000000000000000, 0.8660254037844387076, 1.000000000000000000, 0.8660254037844387076, 1.000000000000000000, 0.9330127018922194093, 0.9330127018922194093 ) ) 
 REPRESENTATION_ITEM ( '' )  );
#18076=CARTESIAN_POINT ( 'NONE',  ( 2.340729813953370519E-16, 21.32270188528330479, -35.01410580289947205 ) ) ;
#18077=CARTESIAN_POINT ( 'NONE',  ( 3.310556943749999981, 15.58864905735836714, -68.43493913623279923 ) ) ;
#18078=CARTESIAN_POINT ( 'NONE',  ( -3.500000000000000888, 19.52072594216371826, -114.0443141357548171 ) ) ;
#18080=CARTESIAN_POINT ( 'NONE',  ( -1.655278471874999990, 20.36702641396249192, -95.93077246956613635 ) ) ;
#18081=CARTESIAN_POINT ( 'NONE',  ( -1.394453263437886604E-15, 14.00000000000001421, -60.40473080337743284 ) ) ;
#18082=CARTESIAN_POINT ( 'NONE',  ( -3.500000000000002220, 15.47927405783633503, -124.5713974700440900 ) ) ;
#18085=CARTESIAN_POINT ( 'NONE',  ( 3.500000000000000000, 15.47927405783632260, -63.54431413575484555 ) ) ;
#18087=CARTESIAN_POINT ( 'NONE',  ( -3.310556943750001313, 17.50000000000001066, -30.76410580289946850 ) ) ;
#18088=CARTESIAN_POINT ( 'NONE',  ( 1.655278471874998436, 14.63297358603754539, -88.51827246956612782 ) ) ;
#18089=EDGE_CURVE ( 'NONE', #38089, #24772, #26602, .T. ) ;
#18090=CARTESIAN_POINT ( 'NONE',  ( 3.500000000000001332, 17.50000000000001421, -55.15473080337743284 ) ) ;
#18091=CARTESIAN_POINT ( 'NONE',  ( -0.9378221735089335986, 21.00000000000002842, -138.1663226036829997 ) ) ;
#18093=CARTESIAN_POINT ( 'NONE',  ( -1.655278471874999990, 20.36702641396249547, -107.0182724695661278 ) ) ;
#18094=CARTESIAN_POINT ( 'NONE',  ( 2.340729813953370519E-16, 21.32270188528330834, -40.10160580289947063 ) ) ;
#18100=CYLINDRICAL_SURFACE ( 'NONE', #724, 3.499999999999999556 ) ;
#18102=CARTESIAN_POINT ( 'NONE',  ( 2.340729813953370519E-16, 21.32270188528331190, -86.01410580289947916 ) ) ;
#18103=CARTESIAN_POINT ( 'NONE',  ( -3.500000000000000000, 19.52072594216371826, -135.7380641367107614 ) ) ;
#18107=CARTESIAN_POINT ( 'NONE',  ( -3.500000000000002220, 15.47927405783632615, -64.87764746908818836 ) ) ;
#18110=CARTESIAN_POINT ( 'NONE',  ( -0.9378221735089291577, 21.00000000000001066, -31.16632260368298901 ) ) ;
#18113=ORIENTED_EDGE ( 'NONE', *, *, #3802, .F. ) ;
#18114=LINE ( 'NONE', #27681, #19104 ) ;
#18115=ORIENTED_EDGE ( 'NONE', *, *, #7204, .F. ) ;
#18120=ADVANCED_FACE ( 'NONE', ( #23465 ), #33698, .T. ) ;
#18125=CARTESIAN_POINT ( 'NONE',  ( -3.310556943750002645, 15.58864905735837958, -138.6807724695661364 ) ) ;
#18126=CARTESIAN_POINT ( 'NONE',  ( 1.749999999999998224, 14.46891108675447946, -78.62764746908817415 ) ) ;
#18127=ORIENTED_EDGE ( 'NONE', *, *, #6019, .T. ) ;
#18128=CARTESIAN_POINT ( 'NONE',  ( 1.655278471875001101, 20.36702641396249547, -125.1849391362327992 ) ) ;
#18129=CARTESIAN_POINT ( 'NONE',  ( -3.310556943750000425, 19.41135094264166128, -54.93493913623280633 ) ) ;
#18132=CARTESIAN_POINT ( 'NONE',  ( 1.749999999999998224, 14.46891108675448834, -138.3213974700441042 ) ) ;
#18134=CARTESIAN_POINT ( 'NONE',  ( 1.750000000000001110, 20.53108891324555785, -128.2943141357548313 ) ) ;
#18135=CARTESIAN_POINT ( 'NONE',  ( -1.655278471875002211, 14.63297358603755072, -110.5974391362328078 ) ) ;
#18139=CARTESIAN_POINT ( 'NONE',  ( 1.750000000000001110, 20.53108891324555429, -78.29431413575484555 ) ) ;
#18141=CARTESIAN_POINT ( 'NONE',  ( 1.655278471874998436, 14.63297358603754006, -49.43077246956615056 ) ) ;
#18142=CARTESIAN_POINT ( 'NONE',  ( 2.340729813953370519E-16, 21.32270188528331900, -107.1016058028994706 ) ) ;
#18144=CARTESIAN_POINT ( 'NONE',  ( -0.9378221735089310451, 14.00000000000001066, -42.44938900211595012 ) ) ;
#18145=CARTESIAN_POINT ( 'NONE',  ( -1.749999999999999778, 20.53108891324555074, -72.82139747004409003 ) ) ;
#18146=CARTESIAN_POINT ( 'NONE',  ( -1.655278471874999990, 20.36702641396249547, -123.0182724695661278 ) ) ;
#18149=CARTESIAN_POINT ( 'NONE',  ( 4.648177544792955347E-16, 21.00000000000002132, -117.2109808024215170 ) ) ;
#18150=CARTESIAN_POINT ( 'NONE',  ( -3.500000000000001332, 17.50000000000001421, -57.65473080337743284 ) ) ;
#18151=CARTESIAN_POINT ( 'NONE',  ( 3.310556943750001313, 17.50000000000001421, -60.35160580289947063 ) ) ;
#18153=CARTESIAN_POINT ( 'NONE',  ( 2.340729813953370519E-16, 21.32270188528331190, -77.10160580289944221 ) ) ;
#18155=CARTESIAN_POINT ( 'NONE',  ( 0.000000000000000000, 17.50000000000002487, -149.5231586289125687 ) ) ;
#18157=CARTESIAN_POINT ( 'NONE',  ( -1.394453263437886604E-15, 14.00000000000001421, -55.71098080242150274 ) ) ;
#18158=EDGE_CURVE ( 'NONE', #20208, #5302, #11609, .T. ) ;
#18159=CARTESIAN_POINT ( 'NONE',  ( 1.743066579297357930E-14, 14.00000000000002132, -128.4047308033774186 ) ) ;
#18162=CARTESIAN_POINT ( 'NONE',  ( 2.340729813953370519E-16, 21.32270188528330834, -38.01410580289947205 ) ) ;
#18163=DIRECTION ( 'NONE',  ( -0.000000000000000000, -0.000000000000000000, 1.000000000000000000 ) ) ;
#18164=VERTEX_POINT ( 'NONE', #26299 ) ;
#18166=ORIENTED_EDGE ( 'NONE', *, *, #1194, .F. ) ;
#18169=CARTESIAN_POINT ( 'NONE',  ( -3.310556943750002645, 15.58864905735836714, -45.68077246956614346 ) ) ;
#18171=ORIENTED_EDGE ( 'NONE', *, *, #22052, .T. ) ;
#18173=CARTESIAN_POINT ( 'NONE',  ( -3.500000000000002220, 15.47927405783632082, -23.87764746908817415 ) ) ;
#18175=CARTESIAN_POINT ( 'NONE',  ( 0.000000000000000000, 21.00000000000002487, -149.5231586289125687 ) ) ;
#18177=CARTESIAN_POINT ( 'NONE',  ( -7.424026671074350129E-16, 13.45854811567263098, -38.71098080242150985 ) ) ;
#18179=CARTESIAN_POINT ( 'NONE',  ( -1.394453263437886604E-15, 14.00000000000001421, -76.71098080242148853 ) ) ;
#18181=CARTESIAN_POINT ( 'NONE',  ( -3.310556943750001313, 17.50000000000001066, -23.85160580289946708 ) ) ;
#18183=CARTESIAN_POINT ( 'NONE',  ( 3.310556943750001313, 19.41135094264167549, -131.1807724695661364 ) ) ;
#18186=DIRECTION ( 'NONE',  ( -0.000000000000000000, 1.259100132267607459E-16, -1.000000000000000000 ) ) ;
#18187=CARTESIAN_POINT ( 'NONE',  ( -7.022189441860112050E-16, 13.67729811471672718, -123.6016058028994564 ) ) ;
#18189=CARTESIAN_POINT ( 'NONE',  ( -3.500000000000000888, 19.52072594216370405, -38.73806413671077564 ) ) ;
#18192=CARTESIAN_POINT ( 'NONE',  ( 1.655278471875001101, 20.36702641396249902, -137.1849391362327992 ) ) ;
#18194=CARTESIAN_POINT ( 'NONE',  ( -7.424026671074350129E-16, 13.45854811567263454, -68.40473080337743284 ) ) ;
#18195=CYLINDRICAL_SURFACE ( 'NONE', #32082, 3.499999999999999556 ) ;
#18196=CARTESIAN_POINT ( 'NONE',  ( 1.655278471875001101, 20.36702641396248836, -50.18493913623279923 ) ) ;
#18198=CARTESIAN_POINT ( 'NONE',  ( -1.750000000000002220, 14.46891108675447768, -41.48806413671076143 ) ) ;
#18199=CARTESIAN_POINT ( 'NONE',  ( 1.655278471875001101, 20.36702641396249192, -77.18493913623279923 ) ) ;
#18201=CARTESIAN_POINT ( 'NONE',  ( -3.310556943750001313, 17.50000000000002132, -102.7641058028994649 ) ) ;
#18202=CARTESIAN_POINT ( 'NONE',  ( -1.655278471874999990, 20.36702641396248836, -70.93077246956613635 ) ) ;
#18203=ORIENTED_EDGE ( 'NONE', *, *, #18840, .F. ) ;
#18204=CARTESIAN_POINT ( 'NONE',  ( 3.310556943749999981, 15.58864905735837070, -95.43493913623279923 ) ) ;
#18205=( BOUNDED_CURVE ( )  B_SPLINE_CURVE ( 2, ( #38238, #31851, #2719, #31433, #37819, #19096, #32063, #28242, #41651 ),
 .UNSPECIFIED., .F., .T. ) 
 B_SPLINE_CURVE_WITH_KNOTS ( ( 3, 2, 2, 2, 3 ),
 ( 0.5020833333333333259, 0.5027777777777777679, 0.5041666666666666519, 0.5055555555555555358, 0.5062499999999999778 ),
 .UNSPECIFIED. ) 
 CURVE ( )  GEOMETRIC_REPRESENTATION_ITEM ( )  RATIONAL_B_SPLINE_CURVE ( ( 0.9330127018922194093, 0.9330127018922194093, 1.000000000000000000, 0.8660254037844387076, 1.000000000000000000, 0.8660254037844387076, 1.000000000000000000, 0.9330127018922194093, 0.9330127018922194093 ) ) 
 REPRESENTATION_ITEM ( '' )  );
#18208=LINE ( 'NONE', #21394, #32213 ) ;
#18210=CARTESIAN_POINT ( 'NONE',  ( -3.310556943750000425, 19.41135094264166483, -54.84743913623281486 ) ) ;
#18211=CARTESIAN_POINT ( 'NONE',  ( -1.394453263437886604E-15, 14.00000000000001421, -62.40473080337742573 ) ) ;
#18212=CARTESIAN_POINT ( 'NONE',  ( 3.310556943750001313, 19.41135094264166838, -112.1807724695661506 ) ) ;
#18213=EDGE_LOOP ( 'NONE', ( #30416, #19003, #26571, #31331 ) ) ;
#18214=VERTEX_POINT ( 'NONE', #36273 ) ;
#18219=CARTESIAN_POINT ( 'NONE',  ( 1.655278471875001101, 20.36702641396248836, -62.09743913623280775 ) ) ;
#18221=EDGE_LOOP ( 'NONE', ( #22191, #911, #35778, #21874 ) ) ;
#18226=VERTEX_POINT ( 'NONE', #30101 ) ;
#18228=CARTESIAN_POINT ( 'NONE',  ( 3.310556943749999981, 15.58864905735837425, -129.3474391362328220 ) ) ;
#18230=CARTESIAN_POINT ( 'NONE',  ( -1.655278471875002211, 14.63297358603754006, -38.68493913623280633 ) ) ;
#18231=CARTESIAN_POINT ( 'NONE',  ( -7.022189441860112050E-16, 13.67729811471671475, -30.60160580289945997 ) ) ;
#18232=CARTESIAN_POINT ( 'NONE',  ( -1.655278471874999990, 20.36702641396249192, -94.01827246956612782 ) ) ;
#18233=CARTESIAN_POINT ( 'NONE',  ( -1.749999999999999778, 20.53108891324554719, -24.82139747004409713 ) ) ;
#18236=CARTESIAN_POINT ( 'NONE',  ( 3.310556943750001313, 19.41135094264167549, -140.2682724695661420 ) ) ;
#18239=CARTESIAN_POINT ( 'NONE',  ( 4.648177544792955347E-16, 21.00000000000001421, -61.90473080337742573 ) ) ;
#18240=CARTESIAN_POINT ( 'NONE',  ( 3.500000000000001332, 17.50000000000001776, -86.15473080337743284 ) ) ;
#18241=CARTESIAN_POINT ( 'NONE',  ( -7.022189441860112050E-16, 13.67729811471672186, -70.60160580289947063 ) ) ;
#18244=CARTESIAN_POINT ( 'NONE',  ( -0.9378221735089291577, 21.00000000000001421, -58.86007260463891555 ) ) ;
#18246=CARTESIAN_POINT ( 'NONE',  ( -3.500000000000001332, 17.50000000000001421, -50.96098080242150985 ) ) ;
#18247=VECTOR ( 'NONE', #2516, 1000.000000000000000 ) ;
#18248=CARTESIAN_POINT ( 'NONE',  ( 1.655278471874998436, 14.63297358603754894, -119.4307724695661364 ) ) ;
#18249=DIRECTION ( 'NONE',  ( -0.000000000000000000, 1.259100132267607459E-16, -1.000000000000000000 ) ) ;
#18251=ORIENTED_EDGE ( 'NONE', *, *, #27718, .T. ) ;
#18252=CARTESIAN_POINT ( 'NONE',  ( -3.500000000000002220, 15.47927405783633503, -111.5713974700441042 ) ) ;
#18254=CARTESIAN_POINT ( 'NONE',  ( 4.286263797015737581E-16, 14.00000000000002487, -149.5231586289125687 ) ) ;
#18255=CARTESIAN_POINT ( 'NONE',  ( 0.000000000000000000, 17.50000000000002487, -149.5231586289125687 ) ) ;
#18258=CARTESIAN_POINT ( 'NONE',  ( -1.655278471874999990, 20.36702641396248836, -69.93077246956613635 ) ) ;
#18259=CARTESIAN_POINT ( 'NONE',  ( 4.648177544792955347E-16, 21.00000000000001776, -78.90473080337741862 ) ) ;
#18260=DIRECTION ( 'NONE',  ( 0.000000000000000000, 1.000000000000000000, 0.000000000000000000 ) ) ;
#18261=ORIENTED_EDGE ( 'NONE', *, *, #9034, .T. ) ;
#18262=CARTESIAN_POINT ( 'NONE',  ( -3.310556943750001313, 17.50000000000001066, -24.76410580289947916 ) ) ;
#18263=CARTESIAN_POINT ( 'NONE',  ( -0.9378221735089310451, 14.00000000000001066, -31.75563900116002714 ) ) ;
#18264=CARTESIAN_POINT ( 'NONE',  ( 3.310556943749999981, 15.58864905735836714, -78.34743913623280775 ) ) ;
#18267=DIRECTION ( 'NONE',  ( 0.000000000000000000, 1.000000000000000000, 0.000000000000000000 ) ) ;
#18268=( BOUNDED_CURVE ( )  B_SPLINE_CURVE ( 2, ( #16954, #39706, #16337, #3550, #366, #23121, #25903, #38870, #20147 ),
 .UNSPECIFIED., .F., .F. ) 
 B_SPLINE_CURVE_WITH_KNOTS ( ( 3, 2, 2, 2, 3 ),
 ( 0.4020833333333333481, 0.4027777777777777901, 0.4041666666666666741, 0.4055555555555555580, 0.4062500000000000000 ),
 .UNSPECIFIED. ) 
 CURVE ( )  GEOMETRIC_REPRESENTATION_ITEM ( )  RATIONAL_B_SPLINE_CURVE ( ( 0.9330127018922194093, 0.9330127018922194093, 1.000000000000000000, 0.8660254037844387076, 1.000000000000000000, 0.8660254037844387076, 1.000000000000000000, 0.9330127018922194093, 0.9330127018922194093 ) ) 
 REPRESENTATION_ITEM ( '' )  );
#18274=CARTESIAN_POINT ( 'NONE',  ( 3.310556943749999981, 15.58864905735836182, -47.43493913623279923 ) ) ;
#18275=CARTESIAN_POINT ( 'NONE',  ( 3.310556943749999981, 15.58864905735837247, -110.4349391362328134 ) ) ;
#18278=CARTESIAN_POINT ( 'NONE',  ( 3.310556943750001313, 17.50000000000001066, -33.26410580289947205 ) ) ;
#18279=CARTESIAN_POINT ( 'NONE',  ( 3.310556943750001313, 17.50000000000001421, -60.35160580289947063 ) ) ;
#18280=CARTESIAN_POINT ( 'NONE',  ( -3.500000000000001332, 17.50000000000002132, -114.9609808024215027 ) ) ;
#18282=CARTESIAN_POINT ( 'NONE',  ( 3.310556943750001313, 17.50000000000001776, -98.26410580289947916 ) ) ;
#18283=CARTESIAN_POINT ( 'NONE',  ( -1.749999999999999778, 20.53108891324554719, -26.12764746908817415 ) ) ;
#18286=CARTESIAN_POINT ( 'NONE',  ( -3.500000000000000888, 19.52072594216370760, -64.04431413575484555 ) ) ;
#18288=CARTESIAN_POINT ( 'NONE',  ( 3.310556943750001313, 17.50000000000001066, -31.26410580289946850 ) ) ;
#18289=CARTESIAN_POINT ( 'NONE',  ( 2.474675557024783212E-16, 21.54145188432739388, -55.90473080337744705 ) ) ;
#18291=CARTESIAN_POINT ( 'NONE',  ( -3.310556943750001313, 17.50000000000002132, -106.8516058028994564 ) ) ;
#18292=CARTESIAN_POINT ( 'NONE',  ( 3.310556943750001313, 17.50000000000001066, -36.35160580289946353 ) ) ;
#18294=CARTESIAN_POINT ( 'NONE',  ( 0.9378221735089367073, 14.00000000000002487, -135.6663226036829712 ) ) ;
#18298=FACE_OUTER_BOUND ( 'NONE', #39556, .T. ) ;
#18301=CARTESIAN_POINT ( 'NONE',  ( 3.310556943749999981, 15.58864905735836892, -87.34743913623280775 ) ) ;
#18302=CARTESIAN_POINT ( 'NONE',  ( 4.648177544792955347E-16, 21.00000000000002132, -116.9047308033774328 ) ) ;
#18303=CARTESIAN_POINT ( 'NONE',  ( -1.750000000000002220, 14.46891108675447413, -23.79431413575484910 ) ) ;
#18304=ORIENTED_EDGE ( 'NONE', *, *, #40777, .F. ) ;
#18307=VERTEX_POINT ( 'NONE', #36059 ) ;
#18311=ORIENTED_EDGE ( 'NONE', *, *, #36751, .F. ) ;
#18313=ORIENTED_EDGE ( 'NONE', *, *, #31575, .F. ) ;
#18319=VERTEX_POINT ( 'NONE', #5207 ) ;
#18320=EDGE_CURVE ( 'NONE', #13141, #7438, #14926, .T. ) ;
#18321=CARTESIAN_POINT ( 'NONE',  ( -1.394453263437886604E-15, 14.00000000000001776, -91.40473080337741862 ) ) ;
#18322=( BOUNDED_CURVE ( )  B_SPLINE_CURVE ( 2, ( #11754, #37300, #14122, #24750, #8359 ),
 .UNSPECIFIED., .F., .T. ) 
 B_SPLINE_CURVE_WITH_KNOTS ( ( 3, 2, 3 ),
 ( 0.000000000000000000, 0.001388888888888888942, 0.002083333333333334605 ),
 .UNSPECIFIED. ) 
 CURVE ( )  GEOMETRIC_REPRESENTATION_ITEM ( )  RATIONAL_B_SPLINE_CURVE ( ( 1.000000000000000000, 0.8660254037844387076, 1.000000000000000000, 0.9330127018922191873, 0.9330127018922192983 ) ) 
 REPRESENTATION_ITEM ( '' )  );
#18323=FACE_OUTER_BOUND ( 'NONE', #15718, .T. ) ;
#18325=CARTESIAN_POINT ( 'NONE',  ( 2.340729813953370519E-16, 21.32270188528332255, -136.0141058028994792 ) ) ;
#18326=CARTESIAN_POINT ( 'NONE',  ( 4.648177544792955347E-16, 21.00000000000001776, -78.21098080242148853 ) ) ;
#18328=FACE_OUTER_BOUND ( 'NONE', #33722, .T. ) ;
#18329=CARTESIAN_POINT ( 'NONE',  ( -1.655278471875002211, 14.63297358603755249, -123.6849391362327992 ) ) ;
#18330=CARTESIAN_POINT ( 'NONE',  ( -1.655278471874999990, 20.36702641396248836, -57.01827246956612782 ) ) ;
#18333=CARTESIAN_POINT ( 'NONE',  ( 2.474675557024783212E-16, 21.54145188432740810, -134.9047308033774186 ) ) ;
#18336=CARTESIAN_POINT ( 'NONE',  ( 1.655278471875001101, 20.36702641396249192, -75.18493913623279923 ) ) ;
#18337=CARTESIAN_POINT ( 'NONE',  ( 3.500000000000001776, 19.52072594216371826, -127.3776474690881741 ) ) ;
#18338=CARTESIAN_POINT ( 'NONE',  ( -7.022189441860112050E-16, 13.67729811471672718, -111.5141058028994649 ) ) ;
#18342=CARTESIAN_POINT ( 'NONE',  ( 3.500000000000001332, 17.50000000000001776, -78.46098080242150274 ) ) ;
#18344=CARTESIAN_POINT ( 'NONE',  ( -1.655278471875002211, 14.63297358603754184, -45.59743913623280775 ) ) ;
#18346=CARTESIAN_POINT ( 'NONE',  ( -3.310556943750000425, 19.41135094264166838, -105.9349391362328134 ) ) ;
#18350=CARTESIAN_POINT ( 'NONE',  ( -3.310556943750000425, 19.41135094264166838, -123.9349391362327850 ) ) ;
#18351=CARTESIAN_POINT ( 'NONE',  ( -3.500000000000001332, 17.50000000000001421, -48.96098080242150274 ) ) ;
#18355=CARTESIAN_POINT ( 'NONE',  ( -1.394453263437886604E-15, 14.00000000000001421, -60.71098080242150985 ) ) ;
#18356=EDGE_CURVE ( 'NONE', #18958, #31245, #15983, .T. ) ;
#18357=CARTESIAN_POINT ( 'NONE',  ( -3.310556943750000425, 19.41135094264166128, -57.93493913623279923 ) ) ;
#18359=ORIENTED_EDGE ( 'NONE', *, *, #3474, .T. ) ;
#18360=CARTESIAN_POINT ( 'NONE',  ( 1.655278471875001101, 20.36702641396249192, -77.18493913623279923 ) ) ;
#18362=DIRECTION ( 'NONE',  ( 0.000000000000000000, 1.000000000000000000, 0.000000000000000000 ) ) ;
#18363=CARTESIAN_POINT ( 'NONE',  ( 3.500000000000001332, 19.52072594216371115, -80.07139747004411845 ) ) ;
#18364=CARTESIAN_POINT ( 'NONE',  ( 3.369928719974892676E-15, 14.00000000000002309, -139.4047308033773618 ) ) ;
#18368=CARTESIAN_POINT ( 'NONE',  ( 3.310556943749999981, 15.58864905735836182, -37.34743913623282197 ) ) ;
#18370=AXIS2_PLACEMENT_3D ( 'NONE', #25638, #38599, #6272 ) ;
#18372=ORIENTED_EDGE ( 'NONE', *, *, #26461, .F. ) ;
#18374=CARTESIAN_POINT ( 'NONE',  ( 2.340729813953370519E-16, 21.32270188528330834, -49.01410580289947205 ) ) ;
#18376=VERTEX_POINT ( 'NONE', #27958 ) ;
#18378=VECTOR ( 'NONE', #36049, 1000.000000000000000 ) ;
#18379=CARTESIAN_POINT ( 'NONE',  ( -3.500000000000001332, 17.50000000000001066, -23.96098080242150985 ) ) ;
#18382=CARTESIAN_POINT ( 'NONE',  ( 4.648177544792955347E-16, 21.00000000000002132, -119.9047308033774328 ) ) ;
#18383=DIRECTION ( 'NONE',  ( -0.000000000000000000, 1.259100132267607459E-16, -1.000000000000000000 ) ) ;
#18384=CARTESIAN_POINT ( 'NONE',  ( 3.500000000000000000, 15.47927405783632082, -39.54431413575485266 ) ) ;
#18386=CARTESIAN_POINT ( 'NONE',  ( -1.394453263437886604E-15, 14.00000000000001421, -63.71098080242150274 ) ) ;
#18387=EDGE_CURVE ( 'NONE', #34018, #16644, #33929, .T. ) ;
#18390=CARTESIAN_POINT ( 'NONE',  ( -3.500000000000001332, 17.50000000000002487, -142.9609808024215170 ) ) ;
#18391=EDGE_CURVE ( 'NONE', #2733, #40441, #5906, .T. ) ;
#18392=DIRECTION ( 'NONE',  ( -0.000000000000000000, 1.259100132267607459E-16, -1.000000000000000000 ) ) ;
#18395=CARTESIAN_POINT ( 'NONE',  ( 4.648177544792955347E-16, 21.00000000000001776, -93.90473080337743284 ) ) ;
#18396=CARTESIAN_POINT ( 'NONE',  ( 3.310556943749999981, 15.58864905735837425, -124.4349391362327992 ) ) ;
#18398=CARTESIAN_POINT ( 'NONE',  ( -3.500000000000001332, 17.50000000000001066, -38.65473080337743284 ) ) ;
#18401=CARTESIAN_POINT ( 'NONE',  ( 1.655278471874998436, 14.63297358603755249, -141.5182724695661420 ) ) ;
#18404=CARTESIAN_POINT ( 'NONE',  ( 3.310556943750001313, 17.50000000000001421, -50.35160580289946353 ) ) ;
#18406=CARTESIAN_POINT ( 'NONE',  ( -3.500000000000002220, 15.47927405783632437, -41.57139747004409713 ) ) ;
#18407=CARTESIAN_POINT ( 'NONE',  ( 1.655278471875001101, 20.36702641396248836, -73.18493913623279923 ) ) ;
#18409=CARTESIAN_POINT ( 'NONE',  ( 3.310556943750001313, 19.41135094264166838, -104.1807724695661221 ) ) ;
#18410=CARTESIAN_POINT ( 'NONE',  ( -3.310556943750000425, 19.41135094264166128, -70.84743913623279354 ) ) ;
#18411=ORIENTED_EDGE ( 'NONE', *, *, #30240, .T. ) ;
#18413=CARTESIAN_POINT ( 'NONE',  ( 1.655278471874998436, 14.63297358603754539, -90.51827246956612782 ) ) ;
#18417=CARTESIAN_POINT ( 'NONE',  ( 0.000000000000000000, 17.50000000000002487, -149.5231586289125687 ) ) ;
#18418=CARTESIAN_POINT ( 'NONE',  ( 0.000000000000000000, 17.50000000000002487, -149.5231586289125687 ) ) ;
#18419=CARTESIAN_POINT ( 'NONE',  ( -1.655278471874999990, 20.36702641396248836, -53.93077246956613635 ) ) ;
#18421=CARTESIAN_POINT ( 'NONE',  ( -1.655278471875002211, 14.63297358603755072, -110.5974391362328078 ) ) ;
#18427=CARTESIAN_POINT ( 'NONE',  ( -3.310556943750000425, 19.41135094264166128, -63.84743913623280775 ) ) ;
#18431=CARTESIAN_POINT ( 'NONE',  ( -1.394453263437886604E-15, 14.00000000000001066, -30.71098080242150630 ) ) ;
#18436=CARTESIAN_POINT ( 'NONE',  ( -1.394453263437886604E-15, 14.00000000000001421, -80.40473080337743284 ) ) ;
#18437=CARTESIAN_POINT ( 'NONE',  ( 2.340729813953370519E-16, 21.32270188528332255, -132.0141058028994507 ) ) ;
#18440=CARTESIAN_POINT ( 'NONE',  ( 3.310556943749999981, 15.58864905735836182, -42.43493913623279212 ) ) ;
#18441=ADVANCED_FACE ( 'NONE', ( #34552 ), #5413, .T. ) ;
#18442=CARTESIAN_POINT ( 'NONE',  ( -3.310556943750001313, 17.50000000000001066, -31.85160580289945997 ) ) ;
#18443=CARTESIAN_POINT ( 'NONE',  ( -1.655278471875002211, 14.63297358603754716, -91.68493913623279923 ) ) ;
#18444=CARTESIAN_POINT ( 'NONE',  ( -3.500000000000000888, 19.52072594216370405, -25.73806413671075788 ) ) ;
#18445=ORIENTED_EDGE ( 'NONE', *, *, #2482, .F. ) ;
#18447=( BOUNDED_CURVE ( )  B_SPLINE_CURVE ( 2, ( #26189, #22982, #19786, #32753, #23839, #13405, #861, #10218, #10648 ),
 .UNSPECIFIED., .F., .T. ) 
 B_SPLINE_CURVE_WITH_KNOTS ( ( 3, 2, 2, 2, 3 ),
 ( 0.6562500000000000000, 0.6569444444444444420, 0.6583333333333333259, 0.6597222222222222099, 0.6604166666666666519 ),
 .UNSPECIFIED. ) 
 CURVE ( )  GEOMETRIC_REPRESENTATION_ITEM ( )  RATIONAL_B_SPLINE_CURVE ( ( 0.9330127018922194093, 0.9330127018922194093, 1.000000000000000000, 0.8660254037844387076, 1.000000000000000000, 0.8660254037844387076, 1.000000000000000000, 0.9330127018922194093, 0.9330127018922194093 ) ) 
 REPRESENTATION_ITEM ( '' )  );
#18448=CARTESIAN_POINT ( 'NONE',  ( 3.310556943750001313, 19.41135094264167549, -138.2682724695661420 ) ) ;
#18450=CARTESIAN_POINT ( 'NONE',  ( -1.750000000000002220, 14.46891108675448123, -73.48806413671076143 ) ) ;
#18451=CARTESIAN_POINT ( 'NONE',  ( -1.655278471874999990, 20.36702641396248836, -59.93077246956614346 ) ) ;
#18452=CARTESIAN_POINT ( 'NONE',  ( -3.500000000000002220, 15.47927405783632793, -82.57139747004410424 ) ) ;
#18453=EDGE_CURVE ( 'NONE', #21422, #10439, #16303, .T. ) ;
#18454=CARTESIAN_POINT ( 'NONE',  ( 3.310556943749999981, 15.58864905735836537, -62.43493913623279923 ) ) ;
#18456=CARTESIAN_POINT ( 'NONE',  ( -1.749999999999999778, 20.53108891324556140, -137.1276474690881741 ) ) ;
#18457=CARTESIAN_POINT ( 'NONE',  ( 4.648177544792955347E-16, 21.00000000000001776, -91.21098080242150274 ) ) ;
#18460=CARTESIAN_POINT ( 'NONE',  ( -1.655278471874999990, 20.36702641396249547, -121.9307724695661364 ) ) ;
#18461=CARTESIAN_POINT ( 'NONE',  ( 3.500000000000000000, 15.47927405783632082, -34.54431413575484555 ) ) ;
#18463=EDGE_LOOP ( 'NONE', ( #31657, #12556, #41124, #6700 ) ) ;
#18464=CARTESIAN_POINT ( 'NONE',  ( 1.750000000000001110, 20.53108891324555785, -110.9880641367107614 ) ) ;
#18469=CARTESIAN_POINT ( 'NONE',  ( -3.310556943750000425, 19.41135094264166483, -72.84743913623280775 ) ) ;
#18471=CARTESIAN_POINT ( 'NONE',  ( -0.9378221735089291577, 21.00000000000001776, -79.16632260368298546 ) ) ;
#18473=CARTESIAN_POINT ( 'NONE',  ( -1.394453263437886604E-15, 14.00000000000001421, -69.71098080242150274 ) ) ;
#18477=CARTESIAN_POINT ( 'NONE',  ( 3.310556943750001313, 19.41135094264166483, -80.18077246956613635 ) ) ;
#18479=VERTEX_POINT ( 'NONE', #2641 ) ;
#18485=EDGE_CURVE ( 'NONE', #37569, #7219, #25201, .T. ) ;
#18486=CARTESIAN_POINT ( 'NONE',  ( 2.340729813953370519E-16, 21.32270188528330834, -47.10160580289945642 ) ) ;
#18487=CARTESIAN_POINT ( 'NONE',  ( 3.310556943750001313, 17.50000000000002132, -108.3516058028994564 ) ) ;
#18488=ORIENTED_EDGE ( 'NONE', *, *, #11838, .T. ) ;
#18489=CARTESIAN_POINT ( 'NONE',  ( 1.655278471874998436, 14.63297358603753828, -32.43077246956614346 ) ) ;
#18490=CARTESIAN_POINT ( 'NONE',  ( -1.655278471875002211, 14.63297358603754361, -62.68493913623279923 ) ) ;
#18491=CARTESIAN_POINT ( 'NONE',  ( -3.500000000000001332, 17.50000000000002132, -109.9609808024215027 ) ) ;
#18493=CARTESIAN_POINT ( 'NONE',  ( 3.310556943750001313, 17.50000000000001776, -89.26410580289947916 ) ) ;
#18494=CARTESIAN_POINT ( 'NONE',  ( 3.500000000000000000, 15.47927405783632793, -96.23806413671076143 ) ) ;
#18496=CARTESIAN_POINT ( 'NONE',  ( -3.500000000000002220, 15.47927405783633326, -108.5713974700441042 ) ) ;
#18497=CARTESIAN_POINT ( 'NONE',  ( 1.749999999999998224, 14.46891108675448123, -85.32139747004409003 ) ) ;
#18499=CARTESIAN_POINT ( 'NONE',  ( 2.474675557024783212E-16, 21.54145188432739388, -64.21098080242150274 ) ) ;
#18500=CARTESIAN_POINT ( 'NONE',  ( -3.500000000000001332, 17.50000000000001421, -71.96098080242151696 ) ) ;
#18501=CARTESIAN_POINT ( 'NONE',  ( -3.310556943750000425, 19.41135094264165772, -28.84743913623280420 ) ) ;
#18502=CARTESIAN_POINT ( 'NONE',  ( -1.750000000000002220, 14.46891108675447946, -54.48806413671076854 ) ) ;
#18504=VECTOR ( 'NONE', #3900, 1000.000000000000000 ) ;
#18505=CARTESIAN_POINT ( 'NONE',  ( -3.310556943750001313, 17.50000000000002132, -108.8516058028994564 ) ) ;
#18506=CARTESIAN_POINT ( 'NONE',  ( 3.310556943750001313, 19.41135094264166128, -37.26827246956612072 ) ) ;
#18512=CARTESIAN_POINT ( 'NONE',  ( 0.9378221735089281585, 14.00000000000001066, -48.66632260368299967 ) ) ;
#18514=CARTESIAN_POINT ( 'NONE',  ( -7.022189441860112050E-16, 13.67729811471672363, -87.51410580289947916 ) ) ;
#18518=EDGE_LOOP ( 'NONE', ( #7546, #6062, #36103, #9585 ) ) ;
#18520=CARTESIAN_POINT ( 'NONE',  ( 4.648177544792955347E-16, 21.00000000000002487, -132.9047308033774186 ) ) ;
#18521=ORIENTED_EDGE ( 'NONE', *, *, #35545, .T. ) ;
#18524=CARTESIAN_POINT ( 'NONE',  ( -3.310556943750000425, 19.41135094264166483, -95.84743913623282197 ) ) ;
#18526=( BOUNDED_CURVE ( )  B_SPLINE_CURVE ( 2, ( #26992, #8253, #31015, #10819, #33794, #1254, #27614, #36991, #18039 ),
 .UNSPECIFIED., .F., .F. ) 
 B_SPLINE_CURVE_WITH_KNOTS ( ( 3, 2, 2, 2, 3 ),
 ( 0.2604166666666666852, 0.2611111111111111271, 0.2625000000000000111, 0.2638888888888888951, 0.2645833333333333370 ),
 .UNSPECIFIED. ) 
 CURVE ( )  GEOMETRIC_REPRESENTATION_ITEM ( )  RATIONAL_B_SPLINE_CURVE ( ( 0.9330127018922194093, 0.9330127018922194093, 1.000000000000000000, 0.8660254037844387076, 1.000000000000000000, 0.8660254037844387076, 1.000000000000000000, 0.9330127018922194093, 0.9330127018922194093 ) ) 
 REPRESENTATION_ITEM ( '' )  );
#18527=ORIENTED_EDGE ( 'NONE', *, *, #22724, .T. ) ;
#18528=CARTESIAN_POINT ( 'NONE',  ( 0.000000000000000000, 21.00000000000002487, -149.5231586289125687 ) ) ;
#18529=ORIENTED_EDGE ( 'NONE', *, *, #9811, .T. ) ;
#18531=LINE ( 'NONE', #37472, #14983 ) ;
#18537=CARTESIAN_POINT ( 'NONE',  ( 3.310556943749999981, 15.58864905735837425, -136.3474391362328220 ) ) ;
#18538=CARTESIAN_POINT ( 'NONE',  ( 0.9378221735089300459, 21.00000000000001776, -78.25563900116003424 ) ) ;
#18540=CARTESIAN_POINT ( 'NONE',  ( 3.500000000000001332, 19.52072594216370760, -54.37764746908818836 ) ) ;
#18541=CARTESIAN_POINT ( 'NONE',  ( -3.310556943750002645, 15.58864905735837780, -122.7682724695661278 ) ) ;
#18542=CARTESIAN_POINT ( 'NONE',  ( -3.310556943750002645, 15.58864905735836714, -50.76827246956612072 ) ) ;
#18543=ORIENTED_EDGE ( 'NONE', *, *, #36536, .T. ) ;
#18545=VECTOR ( 'NONE', #2790, 1000.000000000000000 ) ;
#18547=CARTESIAN_POINT ( 'NONE',  ( -3.500000000000002220, 15.47927405783633503, -133.5713974700441042 ) ) ;
#18549=CARTESIAN_POINT ( 'NONE',  ( -7.022189441860112050E-16, 13.67729811471672186, -74.60160580289947063 ) ) ;
#18550=CARTESIAN_POINT ( 'NONE',  ( -7.424026671074350129E-16, 13.45854811567264164, -129.7109808024214885 ) ) ;
#18551=CARTESIAN_POINT ( 'NONE',  ( -7.022189441860112050E-16, 13.67729811471672718, -109.5141058028994792 ) ) ;
#18554=CARTESIAN_POINT ( 'NONE',  ( 3.500000000000000000, 15.47927405783632437, -80.54431413575484555 ) ) ;
#18556=CARTESIAN_POINT ( 'NONE',  ( -1.655278471875002211, 14.63297358603754184, -40.59743913623280065 ) ) ;
#18557=CARTESIAN_POINT ( 'NONE',  ( 3.310556943749999981, 15.58864905735837070, -101.4349391362328134 ) ) ;
#18558=CARTESIAN_POINT ( 'NONE',  ( 4.648177544792955347E-16, 21.00000000000001421, -58.21098080242150985 ) ) ;
#18560=ORIENTED_EDGE ( 'NONE', *, *, #31363, .T. ) ;
#18561=CARTESIAN_POINT ( 'NONE',  ( 3.310556943750001313, 17.50000000000002132, -125.3516058028994706 ) ) ;
#18565=CARTESIAN_POINT ( 'NONE',  ( 0.000000000000000000, 17.50000000000002487, -149.5231586289125687 ) ) ;
#18566=CARTESIAN_POINT ( 'NONE',  ( -1.750000000000002220, 14.46891108675447946, -57.48806413671076143 ) ) ;
#18567=CARTESIAN_POINT ( 'NONE',  ( 0.000000000000000000, 17.50000000000002487, -149.5231586289125687 ) ) ;
#18570=ORIENTED_EDGE ( 'NONE', *, *, #40047, .F. ) ;
#18571=CARTESIAN_POINT ( 'NONE',  ( 3.310556943749999981, 15.58864905735836714, -76.43493913623278502 ) ) ;
#18576=CARTESIAN_POINT ( 'NONE',  ( -1.750000000000002220, 14.46891108675449011, -139.4880641367107614 ) ) ;
#18578=AXIS2_PLACEMENT_3D ( 'NONE', #38592, #41370, #9457 ) ;
#18580=CARTESIAN_POINT ( 'NONE',  ( -3.310556943750002201, 15.58864905735836537, -32.68077246956614346 ) ) ;
#18582=CYLINDRICAL_SURFACE ( 'NONE', #40677, 3.499999999999999556 ) ;
#18583=( BOUNDED_CURVE ( )  B_SPLINE_CURVE ( 2, ( #24326, #17727, #30486, #34096, #28128, #30697, #8149, #21125, #27516 ),
 .UNSPECIFIED., .F., .T. ) 
 B_SPLINE_CURVE_WITH_KNOTS ( ( 3, 2, 2, 2, 3 ),
 ( 0.3604166666666666630, 0.3611111111111111049, 0.3624999999999999889, 0.3638888888888888729, 0.3645833333333333148 ),
 .UNSPECIFIED. ) 
 CURVE ( )  GEOMETRIC_REPRESENTATION_ITEM ( )  RATIONAL_B_SPLINE_CURVE ( ( 0.9330127018922194093, 0.9330127018922194093, 1.000000000000000000, 0.8660254037844387076, 1.000000000000000000, 0.8660254037844387076, 1.000000000000000000, 0.9330127018922194093, 0.9330127018922194093 ) ) 
 REPRESENTATION_ITEM ( '' )  );
#18587=CARTESIAN_POINT ( 'NONE',  ( 3.310556943749999981, 15.58864905735836182, -47.34743913623280775 ) ) ;
#18588=VERTEX_POINT ( 'NONE', #22207 ) ;
#18593=DIRECTION ( 'NONE',  ( -0.000000000000000000, 1.259100132267607459E-16, -1.000000000000000000 ) ) ;
#18594=ADVANCED_FACE ( 'NONE', ( #41360 ), #16058, .T. ) ;
#18595=CARTESIAN_POINT ( 'NONE',  ( 1.749999999999998224, 14.46891108675448123, -89.62764746908817415 ) ) ;
#18596=CARTESIAN_POINT ( 'NONE',  ( 2.474675557024783212E-16, 21.54145188432739033, -40.21098080242150985 ) ) ;
#18597=CARTESIAN_POINT ( 'NONE',  ( -1.394453263437886604E-15, 14.00000000000001776, -86.71098080242151696 ) ) ;
#18598=ORIENTED_EDGE ( 'NONE', *, *, #40202, .T. ) ;
#18600=EDGE_CURVE ( 'NONE', #12520, #28199, #10250, .T. ) ;
#18602=CARTESIAN_POINT ( 'NONE',  ( 0.000000000000000000, 21.00000000000002487, -149.5231586289125687 ) ) ;
#18604=CARTESIAN_POINT ( 'NONE',  ( -1.655278471875002211, 14.63297358603753828, -23.68493913623280633 ) ) ;
#18606=CARTESIAN_POINT ( 'NONE',  ( -7.022189441860112050E-16, 13.67729811471672718, -126.5141058028994507 ) ) ;
#18610=CARTESIAN_POINT ( 'NONE',  ( -7.022189441860112050E-16, 13.67729811471672718, -115.6016058028994706 ) ) ;
#18612=CARTESIAN_POINT ( 'NONE',  ( 1.750000000000001110, 20.53108891324554719, -37.98806413671076854 ) ) ;
#18614=AXIS2_PLACEMENT_3D ( 'NONE', #10724, #18671, #12277 ) ;
#18616=CARTESIAN_POINT ( 'NONE',  ( -1.655278471875002211, 14.63297358603755427, -141.6849391362327708 ) ) ;
#18618=CARTESIAN_POINT ( 'NONE',  ( 3.310556943750001313, 19.41135094264166483, -49.26827246956613493 ) ) ;
#18620=CARTESIAN_POINT ( 'NONE',  ( -3.500000000000001332, 17.50000000000001066, -41.65473080337743284 ) ) ;
#18621=CARTESIAN_POINT ( 'NONE',  ( 1.655278471875001101, 20.36702641396248836, -72.18493913623279923 ) ) ;
#18623=CARTESIAN_POINT ( 'NONE',  ( -7.022189441860112050E-16, 13.67729811471672541, -98.51410580289945074 ) ) ;
#18624=CARTESIAN_POINT ( 'NONE',  ( 1.655278471875001101, 20.36702641396248836, -71.09743913623280775 ) ) ;
#18625=VERTEX_POINT ( 'NONE', #28998 ) ;
#18626=CARTESIAN_POINT ( 'NONE',  ( 3.310556943750001313, 17.50000000000001776, -91.35160580289947063 ) ) ;
#18628=CARTESIAN_POINT ( 'NONE',  ( 0.9378221735089281585, 14.00000000000001599, -67.66632260368298546 ) ) ;
#18631=CARTESIAN_POINT ( 'NONE',  ( 1.655278471875001101, 20.36702641396248836, -50.09743913623280775 ) ) ;
#18632=DIRECTION ( 'NONE',  ( 0.000000000000000000, 1.000000000000000000, 0.000000000000000000 ) ) ;
#18633=CARTESIAN_POINT ( 'NONE',  ( 1.655278471874998436, 14.63297358603754894, -112.4307724695661506 ) ) ;
#18634=CARTESIAN_POINT ( 'NONE',  ( -3.500000000000001332, 17.50000000000001066, -35.96098080242150985 ) ) ;
#18638=EDGE_CURVE ( 'NONE', #3232, #16494, #25828, .T. ) ;
#18640=ORIENTED_EDGE ( 'NONE', *, *, #22978, .T. ) ;
#18642=CARTESIAN_POINT ( 'NONE',  ( -3.310556943750000425, 19.41135094264166128, -61.84743913623280065 ) ) ;
#18643=VERTEX_POINT ( 'NONE', #9023 ) ;
#18645=CARTESIAN_POINT ( 'NONE',  ( 3.500000000000001332, 19.52072594216370405, -30.37764746908817770 ) ) ;
#18646=CARTESIAN_POINT ( 'NONE',  ( -1.750000000000002220, 14.46891108675449011, -142.4880641367107614 ) ) ;
#18651=EDGE_CURVE ( 'NONE', #41241, #21662, #14612, .T. ) ;
#18653=CARTESIAN_POINT ( 'NONE',  ( -3.310556943750000425, 19.41135094264167549, -132.8474391362328220 ) ) ;
#18655=EDGE_CURVE ( 'NONE', #5083, #38620, #3249, .T. ) ;
#18656=CARTESIAN_POINT ( 'NONE',  ( 3.310556943750001313, 17.50000000000001066, -38.35160580289946353 ) ) ;
#18657=CARTESIAN_POINT ( 'NONE',  ( 2.340729813953370519E-16, 21.32270188528331190, -93.10160580289947063 ) ) ;
#18658=CARTESIAN_POINT ( 'NONE',  ( 3.500000000000000000, 15.47927405783632082, -26.23806413671076143 ) ) ;
#18659=VERTEX_POINT ( 'NONE', #16315 ) ;
#18661=CARTESIAN_POINT ( 'NONE',  ( 3.310556943750001313, 17.50000000000002487, -137.3516058028994564 ) ) ;
#18663=CARTESIAN_POINT ( 'NONE',  ( -0.9378221735089310451, 14.00000000000002132, -83.75563900116002003 ) ) ;
#18664=CARTESIAN_POINT ( 'NONE',  ( 4.648177544792955347E-16, 21.00000000000001776, -86.90473080337741862 ) ) ;
#18665=CARTESIAN_POINT ( 'NONE',  ( 3.500000000000000000, 15.47927405783632970, -95.23806413671076143 ) ) ;
#18666=CARTESIAN_POINT ( 'NONE',  ( 3.500000000000001776, 19.52072594216371115, -80.07139747004410424 ) ) ;
#18668=CARTESIAN_POINT ( 'NONE',  ( 1.655278471875001101, 20.36702641396248836, -66.18493913623279923 ) ) ;
#18671=DIRECTION ( 'NONE',  ( -0.000000000000000000, 1.259100132267607459E-16, -1.000000000000000000 ) ) ;
#18672=DIRECTION ( 'NONE',  ( 0.000000000000000000, 1.000000000000000000, 0.000000000000000000 ) ) ;
#18673=EDGE_LOOP ( 'NONE', ( #462, #41834, #41141, #34571 ) ) ;
#18674=CARTESIAN_POINT ( 'NONE',  ( -1.655278471875002211, 14.63297358603755072, -113.5974391362328078 ) ) ;
#18675=CARTESIAN_POINT ( 'NONE',  ( 1.749999999999998224, 14.46891108675447413, -34.62764746908818125 ) ) ;
#18676=CARTESIAN_POINT ( 'NONE',  ( 3.500000000000000000, 15.47927405783632437, -62.23806413671076143 ) ) ;
#18678=ORIENTED_EDGE ( 'NONE', *, *, #5079, .T. ) ;
#18679=CARTESIAN_POINT ( 'NONE',  ( -3.500000000000002220, 15.47927405783632970, -106.5713974700440900 ) ) ;
#18681=VECTOR ( 'NONE', #11585, 1000.000000000000000 ) ;
#18682=CARTESIAN_POINT ( 'NONE',  ( -3.500000000000002220, 15.47927405783632082, -26.87764746908817770 ) ) ;
#18684=CARTESIAN_POINT ( 'NONE',  ( 2.340729813953370519E-16, 21.32270188528331190, -71.01410580289947916 ) ) ;
#18686=DIRECTION ( 'NONE',  ( -0.000000000000000000, 1.259100132267607459E-16, -1.000000000000000000 ) ) ;
#18687=EDGE_CURVE ( 'NONE', #4773, #12815, #20310, .T. ) ;
#18688=FACE_OUTER_BOUND ( 'NONE', #35328, .T. ) ;
#18691=CARTESIAN_POINT ( 'NONE',  ( 1.655278471874998436, 14.63297358603753651, -23.43077246956613990 ) ) ;
#18693=CARTESIAN_POINT ( 'NONE',  ( 3.310556943750001313, 17.50000000000001776, -77.26410580289946495 ) ) ;
#18696=CARTESIAN_POINT ( 'NONE',  ( -1.394453263437886604E-15, 14.00000000000002132, -127.7109808024214885 ) ) ;
#18698=EDGE_CURVE ( 'NONE', #38542, #6557, #19273, .T. ) ;
#18700=LINE ( 'NONE', #37219, #29397 ) ;
#18702=( BOUNDED_CURVE ( )  B_SPLINE_CURVE ( 2, ( #8100, #18294, #37655, #37862, #24903, #4907, #8307, #17888, #14282 ),
 .UNSPECIFIED., .F., .F. ) 
 B_SPLINE_CURVE_WITH_KNOTS ( ( 3, 2, 2, 2, 3 ),
 ( 0.06458333333333333981, 0.06527777777777778179, 0.06666666666666666574, 0.06805555555555554970, 0.06875000000000000555 ),
 .UNSPECIFIED. ) 
 CURVE ( )  GEOMETRIC_REPRESENTATION_ITEM ( )  RATIONAL_B_SPLINE_CURVE ( ( 0.9330127018922194093, 0.9330127018922200755, 1.000000000000000000, 0.8660254037844387076, 1.000000000000000000, 0.8660254037844387076, 1.000000000000000000, 0.9330127018922187432, 0.9330127018922194093 ) ) 
 REPRESENTATION_ITEM ( '' )  );
#18703=AXIS2_PLACEMENT_3D ( 'NONE', #8566, #4749, #31527 ) ;
#18704=CARTESIAN_POINT ( 'NONE',  ( -3.310556943750000425, 19.41135094264165772, -44.93493913623280633 ) ) ;
#18705=CARTESIAN_POINT ( 'NONE',  ( -1.655278471875002211, 14.63297358603755072, -111.6849391362327992 ) ) ;
#18706=ORIENTED_EDGE ( 'NONE', *, *, #23364, .F. ) ;
#18707=CARTESIAN_POINT ( 'NONE',  ( 3.310556943749999981, 15.58864905735836182, -34.34743913623281486 ) ) ;
#18708=CARTESIAN_POINT ( 'NONE',  ( 1.655278471875001101, 20.36702641396248836, -60.18493913623279923 ) ) ;
#18709=CARTESIAN_POINT ( 'NONE',  ( -1.750000000000002220, 14.46891108675448478, -108.7943141357548456 ) ) ;
#18711=CARTESIAN_POINT ( 'NONE',  ( 1.655278471875001101, 20.36702641396249192, -91.09743913623280775 ) ) ;
#18712=CARTESIAN_POINT ( 'NONE',  ( 2.474675557024783212E-16, 21.54145188432739744, -95.90473080337743284 ) ) ;
#18714=CARTESIAN_POINT ( 'NONE',  ( 3.500000000000000000, 15.47927405783632793, -85.23806413671076143 ) ) ;
#18716=CARTESIAN_POINT ( 'NONE',  ( -1.750000000000002220, 14.46891108675447946, -60.79431413575483845 ) ) ;
#18717=DIRECTION ( 'NONE',  ( -0.000000000000000000, 1.259100132267607459E-16, -1.000000000000000000 ) ) ;
#18718=CARTESIAN_POINT ( 'NONE',  ( 1.655278471875001101, 20.36702641396248481, -26.09743913623280420 ) ) ;
#18719=CARTESIAN_POINT ( 'NONE',  ( 3.500000000000001332, 17.50000000000001421, -51.15473080337743284 ) ) ;
#18721=CARTESIAN_POINT ( 'NONE',  ( 3.310556943749999981, 15.58864905735837070, -107.4349391362327992 ) ) ;
#18723=CARTESIAN_POINT ( 'NONE',  ( 2.340729813953370519E-16, 21.32270188528330834, -30.10160580289947418 ) ) ;
#18729=CARTESIAN_POINT ( 'NONE',  ( 3.310556943749999981, 15.58864905735836892, -90.34743913623280775 ) ) ;
#18730=CARTESIAN_POINT ( 'NONE',  ( -1.749999999999999778, 20.53108891324554719, -24.12764746908817415 ) ) ;
#18733=CARTESIAN_POINT ( 'NONE',  ( 1.750000000000001110, 20.53108891324555074, -74.29431413575483134 ) ) ;
#18737=CARTESIAN_POINT ( 'NONE',  ( 3.310556943750001313, 19.41135094264166483, -97.18077246956613635 ) ) ;
#18739=VERTEX_POINT ( 'NONE', #10130 ) ;
#18746=VECTOR ( 'NONE', #33696, 1000.000000000000000 ) ;
#18749=ORIENTED_EDGE ( 'NONE', *, *, #41054, .F. ) ;
#18750=CARTESIAN_POINT ( 'NONE',  ( 1.750000000000001110, 20.53108891324556140, -134.9880641367107614 ) ) ;
#18752=CARTESIAN_POINT ( 'NONE',  ( -3.310556943750002645, 15.58864905735837780, -135.6807724695661364 ) ) ;
#18753=FACE_OUTER_BOUND ( 'NONE', #16410, .T. ) ;
#18756=CARTESIAN_POINT ( 'NONE',  ( -3.310556943750000425, 19.41135094264166838, -122.9349391362327992 ) ) ;
#18757=CARTESIAN_POINT ( 'NONE',  ( 1.655278471874998436, 14.63297358603754006, -51.51827246956612782 ) ) ;
#18759=CARTESIAN_POINT ( 'NONE',  ( -3.500000000000000888, 19.52072594216372181, -133.7380641367107614 ) ) ;
#18761=CARTESIAN_POINT ( 'NONE',  ( -1.655278471875002211, 14.63297358603754539, -78.68493913623279923 ) ) ;
#18762=CARTESIAN_POINT ( 'NONE',  ( -1.750000000000002220, 14.46891108675448834, -124.7943141357548456 ) ) ;
#18763=CARTESIAN_POINT ( 'NONE',  ( 3.310556943750001313, 19.41135094264166838, -109.1807724695661506 ) ) ;
#18764=EDGE_CURVE ( 'NONE', #34168, #24436, #7605, .T. ) ;
#18768=CARTESIAN_POINT ( 'NONE',  ( -1.750000000000002220, 14.46891108675448301, -81.79431413575484555 ) ) ;
#18769=CARTESIAN_POINT ( 'NONE',  ( 2.340729813953370519E-16, 21.32270188528330479, -41.01410580289947916 ) ) ;
#18770=CARTESIAN_POINT ( 'NONE',  ( -1.655278471875002211, 14.63297358603754894, -101.6849391362327992 ) ) ;
#18771=CARTESIAN_POINT ( 'NONE',  ( 4.648177544792955347E-16, 21.00000000000001421, -73.21098080242151696 ) ) ;
#18773=ORIENTED_EDGE ( 'NONE', *, *, #26378, .F. ) ;
#18774=CARTESIAN_POINT ( 'NONE',  ( 1.655278471874998436, 14.63297358603755072, -125.5182724695661278 ) ) ;
#18775=CARTESIAN_POINT ( 'NONE',  ( 4.648177544792955347E-16, 21.00000000000001776, -92.21098080242150274 ) ) ;
#18778=CARTESIAN_POINT ( 'NONE',  ( 4.648177544792955347E-16, 21.00000000000002132, -121.9047308033774044 ) ) ;
#18779=CARTESIAN_POINT ( 'NONE',  ( 3.500000000000001332, 19.52072594216370760, -60.37764746908817415 ) ) ;
#18780=( BOUNDED_CURVE ( )  B_SPLINE_CURVE ( 2, ( #30872, #31486, #27675, #28500, #34062, #18107, #4918, #29553, #3198 ),
 .UNSPECIFIED., .F., .T. ) 
 B_SPLINE_CURVE_WITH_KNOTS ( ( 3, 2, 2, 2, 3 ),
 ( 0.6520833333333333481, 0.6527777777777777901, 0.6541666666666666741, 0.6555555555555555580, 0.6562500000000000000 ),
 .UNSPECIFIED. ) 
 CURVE ( )  GEOMETRIC_REPRESENTATION_ITEM ( )  RATIONAL_B_SPLINE_CURVE ( ( 0.9330127018922194093, 0.9330127018922194093, 1.000000000000000000, 0.8660254037844387076, 1.000000000000000000, 0.8660254037844387076, 1.000000000000000000, 0.9330127018922194093, 0.9330127018922194093 ) ) 
 REPRESENTATION_ITEM ( '' )  );
#18781=CARTESIAN_POINT ( 'NONE',  ( -0.9378221735089310451, 14.00000000000001599, -62.75563900116003424 ) ) ;
#18784=CARTESIAN_POINT ( 'NONE',  ( -3.310556943750000425, 19.41135094264166483, -73.93493913623278502 ) ) ;
#18790=CARTESIAN_POINT ( 'NONE',  ( -3.310556943750001313, 17.50000000000001066, -35.76410580289947205 ) ) ;
#18793=VERTEX_POINT ( 'NONE', #30108 ) ;
#18795=CARTESIAN_POINT ( 'NONE',  ( 1.655278471874998436, 14.63297358603754006, -49.43077246956615056 ) ) ;
#18799=CARTESIAN_POINT ( 'NONE',  ( 0.000000000000000000, 17.50000000000002487, -149.5231586289125687 ) ) ;
#18801=CARTESIAN_POINT ( 'NONE',  ( -0.9378221735089291577, 21.00000000000002132, -104.8600726046389155 ) ) ;
#18803=CARTESIAN_POINT ( 'NONE',  ( 1.749999999999998224, 14.46891108675447413, -31.62764746908818125 ) ) ;
#18804=CARTESIAN_POINT ( 'NONE',  ( 3.500000000000001332, 19.52072594216370405, -35.37764746908818125 ) ) ;
#18805=CARTESIAN_POINT ( 'NONE',  ( 3.500000000000000000, 15.47927405783632793, -82.54431413575483134 ) ) ;
#18808=CARTESIAN_POINT ( 'NONE',  ( 3.500000000000001776, 19.52072594216372181, -137.3776474690881741 ) ) ;
#18809=CARTESIAN_POINT ( 'NONE',  ( -0.9378221735089310451, 14.00000000000001066, -52.75563900116002714 ) ) ;
#18810=CARTESIAN_POINT ( 'NONE',  ( 3.310556943750001313, 19.41135094264166838, -123.1807724695661364 ) ) ;
#18813=FACE_OUTER_BOUND ( 'NONE', #7639, .T. ) ;
#18814=CARTESIAN_POINT ( 'NONE',  ( -3.500000000000001332, 17.50000000000001776, -94.96098080242150274 ) ) ;
#18815=CARTESIAN_POINT ( 'NONE',  ( -1.655278471875002211, 14.63297358603755072, -117.6849391362327850 ) ) ;
#18816=CARTESIAN_POINT ( 'NONE',  ( -1.749999999999999778, 20.53108891324555074, -55.82139747004409713 ) ) ;
#18817=CARTESIAN_POINT ( 'NONE',  ( -1.749999999999999778, 20.53108891324554719, -39.82139747004409713 ) ) ;
#18818=DIRECTION ( 'NONE',  ( -0.000000000000000000, 1.259100132267607459E-16, -1.000000000000000000 ) ) ;
#18820=CARTESIAN_POINT ( 'NONE',  ( -1.655278471874999990, 20.36702641396249902, -138.0182724695661420 ) ) ;
#18823=CARTESIAN_POINT ( 'NONE',  ( -1.655278471874999990, 20.36702641396248481, -46.01827246956613493 ) ) ;
#18825=CARTESIAN_POINT ( 'NONE',  ( 3.500000000000000000, 15.47927405783632970, -104.5443141357548456 ) ) ;
#18826=CARTESIAN_POINT ( 'NONE',  ( -1.655278471875002211, 14.63297358603754539, -70.68493913623278502 ) ) ;
#18828=CARTESIAN_POINT ( 'NONE',  ( -3.310556943750000425, 19.41135094264166128, -71.84743913623280775 ) ) ;
#18829=VERTEX_POINT ( 'NONE', #37338 ) ;
#18830=( BOUNDED_CURVE ( )  B_SPLINE_CURVE ( 2, ( #39529, #10406, #36344, #14546, #1773, #14755, #21126, #40275, #27309 ),
 .UNSPECIFIED., .F., .T. ) 
 B_SPLINE_CURVE_WITH_KNOTS ( ( 3, 2, 2, 2, 3 ),
 ( 0.4520833333333333370, 0.4527777777777777790, 0.4541666666666666630, 0.4555555555555555469, 0.4562499999999999889 ),
 .UNSPECIFIED. ) 
 CURVE ( )  GEOMETRIC_REPRESENTATION_ITEM ( )  RATIONAL_B_SPLINE_CURVE ( ( 0.9330127018922194093, 0.9330127018922194093, 1.000000000000000000, 0.8660254037844387076, 1.000000000000000000, 0.8660254037844387076, 1.000000000000000000, 0.9330127018922194093, 0.9330127018922194093 ) ) 
 REPRESENTATION_ITEM ( '' )  );
#18831=CARTESIAN_POINT ( 'NONE',  ( 1.655278471875001101, 20.36702641396249192, -92.18493913623279923 ) ) ;
#18834=FACE_OUTER_BOUND ( 'NONE', #38259, .T. ) ;
#18835=CARTESIAN_POINT ( 'NONE',  ( 4.648177544792955347E-16, 21.00000000000001421, -53.21098080242150985 ) ) ;
#18836=CARTESIAN_POINT ( 'NONE',  ( -1.655278471875002211, 14.63297358603754184, -51.59743913623281486 ) ) ;
#18839=CARTESIAN_POINT ( 'NONE',  ( 2.340729813953370519E-16, 21.32270188528331900, -109.0141058028994792 ) ) ;
#18840=EDGE_CURVE ( 'NONE', #32296, #19108, #8953, .T. ) ;
#18844=ORIENTED_EDGE ( 'NONE', *, *, #6630, .T. ) ;
#18846=CARTESIAN_POINT ( 'NONE',  ( 2.340729813953370519E-16, 21.32270188528330834, -64.01410580289947916 ) ) ;
#18847=ORIENTED_EDGE ( 'NONE', *, *, #22872, .T. ) ;
#18850=CARTESIAN_POINT ( 'NONE',  ( 0.000000000000000000, 17.50000000000002487, -149.5231586289125687 ) ) ;
#18853=VERTEX_POINT ( 'NONE', #27560 ) ;
#18855=CARTESIAN_POINT ( 'NONE',  ( 3.310556943750001313, 17.50000000000002132, -124.2641058028994649 ) ) ;
#18858=EDGE_CURVE ( 'NONE', #31803, #20880, #13309, .T. ) ;
#18859=CARTESIAN_POINT ( 'NONE',  ( 1.655278471874998436, 14.63297358603754006, -42.51827246956613493 ) ) ;
#18860=CARTESIAN_POINT ( 'NONE',  ( 1.655278471875001101, 20.36702641396248481, -29.18493913623279568 ) ) ;
#18861=CARTESIAN_POINT ( 'NONE',  ( 3.310556943750001313, 17.50000000000001776, -86.35160580289947063 ) ) ;
#18862=CARTESIAN_POINT ( 'NONE',  ( 2.340729813953370519E-16, 21.32270188528332255, -138.0141058028994507 ) ) ;
#18865=CARTESIAN_POINT ( 'NONE',  ( 3.310556943749999981, 15.58864905735837425, -134.4349391362327992 ) ) ;
#18868=CARTESIAN_POINT ( 'NONE',  ( 4.648177544792955347E-16, 21.00000000000002487, -139.2109808024214885 ) ) ;
#18870=CARTESIAN_POINT ( 'NONE',  ( -3.500000000000000888, 19.52072594216371115, -80.73806413671077564 ) ) ;
#18872=CARTESIAN_POINT ( 'NONE',  ( -1.655278471874999990, 20.36702641396248836, -66.01827246956612782 ) ) ;
#18875=FACE_OUTER_BOUND ( 'NONE', #21404, .T. ) ;
#18876=CARTESIAN_POINT ( 'NONE',  ( -3.310556943750001313, 17.50000000000001776, -83.85160580289947063 ) ) ;
#18877=CARTESIAN_POINT ( 'NONE',  ( -3.500000000000000000, 19.52072594216370760, -48.04431413575484555 ) ) ;
#18878=CARTESIAN_POINT ( 'NONE',  ( -3.310556943750000425, 19.41135094264166838, -116.8474391362327935 ) ) ;
#18880=CARTESIAN_POINT ( 'NONE',  ( -7.460324959392693302E-14, 21.00000000000001776, -86.21098080242150274 ) ) ;
#18882=CARTESIAN_POINT ( 'NONE',  ( 3.500000000000000000, 15.47927405783632970, -109.2380641367107472 ) ) ;
#18883=CARTESIAN_POINT ( 'NONE',  ( -3.500000000000002220, 15.47927405783632082, -28.57139747004410069 ) ) ;
#18887=CARTESIAN_POINT ( 'NONE',  ( -7.022189441860112050E-16, 13.67729811471672186, -67.51410580289947916 ) ) ;
#18889=ADVANCED_FACE ( 'NONE', ( #34352 ), #40726, .T. ) ;
#18890=CARTESIAN_POINT ( 'NONE',  ( 0.9378221735089281585, 14.00000000000001243, -59.66632260368299256 ) ) ;
#18892=EDGE_CURVE ( 'NONE', #40976, #9702, #30955, .T. ) ;
#18894=ORIENTED_EDGE ( 'NONE', *, *, #4578, .T. ) ;
#18895=CARTESIAN_POINT ( 'NONE',  ( 3.310556943750001313, 19.41135094264166128, -25.18077246956613635 ) ) ;
#18897=CARTESIAN_POINT ( 'NONE',  ( 1.655278471875001101, 20.36702641396249192, -80.09743913623280775 ) ) ;
#18900=CARTESIAN_POINT ( 'NONE',  ( -3.500000000000001332, 17.50000000000001421, -48.65473080337742573 ) ) ;
#18903=CARTESIAN_POINT ( 'NONE',  ( 4.648177544792955347E-16, 21.00000000000001776, -95.90473080337743284 ) ) ;
#18904=CARTESIAN_POINT ( 'NONE',  ( 1.655278471874998436, 14.63297358603754006, -44.51827246956613493 ) ) ;
#18905=CARTESIAN_POINT ( 'NONE',  ( -3.310556943750000425, 19.41135094264166838, -106.9349391362327850 ) ) ;
#18906=ORIENTED_EDGE ( 'NONE', *, *, #40681, .F. ) ;
#18908=CARTESIAN_POINT ( 'NONE',  ( 1.655278471875001101, 20.36702641396248481, -30.09743913623280775 ) ) ;
#18909=CARTESIAN_POINT ( 'NONE',  ( -3.310556943750002645, 15.58864905735836892, -62.76827246956612782 ) ) ;
#18910=CARTESIAN_POINT ( 'NONE',  ( -3.500000000000001332, 17.50000000000002132, -108.9609808024215027 ) ) ;
#18911=EDGE_CURVE ( 'NONE', #22611, #18006, #34556, .T. ) ;
#18913=CARTESIAN_POINT ( 'NONE',  ( -1.750000000000002220, 14.46891108675448478, -98.48806413671076143 ) ) ;
#18917=CARTESIAN_POINT ( 'NONE',  ( 2.474675557024783212E-16, 21.54145188432739388, -57.21098080242150985 ) ) ;
#18918=LINE ( 'NONE', #35508, #1329 ) ;
#18919=CARTESIAN_POINT ( 'NONE',  ( 3.310556943749999981, 15.58864905735836182, -28.34743913623280775 ) ) ;
#18920=CARTESIAN_POINT ( 'NONE',  ( -1.750000000000002220, 14.46891108675447768, -48.48806413671076854 ) ) ;
#18922=CARTESIAN_POINT ( 'NONE',  ( -1.655278471874999990, 20.36702641396249192, -102.0182724695661278 ) ) ;
#18923=CARTESIAN_POINT ( 'NONE',  ( -7.022189441860112050E-16, 13.67729811471671653, -31.60160580289945997 ) ) ;
#18926=CARTESIAN_POINT ( 'NONE',  ( -1.394453263437886604E-15, 14.00000000000002132, -130.7109808024214885 ) ) ;
#18927=ADVANCED_FACE ( 'NONE', ( #18813 ), #31773, .T. ) ;
#18931=CARTESIAN_POINT ( 'NONE',  ( 3.310556943750001313, 17.50000000000001776, -83.26410580289947916 ) ) ;
#18935=EDGE_CURVE ( 'NONE', #1125, #1116, #2015, .T. ) ;
#18937=VERTEX_POINT ( 'NONE', #27963 ) ;
#18940=CARTESIAN_POINT ( 'NONE',  ( 2.340729813953370519E-16, 21.32270188528331190, -93.01410580289949337 ) ) ;
#18942=ORIENTED_EDGE ( 'NONE', *, *, #484, .F. ) ;
#18943=CARTESIAN_POINT ( 'NONE',  ( -1.394453263437886604E-15, 14.00000000000001066, -33.71098080242150985 ) ) ;
#18946=( BOUNDED_CURVE ( )  B_SPLINE_CURVE ( 2, ( #5404, #21570, #41351, #34750, #31351, #12202, #15194, #14780, #24984 ),
 .UNSPECIFIED., .F., .F. ) 
 B_SPLINE_CURVE_WITH_KNOTS ( ( 3, 2, 2, 2, 3 ),
 ( 0.6645833333333333037, 0.6652777777777777457, 0.6666666666666666297, 0.6680555555555555136, 0.6687499999999999556 ),
 .UNSPECIFIED. ) 
 CURVE ( )  GEOMETRIC_REPRESENTATION_ITEM ( )  RATIONAL_B_SPLINE_CURVE ( ( 0.9330127018922194093, 0.9330127018922194093, 1.000000000000000000, 0.8660254037844387076, 1.000000000000000000, 0.8660254037844387076, 1.000000000000000000, 0.9330127018922194093, 0.9330127018922194093 ) ) 
 REPRESENTATION_ITEM ( '' )  );
#18947=CARTESIAN_POINT ( 'NONE',  ( 3.369928719974892676E-15, 14.00000000000002309, -139.7109808024214885 ) ) ;
#18948=( BOUNDED_CURVE ( )  B_SPLINE_CURVE ( 2, ( #35462, #28860, #39263, #29701, #3139, #13334, #35871, #39481, #16129 ),
 .UNSPECIFIED., .F., .F. ) 
 B_SPLINE_CURVE_WITH_KNOTS ( ( 3, 2, 2, 2, 3 ),
 ( 0.5437499999999999556, 0.5444444444444443976, 0.5458333333333332815, 0.5472222222222222765, 0.5479166666666667185 ),
 .UNSPECIFIED. ) 
 CURVE ( )  GEOMETRIC_REPRESENTATION_ITEM ( )  RATIONAL_B_SPLINE_CURVE ( ( 0.9330127018922194093, 0.9330127018922194093, 1.000000000000000000, 0.8660254037844387076, 1.000000000000000000, 0.8660254037844387076, 1.000000000000000000, 0.9330127018922194093, 0.9330127018922194093 ) ) 
 REPRESENTATION_ITEM ( '' )  );
#18950=CARTESIAN_POINT ( 'NONE',  ( 1.750000000000001110, 20.53108891324555074, -66.29431413575484555 ) ) ;
#18955=CARTESIAN_POINT ( 'NONE',  ( 0.000000000000000000, 17.50000000000002487, -149.5231586289125687 ) ) ;
#18956=CARTESIAN_POINT ( 'NONE',  ( 1.655278471874998436, 14.63297358603755072, -130.4307724695661364 ) ) ;
#18957=CARTESIAN_POINT ( 'NONE',  ( -1.394453263437886604E-15, 14.00000000000001066, -41.71098080242150274 ) ) ;
#18958=VERTEX_POINT ( 'NONE', #28378 ) ;
#18960=CARTESIAN_POINT ( 'NONE',  ( -7.022189441860112050E-16, 13.67729811471672718, -124.6016058028994564 ) ) ;
#18961=CARTESIAN_POINT ( 'NONE',  ( 2.340729813953370519E-16, 21.32270188528330834, -51.10160580289946353 ) ) ;
#18963=CARTESIAN_POINT ( 'NONE',  ( 3.500000000000001332, 17.50000000000002132, -129.1547308033774186 ) ) ;
#18965=CARTESIAN_POINT ( 'NONE',  ( 3.310556943750001313, 19.41135094264166483, -76.26827246956612782 ) ) ;
#18966=CARTESIAN_POINT ( 'NONE',  ( 3.500000000000001332, 17.50000000000002132, -121.4609808024215170 ) ) ;
#18967=CARTESIAN_POINT ( 'NONE',  ( 3.310556943749999981, 15.58864905735837070, -106.3474391362328078 ) ) ;
#18968=CARTESIAN_POINT ( 'NONE',  ( -3.500000000000002220, 15.47927405783633326, -107.5713974700440900 ) ) ;
#18971=CARTESIAN_POINT ( 'NONE',  ( 3.500000000000000000, 15.47927405783632437, -76.54431413575483134 ) ) ;
#18972=VECTOR ( 'NONE', #32533, 1000.000000000000000 ) ;
#18973=CARTESIAN_POINT ( 'NONE',  ( -3.500000000000001332, 17.50000000000001421, -50.96098080242150985 ) ) ;
#18974=CARTESIAN_POINT ( 'NONE',  ( 2.340729813953370519E-16, 21.32270188528330479, -42.01410580289947916 ) ) ;
#18975=CARTESIAN_POINT ( 'NONE',  ( 3.310556943749999981, 15.58864905735837070, -100.4349391362327992 ) ) ;
#18977=CARTESIAN_POINT ( 'NONE',  ( 1.750000000000001110, 20.53108891324555074, -63.98806413671076143 ) ) ;
#18980=CARTESIAN_POINT ( 'NONE',  ( 3.310556943750001313, 19.41135094264166838, -121.2682724695661278 ) ) ;
#18982=EDGE_CURVE ( 'NONE', #25503, #36901, #8904, .T. ) ;
#18985=CARTESIAN_POINT ( 'NONE',  ( 3.500000000000001332, 17.50000000000001421, -50.46098080242150985 ) ) ;
#18986=CARTESIAN_POINT ( 'NONE',  ( 0.9378221735089281585, 14.00000000000002132, -107.6663226036829855 ) ) ;
#18990=CARTESIAN_POINT ( 'NONE',  ( -3.310556943750001313, 17.50000000000001421, -72.85160580289947063 ) ) ;
#18992=CARTESIAN_POINT ( 'NONE',  ( 4.648177544792955347E-16, 21.00000000000001066, -40.21098080242150274 ) ) ;
#18993=CARTESIAN_POINT ( 'NONE',  ( 0.9378221735089281585, 14.00000000000001599, -80.36007260463890134 ) ) ;
#18997=CARTESIAN_POINT ( 'NONE',  ( -3.310556943750000425, 19.41135094264166128, -33.84743913623280775 ) ) ;
#19002=CARTESIAN_POINT ( 'NONE',  ( -1.749999999999999778, 20.53108891324555429, -100.1276474690881741 ) ) ;
#19003=ORIENTED_EDGE ( 'NONE', *, *, #5491, .T. ) ;
#19006=CARTESIAN_POINT ( 'NONE',  ( 1.750000000000001110, 20.53108891324555429, -90.29431413575483134 ) ) ;
#19008=CARTESIAN_POINT ( 'NONE',  ( 0.000000000000000000, 17.50000000000002487, -149.5231586289125687 ) ) ;
#19009=CARTESIAN_POINT ( 'NONE',  ( 1.749999999999998224, 14.46891108675448478, -121.3213974700441042 ) ) ;
#19010=CARTESIAN_POINT ( 'NONE',  ( -3.500000000000001332, 17.50000000000001066, -33.96098080242150274 ) ) ;
#19011=CARTESIAN_POINT ( 'NONE',  ( 1.750000000000001110, 20.53108891324554719, -31.29431413575484200 ) ) ;
#19012=CARTESIAN_POINT ( 'NONE',  ( 1.750000000000001110, 20.53108891324554719, -35.29431413575484555 ) ) ;
#19013=ORIENTED_EDGE ( 'NONE', *, *, #30771, .F. ) ;
#19016=CARTESIAN_POINT ( 'NONE',  ( 1.750000000000001110, 20.53108891324554719, -36.98806413671076854 ) ) ;
#19018=CARTESIAN_POINT ( 'NONE',  ( 3.500000000000000000, 15.47927405783633503, -137.5443141357548598 ) ) ;
#19019=DIRECTION ( 'NONE',  ( -0.000000000000000000, 1.259100132267607459E-16, -1.000000000000000000 ) ) ;
#19020=CARTESIAN_POINT ( 'NONE',  ( -1.655278471875002211, 14.63297358603755249, -124.5974391362328078 ) ) ;
#19025=CARTESIAN_POINT ( 'NONE',  ( -3.500000000000001332, 17.50000000000001776, -89.96098080242151696 ) ) ;
#19026=CARTESIAN_POINT ( 'NONE',  ( -3.310556943750001313, 17.50000000000002132, -118.8516058028994706 ) ) ;
#19028=CARTESIAN_POINT ( 'NONE',  ( -3.500000000000000888, 19.52072594216370405, -34.73806413671076854 ) ) ;
#19029=CARTESIAN_POINT ( 'NONE',  ( -3.500000000000001332, 17.50000000000002132, -121.6547308033774328 ) ) ;
#19031=CARTESIAN_POINT ( 'NONE',  ( -3.310556943750001313, 17.50000000000002487, -141.8516058028994564 ) ) ;
#19032=EDGE_CURVE ( 'NONE', #15133, #25969, #23291, .T. ) ;
#19034=CARTESIAN_POINT ( 'NONE',  ( -3.310556943750000425, 19.41135094264166483, -50.93493913623280633 ) ) ;
#19036=CARTESIAN_POINT ( 'NONE',  ( -1.749999999999999778, 20.53108891324554719, -41.82139747004409713 ) ) ;
#19037=CARTESIAN_POINT ( 'NONE',  ( -1.655278471874999990, 20.36702641396248836, -71.01827246956612782 ) ) ;
#19038=AXIS2_PLACEMENT_3D ( 'NONE', #10140, #16735, #13531 ) ;
#19040=CARTESIAN_POINT ( 'NONE',  ( -3.310556943750002645, 15.58864905735837070, -67.68077246956613635 ) ) ;
#19042=CARTESIAN_POINT ( 'NONE',  ( -3.310556943750002201, 15.58864905735837247, -89.76827246956612782 ) ) ;
#19044=CARTESIAN_POINT ( 'NONE',  ( 3.500000000000001332, 19.52072594216370760, -49.37764746908818125 ) ) ;
#19046=CARTESIAN_POINT ( 'NONE',  ( -3.500000000000002220, 15.47927405783632437, -41.87764746908817415 ) ) ;
#19047=CARTESIAN_POINT ( 'NONE',  ( 1.655278471874998436, 14.63297358603754006, -48.43077246956614346 ) ) ;
#19049=CARTESIAN_POINT ( 'NONE',  ( 3.310556943750001313, 17.50000000000002132, -106.2641058028994649 ) ) ;
#19050=CARTESIAN_POINT ( 'NONE',  ( -1.394453263437886604E-15, 14.00000000000001776, -101.4047308033774186 ) ) ;
#19051=ORIENTED_EDGE ( 'NONE', *, *, #20951, .T. ) ;
#19055=CARTESIAN_POINT ( 'NONE',  ( 3.310556943750001313, 17.50000000000001421, -59.26410580289947916 ) ) ;
#19056=VERTEX_POINT ( 'NONE', #9242 ) ;
#19057=EDGE_LOOP ( 'NONE', ( #31808, #26592, #20901, #41917 ) ) ;
#19059=CARTESIAN_POINT ( 'NONE',  ( 4.648177544792955347E-16, 21.00000000000001066, -40.90473080337742573 ) ) ;
#19063=CARTESIAN_POINT ( 'NONE',  ( 4.648177544792955347E-16, 21.00000000000001421, -55.21098080242150274 ) ) ;
#19064=CARTESIAN_POINT ( 'NONE',  ( -1.655278471875002211, 14.63297358603755249, -127.5974391362328078 ) ) ;
#19068=CARTESIAN_POINT ( 'NONE',  ( -1.655278471875002211, 14.63297358603754006, -33.68493913623279923 ) ) ;
#19069=CARTESIAN_POINT ( 'NONE',  ( -3.310556943750001313, 17.50000000000001066, -26.85160580289947063 ) ) ;
#19070=CARTESIAN_POINT ( 'NONE',  ( 1.655278471875001101, 20.36702641396249192, -86.18493913623278502 ) ) ;
#19071=CARTESIAN_POINT ( 'NONE',  ( -7.022189441860112050E-16, 13.67729811471672896, -137.5141058028994507 ) ) ;
#19073=EDGE_CURVE ( 'NONE', #34720, #5090, #32311, .T. ) ;
#19075=( BOUNDED_CURVE ( )  B_SPLINE_CURVE ( 2, ( #36119, #7210, #6991, #19967, #16782, #22943, #22737, #35713, #6575 ),
 .UNSPECIFIED., .F., .T. ) 
 B_SPLINE_CURVE_WITH_KNOTS ( ( 3, 2, 2, 2, 3 ),
 ( 0.2020833333333333370, 0.2027777777777777790, 0.2041666666666666630, 0.2055555555555555469, 0.2062499999999999889 ),
 .UNSPECIFIED. ) 
 CURVE ( )  GEOMETRIC_REPRESENTATION_ITEM ( )  RATIONAL_B_SPLINE_CURVE ( ( 0.9330127018922194093, 0.9330127018922194093, 1.000000000000000000, 0.8660254037844387076, 1.000000000000000000, 0.8660254037844387076, 1.000000000000000000, 0.9330127018922194093, 0.9330127018922194093 ) ) 
 REPRESENTATION_ITEM ( '' )  );
#19077=CARTESIAN_POINT ( 'NONE',  ( 3.310556943750001313, 17.50000000000002487, -131.3516058028994564 ) ) ;
#19078=CARTESIAN_POINT ( 'NONE',  ( 0.000000000000000000, 21.00000000000002487, -149.5231586289125687 ) ) ;
#19082=CARTESIAN_POINT ( 'NONE',  ( 1.750000000000001110, 20.53108891324555429, -77.98806413671076143 ) ) ;
#19083=CARTESIAN_POINT ( 'NONE',  ( 3.310556943749999981, 15.58864905735836537, -64.43493913623279923 ) ) ;
#19086=CARTESIAN_POINT ( 'NONE',  ( 3.500000000000001332, 17.50000000000001421, -47.46098080242150274 ) ) ;
#19087=CARTESIAN_POINT ( 'NONE',  ( 1.655278471874998436, 14.63297358603754539, -87.51827246956612782 ) ) ;
#19088=CARTESIAN_POINT ( 'NONE',  ( 3.602337597214540226E-14, 14.00000000000002132, -116.4047308033774328 ) ) ;
#19089=CARTESIAN_POINT ( 'NONE',  ( -1.655278471874999990, 20.36702641396249547, -111.9307724695661506 ) ) ;
#19090=CARTESIAN_POINT ( 'NONE',  ( 4.286263797015737581E-16, 14.00000000000002487, -149.5231586289125687 ) ) ;
#19091=CARTESIAN_POINT ( 'NONE',  ( 0.9378221735089281585, 14.00000000000001243, -62.36007260463890134 ) ) ;
#19092=ORIENTED_EDGE ( 'NONE', *, *, #17358, .F. ) ;
#19093=CARTESIAN_POINT ( 'NONE',  ( 1.749999999999998224, 14.46891108675448301, -108.3213974700441042 ) ) ;
#19094=CARTESIAN_POINT ( 'NONE',  ( 4.648177544792955347E-16, 21.00000000000001066, -28.90473080337742928 ) ) ;
#19096=CARTESIAN_POINT ( 'NONE',  ( -3.500000000000002220, 15.47927405783632970, -82.57139747004410424 ) ) ;
#19097=CARTESIAN_POINT ( 'NONE',  ( 0.000000000000000000, 21.00000000000002487, -149.5231586289125687 ) ) ;
#19100=CARTESIAN_POINT ( 'NONE',  ( -3.310556943750001313, 17.50000000000001421, -67.76410580289947916 ) ) ;
#19103=CARTESIAN_POINT ( 'NONE',  ( -7.022189441860112050E-16, 13.67729811471672718, -119.5141058028994934 ) ) ;
#19104=VECTOR ( 'NONE', #5135, 1000.000000000000000 ) ;
#19108=VERTEX_POINT ( 'NONE', #35807 ) ;
#19110=CARTESIAN_POINT ( 'NONE',  ( -1.394453263437886604E-15, 14.00000000000001776, -104.7109808024215027 ) ) ;
#19111=CARTESIAN_POINT ( 'NONE',  ( -1.655278471874999990, 20.36702641396249192, -78.93077246956615056 ) ) ;
#19115=CARTESIAN_POINT ( 'NONE',  ( -3.500000000000002220, 15.47927405783632437, -53.57139747004409713 ) ) ;
#19120=CARTESIAN_POINT ( 'NONE',  ( -3.310556943750000425, 19.41135094264165772, -42.93493913623279923 ) ) ;
#19121=CARTESIAN_POINT ( 'NONE',  ( 3.310556943750001313, 17.50000000000002132, -104.3516058028994564 ) ) ;
#19125=CARTESIAN_POINT ( 'NONE',  ( -1.655278471874999990, 20.36702641396248481, -29.93077246956614346 ) ) ;
#19126=CARTESIAN_POINT ( 'NONE',  ( 4.648177544792955347E-16, 21.00000000000001421, -68.90473080337741862 ) ) ;
#19127=CARTESIAN_POINT ( 'NONE',  ( 3.500000000000001332, 17.50000000000002132, -105.4609808024215027 ) ) ;
#19130=CARTESIAN_POINT ( 'NONE',  ( 1.750000000000001110, 20.53108891324555429, -98.98806413671076143 ) ) ;
#19131=CARTESIAN_POINT ( 'NONE',  ( 3.500000000000001332, 17.50000000000001421, -63.46098080242150274 ) ) ;
#19134=CARTESIAN_POINT ( 'NONE',  ( -7.424026671074350129E-16, 13.45854811567263454, -59.71098080242151696 ) ) ;
#19135=CARTESIAN_POINT ( 'NONE',  ( -0.9378221735089310451, 14.00000000000001066, -46.75563900116002714 ) ) ;
#19136=CARTESIAN_POINT ( 'NONE',  ( 1.655278471874998436, 14.63297358603753828, -28.43077246956614346 ) ) ;
#19137=CARTESIAN_POINT ( 'NONE',  ( -7.424026671074350129E-16, 13.45854811567263276, -48.40473080337742573 ) ) ;
#19138=DIRECTION ( 'NONE',  ( -0.000000000000000000, 1.259100132267607459E-16, -1.000000000000000000 ) ) ;
#19139=CARTESIAN_POINT ( 'NONE',  ( 3.310556943750001313, 19.41135094264166128, -32.26827246956613493 ) ) ;
#19142=CARTESIAN_POINT ( 'NONE',  ( 1.045839947578414805E-15, 14.00000000000002665, -141.7109808024215170 ) ) ;
#19146=CARTESIAN_POINT ( 'NONE',  ( -7.022189441860112050E-16, 13.67729811471672363, -84.51410580289947916 ) ) ;
#19147=FACE_OUTER_BOUND ( 'NONE', #7172, .T. ) ;
#19148=ORIENTED_EDGE ( 'NONE', *, *, #39217, .F. ) ;
#19149=VERTEX_POINT ( 'NONE', #41791 ) ;
#19152=CARTESIAN_POINT ( 'NONE',  ( 1.655278471874998436, 14.63297358603754539, -94.43077246956613635 ) ) ;
#19155=ORIENTED_EDGE ( 'NONE', *, *, #13119, .T. ) ;
#19157=VERTEX_POINT ( 'NONE', #77 ) ;
#19159=CARTESIAN_POINT ( 'NONE',  ( 3.500000000000000000, 15.47927405783632437, -66.54431413575484555 ) ) ;
#19166=CARTESIAN_POINT ( 'NONE',  ( 3.310556943750001313, 19.41135094264167549, -132.1807724695661364 ) ) ;
#19170=CARTESIAN_POINT ( 'NONE',  ( 3.310556943750001313, 19.41135094264166838, -122.2682724695661278 ) ) ;
#19171=CARTESIAN_POINT ( 'NONE',  ( 2.340729813953370519E-16, 21.32270188528330834, -53.10160580289946353 ) ) ;
#19172=VERTEX_POINT ( 'NONE', #3686 ) ;
#19173=CARTESIAN_POINT ( 'NONE',  ( -3.500000000000001332, 17.50000000000002132, -128.6547308033774186 ) ) ;
#19174=ADVANCED_FACE ( 'NONE', ( #26451 ), #39002, .T. ) ;
#19176=CARTESIAN_POINT ( 'NONE',  ( 1.655278471874998436, 14.63297358603754361, -77.51827246956614204 ) ) ;
#19177=CARTESIAN_POINT ( 'NONE',  ( 3.500000000000000000, 15.47927405783633503, -124.5443141357548456 ) ) ;
#19178=CARTESIAN_POINT ( 'NONE',  ( 2.340729813953370519E-16, 21.32270188528331900, -110.0141058028994649 ) ) ;
#19179=FACE_OUTER_BOUND ( 'NONE', #17544, .T. ) ;
#19182=CARTESIAN_POINT ( 'NONE',  ( 2.474675557024783212E-16, 21.54145188432739744, -75.21098080242153117 ) ) ;
#19184=CARTESIAN_POINT ( 'NONE',  ( 1.655278471875001101, 20.36702641396248481, -41.09743913623280065 ) ) ;
#19185=CARTESIAN_POINT ( 'NONE',  ( -1.655278471875002211, 14.63297358603754894, -103.6849391362328134 ) ) ;
#19186=CARTESIAN_POINT ( 'NONE',  ( 3.500000000000001332, 17.50000000000001421, -73.46098080242151696 ) ) ;
#19187=CARTESIAN_POINT ( 'NONE',  ( 3.500000000000001332, 17.50000000000001421, -67.15473080337743284 ) ) ;
#19189=ORIENTED_EDGE ( 'NONE', *, *, #17820, .F. ) ;
#19190=CARTESIAN_POINT ( 'NONE',  ( 3.310556943750001313, 17.50000000000002132, -118.3516058028994706 ) ) ;
#19191=CARTESIAN_POINT ( 'NONE',  ( 4.648177544792955347E-16, 21.00000000000001066, -28.21098080242150985 ) ) ;
#19194=CARTESIAN_POINT ( 'NONE',  ( 3.500000000000001332, 19.52072594216370405, -32.07139747004410424 ) ) ;
#19199=( BOUNDED_CURVE ( )  B_SPLINE_CURVE ( 2, ( #24876, #17859, #1695, #40406, #21665, #24250, #34437, #34643, #34227 ),
 .UNSPECIFIED., .F., .T. ) 
 B_SPLINE_CURVE_WITH_KNOTS ( ( 3, 2, 2, 2, 3 ),
 ( 0.3395833333333333481, 0.3402777777777777901, 0.3416666666666666741, 0.3430555555555555580, 0.3437500000000000000 ),
 .UNSPECIFIED. ) 
 CURVE ( )  GEOMETRIC_REPRESENTATION_ITEM ( )  RATIONAL_B_SPLINE_CURVE ( ( 0.9330127018922194093, 0.9330127018922194093, 1.000000000000000000, 0.8660254037844387076, 1.000000000000000000, 0.8660254037844387076, 1.000000000000000000, 0.9330127018922194093, 0.9330127018922194093 ) ) 
 REPRESENTATION_ITEM ( '' )  );
#19200=CARTESIAN_POINT ( 'NONE',  ( 4.648177544792955347E-16, 21.00000000000001421, -56.90473080337742573 ) ) ;
#19201=CARTESIAN_POINT ( 'NONE',  ( 1.750000000000001110, 20.53108891324555074, -47.98806413671076143 ) ) ;
#19206=CARTESIAN_POINT ( 'NONE',  ( 3.310556943749999981, 15.58864905735836182, -34.34743913623280775 ) ) ;
#19207=CARTESIAN_POINT ( 'NONE',  ( 0.9378221735089281585, 14.00000000000002132, -107.3600726046389155 ) ) ;
#19208=AXIS2_PLACEMENT_3D ( 'NONE', #658, #878, #17676 ) ;
#19210=EDGE_LOOP ( 'NONE', ( #7247, #29670, #17966, #17911 ) ) ;
#19211=EDGE_CURVE ( 'NONE', #26058, #4034, #19233, .T. ) ;
#19214=CARTESIAN_POINT ( 'NONE',  ( -0.9378221735089291577, 21.00000000000002487, -138.8600726046389298 ) ) ;
#19217=DIRECTION ( 'NONE',  ( -0.000000000000000000, 1.259100132267607459E-16, -1.000000000000000000 ) ) ;
#19218=CARTESIAN_POINT ( 'NONE',  ( -1.394453263437886604E-15, 14.00000000000001776, -87.71098080242151696 ) ) ;
#19220=CARTESIAN_POINT ( 'NONE',  ( 2.474675557024783212E-16, 21.54145188432740099, -116.9047308033774470 ) ) ;
#19223=CARTESIAN_POINT ( 'NONE',  ( -3.500000000000001332, 17.50000000000001066, -33.96098080242150274 ) ) ;
#19224=CARTESIAN_POINT ( 'NONE',  ( 4.648177544792955347E-16, 21.00000000000001066, -35.21098080242151696 ) ) ;
#19226=CARTESIAN_POINT ( 'NONE',  ( 4.648177544792955347E-16, 21.00000000000002132, -105.9047308033774186 ) ) ;
#19228=CARTESIAN_POINT ( 'NONE',  ( -3.500000000000000888, 19.52072594216372181, -140.0443141357548313 ) ) ;
#19230=CARTESIAN_POINT ( 'NONE',  ( -3.310556943750002645, 15.58864905735837780, -122.6807724695661506 ) ) ;
#19233=LINE ( 'NONE', #13057, #28607 ) ;
#19234=CARTESIAN_POINT ( 'NONE',  ( 1.749999999999998224, 14.46891108675448123, -90.62764746908817415 ) ) ;
#19235=CARTESIAN_POINT ( 'NONE',  ( -1.749999999999999778, 20.53108891324554719, -45.82139747004410424 ) ) ;
#19236=CARTESIAN_POINT ( 'NONE',  ( 1.655278471874998436, 14.63297358603754184, -58.43077246956614346 ) ) ;
#19237=CARTESIAN_POINT ( 'NONE',  ( -7.022189441860112050E-16, 13.67729811471672718, -119.6016058028994706 ) ) ;
#19238=CYLINDRICAL_SURFACE ( 'NONE', #39741, 3.499999999999999556 ) ;
#19239=CARTESIAN_POINT ( 'NONE',  ( -3.500000000000000888, 19.52072594216370405, -32.73806413671076854 ) ) ;
#19242=CARTESIAN_POINT ( 'NONE',  ( -1.655278471875002211, 14.63297358603755249, -134.6849391362327992 ) ) ;
#19243=VECTOR ( 'NONE', #19914, 1000.000000000000000 ) ;
#19245=CARTESIAN_POINT ( 'NONE',  ( -1.750000000000002220, 14.46891108675447946, -66.48806413671076143 ) ) ;
#19246=CARTESIAN_POINT ( 'NONE',  ( -3.310556943750001313, 17.50000000000001066, -44.85160580289947063 ) ) ;
#19247=CARTESIAN_POINT ( 'NONE',  ( -1.394453263437886604E-15, 14.00000000000001066, -36.71098080242150985 ) ) ;
#19248=CARTESIAN_POINT ( 'NONE',  ( 3.310556943750001313, 17.50000000000001421, -67.35160580289947063 ) ) ;
#19250=CARTESIAN_POINT ( 'NONE',  ( -1.655278471875002211, 14.63297358603754361, -62.59743913623280775 ) ) ;
#19252=CARTESIAN_POINT ( 'NONE',  ( 3.310556943750001313, 17.50000000000001776, -89.35160580289947063 ) ) ;
#19254=DIRECTION ( 'NONE',  ( -0.000000000000000000, 1.259100132267607459E-16, -1.000000000000000000 ) ) ;
#19255=CARTESIAN_POINT ( 'NONE',  ( -1.750000000000002220, 14.46891108675447590, -39.79431413575484555 ) ) ;
#19256=CARTESIAN_POINT ( 'NONE',  ( -1.750000000000002220, 14.46891108675447768, -41.79431413575483845 ) ) ;
#19257=CARTESIAN_POINT ( 'NONE',  ( 3.310556943749999981, 15.58864905735836182, -52.34743913623281486 ) ) ;
#19259=CARTESIAN_POINT ( 'NONE',  ( 1.655278471874998436, 14.63297358603754716, -106.4307724695661364 ) ) ;
#19264=CARTESIAN_POINT ( 'NONE',  ( 3.310556943750001313, 17.50000000000001421, -57.26410580289947916 ) ) ;
#19270=CARTESIAN_POINT ( 'NONE',  ( 0.000000000000000000, 17.50000000000002487, -149.5231586289125687 ) ) ;
#19272=ORIENTED_EDGE ( 'NONE', *, *, #33482, .F. ) ;
#19273=( BOUNDED_CURVE ( )  B_SPLINE_CURVE ( 2, ( #10340, #12905, #3738, #3327, #29255, #19492, #39249, #32663, #129 ),
 .UNSPECIFIED., .F., .F. ) 
 B_SPLINE_CURVE_WITH_KNOTS ( ( 3, 2, 2, 2, 3 ),
 ( 0.6354166666666666297, 0.6361111111111110716, 0.6374999999999999556, 0.6388888888888888395, 0.6395833333333332815 ),
 .UNSPECIFIED. ) 
 CURVE ( )  GEOMETRIC_REPRESENTATION_ITEM ( )  RATIONAL_B_SPLINE_CURVE ( ( 0.9330127018922194093, 0.9330127018922194093, 1.000000000000000000, 0.8660254037844387076, 1.000000000000000000, 0.8660254037844387076, 1.000000000000000000, 0.9330127018922194093, 0.9330127018922194093 ) ) 
 REPRESENTATION_ITEM ( '' )  );
#19274=CARTESIAN_POINT ( 'NONE',  ( -3.500000000000001332, 17.50000000000001066, -38.96098080242150985 ) ) ;
#19275=CARTESIAN_POINT ( 'NONE',  ( -3.310556943750002201, 15.58864905735837780, -122.6807724695661364 ) ) ;
#19276=CARTESIAN_POINT ( 'NONE',  ( -1.749999999999999778, 20.53108891324555785, -117.8213974700440900 ) ) ;
#19279=CARTESIAN_POINT ( 'NONE',  ( 1.655278471874998436, 14.63297358603753828, -35.51827246956612782 ) ) ;
#19280=CARTESIAN_POINT ( 'NONE',  ( -3.310556943750000425, 19.41135094264165772, -28.93493913623279568 ) ) ;
#19281=CARTESIAN_POINT ( 'NONE',  ( -3.310556943750002645, 15.58864905735837247, -87.76827246956614204 ) ) ;
#19282=CARTESIAN_POINT ( 'NONE',  ( -3.310556943750002645, 15.58864905735837958, -138.6807724695661364 ) ) ;
#19285=CARTESIAN_POINT ( 'NONE',  ( 4.648177544792955347E-16, 21.00000000000001066, -34.90473080337743284 ) ) ;
#19286=CARTESIAN_POINT ( 'NONE',  ( 1.655278471874998436, 14.63297358603755072, -134.5182724695661420 ) ) ;
#19287=CARTESIAN_POINT ( 'NONE',  ( 0.000000000000000000, 17.50000000000002487, -149.5231586289125687 ) ) ;
#19288=DIRECTION ( 'NONE',  ( 0.000000000000000000, 1.000000000000000000, 0.000000000000000000 ) ) ;
#19289=CARTESIAN_POINT ( 'NONE',  ( -0.9378221735089310451, 14.00000000000002309, -125.7556390011600485 ) ) ;
#19291=CARTESIAN_POINT ( 'NONE',  ( 1.749999999999998224, 14.46891108675447946, -78.32139747004410424 ) ) ;
#19292=CARTESIAN_POINT ( 'NONE',  ( -1.655278471875002211, 14.63297358603754361, -63.68493913623279923 ) ) ;
#19295=LINE ( 'NONE', #562, #14580 ) ;
#19296=CARTESIAN_POINT ( 'NONE',  ( -3.310556943750000425, 19.41135094264166483, -87.93493913623279923 ) ) ;
#19298=CARTESIAN_POINT ( 'NONE',  ( 3.310556943750001313, 17.50000000000002132, -115.2641058028994792 ) ) ;
#19299=CARTESIAN_POINT ( 'NONE',  ( 1.655278471874998436, 14.63297358603754361, -80.43077246956615056 ) ) ;
#19300=CARTESIAN_POINT ( 'NONE',  ( -0.9378221735089310451, 14.00000000000002132, -96.44938900211596433 ) ) ;
#19302=CARTESIAN_POINT ( 'NONE',  ( 1.750000000000001110, 20.53108891324555785, -106.9880641367107614 ) ) ;
#19305=CARTESIAN_POINT ( 'NONE',  ( 3.500000000000001332, 19.52072594216370760, -48.37764746908817415 ) ) ;
#19306=LINE ( 'NONE', #22708, #31238 ) ;
#19309=CARTESIAN_POINT ( 'NONE',  ( -1.655278471875002211, 14.63297358603754361, -64.59743913623280775 ) ) ;
#19311=CARTESIAN_POINT ( 'NONE',  ( 1.655278471874998436, 14.63297358603754894, -119.4307724695661364 ) ) ;
#19313=CARTESIAN_POINT ( 'NONE',  ( 4.648177544792955347E-16, 21.00000000000002132, -125.9047308033774186 ) ) ;
#19314=VERTEX_POINT ( 'NONE', #3475 ) ;
#19317=CARTESIAN_POINT ( 'NONE',  ( 3.310556943750001313, 17.50000000000001776, -75.26410580289947916 ) ) ;
#19318=ORIENTED_EDGE ( 'NONE', *, *, #34112, .F. ) ;
#19319=ORIENTED_EDGE ( 'NONE', *, *, #17415, .T. ) ;
#19322=CARTESIAN_POINT ( 'NONE',  ( 2.340729813953370519E-16, 21.32270188528332255, -140.0141058028994792 ) ) ;
#19325=CARTESIAN_POINT ( 'NONE',  ( 0.000000000000000000, 21.00000000000002487, -149.5231586289125687 ) ) ;
#19326=CARTESIAN_POINT ( 'NONE',  ( -3.310556943750001313, 17.50000000000001066, -42.85160580289947063 ) ) ;
#19327=CARTESIAN_POINT ( 'NONE',  ( 3.310556943750001313, 19.41135094264166838, -103.2682724695661278 ) ) ;
#19328=EDGE_CURVE ( 'NONE', #3869, #18011, #39298, .T. ) ;
#19329=EDGE_CURVE ( 'NONE', #4567, #31508, #9884, .T. ) ;
#19330=CARTESIAN_POINT ( 'NONE',  ( -3.310556943750002645, 15.58864905735836537, -31.68077246956614701 ) ) ;
#19333=CARTESIAN_POINT ( 'NONE',  ( 3.500000000000001776, 19.52072594216371826, -106.3776474690881741 ) ) ;
#19336=CARTESIAN_POINT ( 'NONE',  ( 3.500000000000001776, 19.52072594216371115, -95.07139747004409003 ) ) ;
#19337=CARTESIAN_POINT ( 'NONE',  ( -3.500000000000001332, 17.50000000000002132, -108.6547308033774186 ) ) ;
#19340=CARTESIAN_POINT ( 'NONE',  ( -3.500000000000002220, 15.47927405783632437, -59.87764746908818125 ) ) ;
#19342=CARTESIAN_POINT ( 'NONE',  ( 1.655278471875001101, 20.36702641396248481, -25.09743913623281486 ) ) ;
#19343=CARTESIAN_POINT ( 'NONE',  ( -1.749999999999999778, 20.53108891324555074, -50.82139747004409003 ) ) ;
#19344=CARTESIAN_POINT ( 'NONE',  ( 3.500000000000001332, 17.50000000000002132, -106.4609808024215027 ) ) ;
#19345=CARTESIAN_POINT ( 'NONE',  ( -3.310556943750002201, 15.58864905735836537, -30.76827246956613848 ) ) ;
#19348=CARTESIAN_POINT ( 'NONE',  ( -1.749999999999999778, 20.53108891324555785, -121.1276474690881741 ) ) ;
#19352=CARTESIAN_POINT ( 'NONE',  ( -3.310556943750000425, 19.41135094264166838, -79.84743913623279354 ) ) ;
#19353=FACE_OUTER_BOUND ( 'NONE', #18463, .T. ) ;
#19355=CARTESIAN_POINT ( 'NONE',  ( 3.500000000000001332, 17.50000000000001066, -34.15473080337742573 ) ) ;
#19360=CARTESIAN_POINT ( 'NONE',  ( -1.655278471875002211, 14.63297358603754716, -88.59743913623280775 ) ) ;
#19361=ADVANCED_FACE ( 'NONE', ( #16674 ), #35180, .T. ) ;
#19363=DIRECTION ( 'NONE',  ( -0.000000000000000000, 1.259100132267607459E-16, -1.000000000000000000 ) ) ;
#19364=ORIENTED_EDGE ( 'NONE', *, *, #36218, .T. ) ;
#19365=AXIS2_PLACEMENT_3D ( 'NONE', #38892, #9771, #35705 ) ;
#19367=VECTOR ( 'NONE', #24743, 1000.000000000000000 ) ;
#19373=CYLINDRICAL_SURFACE ( 'NONE', #38435, 3.499999999999999556 ) ;
#19374=CARTESIAN_POINT ( 'NONE',  ( 1.655278471874998436, 14.63297358603755072, -132.4307724695661364 ) ) ;
#19376=DIRECTION ( 'NONE',  ( -0.000000000000000000, 1.259100132267607459E-16, -1.000000000000000000 ) ) ;
#19377=CARTESIAN_POINT ( 'NONE',  ( 1.655278471874998436, 14.63297358603754894, -119.5182724695661278 ) ) ;
#19378=CARTESIAN_POINT ( 'NONE',  ( -3.310556943750000425, 19.41135094264166128, -48.93493913623281344 ) ) ;
#19380=CARTESIAN_POINT ( 'NONE',  ( -7.424026671074350129E-16, 13.45854811567264164, -132.4047308033774186 ) ) ;
#19381=EDGE_CURVE ( 'NONE', #13712, #30038, #27638, .T. ) ;
#19382=CARTESIAN_POINT ( 'NONE',  ( 3.310556943749999981, 15.58864905735836714, -74.43493913623279923 ) ) ;
#19383=CARTESIAN_POINT ( 'NONE',  ( -7.424026671074350129E-16, 13.45854811567264164, -125.7109808024215170 ) ) ;
#19384=CARTESIAN_POINT ( 'NONE',  ( 2.340729813953370519E-16, 21.32270188528331900, -106.0141058028994792 ) ) ;
#19385=( BOUNDED_CURVE ( )  B_SPLINE_CURVE ( 2, ( #26511, #29901, #988, #10758, #1195, #33299, #23959, #23320, #39469 ),
 .UNSPECIFIED., .F., .T. ) 
 B_SPLINE_CURVE_WITH_KNOTS ( ( 3, 2, 2, 2, 3 ),
 ( 0.6187500000000000222, 0.6194444444444444642, 0.6208333333333333481, 0.6222222222222222321, 0.6229166666666666741 ),
 .UNSPECIFIED. ) 
 CURVE ( )  GEOMETRIC_REPRESENTATION_ITEM ( )  RATIONAL_B_SPLINE_CURVE ( ( 0.9330127018922194093, 0.9330127018922194093, 1.000000000000000000, 0.8660254037844387076, 1.000000000000000000, 0.8660254037844387076, 1.000000000000000000, 0.9330127018922194093, 0.9330127018922194093 ) ) 
 REPRESENTATION_ITEM ( '' )  );
#19386=CARTESIAN_POINT ( 'NONE',  ( 0.000000000000000000, 17.50000000000002487, -149.5231586289125687 ) ) ;
#19389=CARTESIAN_POINT ( 'NONE',  ( -1.750000000000002220, 14.46891108675448123, -76.79431413575484555 ) ) ;
#19390=CARTESIAN_POINT ( 'NONE',  ( 1.749999999999998224, 14.46891108675448656, -126.3213974700440900 ) ) ;
#19391=CARTESIAN_POINT ( 'NONE',  ( -3.310556943750001313, 17.50000000000001066, -42.76410580289947916 ) ) ;
#19392=CARTESIAN_POINT ( 'NONE',  ( 1.655278471874998436, 14.63297358603754716, -100.5182724695661278 ) ) ;
#19394=CARTESIAN_POINT ( 'NONE',  ( -3.500000000000001332, 17.50000000000001421, -62.65473080337742573 ) ) ;
#19397=CARTESIAN_POINT ( 'NONE',  ( 2.340729813953370519E-16, 21.32270188528331900, -119.1016058028994564 ) ) ;
#19403=CARTESIAN_POINT ( 'NONE',  ( 1.655278471875001101, 20.36702641396249192, -99.09743913623280775 ) ) ;
#19404=CARTESIAN_POINT ( 'NONE',  ( -3.500000000000000000, 19.52072594216370760, -52.73806413671076854 ) ) ;
#19406=EDGE_LOOP ( 'NONE', ( #23192, #27886, #21249, #19272 ) ) ;
#19407=CARTESIAN_POINT ( 'NONE',  ( 0.9378221735089300459, 21.00000000000002487, -136.2556390011600911 ) ) ;
#19409=CARTESIAN_POINT ( 'NONE',  ( -3.500000000000002220, 15.47927405783633503, -112.5713974700440900 ) ) ;
#19412=VECTOR ( 'NONE', #33704, 1000.000000000000000 ) ;
#19414=CARTESIAN_POINT ( 'NONE',  ( -1.655278471875002211, 14.63297358603754006, -35.59743913623280775 ) ) ;
#19415=EDGE_CURVE ( 'NONE', #6800, #167, #23691, .T. ) ;
#19417=ADVANCED_FACE ( 'NONE', ( #4107 ), #14537, .T. ) ;
#19419=VERTEX_POINT ( 'NONE', #7943 ) ;
#19421=CARTESIAN_POINT ( 'NONE',  ( 4.648177544792955347E-16, 21.00000000000001776, -100.2109808024215027 ) ) ;
#19423=CARTESIAN_POINT ( 'NONE',  ( 0.9378221735089300459, 21.00000000000001776, -90.25563900116003424 ) ) ;
#19426=CARTESIAN_POINT ( 'NONE',  ( 3.500000000000001776, 19.52072594216371826, -118.0713974700440900 ) ) ;
#19428=CARTESIAN_POINT ( 'NONE',  ( 2.340729813953370519E-16, 21.32270188528332255, -137.1016058028994564 ) ) ;
#19429=CARTESIAN_POINT ( 'NONE',  ( -3.500000000000002220, 15.47927405783632082, -33.87764746908818125 ) ) ;
#19432=CARTESIAN_POINT ( 'NONE',  ( 0.9378221735089300459, 21.00000000000001066, -41.25563900116003424 ) ) ;
#19434=CARTESIAN_POINT ( 'NONE',  ( -7.424026671074350129E-16, 13.45854811567264164, -137.7109808024214885 ) ) ;
#19435=CARTESIAN_POINT ( 'NONE',  ( 3.310556943750001313, 17.50000000000001066, -38.26410580289947916 ) ) ;
#19436=CARTESIAN_POINT ( 'NONE',  ( -7.022189441860112050E-16, 13.67729811471672718, -122.5141058028994934 ) ) ;
#19440=CARTESIAN_POINT ( 'NONE',  ( 1.750000000000001110, 20.53108891324555429, -89.29431413575483134 ) ) ;
#19444=CARTESIAN_POINT ( 'NONE',  ( -3.310556943750002645, 15.58864905735836892, -58.68077246956613635 ) ) ;
#19445=CARTESIAN_POINT ( 'NONE',  ( -7.022189441860112050E-16, 13.67729811471672718, -117.6016058028994564 ) ) ;
#19446=CARTESIAN_POINT ( 'NONE',  ( 4.648177544792955347E-16, 21.00000000000002132, -122.2109808024215170 ) ) ;
#19447=CARTESIAN_POINT ( 'NONE',  ( -1.749999999999999778, 20.53108891324554719, -30.82139747004410069 ) ) ;
#19448=CARTESIAN_POINT ( 'NONE',  ( 0.000000000000000000, 17.50000000000002487, -149.5231586289125687 ) ) ;
#19451=CARTESIAN_POINT ( 'NONE',  ( -3.310556943750001313, 17.50000000000002487, -132.8516058028994564 ) ) ;
#19453=CARTESIAN_POINT ( 'NONE',  ( -0.9378221735089291577, 21.00000000000001066, -29.86007260463891555 ) ) ;
#19455=CARTESIAN_POINT ( 'NONE',  ( 1.655278471874998436, 14.63297358603754361, -68.51827246956612782 ) ) ;
#19457=CARTESIAN_POINT ( 'NONE',  ( -3.310556943750002645, 15.58864905735836892, -63.68077246956615056 ) ) ;
#19458=VERTEX_POINT ( 'NONE', #232 ) ;
#19459=CARTESIAN_POINT ( 'NONE',  ( -3.310556943750000425, 19.41135094264166838, -86.93493913623278502 ) ) ;
#19460=AXIS2_PLACEMENT_3D ( 'NONE', #20999, #33973, #17401 ) ;
#19464=CARTESIAN_POINT ( 'NONE',  ( 0.000000000000000000, 21.00000000000002487, -149.5231586289125687 ) ) ;
#19465=CARTESIAN_POINT ( 'NONE',  ( 3.310556943750001313, 17.50000000000001421, -49.26410580289947205 ) ) ;
#19467=CARTESIAN_POINT ( 'NONE',  ( 3.310556943749999981, 15.58864905735837070, -103.3474391362328220 ) ) ;
#19469=ORIENTED_EDGE ( 'NONE', *, *, #10829, .F. ) ;
#19472=VERTEX_POINT ( 'NONE', #26200 ) ;
#19474=CARTESIAN_POINT ( 'NONE',  ( 3.310556943749999981, 15.58864905735836537, -59.34743913623280775 ) ) ;
#19477=CARTESIAN_POINT ( 'NONE',  ( 1.749999999999998224, 14.46891108675447946, -76.62764746908817415 ) ) ;
#19478=CARTESIAN_POINT ( 'NONE',  ( -3.500000000000002220, 15.47927405783632437, -40.57139747004410424 ) ) ;
#19480=CARTESIAN_POINT ( 'NONE',  ( 3.500000000000001332, 19.52072594216371826, -114.3776474690881599 ) ) ;
#19481=EDGE_LOOP ( 'NONE', ( #39016, #24245, #28546, #31690 ) ) ;
#19483=CARTESIAN_POINT ( 'NONE',  ( 1.655278471874998436, 14.63297358603754894, -122.4307724695661364 ) ) ;
#19484=CARTESIAN_POINT ( 'NONE',  ( 3.500000000000001332, 17.50000000000001066, -23.46098080242150985 ) ) ;
#19486=CARTESIAN_POINT ( 'NONE',  ( -3.310556943750000425, 19.41135094264165772, -36.93493913623279923 ) ) ;
#19487=CARTESIAN_POINT ( 'NONE',  ( -1.655278471875002211, 14.63297358603754006, -27.68493913623279568 ) ) ;
#19488=CARTESIAN_POINT ( 'NONE',  ( 2.340729813953370519E-16, 21.32270188528331190, -87.10160580289945642 ) ) ;
#19489=CARTESIAN_POINT ( 'NONE',  ( -3.310556943750001313, 17.50000000000002487, -139.7641058028994792 ) ) ;
#19492=CARTESIAN_POINT ( 'NONE',  ( -3.500000000000002220, 15.47927405783632615, -66.87764746908817415 ) ) ;
#19493=CARTESIAN_POINT ( 'NONE',  ( -3.310556943750002645, 15.58864905735837780, -134.7682724695661420 ) ) ;
#19494=CARTESIAN_POINT ( 'NONE',  ( 0.9378221735089281585, 14.00000000000001599, -70.36007260463891555 ) ) ;
#19495=CARTESIAN_POINT ( 'NONE',  ( 3.310556943750001313, 17.50000000000001776, -91.26410580289947916 ) ) ;
#19498=CARTESIAN_POINT ( 'NONE',  ( 3.500000000000001332, 19.52072594216371826, -132.0713974700441042 ) ) ;
#19499=CARTESIAN_POINT ( 'NONE',  ( 2.474675557024783212E-16, 21.54145188432739388, -72.90473080337744705 ) ) ;
#19500=CARTESIAN_POINT ( 'NONE',  ( 2.340729813953370519E-16, 21.32270188528331190, -60.10160580289947063 ) ) ;
#19503=DIRECTION ( 'NONE',  ( -0.000000000000000000, 1.259100132267607459E-16, -1.000000000000000000 ) ) ;
#19504=CARTESIAN_POINT ( 'NONE',  ( -1.655278471875002211, 14.63297358603754716, -83.68493913623278502 ) ) ;
#19507=CARTESIAN_POINT ( 'NONE',  ( 3.310556943750001313, 19.41135094264166838, -112.1807724695661506 ) ) ;
#19508=CARTESIAN_POINT ( 'NONE',  ( 2.340729813953370519E-16, 21.32270188528331190, -83.01410580289946495 ) ) ;
#19509=CARTESIAN_POINT ( 'NONE',  ( 0.9378221735089281585, 14.00000000000001243, -57.36007260463890844 ) ) ;
#19511=CARTESIAN_POINT ( 'NONE',  ( -7.424026671074350129E-16, 13.45854811567263809, -106.4047308033774328 ) ) ;
#19513=CARTESIAN_POINT ( 'NONE',  ( 1.749999999999998224, 14.46891108675447946, -71.62764746908817415 ) ) ;
#19514=CARTESIAN_POINT ( 'NONE',  ( 0.9378221735088952959, 21.00000000000003908, -87.94938900211595012 ) ) ;
#19517=CARTESIAN_POINT ( 'NONE',  ( 4.648177544792955347E-16, 21.00000000000001421, -65.21098080242150274 ) ) ;
#19519=CARTESIAN_POINT ( 'NONE',  ( 2.340729813953370519E-16, 21.32270188528331190, -69.01410580289947916 ) ) ;
#19521=CARTESIAN_POINT ( 'NONE',  ( 2.340729813953370519E-16, 21.32270188528331900, -124.0141058028994792 ) ) ;
#19522=CARTESIAN_POINT ( 'NONE',  ( 4.648177544792955347E-16, 21.00000000000001776, -92.90473080337741862 ) ) ;
#19525=CARTESIAN_POINT ( 'NONE',  ( -1.394453263437886604E-15, 14.00000000000001066, -42.71098080242150274 ) ) ;
#19527=CARTESIAN_POINT ( 'NONE',  ( 1.655278471874998436, 14.63297358603754361, -75.43077246956613635 ) ) ;
#19528=ORIENTED_EDGE ( 'NONE', *, *, #34349, .F. ) ;
#19531=CARTESIAN_POINT ( 'NONE',  ( -3.310556943750002201, 15.58864905735837958, -139.6807724695661364 ) ) ;
#19533=CARTESIAN_POINT ( 'NONE',  ( -1.394453263437886604E-15, 14.00000000000001776, -89.40473080337741862 ) ) ;
#19534=CARTESIAN_POINT ( 'NONE',  ( -7.022189441860112050E-16, 13.67729811471671653, -42.60160580289946353 ) ) ;
#19535=CARTESIAN_POINT ( 'NONE',  ( -3.310556943750000425, 19.41135094264166838, -103.9349391362328134 ) ) ;
#19536=CARTESIAN_POINT ( 'NONE',  ( -3.310556943750000425, 19.41135094264165772, -28.84743913623280420 ) ) ;
#19538=CARTESIAN_POINT ( 'NONE',  ( -3.500000000000002220, 15.47927405783632970, -99.87764746908817415 ) ) ;
#19541=CARTESIAN_POINT ( 'NONE',  ( 2.474675557024783212E-16, 21.54145188432739744, -90.90473080337743284 ) ) ;
#19542=CARTESIAN_POINT ( 'NONE',  ( -1.749999999999999778, 20.53108891324555429, -78.12764746908817415 ) ) ;
#19545=CARTESIAN_POINT ( 'NONE',  ( 1.750000000000001110, 20.53108891324555074, -60.29431413575483845 ) ) ;
#19547=CARTESIAN_POINT ( 'NONE',  ( -1.655278471875002211, 14.63297358603753828, -23.59743913623281486 ) ) ;
#19548=CARTESIAN_POINT ( 'NONE',  ( 3.500000000000000000, 15.47927405783632082, -51.23806413671076854 ) ) ;
#19549=CARTESIAN_POINT ( 'NONE',  ( -1.750000000000002220, 14.46891108675448834, -131.7943141357548598 ) ) ;
#19550=CARTESIAN_POINT ( 'NONE',  ( 3.310556943749999981, 15.58864905735836182, -34.43493913623279923 ) ) ;
#19553=CARTESIAN_POINT ( 'NONE',  ( -0.9378221735089304900, 21.00000000000002487, -142.1663226036830281 ) ) ;
#19557=CARTESIAN_POINT ( 'NONE',  ( 3.310556943750001313, 19.41135094264166838, -84.18077246956615056 ) ) ;
#19558=CARTESIAN_POINT ( 'NONE',  ( -0.9378221735089304900, 21.00000000000002487, -141.8600726046389298 ) ) ;
#19559=ORIENTED_EDGE ( 'NONE', *, *, #37416, .F. ) ;
#19560=CARTESIAN_POINT ( 'NONE',  ( 0.9378221735089281585, 14.00000000000000888, -34.36007260463890844 ) ) ;
#19562=( BOUNDED_CURVE ( )  B_SPLINE_CURVE ( 2, ( #20429, #10019, #7244, #4476, #32969, #23189, #29779, #14053, #17457 ),
 .UNSPECIFIED., .F., .F. ) 
 B_SPLINE_CURVE_WITH_KNOTS ( ( 3, 2, 2, 2, 3 ),
 ( 0.4020833333333333481, 0.4027777777777777901, 0.4041666666666666741, 0.4055555555555555580, 0.4062500000000000000 ),
 .UNSPECIFIED. ) 
 CURVE ( )  GEOMETRIC_REPRESENTATION_ITEM ( )  RATIONAL_B_SPLINE_CURVE ( ( 0.9330127018922194093, 0.9330127018922194093, 1.000000000000000000, 0.8660254037844387076, 1.000000000000000000, 0.8660254037844387076, 1.000000000000000000, 0.9330127018922194093, 0.9330127018922194093 ) ) 
 REPRESENTATION_ITEM ( '' )  );
#19563=ORIENTED_EDGE ( 'NONE', *, *, #34176, .T. ) ;
#19565=CARTESIAN_POINT ( 'NONE',  ( -3.310556943750002645, 15.58864905735837247, -90.68077246956613635 ) ) ;
#19567=VERTEX_POINT ( 'NONE', #22577 ) ;
#19569=CARTESIAN_POINT ( 'NONE',  ( 0.9378221735089300459, 21.00000000000001421, -66.25563900116002003 ) ) ;
#19571=CARTESIAN_POINT ( 'NONE',  ( 0.000000000000000000, 17.50000000000002487, -149.5231586289125687 ) ) ;
#19573=CARTESIAN_POINT ( 'NONE',  ( -3.310556943750002645, 15.58864905735837780, -130.6807724695661364 ) ) ;
#19575=ORIENTED_EDGE ( 'NONE', *, *, #17400, .T. ) ;
#19576=CARTESIAN_POINT ( 'NONE',  ( 1.749999999999998224, 14.46891108675447946, -73.32139747004410424 ) ) ;
#19577=CARTESIAN_POINT ( 'NONE',  ( 3.310556943749999981, 15.58864905735837247, -119.4349391362327992 ) ) ;
#19579=CARTESIAN_POINT ( 'NONE',  ( -7.424026671074350129E-16, 13.45854811567264164, -128.4047308033774470 ) ) ;
#19580=CARTESIAN_POINT ( 'NONE',  ( 3.310556943750001313, 19.41135094264166128, -73.26827246956614204 ) ) ;
#19581=CARTESIAN_POINT ( 'NONE',  ( 2.474675557024783212E-16, 21.54145188432740099, -121.2109808024215170 ) ) ;
#19582=CARTESIAN_POINT ( 'NONE',  ( 3.310556943750001313, 19.41135094264166483, -101.1807724695661364 ) ) ;
#19584=DIRECTION ( 'NONE',  ( -0.000000000000000000, 1.259100132267607459E-16, -1.000000000000000000 ) ) ;
#19587=CARTESIAN_POINT ( 'NONE',  ( -7.424026671074350129E-16, 13.45854811567263454, -77.71098080242150274 ) ) ;
#19589=CARTESIAN_POINT ( 'NONE',  ( -3.310556943750001313, 17.50000000000001066, -39.76410580289947916 ) ) ;
#19590=CARTESIAN_POINT ( 'NONE',  ( 3.310556943750001313, 17.50000000000001776, -98.35160580289947063 ) ) ;
#19591=CARTESIAN_POINT ( 'NONE',  ( -1.750000000000002220, 14.46891108675447946, -65.48806413671076143 ) ) ;
#19593=CARTESIAN_POINT ( 'NONE',  ( 2.340729813953370519E-16, 21.32270188528331900, -118.1016058028994706 ) ) ;
#19599=CARTESIAN_POINT ( 'NONE',  ( -3.310556943750002201, 15.58864905735837425, -98.68077246956613635 ) ) ;
#19600=CARTESIAN_POINT ( 'NONE',  ( 0.000000000000000000, 17.50000000000002487, -149.5231586289125687 ) ) ;
#19605=CARTESIAN_POINT ( 'NONE',  ( 0.9378221735089281585, 14.00000000000001776, -81.66632260368297125 ) ) ;
#19611=CARTESIAN_POINT ( 'NONE',  ( -3.310556943750000425, 19.41135094264166128, -26.84743913623280420 ) ) ;
#19613=ADVANCED_FACE ( 'NONE', ( #6415 ), #29150, .T. ) ;
#19615=EDGE_CURVE ( 'NONE', #5345, #24347, #38032, .T. ) ;
#19618=CARTESIAN_POINT ( 'NONE',  ( -3.500000000000002220, 15.47927405783633326, -99.87764746908817415 ) ) ;
#19620=CARTESIAN_POINT ( 'NONE',  ( 0.000000000000000000, 21.00000000000002487, -149.5231586289125687 ) ) ;
#19621=CARTESIAN_POINT ( 'NONE',  ( -3.500000000000001332, 17.50000000000001776, -85.96098080242151696 ) ) ;
#19622=DIRECTION ( 'NONE',  ( -0.000000000000000000, 1.259100132267607459E-16, -1.000000000000000000 ) ) ;
#19623=CARTESIAN_POINT ( 'NONE',  ( 1.749999999999998224, 14.46891108675448478, -120.3213974700441042 ) ) ;
#19625=CARTESIAN_POINT ( 'NONE',  ( 3.310556943750001313, 17.50000000000002487, -135.3516058028994564 ) ) ;
#19626=CARTESIAN_POINT ( 'NONE',  ( 1.750000000000001110, 20.53108891324554719, -33.29431413575484555 ) ) ;
#19627=( BOUNDED_CURVE ( )  B_SPLINE_CURVE ( 2, ( #6226, #38554, #5812, #31744, #2615, #4078, #6440, #678, #26220 ),
 .UNSPECIFIED., .F., .T. ) 
 B_SPLINE_CURVE_WITH_KNOTS ( ( 3, 2, 2, 2, 3 ),
 ( 0.8145833333333333259, 0.8152777777777777679, 0.8166666666666666519, 0.8180555555555555358, 0.8187499999999999778 ),
 .UNSPECIFIED. ) 
 CURVE ( )  GEOMETRIC_REPRESENTATION_ITEM ( )  RATIONAL_B_SPLINE_CURVE ( ( 0.9330127018922194093, 0.9330127018922194093, 1.000000000000000000, 0.8660254037844387076, 1.000000000000000000, 0.8660254037844387076, 1.000000000000000000, 0.9330127018922194093, 0.9330127018922194093 ) ) 
 REPRESENTATION_ITEM ( '' )  );
#19629=CARTESIAN_POINT ( 'NONE',  ( -1.394453263437886604E-15, 14.00000000000001066, -32.71098080242150274 ) ) ;
#19631=CARTESIAN_POINT ( 'NONE',  ( -3.500000000000002220, 15.47927405783632615, -65.57139747004409003 ) ) ;
#19633=CARTESIAN_POINT ( 'NONE',  ( -1.749999999999999778, 20.53108891324556140, -139.1276474690881741 ) ) ;
#19634=CARTESIAN_POINT ( 'NONE',  ( -1.655278471875002211, 14.63297358603755249, -125.5974391362328078 ) ) ;
#19640=CARTESIAN_POINT ( 'NONE',  ( 1.750000000000001110, 20.53108891324555429, -90.29431413575483134 ) ) ;
#19641=AXIS2_PLACEMENT_3D ( 'NONE', #16830, #4058, #7895 ) ;
#19642=CARTESIAN_POINT ( 'NONE',  ( -1.749999999999999778, 20.53108891324554719, -37.12764746908817415 ) ) ;
#19643=CARTESIAN_POINT ( 'NONE',  ( -3.310556943750000425, 19.41135094264166128, -56.84743913623280775 ) ) ;
#19645=EDGE_CURVE ( 'NONE', #22806, #19567, #7681, .T. ) ;
#19646=CARTESIAN_POINT ( 'NONE',  ( 1.655278471874998436, 14.63297358603754894, -109.5182724695661420 ) ) ;
#19647=CARTESIAN_POINT ( 'NONE',  ( -1.394453263437886604E-15, 14.00000000000002132, -122.7109808024214885 ) ) ;
#19648=CARTESIAN_POINT ( 'NONE',  ( -3.500000000000002220, 15.47927405783632082, -31.57139747004410069 ) ) ;
#19650=CARTESIAN_POINT ( 'NONE',  ( -1.655278471874999990, 20.36702641396249902, -135.0182724695661420 ) ) ;
#19654=CARTESIAN_POINT ( 'NONE',  ( -3.310556943750000425, 19.41135094264166128, -70.93493913623278502 ) ) ;
#19656=CARTESIAN_POINT ( 'NONE',  ( 1.655278471874998436, 14.63297358603754184, -64.43077246956615056 ) ) ;
#19658=CARTESIAN_POINT ( 'NONE',  ( 1.655278471875001101, 20.36702641396249192, -87.18493913623278502 ) ) ;
#19660=DIRECTION ( 'NONE',  ( 0.000000000000000000, 1.000000000000000000, 0.000000000000000000 ) ) ;
#19662=CARTESIAN_POINT ( 'NONE',  ( -3.310556943750002201, 15.58864905735836714, -42.68077246956615056 ) ) ;
#19664=CARTESIAN_POINT ( 'NONE',  ( -1.655278471874999990, 20.36702641396249547, -106.9307724695661364 ) ) ;
#19666=AXIS2_PLACEMENT_3D ( 'NONE', #13236, #12611, #13436 ) ;
#19667=VERTEX_POINT ( 'NONE', #17469 ) ;
#19669=VERTEX_POINT ( 'NONE', #10660 ) ;
#19671=CARTESIAN_POINT ( 'NONE',  ( -7.022189441860112050E-16, 13.67729811471671830, -56.51410580289947205 ) ) ;
#19673=VERTEX_POINT ( 'NONE', #26611 ) ;
#19676=VECTOR ( 'NONE', #38233, 1000.000000000000000 ) ;
#19677=CYLINDRICAL_SURFACE ( 'NONE', #38273, 3.499999999999999556 ) ;
#19679=CARTESIAN_POINT ( 'NONE',  ( -1.394453263437886604E-15, 14.00000000000001066, -47.40473080337742573 ) ) ;
#19681=ORIENTED_EDGE ( 'NONE', *, *, #10494, .F. ) ;
#19682=CARTESIAN_POINT ( 'NONE',  ( 0.9378221735089286026, 21.00000000000002842, -143.2556390011600342 ) ) ;
#19683=CARTESIAN_POINT ( 'NONE',  ( -1.655278471875002211, 14.63297358603755249, -123.5974391362328078 ) ) ;
#19684=CARTESIAN_POINT ( 'NONE',  ( -1.394453263437886604E-15, 14.00000000000002132, -125.7109808024214885 ) ) ;
#19685=( BOUNDED_CURVE ( )  B_SPLINE_CURVE ( 2, ( #1069, #37212, #17649, #8068, #30614, #1481, #14458, #21042, #34020 ),
 .UNSPECIFIED., .F., .F. ) 
 B_SPLINE_CURVE_WITH_KNOTS ( ( 3, 2, 2, 2, 3 ),
 ( 0.6604166666666666519, 0.6611111111111110938, 0.6624999999999999778, 0.6638888888888888618, 0.6645833333333333037 ),
 .UNSPECIFIED. ) 
 CURVE ( )  GEOMETRIC_REPRESENTATION_ITEM ( )  RATIONAL_B_SPLINE_CURVE ( ( 0.9330127018922194093, 0.9330127018922194093, 1.000000000000000000, 0.8660254037844387076, 1.000000000000000000, 0.8660254037844387076, 1.000000000000000000, 0.9330127018922194093, 0.9330127018922194093 ) ) 
 REPRESENTATION_ITEM ( '' )  );
#19687=CARTESIAN_POINT ( 'NONE',  ( 3.310556943750001313, 17.50000000000001066, -36.35160580289946353 ) ) ;
#19690=CARTESIAN_POINT ( 'NONE',  ( -1.655278471874999990, 20.36702641396249192, -89.01827246956612782 ) ) ;
#19691=CARTESIAN_POINT ( 'NONE',  ( -1.655278471874999990, 20.36702641396249902, -141.9307724695661364 ) ) ;
#19693=DIRECTION ( 'NONE',  ( 0.000000000000000000, 1.000000000000000000, 0.000000000000000000 ) ) ;
#19694=EDGE_CURVE ( 'NONE', #27788, #20830, #7256, .T. ) ;
#19695=CARTESIAN_POINT ( 'NONE',  ( -3.500000000000001332, 17.50000000000001066, -34.65473080337742573 ) ) ;
#19697=ADVANCED_FACE ( 'NONE', ( #14482 ), #874, .T. ) ;
#19698=CARTESIAN_POINT ( 'NONE',  ( -1.655278471875002211, 14.63297358603755249, -131.6849391362327992 ) ) ;
#19699=CARTESIAN_POINT ( 'NONE',  ( -1.394453263437886604E-15, 14.00000000000001421, -56.71098080242150985 ) ) ;
#19700=CARTESIAN_POINT ( 'NONE',  ( -3.310556943750000425, 19.41135094264166483, -91.84743913623280775 ) ) ;
#19703=CARTESIAN_POINT ( 'NONE',  ( 1.750000000000001110, 20.53108891324556140, -131.9880641367107614 ) ) ;
#19704=CARTESIAN_POINT ( 'NONE',  ( 1.749999999999998224, 14.46891108675447946, -77.32139747004410424 ) ) ;
#19705=CARTESIAN_POINT ( 'NONE',  ( -1.655278471875002211, 14.63297358603754361, -58.68493913623279212 ) ) ;
#19709=CARTESIAN_POINT ( 'NONE',  ( -3.310556943750001313, 17.50000000000001776, -85.85160580289947063 ) ) ;
#19712=CARTESIAN_POINT ( 'NONE',  ( -1.655278471875002211, 14.63297358603754894, -106.5974391362328078 ) ) ;
#19713=CARTESIAN_POINT ( 'NONE',  ( -3.310556943750001313, 17.50000000000001776, -81.76410580289947916 ) ) ;
#19715=ORIENTED_EDGE ( 'NONE', *, *, #27015, .F. ) ;
#19717=CARTESIAN_POINT ( 'NONE',  ( 3.310556943749999981, 15.58864905735837070, -101.4349391362327992 ) ) ;
#19718=CARTESIAN_POINT ( 'NONE',  ( -7.424026671074350129E-16, 13.45854811567263809, -102.4047308033774186 ) ) ;
#19720=DIRECTION ( 'NONE',  ( 0.000000000000000000, 1.000000000000000000, 0.000000000000000000 ) ) ;
#19721=CARTESIAN_POINT ( 'NONE',  ( -3.500000000000002220, 15.47927405783633326, -95.57139747004409003 ) ) ;
#19722=CARTESIAN_POINT ( 'NONE',  ( 1.750000000000001110, 20.53108891324554719, -45.29431413575483845 ) ) ;
#19724=CARTESIAN_POINT ( 'NONE',  ( -1.655278471875002211, 14.63297358603754361, -65.59743913623280775 ) ) ;
#19725=CARTESIAN_POINT ( 'NONE',  ( -3.500000000000002220, 15.47927405783632082, -29.87764746908817770 ) ) ;
#19726=CARTESIAN_POINT ( 'NONE',  ( -3.310556943750000425, 19.41135094264166838, -123.8474391362327935 ) ) ;
#19729=ORIENTED_EDGE ( 'NONE', *, *, #12387, .T. ) ;
#19730=CARTESIAN_POINT ( 'NONE',  ( -1.750000000000002220, 14.46891108675447768, -42.79431413575483845 ) ) ;
#19731=CARTESIAN_POINT ( 'NONE',  ( -1.749999999999999778, 20.53108891324555429, -90.12764746908817415 ) ) ;
#19732=CARTESIAN_POINT ( 'NONE',  ( -3.310556943750000425, 19.41135094264166128, -71.84743913623280775 ) ) ;
#19733=ORIENTED_EDGE ( 'NONE', *, *, #41167, .T. ) ;
#19734=VERTEX_POINT ( 'NONE', #1094 ) ;
#19739=CARTESIAN_POINT ( 'NONE',  ( 3.310556943749999981, 15.58864905735837780, -140.3474391362327935 ) ) ;
#19742=CARTESIAN_POINT ( 'NONE',  ( 0.9378221735089300459, 21.00000000000002487, -134.2556390011600627 ) ) ;
#19743=CARTESIAN_POINT ( 'NONE',  ( -1.655278471874999990, 20.36702641396248481, -37.01827246956612782 ) ) ;
#19745=CARTESIAN_POINT ( 'NONE',  ( 2.340729813953370519E-16, 21.32270188528331900, -104.1016058028994422 ) ) ;
#19746=CARTESIAN_POINT ( 'NONE',  ( 3.310556943750001313, 17.50000000000001066, -29.26410580289948271 ) ) ;
#19748=CARTESIAN_POINT ( 'NONE',  ( 2.474675557024783212E-16, 21.54145188432739744, -101.2109808024215170 ) ) ;
#19750=LINE ( 'NONE', #32717, #25445 ) ;
#19751=CARTESIAN_POINT ( 'NONE',  ( 1.749999999999998224, 14.46891108675448123, -90.32139747004410424 ) ) ;
#19756=CARTESIAN_POINT ( 'NONE',  ( 1.750000000000001110, 20.53108891324555074, -55.29431413575484555 ) ) ;
#19758=CARTESIAN_POINT ( 'NONE',  ( -1.394453263437886604E-15, 14.00000000000001421, -66.71098080242148853 ) ) ;
#19759=CARTESIAN_POINT ( 'NONE',  ( -7.022189441860112050E-16, 13.67729811471671297, -23.51410580289947561 ) ) ;
#19760=CARTESIAN_POINT ( 'NONE',  ( 3.500000000000001776, 19.52072594216370405, -41.07139747004409003 ) ) ;
#19762=CARTESIAN_POINT ( 'NONE',  ( -1.655278471874999990, 20.36702641396248481, -29.01827246956613493 ) ) ;
#19764=CARTESIAN_POINT ( 'NONE',  ( -3.500000000000001332, 17.50000000000001776, -80.65473080337743284 ) ) ;
#19766=CARTESIAN_POINT ( 'NONE',  ( -3.500000000000002220, 15.47927405783632082, -33.57139747004410424 ) ) ;
#19768=CARTESIAN_POINT ( 'NONE',  ( 2.340729813953370519E-16, 21.32270188528331190, -85.01410580289947916 ) ) ;
#19771=CARTESIAN_POINT ( 'NONE',  ( -0.9378221735089310451, 14.00000000000002309, -123.7556390011600200 ) ) ;
#19773=CARTESIAN_POINT ( 'NONE',  ( 0.000000000000000000, 21.00000000000002487, -149.5231586289125687 ) ) ;
#19774=ORIENTED_EDGE ( 'NONE', *, *, #31450, .F. ) ;
#19775=EDGE_CURVE ( 'NONE', #6503, #15014, #14065, .T. ) ;
#19777=CARTESIAN_POINT ( 'NONE',  ( -3.310556943750000425, 19.41135094264166483, -91.84743913623280775 ) ) ;
#19781=ADVANCED_FACE ( 'NONE', ( #20016 ), #36389, .T. ) ;
#19783=CARTESIAN_POINT ( 'NONE',  ( -1.750000000000002220, 14.46891108675449011, -142.7943141357548313 ) ) ;
#19784=CARTESIAN_POINT ( 'NONE',  ( -7.022189441860112050E-16, 13.67729811471672718, -133.5141058028994507 ) ) ;
#19786=CARTESIAN_POINT ( 'NONE',  ( 1.749999999999998224, 14.46891108675447768, -64.32139747004410424 ) ) ;
#19787=EDGE_CURVE ( 'NONE', #15700, #17995, #28993, .T. ) ;
#19788=CARTESIAN_POINT ( 'NONE',  ( 3.310556943750001313, 19.41135094264166838, -117.2682724695661278 ) ) ;
#19789=ORIENTED_EDGE ( 'NONE', *, *, #36779, .F. ) ;
#19790=ORIENTED_EDGE ( 'NONE', *, *, #35483, .T. ) ;
#19791=CARTESIAN_POINT ( 'NONE',  ( 1.750000000000001110, 20.53108891324556140, -132.9880641367107614 ) ) ;
#19793=CARTESIAN_POINT ( 'NONE',  ( -3.310556943750000425, 19.41135094264166128, -73.93493913623278502 ) ) ;
#19794=CARTESIAN_POINT ( 'NONE',  ( -3.500000000000000888, 19.52072594216371826, -117.0443141357548313 ) ) ;
#19795=CARTESIAN_POINT ( 'NONE',  ( -1.394453263437886604E-15, 14.00000000000001776, -99.40473080337743284 ) ) ;
#19796=CARTESIAN_POINT ( 'NONE',  ( 3.500000000000001332, 17.50000000000002132, -105.4609808024215027 ) ) ;
#19798=CARTESIAN_POINT ( 'NONE',  ( 1.749999999999998224, 14.46891108675447946, -72.62764746908817415 ) ) ;
#19800=CARTESIAN_POINT ( 'NONE',  ( -1.655278471875002211, 14.63297358603754006, -39.59743913623281486 ) ) ;
#19801=CARTESIAN_POINT ( 'NONE',  ( 1.655278471874998436, 14.63297358603754716, -96.51827246956612782 ) ) ;
#19802=( BOUNDED_CURVE ( )  B_SPLINE_CURVE ( 2, ( #18775, #9197, #31735, #12602, #28548, #41536, #28750, #25375, #38335 ),
 .UNSPECIFIED., .F., .T. ) 
 B_SPLINE_CURVE_WITH_KNOTS ( ( 3, 2, 2, 2, 3 ),
 ( 0.4270833333333333148, 0.4277777777777777568, 0.4291666666666666408, 0.4305555555555555802, 0.4312500000000000222 ),
 .UNSPECIFIED. ) 
 CURVE ( )  GEOMETRIC_REPRESENTATION_ITEM ( )  RATIONAL_B_SPLINE_CURVE ( ( 0.9330127018922194093, 0.9330127018922194093, 1.000000000000000000, 0.8660254037844387076, 1.000000000000000000, 0.8660254037844387076, 1.000000000000000000, 0.9330127018922194093, 0.9330127018922194093 ) ) 
 REPRESENTATION_ITEM ( '' )  );
#19803=CARTESIAN_POINT ( 'NONE',  ( 2.474675557024783212E-16, 21.54145188432739388, -60.90473080337742573 ) ) ;
#19805=CARTESIAN_POINT ( 'NONE',  ( -3.310556943750002201, 15.58864905735837780, -115.7682724695661278 ) ) ;
#19812=CARTESIAN_POINT ( 'NONE',  ( 1.655278471875001101, 20.36702641396249192, -96.09743913623280775 ) ) ;
#19816=CARTESIAN_POINT ( 'NONE',  ( -3.500000000000002220, 15.47927405783632970, -87.57139747004409003 ) ) ;
#19817=CARTESIAN_POINT ( 'NONE',  ( -1.394453263437886604E-15, 14.00000000000001776, -81.71098080242150274 ) ) ;
#19818=CARTESIAN_POINT ( 'NONE',  ( -1.394453263437886604E-15, 14.00000000000001421, -70.71098080242150274 ) ) ;
#19823=CARTESIAN_POINT ( 'NONE',  ( -3.310556943750002201, 15.58864905735836537, -28.68077246956614346 ) ) ;
#19824=ORIENTED_EDGE ( 'NONE', *, *, #3927, .T. ) ;
#19829=CARTESIAN_POINT ( 'NONE',  ( -0.9378221735089310451, 14.00000000000001599, -57.75563900116002714 ) ) ;
#19831=ORIENTED_EDGE ( 'NONE', *, *, #20690, .T. ) ;
#19832=CARTESIAN_POINT ( 'NONE',  ( -3.500000000000002220, 15.47927405783632082, -37.57139747004409003 ) ) ;
#19833=DIRECTION ( 'NONE',  ( -0.000000000000000000, 1.259100132267607459E-16, -1.000000000000000000 ) ) ;
#19835=CARTESIAN_POINT ( 'NONE',  ( 2.474675557024783212E-16, 21.54145188432740099, -118.9047308033774328 ) ) ;
#19836=CARTESIAN_POINT ( 'NONE',  ( -3.500000000000000000, 19.52072594216371826, -136.0443141357548598 ) ) ;
#19837=CARTESIAN_POINT ( 'NONE',  ( 3.310556943750001313, 19.41135094264167549, -135.2682724695661420 ) ) ;
#19838=CARTESIAN_POINT ( 'NONE',  ( 3.500000000000001776, 19.52072594216370405, -26.37764746908817415 ) ) ;
#19842=CARTESIAN_POINT ( 'NONE',  ( 1.750000000000001110, 20.53108891324554719, -41.29431413575483845 ) ) ;
#19844=CARTESIAN_POINT ( 'NONE',  ( 1.750000000000001110, 20.53108891324556140, -134.2943141357548598 ) ) ;
#19845=CARTESIAN_POINT ( 'NONE',  ( -1.655278471874999990, 20.36702641396249547, -119.9307724695661364 ) ) ;
#19849=CARTESIAN_POINT ( 'NONE',  ( -1.394453263437886604E-15, 14.00000000000001776, -81.71098080242150274 ) ) ;
#19850=CARTESIAN_POINT ( 'NONE',  ( -1.749999999999999778, 20.53108891324555429, -93.12764746908815994 ) ) ;
#19851=CARTESIAN_POINT ( 'NONE',  ( 4.648177544792955347E-16, 21.00000000000001066, -41.21098080242150274 ) ) ;
#19852=CARTESIAN_POINT ( 'NONE',  ( -3.310556943750001313, 17.50000000000001421, -51.76410580289947205 ) ) ;
#19853=CARTESIAN_POINT ( 'NONE',  ( 1.655278471875001101, 20.36702641396249547, -113.1849391362327992 ) ) ;
#19854=EDGE_CURVE ( 'NONE', #30193, #25980, #34244, .T. ) ;
#19855=CARTESIAN_POINT ( 'NONE',  ( 3.500000000000000000, 15.47927405783633326, -111.2380641367107614 ) ) ;
#19856=CARTESIAN_POINT ( 'NONE',  ( -1.749999999999999778, 20.53108891324554719, -27.82139747004409713 ) ) ;
#19859=CARTESIAN_POINT ( 'NONE',  ( -1.655278471874999990, 20.36702641396249902, -132.0182724695661420 ) ) ;
#19863=CARTESIAN_POINT ( 'NONE',  ( 1.655278471874998436, 14.63297358603754184, -65.51827246956614204 ) ) ;
#19865=CARTESIAN_POINT ( 'NONE',  ( 1.655278471874998436, 14.63297358603754184, -65.43077246956615056 ) ) ;
#19867=CARTESIAN_POINT ( 'NONE',  ( 3.310556943750001313, 17.50000000000001776, -88.35160580289947063 ) ) ;
#19870=CARTESIAN_POINT ( 'NONE',  ( -1.750000000000002220, 14.46891108675448478, -103.4880641367107756 ) ) ;
#19873=CARTESIAN_POINT ( 'NONE',  ( -3.310556943750002201, 15.58864905735836714, -43.68077246956614346 ) ) ;
#19876=CARTESIAN_POINT ( 'NONE',  ( 1.655278471874998436, 14.63297358603754716, -105.4307724695661364 ) ) ;
#19878=ORIENTED_EDGE ( 'NONE', *, *, #8226, .F. ) ;
#19884=CARTESIAN_POINT ( 'NONE',  ( -1.655278471875002211, 14.63297358603754361, -58.59743913623280065 ) ) ;
#19886=( BOUNDED_CURVE ( )  B_SPLINE_CURVE ( 2, ( #8681, #18471, #21654, #34632, #1115, #36842, #15293, #17490, #1322 ),
 .UNSPECIFIED., .F., .F. ) 
 B_SPLINE_CURVE_WITH_KNOTS ( ( 3, 2, 2, 2, 3 ),
 ( 0.5354166666666666519, 0.5361111111111110938, 0.5374999999999999778, 0.5388888888888888618, 0.5395833333333333037 ),
 .UNSPECIFIED. ) 
 CURVE ( )  GEOMETRIC_REPRESENTATION_ITEM ( )  RATIONAL_B_SPLINE_CURVE ( ( 0.9330127018922194093, 0.9330127018922194093, 1.000000000000000000, 0.8660254037844387076, 1.000000000000000000, 0.8660254037844387076, 1.000000000000000000, 0.9330127018922194093, 0.9330127018922194093 ) ) 
 REPRESENTATION_ITEM ( '' )  );
#19887=VERTEX_POINT ( 'NONE', #34869 ) ;
#19888=ORIENTED_EDGE ( 'NONE', *, *, #14424, .T. ) ;
#19889=CARTESIAN_POINT ( 'NONE',  ( 0.000000000000000000, 21.00000000000002487, -149.5231586289125687 ) ) ;
#19895=ORIENTED_EDGE ( 'NONE', *, *, #4443, .F. ) ;
#19896=CARTESIAN_POINT ( 'NONE',  ( -7.424026671074350129E-16, 13.45854811567263276, -41.71098080242151696 ) ) ;
#19897=CARTESIAN_POINT ( 'NONE',  ( 3.310556943750001313, 17.50000000000001066, -44.26410580289947916 ) ) ;
#19898=CARTESIAN_POINT ( 'NONE',  ( -0.9378221735089291577, 21.00000000000002487, -139.1663226036829712 ) ) ;
#19900=DIRECTION ( 'NONE',  ( 0.000000000000000000, 0.000000000000000000, 1.000000000000000000 ) ) ;
#19902=CARTESIAN_POINT ( 'NONE',  ( 3.310556943750001313, 19.41135094264165772, -36.26827246956612782 ) ) ;
#19903=CARTESIAN_POINT ( 'NONE',  ( 3.310556943750001313, 17.50000000000001066, -23.35160580289946708 ) ) ;
#19904=CARTESIAN_POINT ( 'NONE',  ( -7.022189441860112050E-16, 13.67729811471672363, -84.60160580289947063 ) ) ;
#19905=CARTESIAN_POINT ( 'NONE',  ( -1.655278471875002211, 14.63297358603755249, -135.5974391362328220 ) ) ;
#19907=CARTESIAN_POINT ( 'NONE',  ( 4.648177544792955347E-16, 21.00000000000001421, -48.90473080337742573 ) ) ;
#19909=CARTESIAN_POINT ( 'NONE',  ( -3.500000000000000000, 19.52072594216370405, -34.73806413671076854 ) ) ;
#19910=UNCERTAINTY_MEASURE_WITH_UNIT (LENGTH_MEASURE( 1.000000000000000082E-05 ), #38027, 'distance_accuracy_value', 'NONE');
#19911=CARTESIAN_POINT ( 'NONE',  ( 3.310556943750001313, 19.41135094264166838, -129.2682724695661420 ) ) ;
#19912=CARTESIAN_POINT ( 'NONE',  ( 3.500000000000001332, 19.52072594216370760, -70.07139747004409003 ) ) ;
#19913=CARTESIAN_POINT ( 'NONE',  ( 3.310556943750001313, 19.41135094264166483, -89.18077246956613635 ) ) ;
#19914=DIRECTION ( 'NONE',  ( -0.000000000000000000, 1.259100132267607459E-16, -1.000000000000000000 ) ) ;
#19915=CARTESIAN_POINT ( 'NONE',  ( -1.750000000000002220, 14.46891108675448301, -92.79431413575484555 ) ) ;
#19916=DIRECTION ( 'NONE',  ( -0.000000000000000000, 1.259100132267607459E-16, -1.000000000000000000 ) ) ;
#19917=CARTESIAN_POINT ( 'NONE',  ( -1.750000000000002220, 14.46891108675448123, -74.48806413671076143 ) ) ;
#19918=CARTESIAN_POINT ( 'NONE',  ( 2.340729813953370519E-16, 21.32270188528331190, -61.10160580289945642 ) ) ;
#19921=CARTESIAN_POINT ( 'NONE',  ( 3.310556943750001313, 17.50000000000002487, -143.2641058028994792 ) ) ;
#19922=CARTESIAN_POINT ( 'NONE',  ( -3.310556943750000425, 19.41135094264166483, -77.93493913623279923 ) ) ;
#19923=CYLINDRICAL_SURFACE ( 'NONE', #7843, 3.499999999999999556 ) ;
#19925=CARTESIAN_POINT ( 'NONE',  ( -7.022189441860112050E-16, 13.67729811471672541, -108.5141058028994649 ) ) ;
#19926=CARTESIAN_POINT ( 'NONE',  ( 3.310556943750001313, 17.50000000000001776, -82.26410580289947916 ) ) ;
#19929=CARTESIAN_POINT ( 'NONE',  ( 1.655278471874998436, 14.63297358603754716, -100.5182724695661278 ) ) ;
#19930=CARTESIAN_POINT ( 'NONE',  ( 3.500000000000001776, 19.52072594216371826, -103.0713974700440900 ) ) ;
#19931=EDGE_CURVE ( 'NONE', #21455, #12464, #36332, .T. ) ;
#19933=CARTESIAN_POINT ( 'NONE',  ( 3.500000000000001332, 17.50000000000001421, -71.46098080242151696 ) ) ;
#19934=CARTESIAN_POINT ( 'NONE',  ( -1.394453263437886604E-15, 14.00000000000001066, -44.40473080337743284 ) ) ;
#19935=CARTESIAN_POINT ( 'NONE',  ( 4.648177544792955347E-16, 21.00000000000001066, -45.21098080242150985 ) ) ;
#19937=CARTESIAN_POINT ( 'NONE',  ( 1.655278471875001101, 20.36702641396248836, -60.09743913623280775 ) ) ;
#19939=CARTESIAN_POINT ( 'NONE',  ( -3.310556943750001313, 17.50000000000002132, -122.7641058028994649 ) ) ;
#19940=DIRECTION ( 'NONE',  ( 0.000000000000000000, 1.000000000000000000, 0.000000000000000000 ) ) ;
#19942=EDGE_LOOP ( 'NONE', ( #3779, #34432, #4079, #15823 ) ) ;
#19945=DIRECTION ( 'NONE',  ( -0.000000000000000000, 1.259100132267607459E-16, -1.000000000000000000 ) ) ;
#19946=CARTESIAN_POINT ( 'NONE',  ( 3.500000000000001332, 17.50000000000001776, -79.15473080337743284 ) ) ;
#19947=CARTESIAN_POINT ( 'NONE',  ( 2.340729813953370519E-16, 21.32270188528331190, -75.01410580289947916 ) ) ;
#19949=ORIENTED_EDGE ( 'NONE', *, *, #31200, .T. ) ;
#19951=( BOUNDED_CURVE ( )  B_SPLINE_CURVE ( 2, ( #18081, #4690, #7889, #39999, #39793, #11279, #27036, #10658, #30848 ),
 .UNSPECIFIED., .F., .T. ) 
 B_SPLINE_CURVE_WITH_KNOTS ( ( 3, 2, 2, 2, 3 ),
 ( 0.6895833333333333259, 0.6902777777777777679, 0.6916666666666666519, 0.6930555555555555358, 0.6937499999999999778 ),
 .UNSPECIFIED. ) 
 CURVE ( )  GEOMETRIC_REPRESENTATION_ITEM ( )  RATIONAL_B_SPLINE_CURVE ( ( 0.9330127018922194093, 0.9330127018922194093, 1.000000000000000000, 0.8660254037844387076, 1.000000000000000000, 0.8660254037844387076, 1.000000000000000000, 0.9330127018922194093, 0.9330127018922194093 ) ) 
 REPRESENTATION_ITEM ( '' )  );
#19957=CARTESIAN_POINT ( 'NONE',  ( -1.750000000000002220, 14.46891108675448834, -128.7943141357548313 ) ) ;
#19958=CARTESIAN_POINT ( 'NONE',  ( 4.286263797015737581E-16, 14.00000000000002487, -149.5231586289125687 ) ) ;
#19959=CARTESIAN_POINT ( 'NONE',  ( -3.500000000000000000, 19.52072594216371115, -89.73806413671076143 ) ) ;
#19960=CARTESIAN_POINT ( 'NONE',  ( -3.310556943750000425, 19.41135094264165772, -36.93493913623279923 ) ) ;
#19961=CARTESIAN_POINT ( 'NONE',  ( 3.310556943749999981, 15.58864905735837070, -103.4349391362327992 ) ) ;
#19963=CARTESIAN_POINT ( 'NONE',  ( -3.310556943750001313, 17.50000000000002487, -141.8516058028994564 ) ) ;
#19965=CARTESIAN_POINT ( 'NONE',  ( -7.424026671074350129E-16, 13.45854811567263809, -100.7109808024215027 ) ) ;
#19967=CARTESIAN_POINT ( 'NONE',  ( -3.500000000000000000, 19.52072594216371826, -119.0443141357548171 ) ) ;
#19968=CARTESIAN_POINT ( 'NONE',  ( 1.749999999999998224, 14.46891108675448123, -91.32139747004410424 ) ) ;
#19972=CARTESIAN_POINT ( 'NONE',  ( -3.500000000000001332, 17.50000000000001421, -55.96098080242150985 ) ) ;
#19974=CARTESIAN_POINT ( 'NONE',  ( 1.655278471874998436, 14.63297358603753651, -23.43077246956613990 ) ) ;
#19976=CARTESIAN_POINT ( 'NONE',  ( -3.500000000000002220, 15.47927405783632260, -41.57139747004409713 ) ) ;
#19978=AXIS2_PLACEMENT_3D ( 'NONE', #18417, #2460, #15653 ) ;
#19979=EDGE_CURVE ( 'NONE', #10589, #11928, #11934, .T. ) ;
#19980=CARTESIAN_POINT ( 'NONE',  ( -7.022189441860112050E-16, 13.67729811471671653, -28.60160580289947063 ) ) ;
#19982=DIRECTION ( 'NONE',  ( -0.000000000000000000, 1.259100132267607459E-16, -1.000000000000000000 ) ) ;
#19985=CARTESIAN_POINT ( 'NONE',  ( 1.750000000000001110, 20.53108891324555785, -101.9880641367107756 ) ) ;
#19987=CARTESIAN_POINT ( 'NONE',  ( -1.655278471875002211, 14.63297358603754539, -79.59743913623280775 ) ) ;
#19989=VERTEX_POINT ( 'NONE', #2119 ) ;
#19990=DIRECTION ( 'NONE',  ( -0.000000000000000000, 1.259100132267607459E-16, -1.000000000000000000 ) ) ;
#19991=CARTESIAN_POINT ( 'NONE',  ( 3.500000000000001332, 19.52072594216370405, -27.07139747004409358 ) ) ;
#19995=CARTESIAN_POINT ( 'NONE',  ( -3.310556943750002645, 15.58864905735837247, -91.68077246956613635 ) ) ;
#19997=ORIENTED_EDGE ( 'NONE', *, *, #20951, .F. ) ;
#20001=CARTESIAN_POINT ( 'NONE',  ( -1.394453263437886604E-15, 14.00000000000002132, -115.7109808024214885 ) ) ;
#20002=CARTESIAN_POINT ( 'NONE',  ( 2.340729813953370519E-16, 21.32270188528331900, -125.0141058028994792 ) ) ;
#20003=VECTOR ( 'NONE', #16533, 1000.000000000000000 ) ;
#20006=CARTESIAN_POINT ( 'NONE',  ( 1.655278471874998436, 14.63297358603754184, -54.51827246956612782 ) ) ;
#20007=CARTESIAN_POINT ( 'NONE',  ( 1.655278471874998436, 14.63297358603754894, -118.5182724695661278 ) ) ;
#20009=ORIENTED_EDGE ( 'NONE', *, *, #9086, .F. ) ;
#20010=CARTESIAN_POINT ( 'NONE',  ( 3.500000000000001332, 17.50000000000002132, -126.1547308033774470 ) ) ;
#20011=CARTESIAN_POINT ( 'NONE',  ( 3.310556943750001313, 17.50000000000001421, -71.35160580289947063 ) ) ;
#20012=CARTESIAN_POINT ( 'NONE',  ( -3.500000000000000888, 19.52072594216371826, -119.0443141357548456 ) ) ;
#20013=EDGE_CURVE ( 'NONE', #23833, #4297, #20645, .T. ) ;
#20014=CARTESIAN_POINT ( 'NONE',  ( -7.022189441860112050E-16, 13.67729811471672541, -100.5141058028994792 ) ) ;
#20016=FACE_OUTER_BOUND ( 'NONE', #16649, .T. ) ;
#20018=CARTESIAN_POINT ( 'NONE',  ( -3.500000000000002220, 15.47927405783632615, -70.87764746908817415 ) ) ;
#20020=CARTESIAN_POINT ( 'NONE',  ( -1.655278471874999990, 20.36702641396248481, -36.93077246956613635 ) ) ;
#20021=CARTESIAN_POINT ( 'NONE',  ( -3.310556943750001313, 17.50000000000001776, -97.85160580289945642 ) ) ;
#20022=VECTOR ( 'NONE', #41732, 1000.000000000000000 ) ;
#20023=CARTESIAN_POINT ( 'NONE',  ( -3.500000000000001332, 17.50000000000001421, -58.65473080337743284 ) ) ;
#20025=CARTESIAN_POINT ( 'NONE',  ( -3.310556943750001313, 17.50000000000002132, -114.8516058028994706 ) ) ;
#20026=CARTESIAN_POINT ( 'NONE',  ( -3.310556943750001313, 17.50000000000001066, -42.85160580289947063 ) ) ;
#20028=CARTESIAN_POINT ( 'NONE',  ( -3.500000000000001332, 17.50000000000001421, -60.96098080242150274 ) ) ;
#20031=CARTESIAN_POINT ( 'NONE',  ( 3.500000000000000000, 15.47927405783632615, -79.54431413575484555 ) ) ;
#20032=CARTESIAN_POINT ( 'NONE',  ( 1.750000000000001110, 20.53108891324555074, -61.29431413575483845 ) ) ;
#20033=CARTESIAN_POINT ( 'NONE',  ( -3.310556943750001313, 17.50000000000001776, -100.7641058028994792 ) ) ;
#20034=CARTESIAN_POINT ( 'NONE',  ( 4.648177544792955347E-16, 21.00000000000001066, -38.90473080337743284 ) ) ;
#20038=LINE ( 'NONE', #13028, #8422 ) ;
#20039=VECTOR ( 'NONE', #42005, 1000.000000000000000 ) ;
#20042=FACE_OUTER_BOUND ( 'NONE', #19057, .T. ) ;
#20044=EDGE_CURVE ( 'NONE', #12774, #15353, #39949, .T. ) ;
#20046=CARTESIAN_POINT ( 'NONE',  ( 1.655278471874998436, 14.63297358603753828, -29.43077246956614346 ) ) ;
#20053=DIRECTION ( 'NONE',  ( 0.000000000000000000, 0.000000000000000000, -1.000000000000000000 ) ) ;
#20055=CARTESIAN_POINT ( 'NONE',  ( 3.310556943749999981, 15.58864905735837780, -140.3474391362327935 ) ) ;
#20057=CARTESIAN_POINT ( 'NONE',  ( 1.743066579297357930E-14, 14.00000000000002132, -135.7109808024214885 ) ) ;
#20058=CARTESIAN_POINT ( 'NONE',  ( -7.022189441860112050E-16, 13.67729811471672896, -136.6016058028994564 ) ) ;
#20059=CARTESIAN_POINT ( 'NONE',  ( -1.749999999999999778, 20.53108891324554719, -30.12764746908817770 ) ) ;
#20063=( BOUNDED_CURVE ( )  B_SPLINE_CURVE ( 2, ( #699, #4314, #13455, #36864, #23467, #10910, #23896, #17078, #23681 ),
 .UNSPECIFIED., .F., .T. ) 
 B_SPLINE_CURVE_WITH_KNOTS ( ( 3, 2, 2, 2, 3 ),
 ( 0.5687499999999999778, 0.5694444444444444198, 0.5708333333333333037, 0.5722222222222221877, 0.5729166666666666297 ),
 .UNSPECIFIED. ) 
 CURVE ( )  GEOMETRIC_REPRESENTATION_ITEM ( )  RATIONAL_B_SPLINE_CURVE ( ( 0.9330127018922194093, 0.9330127018922194093, 1.000000000000000000, 0.8660254037844387076, 1.000000000000000000, 0.8660254037844387076, 1.000000000000000000, 0.9330127018922194093, 0.9330127018922194093 ) ) 
 REPRESENTATION_ITEM ( '' )  );
#20066=CARTESIAN_POINT ( 'NONE',  ( 3.500000000000001332, 17.50000000000002487, -131.4609808024214885 ) ) ;
#20067=CARTESIAN_POINT ( 'NONE',  ( 1.655278471875001101, 20.36702641396249547, -118.0974391362328078 ) ) ;
#20071=CARTESIAN_POINT ( 'NONE',  ( -3.500000000000001332, 17.50000000000001776, -84.96098080242150274 ) ) ;
#20072=CARTESIAN_POINT ( 'NONE',  ( -0.9378221735089310451, 14.00000000000001066, -40.75563900116003424 ) ) ;
#20073=CARTESIAN_POINT ( 'NONE',  ( 2.340729813953370519E-16, 21.32270188528330834, -51.01410580289947205 ) ) ;
#20074=CARTESIAN_POINT ( 'NONE',  ( -1.655278471874999990, 20.36702641396249547, -112.0182724695661420 ) ) ;
#20075=CARTESIAN_POINT ( 'NONE',  ( 2.474675557024783212E-16, 21.54145188432739033, -28.90473080337743639 ) ) ;
#20078=CARTESIAN_POINT ( 'NONE',  ( -3.310556943750000425, 19.41135094264167549, -132.9349391362327992 ) ) ;
#20082=CARTESIAN_POINT ( 'NONE',  ( -3.310556943750001313, 17.50000000000001421, -64.85160580289945642 ) ) ;
#20084=CARTESIAN_POINT ( 'NONE',  ( 1.655278471875001101, 20.36702641396248836, -65.09743913623280775 ) ) ;
#20086=CARTESIAN_POINT ( 'NONE',  ( -3.310556943750002201, 15.58864905735837247, -87.76827246956614204 ) ) ;
#20088=CARTESIAN_POINT ( 'NONE',  ( 0.000000000000000000, 17.50000000000002487, -149.5231586289125687 ) ) ;
#20090=CARTESIAN_POINT ( 'NONE',  ( -3.310556943750001313, 17.50000000000001066, -45.76410580289946495 ) ) ;
#20092=CARTESIAN_POINT ( 'NONE',  ( 2.340729813953370519E-16, 21.32270188528331190, -101.0141058028994792 ) ) ;
#20099=CARTESIAN_POINT ( 'NONE',  ( 2.340729813953370519E-16, 21.32270188528330834, -55.01410580289947205 ) ) ;
#20101=ORIENTED_EDGE ( 'NONE', *, *, #12405, .F. ) ;
#20102=DIRECTION ( 'NONE',  ( 0.000000000000000000, 1.000000000000000000, 0.000000000000000000 ) ) ;
#20103=CARTESIAN_POINT ( 'NONE',  ( 4.648177544792955347E-16, 21.00000000000001066, -31.21098080242150630 ) ) ;
#20106=DIRECTION ( 'NONE',  ( -0.000000000000000000, 1.259100132267607459E-16, -1.000000000000000000 ) ) ;
#20107=ORIENTED_EDGE ( 'NONE', *, *, #5292, .F. ) ;
#20109=CARTESIAN_POINT ( 'NONE',  ( 2.474675557024783212E-16, 21.54145188432739033, -45.21098080242151696 ) ) ;
#20110=CARTESIAN_POINT ( 'NONE',  ( 1.655278471875001101, 20.36702641396248481, -43.09743913623280065 ) ) ;
#20111=CARTESIAN_POINT ( 'NONE',  ( -1.749999999999999778, 20.53108891324556140, -139.1276474690881741 ) ) ;
#20112=CARTESIAN_POINT ( 'NONE',  ( 4.648177544792955347E-16, 21.00000000000001066, -43.21098080242150985 ) ) ;
#20115=CARTESIAN_POINT ( 'NONE',  ( 3.310556943749999981, 15.58864905735836182, -28.43493913623279212 ) ) ;
#20116=CARTESIAN_POINT ( 'NONE',  ( 1.655278471874998436, 14.63297358603753651, -23.51827246956612782 ) ) ;
#20117=CARTESIAN_POINT ( 'NONE',  ( 1.655278471875001101, 20.36702641396249192, -81.18493913623279923 ) ) ;
#20118=CARTESIAN_POINT ( 'NONE',  ( -7.022189441860112050E-16, 13.67729811471672718, -134.5141058028994507 ) ) ;
#20120=CARTESIAN_POINT ( 'NONE',  ( 0.9378221735089281585, 14.00000000000001066, -49.36007260463891555 ) ) ;
#20122=CARTESIAN_POINT ( 'NONE',  ( -1.655278471874999990, 20.36702641396249902, -130.0182724695661136 ) ) ;
#20123=VECTOR ( 'NONE', #38836, 1000.000000000000000 ) ;
#20125=CARTESIAN_POINT ( 'NONE',  ( -3.310556943750002645, 15.58864905735837247, -83.68077246956615056 ) ) ;
#20126=CARTESIAN_POINT ( 'NONE',  ( 0.000000000000000000, 17.50000000000002487, -149.5231586289125687 ) ) ;
#20127=CARTESIAN_POINT ( 'NONE',  ( 3.500000000000001332, 19.52072594216371115, -101.0713974700440900 ) ) ;
#20128=CARTESIAN_POINT ( 'NONE',  ( 0.9378221735089300459, 21.00000000000002132, -111.2556390011600200 ) ) ;
#20129=CARTESIAN_POINT ( 'NONE',  ( 1.750000000000001110, 20.53108891324555429, -76.98806413671076143 ) ) ;
#20131=CARTESIAN_POINT ( 'NONE',  ( -1.655278471874999990, 20.36702641396248836, -58.01827246956613493 ) ) ;
#20136=CARTESIAN_POINT ( 'NONE',  ( 3.310556943749999981, 15.58864905735836892, -81.43493913623278502 ) ) ;
#20137=FACE_OUTER_BOUND ( 'NONE', #1529, .T. ) ;
#20139=CARTESIAN_POINT ( 'NONE',  ( -3.310556943750000425, 19.41135094264166838, -110.8474391362328078 ) ) ;
#20140=CARTESIAN_POINT ( 'NONE',  ( 3.310556943750001313, 19.41135094264166483, -81.18077246956615056 ) ) ;
#20141=CARTESIAN_POINT ( 'NONE',  ( 3.500000000000000000, 15.47927405783632437, -57.23806413671076854 ) ) ;
#20143=CARTESIAN_POINT ( 'NONE',  ( 3.310556943750001313, 17.50000000000001776, -99.35160580289947063 ) ) ;
#20145=CARTESIAN_POINT ( 'NONE',  ( 3.500000000000001776, 19.52072594216371826, -104.0713974700440900 ) ) ;
#20147=CARTESIAN_POINT ( 'NONE',  ( -1.394453263437886604E-15, 14.00000000000001776, -94.40473080337744705 ) ) ;
#20148=CARTESIAN_POINT ( 'NONE',  ( 7.367361408496833051E-14, 14.00000000000001776, -95.40473080337743284 ) ) ;
#20149=CARTESIAN_POINT ( 'NONE',  ( 4.648177544792955347E-16, 21.00000000000001421, -57.90473080337742573 ) ) ;
#20151=CARTESIAN_POINT ( 'NONE',  ( 2.340729813953370519E-16, 21.32270188528331190, -62.01410580289947205 ) ) ;
#20154=CARTESIAN_POINT ( 'NONE',  ( -3.310556943750000425, 19.41135094264166838, -113.8474391362328078 ) ) ;
#20155=LINE ( 'NONE', #39713, #35247 ) ;
#20158=ORIENTED_EDGE ( 'NONE', *, *, #40371, .F. ) ;
#20161=CARTESIAN_POINT ( 'NONE',  ( 0.000000000000000000, 17.50000000000002487, -149.5231586289125687 ) ) ;
#20162=CARTESIAN_POINT ( 'NONE',  ( -3.310556943750002645, 15.58864905735837070, -73.68077246956615056 ) ) ;
#20164=ORIENTED_EDGE ( 'NONE', *, *, #6019, .F. ) ;
#20165=EDGE_CURVE ( 'NONE', #15124, #18319, #40678, .T. ) ;
#20169=ORIENTED_EDGE ( 'NONE', *, *, #18600, .T. ) ;
#20170=CARTESIAN_POINT ( 'NONE',  ( 1.655278471875001101, 20.36702641396249902, -133.0974391362328220 ) ) ;
#20171=DIRECTION ( 'NONE',  ( -0.000000000000000000, 1.259100132267607459E-16, -1.000000000000000000 ) ) ;
#20172=CARTESIAN_POINT ( 'NONE',  ( 2.340729813953370519E-16, 21.32270188528330479, -46.10160580289946353 ) ) ;
#20174=CARTESIAN_POINT ( 'NONE',  ( 1.655278471874998436, 14.63297358603753828, -37.51827246956612782 ) ) ;
#20175=CARTESIAN_POINT ( 'NONE',  ( 2.340729813953370519E-16, 21.32270188528331190, -97.10160580289947063 ) ) ;
#20177=CARTESIAN_POINT ( 'NONE',  ( 3.310556943749999981, 15.58864905735836004, -24.34743913623281486 ) ) ;
#20178=CARTESIAN_POINT ( 'NONE',  ( 4.648177544792955347E-16, 21.00000000000001776, -80.21098080242148853 ) ) ;
#20179=CARTESIAN_POINT ( 'NONE',  ( -1.750000000000002220, 14.46891108675448478, -99.79431413575484555 ) ) ;
#20180=CARTESIAN_POINT ( 'NONE',  ( 1.750000000000001110, 20.53108891324556140, -141.9880641367107614 ) ) ;
#20181=CARTESIAN_POINT ( 'NONE',  ( 1.750000000000001110, 20.53108891324555429, -89.98806413671076143 ) ) ;
#20188=CARTESIAN_POINT ( 'NONE',  ( 1.750000000000001110, 20.53108891324555074, -54.29431413575484555 ) ) ;
#20189=CARTESIAN_POINT ( 'NONE',  ( -1.749999999999999778, 20.53108891324555074, -46.82139747004410424 ) ) ;
#20190=CARTESIAN_POINT ( 'NONE',  ( -3.310556943750002645, 15.58864905735836182, -23.68077246956613635 ) ) ;
#20192=EDGE_CURVE ( 'NONE', #21662, #36251, #24997, .T. ) ;
#20193=CARTESIAN_POINT ( 'NONE',  ( -3.500000000000000888, 19.52072594216370405, -44.73806413671075433 ) ) ;
#20195=CARTESIAN_POINT ( 'NONE',  ( 2.340729813953370519E-16, 21.32270188528330834, -25.10160580289946708 ) ) ;
#20197=CARTESIAN_POINT ( 'NONE',  ( 4.648177544792955347E-16, 21.00000000000001066, -44.21098080242150985 ) ) ;
#20200=CARTESIAN_POINT ( 'NONE',  ( 1.655278471875001101, 20.36702641396249192, -79.09743913623280775 ) ) ;
#20202=CARTESIAN_POINT ( 'NONE',  ( -1.750000000000002220, 14.46891108675448478, -97.79431413575484555 ) ) ;
#20203=( BOUNDED_CURVE ( )  B_SPLINE_CURVE ( 2, ( #28539, #25367, #9189, #2176, #34092, #4950, #1768, #14750, #27706 ),
 .UNSPECIFIED., .F., .T. ) 
 B_SPLINE_CURVE_WITH_KNOTS ( ( 3, 2, 2, 2, 3 ),
 ( 0.7645833333333332815, 0.7652777777777777235, 0.7666666666666667185, 0.7680555555555556024, 0.7687500000000000444 ),
 .UNSPECIFIED. ) 
 CURVE ( )  GEOMETRIC_REPRESENTATION_ITEM ( )  RATIONAL_B_SPLINE_CURVE ( ( 0.9330127018922194093, 0.9330127018922194093, 1.000000000000000000, 0.8660254037844387076, 1.000000000000000000, 0.8660254037844387076, 1.000000000000000000, 0.9330127018922194093, 0.9330127018922194093 ) ) 
 REPRESENTATION_ITEM ( '' )  );
#20204=CARTESIAN_POINT ( 'NONE',  ( -1.394453263437886604E-15, 14.00000000000001066, -27.40473080337743284 ) ) ;
#20205=ORIENTED_EDGE ( 'NONE', *, *, #1488, .F. ) ;
#20206=FACE_OUTER_BOUND ( 'NONE', #2296, .T. ) ;
#20207=CARTESIAN_POINT ( 'NONE',  ( 1.655278471875001101, 20.36702641396249192, -90.09743913623280775 ) ) ;
#20208=VERTEX_POINT ( 'NONE', #40376 ) ;
#20212=CARTESIAN_POINT ( 'NONE',  ( 1.750000000000001110, 20.53108891324555785, -115.2943141357548313 ) ) ;
#20214=CARTESIAN_POINT ( 'NONE',  ( -1.655278471875002211, 14.63297358603755249, -126.5974391362328078 ) ) ;
#20215=ADVANCED_FACE ( 'NONE', ( #8043 ), #40577, .T. ) ;
#20218=CARTESIAN_POINT ( 'NONE',  ( -1.655278471875002211, 14.63297358603754184, -52.68493913623280633 ) ) ;
#20219=CARTESIAN_POINT ( 'NONE',  ( -1.655278471874999990, 20.36702641396249547, -114.0182724695661278 ) ) ;
#20220=ORIENTED_EDGE ( 'NONE', *, *, #20521, .F. ) ;
#20221=CARTESIAN_POINT ( 'NONE',  ( 1.750000000000001110, 20.53108891324555785, -125.9880641367107614 ) ) ;
#20222=CARTESIAN_POINT ( 'NONE',  ( -7.022189441860112050E-16, 13.67729811471671653, -42.51410580289947916 ) ) ;
#20223=CARTESIAN_POINT ( 'NONE',  ( 3.310556943750001313, 19.41135094264166128, -74.26827246956614204 ) ) ;
#20224=CARTESIAN_POINT ( 'NONE',  ( -3.500000000000001332, 17.50000000000002132, -115.9609808024215027 ) ) ;
#20225=CARTESIAN_POINT ( 'NONE',  ( 1.655278471875001101, 20.36702641396249547, -102.0974391362328220 ) ) ;
#20226=EDGE_CURVE ( 'NONE', #19149, #30668, #23630, .T. ) ;
#20230=CARTESIAN_POINT ( 'NONE',  ( -3.500000000000000888, 19.52072594216370760, -71.04431413575484555 ) ) ;
#20231=CYLINDRICAL_SURFACE ( 'NONE', #19208, 3.499999999999999556 ) ;
#20232=CARTESIAN_POINT ( 'NONE',  ( 1.655278471875001101, 20.36702641396248481, -35.09743913623280775 ) ) ;
#20233=CARTESIAN_POINT ( 'NONE',  ( -1.655278471875002211, 14.63297358603754894, -96.68493913623279923 ) ) ;
#20235=CARTESIAN_POINT ( 'NONE',  ( -3.500000000000001332, 17.50000000000001421, -59.65473080337743994 ) ) ;
#20237=CARTESIAN_POINT ( 'NONE',  ( 1.655278471874998436, 14.63297358603754894, -113.5182724695661278 ) ) ;
#20238=CARTESIAN_POINT ( 'NONE',  ( -7.022189441860112050E-16, 13.67729811471671830, -41.60160580289947063 ) ) ;
#20245=CARTESIAN_POINT ( 'NONE',  ( -3.310556943750001313, 17.50000000000001776, -91.76410580289947916 ) ) ;
#20250=CARTESIAN_POINT ( 'NONE',  ( -3.500000000000002220, 15.47927405783632793, -70.87764746908817415 ) ) ;
#20251=ORIENTED_EDGE ( 'NONE', *, *, #24616, .F. ) ;
#20254=CARTESIAN_POINT ( 'NONE',  ( -7.022189441860112050E-16, 13.67729811471671653, -31.51410580289946850 ) ) ;
#20263=CARTESIAN_POINT ( 'NONE',  ( -3.310556943750000425, 19.41135094264167549, -141.8474391362327935 ) ) ;
#20264=CARTESIAN_POINT ( 'NONE',  ( -3.500000000000000000, 19.52072594216371115, -81.04431413575484555 ) ) ;
#20265=CARTESIAN_POINT ( 'NONE',  ( 4.648177544792955347E-16, 21.00000000000001776, -74.90473080337743284 ) ) ;
#20266=CARTESIAN_POINT ( 'NONE',  ( 2.340729813953370519E-16, 21.32270188528332255, -136.1016058028994564 ) ) ;
#20267=CARTESIAN_POINT ( 'NONE',  ( -1.750000000000002220, 14.46891108675447590, -29.79431413575483845 ) ) ;
#20270=CARTESIAN_POINT ( 'NONE',  ( -7.424026671074350129E-16, 13.45854811567264164, -141.4047308033774186 ) ) ;
#20272=CARTESIAN_POINT ( 'NONE',  ( -1.749999999999999778, 20.53108891324556140, -133.1276474690881741 ) ) ;
#20273=CARTESIAN_POINT ( 'NONE',  ( -3.310556943750000425, 19.41135094264166838, -116.8474391362328078 ) ) ;
#20276=CARTESIAN_POINT ( 'NONE',  ( 1.743066579297357930E-14, 14.00000000000002132, -128.7109808024214885 ) ) ;
#20277=CARTESIAN_POINT ( 'NONE',  ( 2.474675557024783212E-16, 21.54145188432739744, -84.21098080242148853 ) ) ;
#20280=CARTESIAN_POINT ( 'NONE',  ( 3.310556943750001313, 19.41135094264166128, -53.18077246956613635 ) ) ;
#20281=CARTESIAN_POINT ( 'NONE',  ( 1.655278471874998436, 14.63297358603754894, -114.5182724695661278 ) ) ;
#20283=CARTESIAN_POINT ( 'NONE',  ( -3.500000000000001332, 17.50000000000001066, -29.65473080337743994 ) ) ;
#20285=CARTESIAN_POINT ( 'NONE',  ( -3.310556943750002201, 15.58864905735837780, -126.7682724695661136 ) ) ;
#20288=DIRECTION ( 'NONE',  ( -0.000000000000000000, 1.259100132267607459E-16, -1.000000000000000000 ) ) ;
#20289=CARTESIAN_POINT ( 'NONE',  ( -7.022189441860112050E-16, 13.67729811471671830, -66.60160580289947063 ) ) ;
#20291=CARTESIAN_POINT ( 'NONE',  ( 3.310556943750001313, 19.41135094264166128, -62.18077246956614346 ) ) ;
#20293=CARTESIAN_POINT ( 'NONE',  ( 1.655278471874998436, 14.63297358603754539, -83.51827246956614204 ) ) ;
#20294=CARTESIAN_POINT ( 'NONE',  ( 1.749999999999998224, 14.46891108675447413, -26.32139747004409713 ) ) ;
#20298=CARTESIAN_POINT ( 'NONE',  ( 3.310556943750001313, 19.41135094264166128, -43.18077246956614346 ) ) ;
#20300=CARTESIAN_POINT ( 'NONE',  ( -3.310556943750000425, 19.41135094264166483, -99.84743913623282197 ) ) ;
#20301=CARTESIAN_POINT ( 'NONE',  ( 0.9378221735089300459, 21.00000000000001421, -52.94938900211595723 ) ) ;
#20302=EDGE_LOOP ( 'NONE', ( #24541, #40921, #27576, #20847 ) ) ;
#20306=CARTESIAN_POINT ( 'NONE',  ( -7.022189441860112050E-16, 13.67729811471671653, -51.51410580289947916 ) ) ;
#20307=ORIENTED_EDGE ( 'NONE', *, *, #20226, .F. ) ;
#20308=ORIENTED_EDGE ( 'NONE', *, *, #23653, .F. ) ;
#20310=( BOUNDED_CURVE ( )  B_SPLINE_CURVE ( 2, ( #39466, #25678, #32875, #13109, #25884, #340, #6309, #33084, #41846 ),
 .UNSPECIFIED., .F., .F. ) 
 B_SPLINE_CURVE_WITH_KNOTS ( ( 3, 2, 2, 2, 3 ),
 ( 0.2395833333333333426, 0.2402777777777777846, 0.2416666666666666685, 0.2430555555555555525, 0.2437499999999999944 ),
 .UNSPECIFIED. ) 
 CURVE ( )  GEOMETRIC_REPRESENTATION_ITEM ( )  RATIONAL_B_SPLINE_CURVE ( ( 0.9330127018922194093, 0.9330127018922194093, 1.000000000000000000, 0.8660254037844387076, 1.000000000000000000, 0.8660254037844387076, 1.000000000000000000, 0.9330127018922194093, 0.9330127018922194093 ) ) 
 REPRESENTATION_ITEM ( '' )  );
#20311=CARTESIAN_POINT ( 'NONE',  ( -1.749999999999999778, 20.53108891324555429, -98.82139747004409003 ) ) ;
#20312=CARTESIAN_POINT ( 'NONE',  ( -1.749999999999999778, 20.53108891324555429, -96.12764746908817415 ) ) ;
#20314=( BOUNDED_CURVE ( )  B_SPLINE_CURVE ( 2, ( #31866, #2735, #41453, #25286, #22298, #19115, #2949, #15939, #29514 ),
 .UNSPECIFIED., .F., .T. ) 
 B_SPLINE_CURVE_WITH_KNOTS ( ( 3, 2, 2, 2, 3 ),
 ( 0.7437500000000000222, 0.7444444444444444642, 0.7458333333333333481, 0.7472222222222222321, 0.7479166666666666741 ),
 .UNSPECIFIED. ) 
 CURVE ( )  GEOMETRIC_REPRESENTATION_ITEM ( )  RATIONAL_B_SPLINE_CURVE ( ( 0.9330127018922194093, 0.9330127018922194093, 1.000000000000000000, 0.8660254037844387076, 1.000000000000000000, 0.8660254037844387076, 1.000000000000000000, 0.9330127018922194093, 0.9330127018922194093 ) ) 
 REPRESENTATION_ITEM ( '' )  );
#20315=CARTESIAN_POINT ( 'NONE',  ( -1.394453263437886604E-15, 14.00000000000001776, -102.4047308033774186 ) ) ;
#20316=EDGE_LOOP ( 'NONE', ( #36743, #25866, #12034, #4980 ) ) ;
#20317=CARTESIAN_POINT ( 'NONE',  ( 2.474675557024783212E-16, 21.54145188432739033, -46.21098080242150274 ) ) ;
#20318=CARTESIAN_POINT ( 'NONE',  ( 1.749999999999998224, 14.46891108675448301, -108.6276474690881741 ) ) ;
#20319=CARTESIAN_POINT ( 'NONE',  ( 1.749999999999998224, 14.46891108675448301, -97.32139747004409003 ) ) ;
#20320=CARTESIAN_POINT ( 'NONE',  ( 0.9378221735089300459, 21.00000000000001776, -77.94938900211595012 ) ) ;
#20322=CARTESIAN_POINT ( 'NONE',  ( 3.310556943750001313, 19.41135094264165772, -29.26827246956613138 ) ) ;
#20323=CARTESIAN_POINT ( 'NONE',  ( -1.749999999999999778, 20.53108891324555429, -97.82139747004409003 ) ) ;
#20324=CARTESIAN_POINT ( 'NONE',  ( 3.310556943749999981, 15.58864905735836892, -83.43493913623279923 ) ) ;
#20325=CARTESIAN_POINT ( 'NONE',  ( 1.655278471874998436, 14.63297358603755072, -135.4307724695661364 ) ) ;
#20326=EDGE_CURVE ( 'NONE', #11775, #37668, #39636, .T. ) ;
#20330=CARTESIAN_POINT ( 'NONE',  ( 1.750000000000001110, 20.53108891324555429, -85.29431413575483134 ) ) ;
#20331=CARTESIAN_POINT ( 'NONE',  ( 2.340729813953370519E-16, 21.32270188528331900, -126.1016058028994706 ) ) ;
#20332=CARTESIAN_POINT ( 'NONE',  ( 4.648177544792955347E-16, 21.00000000000001421, -50.90473080337743284 ) ) ;
#20333=CARTESIAN_POINT ( 'NONE',  ( -3.310556943750001313, 17.50000000000001776, -87.76410580289947916 ) ) ;
#20335=CARTESIAN_POINT ( 'NONE',  ( 1.749999999999998224, 14.46891108675448301, -101.3213974700440900 ) ) ;
#20336=CYLINDRICAL_SURFACE ( 'NONE', #7808, 3.499999999999999556 ) ;
#20337=CARTESIAN_POINT ( 'NONE',  ( -3.500000000000001332, 17.50000000000001421, -73.65473080337743284 ) ) ;
#20338=CARTESIAN_POINT ( 'NONE',  ( -3.310556943750001313, 17.50000000000001421, -52.85160580289946353 ) ) ;
#20340=CARTESIAN_POINT ( 'NONE',  ( -1.394453263437886604E-15, 14.00000000000001066, -41.40473080337741862 ) ) ;
#20341=CARTESIAN_POINT ( 'NONE',  ( -3.500000000000001332, 17.50000000000001776, -98.96098080242150274 ) ) ;
#20342=CARTESIAN_POINT ( 'NONE',  ( 1.655278471875001101, 20.36702641396249192, -82.18493913623278502 ) ) ;
#20343=CARTESIAN_POINT ( 'NONE',  ( 3.310556943750001313, 19.41135094264167549, -140.2682724695661420 ) ) ;
#20346=CARTESIAN_POINT ( 'NONE',  ( -3.310556943750002201, 15.58864905735837780, -109.6807724695661506 ) ) ;
#20347=CARTESIAN_POINT ( 'NONE',  ( -7.022189441860112050E-16, 13.67729811471672186, -75.51410580289946495 ) ) ;
#20348=CARTESIAN_POINT ( 'NONE',  ( -7.460324959392693302E-14, 21.00000000000001776, -101.2109808024215170 ) ) ;
#20350=CARTESIAN_POINT ( 'NONE',  ( 3.310556943750001313, 17.50000000000002132, -104.3516058028994564 ) ) ;
#20351=CARTESIAN_POINT ( 'NONE',  ( -3.500000000000001332, 17.50000000000002132, -103.6547308033774186 ) ) ;
#20353=CARTESIAN_POINT ( 'NONE',  ( 0.9378221735089281585, 14.00000000000001599, -71.66632260368301388 ) ) ;
#20357=CARTESIAN_POINT ( 'NONE',  ( 3.310556943750001313, 19.41135094264166483, -61.18077246956614346 ) ) ;
#20359=CARTESIAN_POINT ( 'NONE',  ( -3.310556943750001313, 17.50000000000002132, -115.7641058028994792 ) ) ;
#20363=ORIENTED_EDGE ( 'NONE', *, *, #17303, .F. ) ;
#20364=ORIENTED_EDGE ( 'NONE', *, *, #30701, .T. ) ;
#20367=CARTESIAN_POINT ( 'NONE',  ( -1.394453263437886604E-15, 14.00000000000002132, -109.7109808024215170 ) ) ;
#20368=CARTESIAN_POINT ( 'NONE',  ( -1.655278471874999990, 20.36702641396248836, -70.93077246956613635 ) ) ;
#20372=CARTESIAN_POINT ( 'NONE',  ( 0.000000000000000000, 20.99999999999998934, 153.5815388724490163 ) ) ;
#20376=EDGE_CURVE ( 'NONE', #13874, #24713, #8248, .T. ) ;
#20377=CARTESIAN_POINT ( 'NONE',  ( 3.310556943750001313, 17.50000000000002487, -135.2641058028994507 ) ) ;
#20379=CARTESIAN_POINT ( 'NONE',  ( -1.836030130193217234E-14, 21.00000000000002487, -135.2109808024214885 ) ) ;
#20380=CARTESIAN_POINT ( 'NONE',  ( 3.310556943749999981, 15.58864905735836182, -46.43493913623279212 ) ) ;
#20381=CARTESIAN_POINT ( 'NONE',  ( -3.310556943750002645, 15.58864905735836714, -40.76827246956613493 ) ) ;
#20382=CARTESIAN_POINT ( 'NONE',  ( 2.340729813953370519E-16, 21.32270188528331190, -100.1016058028994564 ) ) ;
#20385=CARTESIAN_POINT ( 'NONE',  ( 3.310556943749999981, 15.58864905735836182, -26.34743913623280065 ) ) ;
#20386=CARTESIAN_POINT ( 'NONE',  ( 0.9378221735089281585, 14.00000000000002132, -121.6663226036829855 ) ) ;
#20387=CARTESIAN_POINT ( 'NONE',  ( 1.750000000000001110, 20.53108891324555429, -101.2943141357548456 ) ) ;
#20390=FACE_OUTER_BOUND ( 'NONE', #28983, .T. ) ;
#20391=CARTESIAN_POINT ( 'NONE',  ( -7.424026671074350129E-16, 13.45854811567263631, -89.40473080337743284 ) ) ;
#20393=( BOUNDED_SURFACE ( )  B_SPLINE_SURFACE ( 1, 2, ( 
 ( #4736, #4318, #10701, #7728, #23471, #39840, #13889, #7512, #17300, #30264, #703, #33676, #26656, #1551, #26868, #13675, #17714, #24312, #27079, #10486, #7299, #20270, #14531, #20699, #33236, #40045, #23685, #4529, #3891, #33455, #1135, #4100, #17083, #30049, #17509, #922, #14106, #16872, #30473, #27503, #10914, #23900, #30685, #36868, #40260, #1343, #14316, #11129, #24110, #37082, #7937, #40471, #37282, #8134, #21113, #37694, #21321, #28113, #18132, #40880, #14937, #31718, #24941, #31514, #15372, #8551, #34498, #2383, #14739, #31304, #28320, #4943, #31102, #41097, #21529, #37487, #2164, #5356, #34291, #24731, #15150, #27698, #5155, #41519, #41306, #25145, #34706, #2586, #8758, #12154, #17922, #25355, #12370, #30899, #8341, #1956, #38313, #27906, #38110, #18333, #11735, #40668, #5571, #11526, #9178, #1759, #5783, #8967, #34085, #21940, #11946, #24518, #37900, #18759, #21732, #18547, #34916, #15571, #28529, #9607, #22356, #29354, #19791, #26194, #29574, #32757, #16001, #6409, #3009, #19380, #28942, #5989, #29145, #13207, #32353, #22568, #22783, #438, #25770, #10024, #25566, #38527, #35333, #39143, #25981, #13002, #41727, #35953, #3626, #13410, #26394, #39345, #31928, #3419, #12787, #41939, #22986, #9393, #16411, #38736, #6817, #35755, #3217, #226, #16614, #35546, #22154, #35125, #18963, #38946, #6198, #16202, #2799, #21, #19173, #9824, #6616, #19579, #32552, #15783, #28731, #12581, #32146, #39788, #27240, #40203, #33399, #39993, #10860, #7249, #866, #36812, #27446, #17031, #10223, #7884, #17462, #17248, #39562, #13838, #7032, #23632, #4480, #7459, #20010, #30210, #20221, #29784, #29994, #26820, #1291, #4048, #24057, #4264, #14262, #13620, #10653, #14058, #23194, #11073, #36595, #32974, #1087, #37026, #3841, #33624, #36159, #647, #20434, #23845, #26604, #16820, #20852, #27030, #17664, #10440, #7672, #23417, #20646, #36382, #30421, #33183, #33826, #4684, #30628, #1494, #14473, #8081, #4886, #11273, #21057, #17867, #40414, #34033, #30840, #1703, #37226, #14684, #24256, #38571, #28988, #35593, #19009, #25609, #3672, #3462, #29402, #38989, #35997, #13043, #32596, #22200, #29617, #16658, #19623, #28778, #10065, #35168, #483, #32395, #6244, #31976, #23028, #16245, #9436, #16451, #13253, #6456, #26238, #6863, #41774, #19835, #6658, #13454, #22403, #271, #39188, #65, #9871, #38363, #29187, #19426, #3261, #32803, #22827, #35796, #6033, #9228, #2844, #15835, #38782, #3056, #26025, #12630, #32192, #19220, #41985, #9653, #22615, #35381, #16048, #12834, #25818, #37202, #40175, #2084, #21646, #37405, #20831, #4658, #30602, #24858, #31023, #33802, #8262, #24232, #14858, #14233, #8057, #21031, #24026, #14445, #27421, #27826, #17637, #1470, #27212, #40798, #37817, #40389, #11250, #34007, #8673, #1876, #4860, #21237, #17840, #11651, #11045, #30812, #1674, #36998, #14659, #27621, #24648, #40590, #11447, #7860, #37610, #34623, #24438, #34209, #15068, #5068, #8466, #18049, #21444, #34419, #5278, #18252, #31222, #28032, #41012, #5488, #31431, #11863, #18464, #38451, #28447, #9097, #25269, #42069, #35252, #41865, #25694, #5910, #2717, #12716, #25064, #41648, #38657, #15284, #41435, #9313, #31849, #5702, #12501, #18882, #2507, #35047, #25488, #38025, #31641, #9743, #9525, #35467, #2929, #12924, #19093, #22486, #28240, #35682, #22703, #6327, #34835, #16134, #41227, #6546, #22279, #12285, #8888, #29074, #6115, #15494, #19302, #32277, #32059, #3144, #25901, #18679, #38868, #19511, #2297, #38236, #12069, #21859, #15918, #28866, #22077, #15702, #28656, #571, #790, #33104, #3971, #29276, #30129, #16952, #7376, #32895, #39270, #36299, #9955, #26323, #363, #23119, #3761, #16745, #16335, #20145, #13131, #1006, #13341, #149, #20351, #39915, #13542, #26743, #3347, #29493, #26530, #19930, #35879, #29708, #36086, #32686, #6955, #39488, #26113, #19718, #10777, #39703, #23555, #29919, #13974, #7174, #10576, #39071, #23760, #36727, #13764, #22915, #4185, #6744, #7589, #10362, #10150, #3547, #17168, #23338, #16542, #36515, #33318, #26953, #32481, #23979, #33540, #36946, #40124, #20565, #30340, #4401, #17379, #1213, #14180, #27157, #10992, #28687, #41679, #28902, #19130, #32095, #15319, #16165, #2963, #35503, #18913, #25302, #22312, #38058, #12319, #28479, #9129, #31879, #2749, #2332, #6150, #41256, #29105, #41468, #28275, #6361, #25938, #12534, #25094, #8917, #34866, #42104, #35288, #21889, #25518, #38264, #15953, #18494, #22108, #35079, #12102, #18712, #31671, #41898, #5736, #2539, #31464, #12747, #12957, #15522, #38484, #19336, #5939, #25727, #15732, #9346, #38690, #9562, #22518, #32308, #3177, #38901, #9780, #35714, #22738, #35912, #605, #32718, #13372, #29530, #4224, #39521, #4006, #29954, #10185, #6992, #16991, #29311, #3798, #22944, #3382, #39746, #10400, #14018, #23802, #23152, #6778, #13580, #3581, #26354, #397, #17206, #23375, #827, #13800, #36120, #19968, #26781, #184, #16783, #10613, #19541, #16577, #26564, #32934, #9982, #29741, #36339, #19751, #39305, #7211, #13163, #20181, #26989, #23593, #36551, #33143, #30168, #7418, #20391, #32512, #39952, #10815, #33356, #39101, #1045, #16368, #6576, #26151, #4646, #30381, #21434, #14648, #24016, #1866, #11641, #33995, #24637, #8455, #40165, #34407, #5057, #28022, #36988, #18036, #37600, #40579, #37394, #2072, #27611, #4849, #17827, #31012, #8250, #21226, #33582, #5267, #34197, #18240, #37190, #1459, #11433, #14221, #30591, #17625, #27408, #8045, #21019, #20603, #24426, #17422, #31212, #14433, #4442, #15057, #41001, #30801, #1251, #27199, #11032, #11851, #14846, #7849, #1661, #40377, #27815, #36766, #11239, #24221, #20818, #33791, #40788, #7629, #31421, #28230, #24850, #38440, #6316, #5476, #2705, #12705, #18452, #6101, #8662, #15271, #9085, #9302, #22267, #2287, #42057, #21634, #38644, #32049, #16122, #35240, #22065, #37807, #2495, #9512, #8877, #38224, #25051, #38013, #18870, #12273, #21848, #2918, #22473, #28854, #32266, #35455, #18666, #35036, #5691, #5897, #31630, #34612, #31834, #15907, #15691, #25257, #25475, #3132, #28435, #25683, #41217, #12059, #34823, #41853, #28647, #41637, #15481, #19291, #29063, #41424, #12490, #19082, #22692, #36286, #3533, #6729, #3958, #16322, #7160, #19704, #26729, #26516, #23104, #20129, #776, #16529, #36502, #4170, #13749, #3746, #39059, #32672, #7364, #6940, #135, #29478, #29694, #10137, #349, #13327, #23325, #32469, #39690, #26310, #29906, #10563, #36073, #558, #13528, #9943, #39257, #39474, #30116, #19917, #12912, #23543, #33091, #32882, #13118, #16732, #9732, #10348, #16938, #20337, #35669, #33304, #22901, #3334, #17152, #25890, #38854, #6533, #19499, #29264, #26101, #35865, #4594, #4801, #13961, #34145, #7795, #26940, #17367, #30328, #34360, #14166, #8199, #14380, #40110, #7577, #21172, #7998, #1200, #33740, #39901, #27355, #37345, #40329, #10763, #20969, #10979, #20551, #20769, #30537, #5005, #36933, #14799, #24176, #17986, #4388, #1405, #17779, #23746, #30963, #11192, #36713, #27142, #23965, #5218, #37145, #1820, #33942, #30751, #33527, #14594, #1615, #18194, #27568, #27763, #40734, #993, #40535, #11390, #24376, #11590, #24585, #37548, #8402, #21381, #31944, #25785, #19187, #2815, #38960, #29370, #35767, #39154, #238, #25579, #16015, #12597, #28957, #38540, #15585, #38751, #22795, #41953, #32159, #32366, #10036, #35349, #19591, #35139, #6001, #15798, #6628, #35560, #22585, #9193, #3431, #13221, #22996, #35967, #6830, #41532, #13016, #22371, #9407, #32564, #18977, #25995, #6213, #16423, #3230, #12801, #9837, #26206, #3022, #31162, #2599, #28544, #6423, #28746, #9621, #12385, #19394, #41742, #16213, #29157, #35, #25371, #38331, #22170, #39357, #20660, #7262, #36826, #7687, #881, #7474, #20448, #16834, #10453, #4279, #37039, #26617, #19803, #17476, #27258, #32772, #23430, #7044, #13852, #3855, #39578, #661, #30435, #10666, #17262, #1100, #36395, #20235, #30224, #450, #17045, #14071, #3639, #29796, #26832, #33196, #23206, #30008, #4061, #20023, #39801, #23647, #13421, #32987, #40218, #27044, #10877, #33414, #1304, #36610, #40007, #16627, #11089, #24073, #23862, #10237, #33639, #29586, #26407, #4493, #13634, #36173, #14277, #27862, #37241, #15108, #24897, #5111, #37857, #21688, #11286, #34662, #18289, #41265, #8095, #31262, #8715, #11690, #8508, #15326, #40838, #18090, #31061, #2125, #21483, #34456, #4698, #5530, #5316, #18502, #8302, #14699, #24689, #27461, #1718, #17884, #40628, #21281, #34251, #33839, #37650, #30646, #31472, #30856, #17679, #2339, #28280, #1914, #14490, #40428, #24271, #12109, #28071, #21073, #14893, #27657, #41051, #7899, #11488, #24478, #1511, #34046, #4902, #11903, #37447, #25103, #20868, #9570, #19548, #18719, #15960, #25946, #31678, #19343, #21896, #28485, #22319, #22528, #12326, #34875, #29112, #28909, #35510, #35296, #13172, #15742, #22746, #22114, #9353, #38271, #9137, #32105, #25527, #35085, #3185, #35721, #42111, #3389, #6583, #31888, #6160, #18920, #19137, #2757, #5743, #2969, #12965, #41906, #38491, #38699, #16377, #41687, #38910, #41478, #25309, #5946, #9787, #12754, #25734, #15531, #32520, #29320, #191, #38066, #8925, #2547, #32317, #28694, #12541, #6370, #16172, #7428, #32942, #39963, #39755, #36348, #20403, #14029, #16790, #7640, #17434, #27000, #17000, #10191, #3808, #20614, #20193, #13381, #612, #837, #23385, #29751, #13588, #36563, #3590, #10830, #26572, #1054, #23814, #7220, #13810, #26791, #23162, #39532, #10623, #1264, #10409, #26158, #36780, #33367, #33152, #26361, #4017, #22951, #29963, #4236, #23602, #35919, #17217, #36128, #16584, #30180, #33592, #4453, #19976, #30392, #39110, #9989, #29540, #6786, #19760, #32726, #405, #39312, #6999, #17982, #30959, #34983, #14795, #8824, #15002, #40730, #8195, #15213, #21168, #18817, #27563, #15428, #21797, #5847, #1610, #31577, #34559, #27759, #8397, #38169, #37757, #1815, #18189, #18398, #40944, #21377, #34356, #12009, #34140, #2444, #31158, #18612, #28382, #24794, #31370, #2232, #11586, #5214, #28176, #14590, #2018, #40530, #41369, #34767, #8612, #24581, #27966, #11387, #11799, #37963, #21585, #24372, #5420, #37543, #5000, #41162, #25001, #5636, #12218, #25207, #9030, #22010, #37342, #35400, #35614, #2649, #22845, #38591, #15637, #6050, #19028, #23049, #2863, #39008, #3076, #28798, #38384, #3281, #9246, #6881, #28594, #3482, #9889, #36018, #29208, #16068, #31777, #9456, #16472, #15853, #29010, #31997, #41797, #25837, #19239, #12651, #35814, #29421, #6676, #39205, #291, #25630, #42006, #22423, #12857, #6265, #41581, #38802, #19648, #9675, #32211, #32414, #10085, #22638, #32616, #35184, #6477, #19447, #13274, #16267, #83, #22217, #26257, #12435, #25419, #13063, #26045, #3692, #36448, #7099, #23259, #20283, #502, #7311, #36226, #17097, #10503, #16886, #33249, #4113, #20075, #935, #16680, #30060, #33038, #3904, #13901, #13473, #26883, #29850, #39851, #23485, #716, #19856, #32822, #13688, #29637, #26458, #39413, #10290, #26669, #39629, #12264, #11842, #5046, #34398, #34603, #15048, #24627, #37592, #28221, #37385, #18658, #5258, #34815, #5684, #40993, #5466, #18444, #14838, #8444, #2280, #35027, #21421, #17819, #15472, #25043, #24840, #18025, #18233, #14638, #31203, #12050, #28013, #27605, #37798, #27806, #8242, #2063, #8654, #8867, #11632, #31623, #21626, #21842, #21217, #31413, #15263, #30792, #2488 ),
 ( #1653, #41209, #28426, #38006, #41415, #25249, #38215, #9078, #22054, #34188, #31004, #1858, #40572, #11427, #24418, #40779, #19691, #16518, #13315, #26301, #39246, #25881, #35232, #13105, #22889, #3121, #35855, #32661, #9293, #3524, #16312, #10127, #6093, #29252, #6719, #9720, #6521, #23094, #38843, #16112, #29054, #126, #19489, #32458, #2694, #29467, #3324, #336, #6305, #12695, #22682, #25466, #41843, #15900, #38635, #19282, #32255, #31823, #35658, #28639, #5889, #28844, #15681, #18862, #41626, #42050, #12481, #38430, #22259, #19071, #26090, #32041, #12902, #25675, #39048, #2909, #9502, #22464, #35445, #9932, #36275, #36701, #547, #39463, #36062, #7565, #17562, #16721, #13950, #23954, #29681, #17355, #19905, #26505, #20325, #20539, #10337, #32872, #27132, #26927, #1395, #11182, #39680, #23313, #30104, #20118, #763, #16928, #33730, #39891, #33513, #30317, #10549, #36491, #4377, #13518, #33292, #1186, #6930, #33081, #980, #23531, #7148, #4158, #7353, #3946, #26715, #17141, #29894, #13738, #14369, #14156, #40100, #10967, #4583, #10752, #36920, #3735, #27343, #40316, #7784, #23737, #20759, #30527, #2438, #18183, #34134, #17768, #8818, #27753, #11382, #31152, #8187, #30952, #4995, #21788, #14994, #21579, #5414, #40722, #24572, #34553, #4790, #21371, #31360, #37135, #21162, #2012, #11579, #27557, #34348, #37537, #24364, #14789, #5208, #30740, #37335, #31569, #2226, #15205, #24788, #34761, #40936, #28170, #7986, #15422, #28375, #41156, #14584, #37957, #20959, #41361, #27959, #17975, #1603, #5628, #11792, #1809, #12003, #24993, #37749, #18606, #24165, #40524, #33930, #8392, #8606, #41573, #35605, #13053, #16059, #12845, #19634, #32202, #22413, #35390, #22628, #25829, #38793, #9024, #9881, #9665, #29196, #12639, #19020, #28999, #31770, #6043, #22208, #2854, #25621, #38580, #38162, #41997, #34976, #22836, #35177, #22000, #74, #32608, #6254, #18810, #2642, #28586, #35804, #6468, #15629, #19230, #31988, #19436, #12212, #15844, #28788, #5839, #12427, #25412, #32406, #38374, #9239, #25202, #3270, #6667, #41787, #3066, #26036, #9445, #16257, #38998, #3471, #16462, #29412, #16669, #39196, #33459, #33240, #7731, #17512, #707, #7089, #4104, #19845, #36215, #10279, #33029, #13679, #26659, #26248, #30052, #23039, #40050, #23250, #10073, #30268, #20705, #23476, #6874, #32812, #29627, #10919, #17088, #3683, #36439, #20067, #926, #281, #3894, #16876, #36007, #493, #13462, #13893, #26448, #39404, #13264, #26873, #23903, #29840, #20273, #1139, #39620, #23689, #10491, #7302, #39843, #10705, #36653, #7517, #4322, #20491, #33682, #17304, #14110, #27083, #36871, #4532, #37285, #11330, #28118, #21324, #27911, #11740, #34088, #30903, #40884, #11134, #27701, #24735, #1347, #27507, #24522, #17926, #33880, #40671, #4946, #30689, #21117, #11530, #24115, #17719, #37907, #37700, #21534, #31105, #41103, #5161, #8556, #14320, #21737, #8763, #34502, #20908, #2169, #27299, #34711, #37490, #40475, #37086, #15154, #8345, #1555, #5360, #18338, #34296, #31310, #11952, #4741, #24945, #5576, #30477, #14535, #40264, #7941, #18135, #1959, #24316, #14942, #8140, #1763, #14744, #19178, #32150, #15378, #16205, #3014, #35551, #18551, #28534, #41524, #28325, #18763, #31722, #16005, #25150, #21944, #31519, #28947, #25, #41311, #38532, #6413, #12159, #41944, #2388, #8972, #2806, #12792, #34920, #38115, #9612, #9398, #25986, #35760, #22161, #5790, #12586, #2591, #25360, #12374, #29148, #22360, #25774, #38741, #35130, #18967, #22573, #15575, #15787, #19384, #38318, #9183, #25570, #5993, #31933, #28736, #41731, #35338, #6203, #32357, #3220, #13007, #38951, #9828, #22786, #7254, #4268, #23421, #13843, #32555, #39998, #14062, #30000, #39146, #20438, #3422, #27035, #652, #16618, #230, #33405, #26608, #35957, #26824, #23637, #3845, #36599, #17252, #10028, #30214, #17037, #10864, #6821, #39792, #7464, #10445, #20225, #23852, #39568, #16825, #29788, #10657, #33188, #4052, #16415, #1091, #6619, #19582, #7036, #13413, #36387, #26198, #442, #29577, #39348, #20014, #32979, #29360, #13211, #22989, #32761, #26398, #3631, #10227, #23198, #13625, #36163, #27245, #11077, #5309, #11476, #1295, #17872, #4689, #37438, #30847, #24261, #37030, #1904, #34448, #40831, #2116, #18282, #30636, #21063, #17669, #34039, #1500, #20651, #1708, #27854, #4894, #37231, #8293, #15101, #40420, #24681, #40209, #24064, #7888, #11683, #40618, #27648, #14268, #8498, #31254, #28062, #41044, #11897, #4484, #18080, #27452, #14479, #37643, #20857, #31052, #11278, #21476, #21270, #14690, #14886, #36817, #8086, #7677, #33628, #17466, #24468, #33831, #34241, #30425, #5101, #12101, #41467, #132, #22688, #31670, #2538, #35861, #2331, #26306, #12318, #345, #13323, #6528, #13114, #26097, #21888, #15521, #9939, #554, #28478, #24887, #23101, #32668, #32465, #25093, #25301, #21681, #38850, #19700, #35665, #34654, #3331, #34864, #15318, #9728, #19495, #16526, #18711, #39252, #16318, #29474, #28274, #29260, #39055, #37850, #10134, #22896, #8706, #41255, #38057, #16728, #8916, #3529, #6725, #5735, #31462, #36069, #6936, #5521, #18493, #19913, #32878, #29690, #3742, #39897, #30746, #33300, #40324, #39687, #26936, #13745, #26725, #37141, #4797, #1402, #4384, #10559, #20333, #7994, #7573, #772, #30112, #30324, #10759, #4166, #17147, #23960, #33087, #14377, #989, #30533, #27350, #36709, #1196, #14162, #23539, #13957, #40107, #13524, #23742, #26512, #11188, #20765, #20546, #36498, #33521, #10344, #17363, #7790, #27138, #23321, #10975, #7360, #3954, #36927, #33738, #4590, #17570, #24171, #20965, #33938, #16934, #17775, #39470, #36282, #7156, #20125, #29902, #38864, #9740, #13760, #35678, #29704, #35875, #19508, #29071, #36082, #42066, #39699, #6324, #36295, #567, #26739, #19926, #6740, #22482, #145, #7169, #6542, #19713, #22700, #32478, #16538, #9951, #3343, #13538, #20140, #26525, #29915, #33100, #16330, #32682, #29272, #3544, #13127, #19299, #29488, #39484, #358, #22911, #23114, #786, #26109, #10358, #25898, #39066, #13337, #23334, #26319, #39266, #12920, #3967, #16948, #35464, #32273, #3141, #16131, #3756, #10147, #6951, #32892, #16741, #33951, #17376, #24383, #24185, #20779, #4809, #40542, #1209, #33536, #7804, #4398, #36511, #17582, #1622, #33749, #10988, #11201, #17994, #14176, #11398, #13970, #26949, #10773, #14601, #14389, #1415, #30126, #37352, #21179, #30971, #1828, #14807, #20347, #17787, #27153, #30336, #27575, #39911, #30759, #40119, #8206, #37155, #4603, #34155, #5013, #23976, #27772, #10572, #23552, #27366, #36721, #36942, #7373, #30547, #23757, #40339, #8007, #20977, #33313, #4181, #17164, #1002, #7586, #20561, #15648, #28605, #21809, #28394, #41380, #37768, #31380, #25217, #15865, #5433, #40743, #38395, #18828, #5649, #27977, #2245, #37558, #12020, #34994, #37974, #8411, #18624, #8623, #18202, #18410, #15225, #31789, #34570, #12449, #34779, #2661, #2031, #28187, #2454, #11598, #41592, #41174, #24593, #15013, #40958, #32008, #11810, #25432, #25012, #21596, #5226, #12230, #31170, #21388, #34368, #9257, #22227, #2874, #38179, #8834, #24806, #31588, #35195, #15440, #9044, #22021, #6061, #19040, #16276, #29020, #36028, #26468, #32832, #36236, #39424, #22649, #13072, #42016, #12867, #22854, #29218, #25848, #6891, #10299, #3701, #7109, #23269, #35624, #26057, #9686, #9898, #6487, #12662, #35824, #19865, #6686, #92, #29432, #20084, #32424, #16690, #32221, #3087, #38811, #29646, #32627, #19656, #6274, #510, #33048, #3913, #28811, #41808, #38602, #10095, #19457, #3290, #13482, #16079, #23059, #3491, #25641, #302, #16481, #9467, #22433, #13283, #35411, #19250, #26266, #39214, #726, #13698, #20291, #10513, #26678, #39640, #23494, #36457, #7321, #33257, #16894, #29860, #16264, #2860, #32412, #3277, #38587, #3073, #16066, #11849, #5474, #42003, #32613, #21632, #14844, #13060, #22635, #22420, #2070, #18451, #11639, #28795, #9672, #12647, #24635, #35397, #24848, #34405, #34610, #31994, #6474, #8660, #29204, #9452, #19444, #31210, #15850, #19236, #27813, #80, #41794, #40786, #15055, #28020, #6673, #40999, #35611, #25627, #37805, #21432, #29007, #5265, #37598, #8453, #26043, #39005, #19643, #12852, #6262, #32208, #25834, #9886, #38799, #22842, #35811, #29418, #23908, #39626, #13470, #39202, #30273, #23482, #32819, #10709, #20496, #713, #33465, #17311, #6878, #1145, #13898, #36876, #3689, #26879, #4327, #7308, #4110, #10924, #36445, #13685, #26665, #39848, #17094, #30057, #288, #14114, #931, #27089, #3901, #10286, #20280, #23046, #39410, #26455, #36222, #16883, #29846, #13271, #33245, #26254, #40055, #23256, #10082, #7737, #20711, #10499, #36014, #19852, #16677, #3478, #23695, #29634, #36659, #7096, #7523, #16469, #20073, #33035, #499, #33886, #4746, #34305, #40270, #37091, #33687, #5167, #15160, #14325, #11536, #21540, #27305, #14949, #17517, #24121, #17933, #18141, #7946, #30483, #24741, #24529, #41110, #8770, #37292, #20913, #27707, #17724, #40481, #14540, #31318, #37496, #31111, #27917, #8146, #34093, #1966, #11139, #30910, #40891, #4538, #30694, #40680, #21122, #1562, #1769, #4951, #27513, #24322, #14751, #11335, #8351, #11958, #11746, #37707, #8564, #2177, #21330, #34508, #1352, #24952, #37912, #5366, #18344, #28124, #22368, #29154, #25368, #9618, #25156, #38121, #21951, #25781, #25576, #12593, #41318, #35557, #32363, #31, #13013, #25993, #31525, #3020, #12382, #15582, #12798, #8980, #16012, #28540, #6419, #35345, #31940, #28954, #22582, #38325, #3227, #38958, #19391, #38537, #5797, #41529, #16210, #15795, #34926, #9190, #9404, #18974, #22167, #35136, #32156, #12166, #21742, #5998, #38747, #34716, #2812, #6210, #19184, #18769, #28742, #41950, #5584, #41738, #18556, #2393, #15384, #28332, #31728, #2596, #6626, #23204, #4059, #7042, #19589, #16831, #19800, #29367, #16624, #448, #879, #3637, #23645, #32985, #13849, #13218, #13419, #13631, #22792, #26830, #29584, #35765, #26204, #39152, #1098, #22994, #17043, #36171, #6827, #16421, #23426, #236, #27042, #32562, #36607, #30006, #14069, #7260, #20020, #9834, #26404, #7472, #35965, #3852, #10034, #32770, #29794, #39355, #10234, #39799, #20444, #10664, #17260, #33412, #659, #26615, #39576, #10451, #36393, #3428, #20232, #4277, #33194, #30221, #27254, #5108, #14892, #37239, #27861, #11689, #1302, #24688, #8300, #31261, #40216, #21279, #40837, #1714, #40626, #5315, #17881, #8093, #21071, #34248, #11484, #24476, #36824, #37649, #37445, #8505, #40425, #4696, #14697, #17473, #33837, #7896, #30643, #11284, #24269, #23859, #27655, #20658, #21482, #20865, #7685, #34454, #18288, #34044, #4491, #30433, #14275, #2123, #18087, #11087, #4900, #17677, #31059, #40005, #1508, #14487, #33636, #24071, #37037, #1911, #27459, #30854, #10873, #15107, #9569, #8713, #5945, #15959, #21687, #9352, #11902, #18501, #12324, #41685, #2338, #24895, #19136, #18919, #35509, #3184, #31677, #15325, #22113, #12108, #34874, #8923, #25733, #31886, #25526, #22318, #2545, #28484, #38490, #34661, #25308, #35295, #41050, #25101, #35084, #15529, #31471, #38270, #41476, #28279, #18718, #9136, #5527, #41263, #6368, #6158, #32102, #28693, #38697, #2756, #2968, #37856, #19342, #32316, #28908, #38065, #41905, #21895, #28070, #15739, #5742, #12540, #12753, #22525, #6785, #7218, #9988, #29961, #39311, #20190, #19547, #19759, #19974, #29111, #33150 ) ),
 .UNSPECIFIED., .F., .F., .F. ) 
 B_SPLINE_SURFACE_WITH_KNOTS ( ( 2, 2 ),
 ( 3, 2, 2, 2, 2, 2, 2, 2, 2, 2, 2, 2, 2, 2, 2, 2, 2, 2, 2, 2, 2, 2, 2, 2, 2, 2, 2, 2, 2, 2, 2, 2, 2, 2, 2, 2, 2, 2, 2, 2, 2, 2, 2, 2, 2, 2, 2, 2, 2, 2, 2, 2, 2, 2, 2, 2, 2, 2, 2, 2, 2, 2, 2, 2, 2, 2, 2, 2, 2, 2, 2, 2, 2, 2, 2, 2, 2, 2, 2, 2, 2, 2, 2, 2, 2, 2, 2, 2, 2, 2, 2, 2, 2, 2, 2, 2, 2, 2, 2, 2, 2, 2, 2, 2, 2, 2, 2, 2, 2, 2, 2, 2, 2, 2, 2, 2, 2, 2, 2, 2, 2, 2, 2, 2, 2, 2, 2, 2, 2, 2, 2, 2, 2, 2, 2, 2, 2, 2, 2, 2, 2, 2, 2, 2, 2, 2, 2, 2, 2, 2, 2, 2, 2, 2, 2, 2, 2, 2, 2, 2, 2, 2, 2, 2, 2, 2, 2, 2, 2, 2, 2, 2, 2, 2, 2, 2, 2, 2, 2, 2, 2, 2, 2, 2, 2, 2, 2, 2, 2, 2, 2, 2, 2, 2, 2, 2, 2, 2, 2, 2, 2, 2, 2, 2, 2, 2, 2, 2, 2, 2, 2, 2, 2, 2, 2, 2, 2, 2, 2, 2, 2, 2, 2, 2, 2, 2, 2, 2, 2, 2, 2, 2, 2, 2, 2, 2, 2, 2, 2, 2, 2, 2, 2, 2, 2, 2, 2, 2, 2, 2, 2, 2, 2, 2, 2, 2, 2, 2, 2, 2, 2, 2, 2, 2, 2, 2, 2, 2, 2, 2, 2, 2, 2, 2, 2, 2, 2, 2, 2, 2, 2, 2, 2, 2, 2, 2, 2, 2, 2, 2, 2, 2, 2, 2, 2, 2, 2, 2, 2, 2, 2, 2, 2, 2, 2, 2, 2, 2, 2, 2, 2, 2, 2, 2, 2, 2, 2, 2, 2, 2, 2, 2, 2, 2, 2, 2, 2, 2, 2, 2, 2, 2, 2, 2, 2, 2, 2, 2, 2, 2, 2, 2, 2, 2, 2, 2, 2, 2, 2, 2, 2, 2, 2, 2, 2, 2, 2, 2, 2, 2, 2, 2, 2, 2, 2, 2, 2, 2, 2, 2, 2, 2, 2, 2, 2, 2, 2, 2, 2, 2, 2, 2, 2, 2, 2, 2, 2, 2, 2, 2, 2, 2, 2, 2, 2, 2, 2, 2, 2, 2, 2, 2, 2, 2, 2, 2, 2, 2, 2, 2, 2, 2, 2, 2, 2, 2, 2, 2, 2, 2, 2, 2, 2, 2, 2, 2, 2, 2, 2, 2, 2, 2, 2, 2, 2, 2, 2, 2, 2, 2, 2, 2, 2, 2, 2, 2, 2, 2, 2, 2, 2, 2, 2, 2, 2, 2, 2, 2, 2, 2, 2, 2, 2, 2, 2, 2, 2, 2, 2, 2, 2, 2, 2, 2, 2, 2, 2, 2, 2, 2, 2, 2, 2, 2, 2, 2, 2, 2, 2, 2, 2, 2, 2, 2, 2, 2, 2, 2, 2, 2, 2, 2, 2, 2, 2, 2, 2, 2, 2, 2, 2, 2, 2, 2, 2, 2, 2, 2, 2, 2, 2, 2, 2, 2, 2, 2, 2, 2, 2, 2, 2, 2, 2, 2, 2, 2, 2, 2, 2, 2, 2, 2, 2, 2, 2, 2, 2, 2, 2, 2, 2, 2, 2, 2, 2, 2, 2, 2, 2, 2, 2, 2, 2, 2, 2, 2, 2, 2, 2, 2, 2, 2, 2, 2, 2, 2, 2, 2, 2, 2, 2, 2, 2, 2, 2, 2, 2, 2, 2, 2, 2, 2, 2, 2, 2, 2, 2, 2, 2, 2, 2, 2, 2, 2, 2, 2, 2, 2, 2, 2, 2, 2, 2, 2, 2, 2, 2, 2, 2, 2, 2, 2, 2, 2, 2, 2, 2, 2, 2, 2, 2, 2, 2, 2, 2, 2, 2, 2, 2, 2, 2, 2, 2, 2, 2, 2, 2, 2, 2, 2, 2, 2, 2, 2, 2, 2, 2, 2, 2, 2, 2, 2, 2, 2, 2, 2, 2, 2, 2, 2, 2, 2, 2, 2, 2, 2, 2, 2, 2, 2, 2, 2, 2, 2, 2, 2, 2, 2, 2, 2, 2, 2, 2, 2, 2, 2, 2, 2, 2, 2, 2, 2, 2, 2, 2, 2, 2, 2, 2, 2, 2, 2, 2, 2, 2, 2, 2, 2, 2, 2, 3 ),
 ( 0.000000000000000000, 1.000000000000000000 ),
 ( 0.000000000000000000, 0.001388888888888888942, 0.002777777777777777884, 0.004166666666666666609, 0.005555555555555555768, 0.006944444444444444059, 0.008333333333333333218, 0.009722222222222222376, 0.01111111111111111154, 0.01250000000000000069, 0.01388888888888888812, 0.01527777777777777728, 0.01666666666666666644, 0.01805555555555555386, 0.01944444444444444475, 0.02083333333333333218, 0.02222222222222222307, 0.02361111111111111049, 0.02500000000000000139, 0.02638888888888888881, 0.02777777777777777624, 0.02916666666666666713, 0.03055555555555555455, 0.03194444444444444198, 0.03333333333333333287, 0.03472222222222222376, 0.03611111111111110772, 0.03749999999999999861, 0.03888888888888888951, 0.04027777777777778040, 0.04166666666666666435, 0.04305555555555555525, 0.04444444444444444614, 0.04583333333333333010, 0.04722222222222222099, 0.04861111111111111188, 0.05000000000000000278, 0.05138888888888888673, 0.05277777777777777762, 0.05416666666666666852, 0.05555555555555555247, 0.05694444444444444337, 0.05833333333333333426, 0.05972222222222222515, 0.06111111111111110911, 0.06250000000000000000, 0.06388888888888888395, 0.06527777777777778179, 0.06666666666666666574, 0.06805555555555554970, 0.06944444444444444753, 0.07083333333333333148, 0.07222222222222221544, 0.07361111111111111327, 0.07499999999999999722, 0.07638888888888889506, 0.07777777777777777901, 0.07916666666666666297, 0.08055555555555556080, 0.08194444444444444475, 0.08333333333333332871, 0.08472222222222222654, 0.08611111111111111049, 0.08749999999999999445, 0.08888888888888889228, 0.09027777777777777624, 0.09166666666666666019, 0.09305555555555555802, 0.09444444444444444198, 0.09583333333333333981, 0.09722222222222222376, 0.09861111111111110772, 0.1000000000000000056, 0.1013888888888888895, 0.1027777777777777735, 0.1041666666666666713, 0.1055555555555555552, 0.1069444444444444392, 0.1083333333333333370, 0.1097222222222222210, 0.1111111111111111049, 0.1125000000000000028, 0.1138888888888888867, 0.1152777777777777846, 0.1166666666666666685, 0.1180555555555555525, 0.1194444444444444503, 0.1208333333333333343, 0.1222222222222222182, 0.1236111111111111160, 0.1250000000000000000, 0.1263888888888888840, 0.1277777777777777679, 0.1291666666666666796, 0.1305555555555555636, 0.1319444444444444475, 0.1333333333333333315, 0.1347222222222222154, 0.1361111111111110994, 0.1375000000000000111, 0.1388888888888888951, 0.1402777777777777790, 0.1416666666666666630, 0.1430555555555555469, 0.1444444444444444309, 0.1458333333333333426, 0.1472222222222222265, 0.1486111111111111105, 0.1499999999999999944, 0.1513888888888888784, 0.1527777777777777901, 0.1541666666666666741, 0.1555555555555555580, 0.1569444444444444420, 0.1583333333333333259, 0.1597222222222222099, 0.1611111111111111216, 0.1625000000000000056, 0.1638888888888888895, 0.1652777777777777735, 0.1666666666666666574, 0.1680555555555555691, 0.1694444444444444531, 0.1708333333333333370, 0.1722222222222222210, 0.1736111111111111049, 0.1749999999999999889, 0.1763888888888889006, 0.1777777777777777846, 0.1791666666666666685, 0.1805555555555555525, 0.1819444444444444364, 0.1833333333333333204, 0.1847222222222222321, 0.1861111111111111160, 0.1875000000000000000, 0.1888888888888888840, 0.1902777777777777679, 0.1916666666666666796, 0.1930555555555555636, 0.1944444444444444475, 0.1958333333333333315, 0.1972222222222222154, 0.1986111111111110994, 0.2000000000000000111, 0.2013888888888888951, 0.2027777777777777790, 0.2041666666666666630, 0.2055555555555555469, 0.2069444444444444309, 0.2083333333333333426, 0.2097222222222222265, 0.2111111111111111105, 0.2124999999999999944, 0.2138888888888888784, 0.2152777777777777901, 0.2166666666666666741, 0.2180555555555555580, 0.2194444444444444420, 0.2208333333333333259, 0.2222222222222222099, 0.2236111111111111216, 0.2250000000000000056, 0.2263888888888888895, 0.2277777777777777735, 0.2291666666666666574, 0.2305555555555555691, 0.2319444444444444531, 0.2333333333333333370, 0.2347222222222222210, 0.2361111111111111049, 0.2374999999999999889, 0.2388888888888889006, 0.2402777777777777846, 0.2416666666666666685, 0.2430555555555555525, 0.2444444444444444364, 0.2458333333333333204, 0.2472222222222222321, 0.2486111111111111160, 0.2500000000000000000, 0.2513888888888888840, 0.2527777777777777679, 0.2541666666666666519, 0.2555555555555555358, 0.2569444444444444198, 0.2583333333333333592, 0.2597222222222222432, 0.2611111111111111271, 0.2625000000000000111, 0.2638888888888888951, 0.2652777777777777790, 0.2666666666666666630, 0.2680555555555555469, 0.2694444444444444309, 0.2708333333333333148, 0.2722222222222221988, 0.2736111111111111382, 0.2750000000000000222, 0.2763888888888889062, 0.2777777777777777901, 0.2791666666666666741, 0.2805555555555555580, 0.2819444444444444420, 0.2833333333333333259, 0.2847222222222222099, 0.2861111111111110938, 0.2874999999999999778, 0.2888888888888888618, 0.2902777777777778012, 0.2916666666666666852, 0.2930555555555555691, 0.2944444444444444531, 0.2958333333333333370, 0.2972222222222222210, 0.2986111111111111049, 0.2999999999999999889, 0.3013888888888888729, 0.3027777777777777568, 0.3041666666666666408, 0.3055555555555555802, 0.3069444444444444642, 0.3083333333333333481, 0.3097222222222222321, 0.3111111111111111160, 0.3125000000000000000, 0.3138888888888888840, 0.3152777777777777679, 0.3166666666666666519, 0.3180555555555555358, 0.3194444444444444198, 0.3208333333333333592, 0.3222222222222222432, 0.3236111111111111271, 0.3250000000000000111, 0.3263888888888888951, 0.3277777777777777790, 0.3291666666666666630, 0.3305555555555555469, 0.3319444444444444309, 0.3333333333333333148, 0.3347222222222221988, 0.3361111111111111382, 0.3375000000000000222, 0.3388888888888889062, 0.3402777777777777901, 0.3416666666666666741, 0.3430555555555555580, 0.3444444444444444420, 0.3458333333333333259, 0.3472222222222222099, 0.3486111111111110938, 0.3499999999999999778, 0.3513888888888888618, 0.3527777777777778012, 0.3541666666666666852, 0.3555555555555555691, 0.3569444444444444531, 0.3583333333333333370, 0.3597222222222222210, 0.3611111111111111049, 0.3624999999999999889, 0.3638888888888888729, 0.3652777777777777568, 0.3666666666666666408, 0.3680555555555555802, 0.3694444444444444642, 0.3708333333333333481, 0.3722222222222222321, 0.3736111111111111160, 0.3750000000000000000, 0.3763888888888888840, 0.3777777777777777679, 0.3791666666666666519, 0.3805555555555555358, 0.3819444444444444198, 0.3833333333333333592, 0.3847222222222222432, 0.3861111111111111271, 0.3875000000000000111, 0.3888888888888888951, 0.3902777777777777790, 0.3916666666666666630, 0.3930555555555555469, 0.3944444444444444309, 0.3958333333333333148, 0.3972222222222221988, 0.3986111111111111382, 0.4000000000000000222, 0.4013888888888889062, 0.4027777777777777901, 0.4041666666666666741, 0.4055555555555555580, 0.4069444444444444420, 0.4083333333333333259, 0.4097222222222222099, 0.4111111111111110938, 0.4124999999999999778, 0.4138888888888888618, 0.4152777777777778012, 0.4166666666666666852, 0.4180555555555555691, 0.4194444444444444531, 0.4208333333333333370, 0.4222222222222222210, 0.4236111111111111049, 0.4249999999999999889, 0.4263888888888888729, 0.4277777777777777568, 0.4291666666666666408, 0.4305555555555555802, 0.4319444444444444642, 0.4333333333333333481, 0.4347222222222222321, 0.4361111111111111160, 0.4375000000000000000, 0.4388888888888888840, 0.4402777777777777679, 0.4416666666666666519, 0.4430555555555555358, 0.4444444444444444198, 0.4458333333333333592, 0.4472222222222222432, 0.4486111111111111271, 0.4500000000000000111, 0.4513888888888888951, 0.4527777777777777790, 0.4541666666666666630, 0.4555555555555555469, 0.4569444444444444309, 0.4583333333333333148, 0.4597222222222221988, 0.4611111111111111382, 0.4625000000000000222, 0.4638888888888889062, 0.4652777777777777901, 0.4666666666666666741, 0.4680555555555555580, 0.4694444444444444420, 0.4708333333333333259, 0.4722222222222222099, 0.4736111111111110938, 0.4749999999999999778, 0.4763888888888888618, 0.4777777777777778012, 0.4791666666666666852, 0.4805555555555555691, 0.4819444444444444531, 0.4833333333333333370, 0.4847222222222222210, 0.4861111111111111049, 0.4874999999999999889, 0.4888888888888888729, 0.4902777777777777568, 0.4916666666666666408, 0.4930555555555555802, 0.4944444444444444642, 0.4958333333333333481, 0.4972222222222222321, 0.4986111111111111160, 0.5000000000000000000, 0.5013888888888888840, 0.5027777777777777679, 0.5041666666666666519, 0.5055555555555555358, 0.5069444444444444198, 0.5083333333333333037, 0.5097222222222221877, 0.5111111111111110716, 0.5124999999999999556, 0.5138888888888888395, 0.5152777777777777235, 0.5166666666666667185, 0.5180555555555556024, 0.5194444444444444864, 0.5208333333333333703, 0.5222222222222222543, 0.5236111111111111382, 0.5250000000000000222, 0.5263888888888889062, 0.5277777777777777901, 0.5291666666666666741, 0.5305555555555555580, 0.5319444444444444420, 0.5333333333333333259, 0.5347222222222222099, 0.5361111111111110938, 0.5374999999999999778, 0.5388888888888888618, 0.5402777777777777457, 0.5416666666666666297, 0.5430555555555555136, 0.5444444444444443976, 0.5458333333333332815, 0.5472222222222222765, 0.5486111111111111605, 0.5500000000000000444, 0.5513888888888889284, 0.5527777777777778123, 0.5541666666666666963, 0.5555555555555555802, 0.5569444444444444642, 0.5583333333333333481, 0.5597222222222222321, 0.5611111111111111160, 0.5625000000000000000, 0.5638888888888888840, 0.5652777777777777679, 0.5666666666666666519, 0.5680555555555555358, 0.5694444444444444198, 0.5708333333333333037, 0.5722222222222221877, 0.5736111111111110716, 0.5749999999999999556, 0.5763888888888888395, 0.5777777777777777235, 0.5791666666666667185, 0.5805555555555556024, 0.5819444444444444864, 0.5833333333333333703, 0.5847222222222222543, 0.5861111111111111382, 0.5875000000000000222, 0.5888888888888889062, 0.5902777777777777901, 0.5916666666666666741, 0.5930555555555555580, 0.5944444444444444420, 0.5958333333333333259, 0.5972222222222222099, 0.5986111111111110938, 0.5999999999999999778, 0.6013888888888888618, 0.6027777777777777457, 0.6041666666666666297, 0.6055555555555555136, 0.6069444444444443976, 0.6083333333333332815, 0.6097222222222222765, 0.6111111111111111605, 0.6125000000000000444, 0.6138888888888889284, 0.6152777777777778123, 0.6166666666666666963, 0.6180555555555555802, 0.6194444444444444642, 0.6208333333333333481, 0.6222222222222222321, 0.6236111111111111160, 0.6250000000000000000, 0.6263888888888888840, 0.6277777777777777679, 0.6291666666666666519, 0.6305555555555555358, 0.6319444444444444198, 0.6333333333333333037, 0.6347222222222221877, 0.6361111111111110716, 0.6374999999999999556, 0.6388888888888888395, 0.6402777777777777235, 0.6416666666666667185, 0.6430555555555556024, 0.6444444444444444864, 0.6458333333333333703, 0.6472222222222222543, 0.6486111111111111382, 0.6500000000000000222, 0.6513888888888889062, 0.6527777777777777901, 0.6541666666666666741, 0.6555555555555555580, 0.6569444444444444420, 0.6583333333333333259, 0.6597222222222222099, 0.6611111111111110938, 0.6624999999999999778, 0.6638888888888888618, 0.6652777777777777457, 0.6666666666666666297, 0.6680555555555555136, 0.6694444444444443976, 0.6708333333333332815, 0.6722222222222222765, 0.6736111111111111605, 0.6750000000000000444, 0.6763888888888889284, 0.6777777777777778123, 0.6791666666666666963, 0.6805555555555555802, 0.6819444444444444642, 0.6833333333333333481, 0.6847222222222222321, 0.6861111111111111160, 0.6875000000000000000, 0.6888888888888888840, 0.6902777777777777679, 0.6916666666666666519, 0.6930555555555555358, 0.6944444444444444198, 0.6958333333333333037, 0.6972222222222221877, 0.6986111111111110716, 0.6999999999999999556, 0.7013888888888888395, 0.7027777777777777235, 0.7041666666666667185, 0.7055555555555556024, 0.7069444444444444864, 0.7083333333333333703, 0.7097222222222222543, 0.7111111111111111382, 0.7125000000000000222, 0.7138888888888889062, 0.7152777777777777901, 0.7166666666666666741, 0.7180555555555555580, 0.7194444444444444420, 0.7208333333333333259, 0.7222222222222222099, 0.7236111111111110938, 0.7249999999999999778, 0.7263888888888888618, 0.7277777777777777457, 0.7291666666666666297, 0.7305555555555555136, 0.7319444444444443976, 0.7333333333333332815, 0.7347222222222222765, 0.7361111111111111605, 0.7375000000000000444, 0.7388888888888889284, 0.7402777777777778123, 0.7416666666666666963, 0.7430555555555555802, 0.7444444444444444642, 0.7458333333333333481, 0.7472222222222222321, 0.7486111111111111160, 0.7500000000000000000, 0.7513888888888888840, 0.7527777777777777679, 0.7541666666666666519, 0.7555555555555555358, 0.7569444444444444198, 0.7583333333333333037, 0.7597222222222221877, 0.7611111111111110716, 0.7624999999999999556, 0.7638888888888888395, 0.7652777777777777235, 0.7666666666666667185, 0.7680555555555556024, 0.7694444444444444864, 0.7708333333333333703, 0.7722222222222222543, 0.7736111111111111382, 0.7750000000000000222, 0.7763888888888889062, 0.7777777777777777901, 0.7791666666666666741, 0.7805555555555555580, 0.7819444444444444420, 0.7833333333333333259, 0.7847222222222222099, 0.7861111111111110938, 0.7874999999999999778, 0.7888888888888888618, 0.7902777777777777457, 0.7916666666666666297, 0.7930555555555555136, 0.7944444444444443976, 0.7958333333333332815, 0.7972222222222222765, 0.7986111111111111605, 0.8000000000000000444, 0.8013888888888889284, 0.8027777777777778123, 0.8041666666666666963, 0.8055555555555555802, 0.8069444444444444642, 0.8083333333333333481, 0.8097222222222222321, 0.8111111111111111160, 0.8125000000000000000, 0.8138888888888888840, 0.8152777777777777679, 0.8166666666666666519, 0.8180555555555555358, 0.8194444444444444198, 0.8208333333333333037, 0.8222222222222221877, 0.8236111111111110716, 0.8249999999999999556, 0.8263888888888888395, 0.8277777777777777235, 0.8291666666666667185, 0.8305555555555556024, 0.8319444444444444864, 0.8333333333333333703, 0.8347222222222222543, 0.8361111111111111382, 0.8375000000000000222, 0.8388888888888889062, 0.8402777777777777901, 0.8416666666666666741, 0.8430555555555555580, 0.8444444444444444420, 0.8458333333333333259, 0.8472222222222222099, 0.8486111111111110938, 0.8499999999999999778, 0.8513888888888888618, 0.8527777777777777457, 0.8541666666666666297, 0.8555555555555555136, 0.8569444444444443976, 0.8583333333333332815, 0.8597222222222222765, 0.8611111111111111605, 0.8625000000000000444, 0.8638888888888889284, 0.8652777777777778123, 0.8666666666666666963, 0.8680555555555555802, 0.8694444444444444642, 0.8708333333333333481, 0.8722222222222222321, 0.8736111111111111160, 0.8750000000000000000, 0.8763888888888888840, 0.8777777777777777679, 0.8791666666666666519, 0.8805555555555555358, 0.8819444444444444198, 0.8833333333333333037, 0.8847222222222221877, 0.8861111111111110716, 0.8874999999999999556, 0.8888888888888888395, 0.8902777777777777235, 0.8916666666666667185, 0.8930555555555556024, 0.8944444444444444864, 0.8958333333333333703, 0.8972222222222222543, 0.8986111111111111382, 0.9000000000000000222, 0.9013888888888889062, 0.9027777777777777901, 0.9041666666666666741, 0.9055555555555555580, 0.9069444444444444420, 0.9083333333333333259, 0.9097222222222222099, 0.9111111111111110938, 0.9124999999999999778, 0.9138888888888888618, 0.9152777777777777457, 0.9166666666666666297, 0.9180555555555555136, 0.9194444444444443976, 0.9208333333333332815, 0.9222222222222222765, 0.9236111111111111605, 0.9250000000000000444, 0.9263888888888889284, 0.9277777777777778123, 0.9291666666666666963, 0.9305555555555555802, 0.9319444444444444642, 0.9333333333333333481, 0.9347222222222222321, 0.9361111111111111160, 0.9375000000000000000, 0.9388888888888888840, 0.9402777777777777679, 0.9416666666666666519, 0.9430555555555555358, 0.9444444444444444198, 0.9458333333333333037, 0.9472222222222221877, 0.9486111111111110716, 0.9499999999999999556, 0.9513888888888888395, 0.9527777777777777235, 0.9541666666666667185, 0.9555555555555556024, 0.9569444444444444864, 0.9583333333333333703, 0.9597222222222222543, 0.9611111111111111382, 0.9625000000000000222, 0.9638888888888889062, 0.9652777777777777901, 0.9666666666666666741, 0.9680555555555555580, 0.9694444444444444420, 0.9708333333333333259, 0.9722222222222222099, 0.9736111111111110938, 0.9749999999999999778, 0.9763888888888888618, 0.9777777777777777457, 0.9791666666666666297, 0.9805555555555555136, 0.9819444444444443976, 0.9833333333333332815, 0.9847222222222222765, 0.9861111111111111605, 0.9875000000000000444, 0.9888888888888889284, 0.9902777777777778123, 0.9916666666666666963, 0.9930555555555555802, 0.9944444444444444642, 0.9958333333333333481, 0.9972222222222222321, 0.9986111111111111160, 1.000000000000000000 ),
 .UNSPECIFIED. ) 
 GEOMETRIC_REPRESENTATION_ITEM ( )  RATIONAL_B_SPLINE_SURFACE ( (
 ( 1.000000000000000000, 0.8660254037844387076, 1.000000000000000000, 0.8660254037844387076, 1.000000000000000000, 0.8660254037844387076, 1.000000000000000000, 0.8660254037844387076, 1.000000000000000000, 0.8660254037844387076, 1.000000000000000000, 0.8660254037844387076, 1.000000000000000000, 0.8660254037844387076, 1.000000000000000000, 0.8660254037844387076, 1.000000000000000000, 0.8660254037844387076, 1.000000000000000000, 0.8660254037844387076, 1.000000000000000000, 0.8660254037844387076, 1.000000000000000000, 0.8660254037844387076, 1.000000000000000000, 0.8660254037844387076, 1.000000000000000000, 0.8660254037844387076, 1.000000000000000000, 0.8660254037844387076, 1.000000000000000000, 0.8660254037844387076, 1.000000000000000000, 0.8660254037844387076, 1.000000000000000000, 0.8660254037844387076, 1.000000000000000000, 0.8660254037844387076, 1.000000000000000000, 0.8660254037844387076, 1.000000000000000000, 0.8660254037844387076, 1.000000000000000000, 0.8660254037844387076, 1.000000000000000000, 0.8660254037844387076, 1.000000000000000000, 0.8660254037844387076, 1.000000000000000000, 0.8660254037844387076, 1.000000000000000000, 0.8660254037844387076, 1.000000000000000000, 0.8660254037844387076, 1.000000000000000000, 0.8660254037844387076, 1.000000000000000000, 0.8660254037844387076, 1.000000000000000000, 0.8660254037844387076, 1.000000000000000000, 0.8660254037844387076, 1.000000000000000000, 0.8660254037844387076, 1.000000000000000000, 0.8660254037844387076, 1.000000000000000000, 0.8660254037844387076, 1.000000000000000000, 0.8660254037844387076, 1.000000000000000000, 0.8660254037844387076, 1.000000000000000000, 0.8660254037844387076, 1.000000000000000000, 0.8660254037844387076, 1.000000000000000000, 0.8660254037844387076, 1.000000000000000000, 0.8660254037844387076, 1.000000000000000000, 0.8660254037844387076, 1.000000000000000000, 0.8660254037844387076, 1.000000000000000000, 0.8660254037844387076, 1.000000000000000000, 0.8660254037844387076, 1.000000000000000000, 0.8660254037844387076, 1.000000000000000000, 0.8660254037844387076, 1.000000000000000000, 0.8660254037844387076, 1.000000000000000000, 0.8660254037844387076, 1.000000000000000000, 0.8660254037844387076, 1.000000000000000000, 0.8660254037844387076, 1.000000000000000000, 0.8660254037844387076, 1.000000000000000000, 0.8660254037844387076, 1.000000000000000000, 0.8660254037844387076, 1.000000000000000000, 0.8660254037844387076, 1.000000000000000000, 0.8660254037844387076, 1.000000000000000000, 0.8660254037844387076, 1.000000000000000000, 0.8660254037844387076, 1.000000000000000000, 0.8660254037844387076, 1.000000000000000000, 0.8660254037844387076, 1.000000000000000000, 0.8660254037844387076, 1.000000000000000000, 0.8660254037844387076, 1.000000000000000000, 0.8660254037844387076, 1.000000000000000000, 0.8660254037844387076, 1.000000000000000000, 0.8660254037844387076, 1.000000000000000000, 0.8660254037844387076, 1.000000000000000000, 0.8660254037844387076, 1.000000000000000000, 0.8660254037844387076, 1.000000000000000000, 0.8660254037844387076, 1.000000000000000000, 0.8660254037844387076, 1.000000000000000000, 0.8660254037844387076, 1.000000000000000000, 0.8660254037844387076, 1.000000000000000000, 0.8660254037844387076, 1.000000000000000000, 0.8660254037844387076, 1.000000000000000000, 0.8660254037844387076, 1.000000000000000000, 0.8660254037844387076, 1.000000000000000000, 0.8660254037844387076, 1.000000000000000000, 0.8660254037844387076, 1.000000000000000000, 0.8660254037844387076, 1.000000000000000000, 0.8660254037844387076, 1.000000000000000000, 0.8660254037844387076, 1.000000000000000000, 0.8660254037844387076, 1.000000000000000000, 0.8660254037844387076, 1.000000000000000000, 0.8660254037844387076, 1.000000000000000000, 0.8660254037844387076, 1.000000000000000000, 0.8660254037844387076, 1.000000000000000000, 0.8660254037844387076, 1.000000000000000000, 0.8660254037844387076, 1.000000000000000000, 0.8660254037844387076, 1.000000000000000000, 0.8660254037844387076, 1.000000000000000000, 0.8660254037844387076, 1.000000000000000000, 0.8660254037844387076, 1.000000000000000000, 0.8660254037844387076, 1.000000000000000000, 0.8660254037844387076, 1.000000000000000000, 0.8660254037844387076, 1.000000000000000000, 0.8660254037844387076, 1.000000000000000000, 0.8660254037844387076, 1.000000000000000000, 0.8660254037844387076, 1.000000000000000000, 0.8660254037844387076, 1.000000000000000000, 0.8660254037844387076, 1.000000000000000000, 0.8660254037844387076, 1.000000000000000000, 0.8660254037844387076, 1.000000000000000000, 0.8660254037844387076, 1.000000000000000000, 0.8660254037844387076, 1.000000000000000000, 0.8660254037844387076, 1.000000000000000000, 0.8660254037844387076, 1.000000000000000000, 0.8660254037844387076, 1.000000000000000000, 0.8660254037844387076, 1.000000000000000000, 0.8660254037844387076, 1.000000000000000000, 0.8660254037844387076, 1.000000000000000000, 0.8660254037844387076, 1.000000000000000000, 0.8660254037844387076, 1.000000000000000000, 0.8660254037844387076, 1.000000000000000000, 0.8660254037844387076, 1.000000000000000000, 0.8660254037844387076, 1.000000000000000000, 0.8660254037844387076, 1.000000000000000000, 0.8660254037844387076, 1.000000000000000000, 0.8660254037844387076, 1.000000000000000000, 0.8660254037844387076, 1.000000000000000000, 0.8660254037844387076, 1.000000000000000000, 0.8660254037844387076, 1.000000000000000000, 0.8660254037844387076, 1.000000000000000000, 0.8660254037844387076, 1.000000000000000000, 0.8660254037844387076, 1.000000000000000000, 0.8660254037844387076, 1.000000000000000000, 0.8660254037844387076, 1.000000000000000000, 0.8660254037844387076, 1.000000000000000000, 0.8660254037844387076, 1.000000000000000000, 0.8660254037844387076, 1.000000000000000000, 0.8660254037844387076, 1.000000000000000000, 0.8660254037844387076, 1.000000000000000000, 0.8660254037844387076, 1.000000000000000000, 0.8660254037844387076, 1.000000000000000000, 0.8660254037844387076, 1.000000000000000000, 0.8660254037844387076, 1.000000000000000000, 0.8660254037844387076, 1.000000000000000000, 0.8660254037844387076, 1.000000000000000000, 0.8660254037844387076, 1.000000000000000000, 0.8660254037844387076, 1.000000000000000000, 0.8660254037844387076, 1.000000000000000000, 0.8660254037844387076, 1.000000000000000000, 0.8660254037844387076, 1.000000000000000000, 0.8660254037844387076, 1.000000000000000000, 0.8660254037844387076, 1.000000000000000000, 0.8660254037844387076, 1.000000000000000000, 0.8660254037844387076, 1.000000000000000000, 0.8660254037844387076, 1.000000000000000000, 0.8660254037844387076, 1.000000000000000000, 0.8660254037844387076, 1.000000000000000000, 0.8660254037844387076, 1.000000000000000000, 0.8660254037844387076, 1.000000000000000000, 0.8660254037844387076, 1.000000000000000000, 0.8660254037844387076, 1.000000000000000000, 0.8660254037844387076, 1.000000000000000000, 0.8660254037844387076, 1.000000000000000000, 0.8660254037844387076, 1.000000000000000000, 0.8660254037844387076, 1.000000000000000000, 0.8660254037844387076, 1.000000000000000000, 0.8660254037844387076, 1.000000000000000000, 0.8660254037844387076, 1.000000000000000000, 0.8660254037844387076, 1.000000000000000000, 0.8660254037844387076, 1.000000000000000000, 0.8660254037844387076, 1.000000000000000000, 0.8660254037844387076, 1.000000000000000000, 0.8660254037844387076, 1.000000000000000000, 0.8660254037844387076, 1.000000000000000000, 0.8660254037844387076, 1.000000000000000000, 0.8660254037844387076, 1.000000000000000000, 0.8660254037844387076, 1.000000000000000000, 0.8660254037844387076, 1.000000000000000000, 0.8660254037844387076, 1.000000000000000000, 0.8660254037844387076, 1.000000000000000000, 0.8660254037844387076, 1.000000000000000000, 0.8660254037844387076, 1.000000000000000000, 0.8660254037844387076, 1.000000000000000000, 0.8660254037844387076, 1.000000000000000000, 0.8660254037844387076, 1.000000000000000000, 0.8660254037844387076, 1.000000000000000000, 0.8660254037844387076, 1.000000000000000000, 0.8660254037844387076, 1.000000000000000000, 0.8660254037844387076, 1.000000000000000000, 0.8660254037844387076, 1.000000000000000000, 0.8660254037844387076, 1.000000000000000000, 0.8660254037844387076, 1.000000000000000000, 0.8660254037844387076, 1.000000000000000000, 0.8660254037844387076, 1.000000000000000000, 0.8660254037844387076, 1.000000000000000000, 0.8660254037844387076, 1.000000000000000000, 0.8660254037844387076, 1.000000000000000000, 0.8660254037844387076, 1.000000000000000000, 0.8660254037844387076, 1.000000000000000000, 0.8660254037844387076, 1.000000000000000000, 0.8660254037844387076, 1.000000000000000000, 0.8660254037844387076, 1.000000000000000000, 0.8660254037844387076, 1.000000000000000000, 0.8660254037844387076, 1.000000000000000000, 0.8660254037844387076, 1.000000000000000000, 0.8660254037844387076, 1.000000000000000000, 0.8660254037844387076, 1.000000000000000000, 0.8660254037844387076, 1.000000000000000000, 0.8660254037844387076, 1.000000000000000000, 0.8660254037844387076, 1.000000000000000000, 0.8660254037844387076, 1.000000000000000000, 0.8660254037844387076, 1.000000000000000000, 0.8660254037844387076, 1.000000000000000000, 0.8660254037844387076, 1.000000000000000000, 0.8660254037844387076, 1.000000000000000000, 0.8660254037844387076, 1.000000000000000000, 0.8660254037844387076, 1.000000000000000000, 0.8660254037844387076, 1.000000000000000000, 0.8660254037844387076, 1.000000000000000000, 0.8660254037844387076, 1.000000000000000000, 0.8660254037844387076, 1.000000000000000000, 0.8660254037844387076, 1.000000000000000000, 0.8660254037844387076, 1.000000000000000000, 0.8660254037844387076, 1.000000000000000000, 0.8660254037844387076, 1.000000000000000000, 0.8660254037844387076, 1.000000000000000000, 0.8660254037844387076, 1.000000000000000000, 0.8660254037844387076, 1.000000000000000000, 0.8660254037844387076, 1.000000000000000000, 0.8660254037844387076, 1.000000000000000000, 0.8660254037844387076, 1.000000000000000000, 0.8660254037844387076, 1.000000000000000000, 0.8660254037844387076, 1.000000000000000000, 0.8660254037844387076, 1.000000000000000000, 0.8660254037844387076, 1.000000000000000000, 0.8660254037844387076, 1.000000000000000000, 0.8660254037844387076, 1.000000000000000000, 0.8660254037844387076, 1.000000000000000000, 0.8660254037844387076, 1.000000000000000000, 0.8660254037844387076, 1.000000000000000000, 0.8660254037844387076, 1.000000000000000000, 0.8660254037844387076, 1.000000000000000000, 0.8660254037844387076, 1.000000000000000000, 0.8660254037844387076, 1.000000000000000000, 0.8660254037844387076, 1.000000000000000000, 0.8660254037844387076, 1.000000000000000000, 0.8660254037844387076, 1.000000000000000000, 0.8660254037844387076, 1.000000000000000000, 0.8660254037844387076, 1.000000000000000000, 0.8660254037844387076, 1.000000000000000000, 0.8660254037844387076, 1.000000000000000000, 0.8660254037844387076, 1.000000000000000000, 0.8660254037844387076, 1.000000000000000000, 0.8660254037844387076, 1.000000000000000000, 0.8660254037844387076, 1.000000000000000000, 0.8660254037844387076, 1.000000000000000000, 0.8660254037844387076, 1.000000000000000000, 0.8660254037844387076, 1.000000000000000000, 0.8660254037844387076, 1.000000000000000000, 0.8660254037844387076, 1.000000000000000000, 0.8660254037844387076, 1.000000000000000000, 0.8660254037844387076, 1.000000000000000000, 0.8660254037844387076, 1.000000000000000000, 0.8660254037844387076, 1.000000000000000000, 0.8660254037844387076, 1.000000000000000000, 0.8660254037844387076, 1.000000000000000000, 0.8660254037844387076, 1.000000000000000000, 0.8660254037844387076, 1.000000000000000000, 0.8660254037844387076, 1.000000000000000000, 0.8660254037844387076, 1.000000000000000000, 0.8660254037844387076, 1.000000000000000000, 0.8660254037844387076, 1.000000000000000000, 0.8660254037844387076, 1.000000000000000000, 0.8660254037844387076, 1.000000000000000000, 0.8660254037844387076, 1.000000000000000000, 0.8660254037844387076, 1.000000000000000000, 0.8660254037844387076, 1.000000000000000000, 0.8660254037844387076, 1.000000000000000000, 0.8660254037844387076, 1.000000000000000000, 0.8660254037844387076, 1.000000000000000000, 0.8660254037844387076, 1.000000000000000000, 0.8660254037844387076, 1.000000000000000000, 0.8660254037844387076, 1.000000000000000000, 0.8660254037844387076, 1.000000000000000000, 0.8660254037844387076, 1.000000000000000000, 0.8660254037844387076, 1.000000000000000000, 0.8660254037844387076, 1.000000000000000000, 0.8660254037844387076, 1.000000000000000000, 0.8660254037844387076, 1.000000000000000000, 0.8660254037844387076, 1.000000000000000000, 0.8660254037844387076, 1.000000000000000000, 0.8660254037844387076, 1.000000000000000000, 0.8660254037844387076, 1.000000000000000000, 0.8660254037844387076, 1.000000000000000000, 0.8660254037844387076, 1.000000000000000000, 0.8660254037844387076, 1.000000000000000000, 0.8660254037844387076, 1.000000000000000000, 0.8660254037844387076, 1.000000000000000000, 0.8660254037844387076, 1.000000000000000000, 0.8660254037844387076, 1.000000000000000000, 0.8660254037844387076, 1.000000000000000000, 0.8660254037844387076, 1.000000000000000000, 0.8660254037844387076, 1.000000000000000000, 0.8660254037844387076, 1.000000000000000000, 0.8660254037844387076, 1.000000000000000000, 0.8660254037844387076, 1.000000000000000000, 0.8660254037844387076, 1.000000000000000000, 0.8660254037844387076, 1.000000000000000000, 0.8660254037844387076, 1.000000000000000000, 0.8660254037844387076, 1.000000000000000000, 0.8660254037844387076, 1.000000000000000000, 0.8660254037844387076, 1.000000000000000000, 0.8660254037844387076, 1.000000000000000000, 0.8660254037844387076, 1.000000000000000000, 0.8660254037844387076, 1.000000000000000000, 0.8660254037844387076, 1.000000000000000000, 0.8660254037844387076, 1.000000000000000000, 0.8660254037844387076, 1.000000000000000000, 0.8660254037844387076, 1.000000000000000000, 0.8660254037844387076, 1.000000000000000000, 0.8660254037844387076, 1.000000000000000000, 0.8660254037844387076, 1.000000000000000000, 0.8660254037844387076, 1.000000000000000000, 0.8660254037844387076, 1.000000000000000000, 0.8660254037844387076, 1.000000000000000000, 0.8660254037844387076, 1.000000000000000000, 0.8660254037844387076, 1.000000000000000000, 0.8660254037844387076, 1.000000000000000000, 0.8660254037844387076, 1.000000000000000000, 0.8660254037844387076, 1.000000000000000000, 0.8660254037844387076, 1.000000000000000000, 0.8660254037844387076, 1.000000000000000000, 0.8660254037844387076, 1.000000000000000000, 0.8660254037844387076, 1.000000000000000000, 0.8660254037844387076, 1.000000000000000000, 0.8660254037844387076, 1.000000000000000000, 0.8660254037844387076, 1.000000000000000000, 0.8660254037844387076, 1.000000000000000000, 0.8660254037844387076, 1.000000000000000000, 0.8660254037844387076, 1.000000000000000000, 0.8660254037844387076, 1.000000000000000000, 0.8660254037844387076, 1.000000000000000000, 0.8660254037844387076, 1.000000000000000000, 0.8660254037844387076, 1.000000000000000000, 0.8660254037844387076, 1.000000000000000000, 0.8660254037844387076, 1.000000000000000000, 0.8660254037844387076, 1.000000000000000000, 0.8660254037844387076, 1.000000000000000000, 0.8660254037844387076, 1.000000000000000000, 0.8660254037844387076, 1.000000000000000000, 0.8660254037844387076, 1.000000000000000000, 0.8660254037844387076, 1.000000000000000000, 0.8660254037844387076, 1.000000000000000000, 0.8660254037844387076, 1.000000000000000000, 0.8660254037844387076, 1.000000000000000000, 0.8660254037844387076, 1.000000000000000000, 0.8660254037844387076, 1.000000000000000000, 0.8660254037844387076, 1.000000000000000000, 0.8660254037844387076, 1.000000000000000000, 0.8660254037844387076, 1.000000000000000000, 0.8660254037844387076, 1.000000000000000000, 0.8660254037844387076, 1.000000000000000000, 0.8660254037844387076, 1.000000000000000000, 0.8660254037844387076, 1.000000000000000000, 0.8660254037844387076, 1.000000000000000000, 0.8660254037844387076, 1.000000000000000000, 0.8660254037844387076, 1.000000000000000000, 0.8660254037844387076, 1.000000000000000000, 0.8660254037844387076, 1.000000000000000000, 0.8660254037844387076, 1.000000000000000000, 0.8660254037844387076, 1.000000000000000000, 0.8660254037844387076, 1.000000000000000000, 0.8660254037844387076, 1.000000000000000000, 0.8660254037844387076, 1.000000000000000000, 0.8660254037844387076, 1.000000000000000000, 0.8660254037844387076, 1.000000000000000000, 0.8660254037844387076, 1.000000000000000000, 0.8660254037844387076, 1.000000000000000000, 0.8660254037844387076, 1.000000000000000000, 0.8660254037844387076, 1.000000000000000000, 0.8660254037844387076, 1.000000000000000000, 0.8660254037844387076, 1.000000000000000000, 0.8660254037844387076, 1.000000000000000000, 0.8660254037844387076, 1.000000000000000000, 0.8660254037844387076, 1.000000000000000000, 0.8660254037844387076, 1.000000000000000000, 0.8660254037844387076, 1.000000000000000000, 0.8660254037844387076, 1.000000000000000000, 0.8660254037844387076, 1.000000000000000000, 0.8660254037844387076, 1.000000000000000000, 0.8660254037844387076, 1.000000000000000000, 0.8660254037844387076, 1.000000000000000000, 0.8660254037844387076, 1.000000000000000000, 0.8660254037844387076, 1.000000000000000000, 0.8660254037844387076, 1.000000000000000000, 0.8660254037844387076, 1.000000000000000000, 0.8660254037844387076, 1.000000000000000000, 0.8660254037844387076, 1.000000000000000000, 0.8660254037844387076, 1.000000000000000000, 0.8660254037844387076, 1.000000000000000000, 0.8660254037844387076, 1.000000000000000000, 0.8660254037844387076, 1.000000000000000000, 0.8660254037844387076, 1.000000000000000000, 0.8660254037844387076, 1.000000000000000000, 0.8660254037844387076, 1.000000000000000000, 0.8660254037844387076, 1.000000000000000000, 0.8660254037844387076, 1.000000000000000000, 0.8660254037844387076, 1.000000000000000000, 0.8660254037844387076, 1.000000000000000000, 0.8660254037844387076, 1.000000000000000000, 0.8660254037844387076, 1.000000000000000000, 0.8660254037844387076, 1.000000000000000000, 0.8660254037844387076, 1.000000000000000000, 0.8660254037844387076, 1.000000000000000000, 0.8660254037844387076, 1.000000000000000000, 0.8660254037844387076, 1.000000000000000000, 0.8660254037844387076, 1.000000000000000000, 0.8660254037844387076, 1.000000000000000000, 0.8660254037844387076, 1.000000000000000000, 0.8660254037844387076, 1.000000000000000000, 0.8660254037844387076, 1.000000000000000000, 0.8660254037844387076, 1.000000000000000000, 0.8660254037844387076, 1.000000000000000000, 0.8660254037844387076, 1.000000000000000000, 0.8660254037844387076, 1.000000000000000000, 0.8660254037844387076, 1.000000000000000000, 0.8660254037844387076, 1.000000000000000000, 0.8660254037844387076, 1.000000000000000000, 0.8660254037844387076, 1.000000000000000000, 0.8660254037844387076, 1.000000000000000000, 0.8660254037844387076, 1.000000000000000000, 0.8660254037844387076, 1.000000000000000000, 0.8660254037844387076, 1.000000000000000000, 0.8660254037844387076, 1.000000000000000000, 0.8660254037844387076, 1.000000000000000000, 0.8660254037844387076, 1.000000000000000000, 0.8660254037844387076, 1.000000000000000000, 0.8660254037844387076, 1.000000000000000000, 0.8660254037844387076, 1.000000000000000000, 0.8660254037844387076, 1.000000000000000000, 0.8660254037844387076, 1.000000000000000000, 0.8660254037844387076, 1.000000000000000000, 0.8660254037844387076, 1.000000000000000000, 0.8660254037844387076, 1.000000000000000000, 0.8660254037844387076, 1.000000000000000000, 0.8660254037844387076, 1.000000000000000000, 0.8660254037844387076, 1.000000000000000000, 0.8660254037844387076, 1.000000000000000000, 0.8660254037844387076, 1.000000000000000000, 0.8660254037844387076, 1.000000000000000000, 0.8660254037844387076, 1.000000000000000000, 0.8660254037844387076, 1.000000000000000000, 0.8660254037844387076, 1.000000000000000000, 0.8660254037844387076, 1.000000000000000000, 0.8660254037844387076, 1.000000000000000000, 0.8660254037844387076, 1.000000000000000000, 0.8660254037844387076, 1.000000000000000000, 0.8660254037844387076, 1.000000000000000000, 0.8660254037844387076, 1.000000000000000000, 0.8660254037844387076, 1.000000000000000000, 0.8660254037844387076, 1.000000000000000000, 0.8660254037844387076, 1.000000000000000000, 0.8660254037844387076, 1.000000000000000000, 0.8660254037844387076, 1.000000000000000000, 0.8660254037844387076, 1.000000000000000000, 0.8660254037844387076, 1.000000000000000000, 0.8660254037844387076, 1.000000000000000000, 0.8660254037844387076, 1.000000000000000000, 0.8660254037844387076, 1.000000000000000000, 0.8660254037844387076, 1.000000000000000000, 0.8660254037844387076, 1.000000000000000000, 0.8660254037844387076, 1.000000000000000000, 0.8660254037844387076, 1.000000000000000000, 0.8660254037844387076, 1.000000000000000000, 0.8660254037844387076, 1.000000000000000000, 0.8660254037844387076, 1.000000000000000000, 0.8660254037844387076, 1.000000000000000000, 0.8660254037844387076, 1.000000000000000000, 0.8660254037844387076, 1.000000000000000000, 0.8660254037844387076, 1.000000000000000000, 0.8660254037844387076, 1.000000000000000000, 0.8660254037844387076, 1.000000000000000000, 0.8660254037844387076, 1.000000000000000000, 0.8660254037844387076, 1.000000000000000000, 0.8660254037844387076, 1.000000000000000000, 0.8660254037844387076, 1.000000000000000000, 0.8660254037844387076, 1.000000000000000000, 0.8660254037844387076, 1.000000000000000000, 0.8660254037844387076, 1.000000000000000000, 0.8660254037844387076, 1.000000000000000000, 0.8660254037844387076, 1.000000000000000000, 0.8660254037844387076, 1.000000000000000000, 0.8660254037844387076, 1.000000000000000000, 0.8660254037844387076, 1.000000000000000000, 0.8660254037844387076, 1.000000000000000000, 0.8660254037844387076, 1.000000000000000000, 0.8660254037844387076, 1.000000000000000000, 0.8660254037844387076, 1.000000000000000000, 0.8660254037844387076, 1.000000000000000000, 0.8660254037844387076, 1.000000000000000000, 0.8660254037844387076, 1.000000000000000000, 0.8660254037844387076, 1.000000000000000000, 0.8660254037844387076, 1.000000000000000000, 0.8660254037844387076, 1.000000000000000000, 0.8660254037844387076, 1.000000000000000000, 0.8660254037844387076, 1.000000000000000000, 0.8660254037844387076, 1.000000000000000000, 0.8660254037844387076, 1.000000000000000000, 0.8660254037844387076, 1.000000000000000000, 0.8660254037844387076, 1.000000000000000000, 0.8660254037844387076, 1.000000000000000000, 0.8660254037844387076, 1.000000000000000000, 0.8660254037844387076, 1.000000000000000000, 0.8660254037844387076, 1.000000000000000000, 0.8660254037844387076, 1.000000000000000000, 0.8660254037844387076, 1.000000000000000000, 0.8660254037844387076, 1.000000000000000000, 0.8660254037844387076, 1.000000000000000000, 0.8660254037844387076, 1.000000000000000000, 0.8660254037844387076, 1.000000000000000000, 0.8660254037844387076, 1.000000000000000000, 0.8660254037844387076, 1.000000000000000000, 0.8660254037844387076, 1.000000000000000000, 0.8660254037844387076, 1.000000000000000000, 0.8660254037844387076, 1.000000000000000000, 0.8660254037844387076, 1.000000000000000000, 0.8660254037844387076, 1.000000000000000000, 0.8660254037844387076, 1.000000000000000000, 0.8660254037844387076, 1.000000000000000000, 0.8660254037844387076, 1.000000000000000000, 0.8660254037844387076, 1.000000000000000000, 0.8660254037844387076, 1.000000000000000000, 0.8660254037844387076, 1.000000000000000000, 0.8660254037844387076, 1.000000000000000000, 0.8660254037844387076, 1.000000000000000000, 0.8660254037844387076, 1.000000000000000000, 0.8660254037844387076, 1.000000000000000000, 0.8660254037844387076, 1.000000000000000000, 0.8660254037844387076, 1.000000000000000000, 0.8660254037844387076, 1.000000000000000000, 0.8660254037844387076, 1.000000000000000000, 0.8660254037844387076, 1.000000000000000000, 0.8660254037844387076, 1.000000000000000000, 0.8660254037844387076, 1.000000000000000000, 0.8660254037844387076, 1.000000000000000000, 0.8660254037844387076, 1.000000000000000000, 0.8660254037844387076, 1.000000000000000000, 0.8660254037844387076, 1.000000000000000000, 0.8660254037844387076, 1.000000000000000000, 0.8660254037844387076, 1.000000000000000000, 0.8660254037844387076, 1.000000000000000000, 0.8660254037844387076, 1.000000000000000000, 0.8660254037844387076, 1.000000000000000000, 0.8660254037844387076, 1.000000000000000000, 0.8660254037844387076, 1.000000000000000000, 0.8660254037844387076, 1.000000000000000000, 0.8660254037844387076, 1.000000000000000000, 0.8660254037844387076, 1.000000000000000000, 0.8660254037844387076, 1.000000000000000000, 0.8660254037844387076, 1.000000000000000000, 0.8660254037844387076, 1.000000000000000000, 0.8660254037844387076, 1.000000000000000000, 0.8660254037844387076, 1.000000000000000000, 0.8660254037844387076, 1.000000000000000000, 0.8660254037844387076, 1.000000000000000000, 0.8660254037844387076, 1.000000000000000000, 0.8660254037844387076, 1.000000000000000000, 0.8660254037844387076, 1.000000000000000000, 0.8660254037844387076, 1.000000000000000000, 0.8660254037844387076, 1.000000000000000000, 0.8660254037844387076, 1.000000000000000000, 0.8660254037844387076, 1.000000000000000000, 0.8660254037844387076, 1.000000000000000000, 0.8660254037844387076, 1.000000000000000000, 0.8660254037844387076, 1.000000000000000000, 0.8660254037844387076, 1.000000000000000000, 0.8660254037844387076, 1.000000000000000000, 0.8660254037844387076, 1.000000000000000000, 0.8660254037844387076, 1.000000000000000000, 0.8660254037844387076, 1.000000000000000000, 0.8660254037844387076, 1.000000000000000000, 0.8660254037844387076, 1.000000000000000000, 0.8660254037844387076, 1.000000000000000000, 0.8660254037844387076, 1.000000000000000000, 0.8660254037844387076, 1.000000000000000000, 0.8660254037844387076, 1.000000000000000000, 0.8660254037844387076, 1.000000000000000000, 0.8660254037844387076, 1.000000000000000000, 0.8660254037844387076, 1.000000000000000000, 0.8660254037844387076, 1.000000000000000000, 0.8660254037844387076, 1.000000000000000000, 0.8660254037844387076, 1.000000000000000000, 0.8660254037844387076, 1.000000000000000000, 0.8660254037844387076, 1.000000000000000000, 0.8660254037844387076, 1.000000000000000000, 0.8660254037844387076, 1.000000000000000000, 0.8660254037844387076, 1.000000000000000000, 0.8660254037844387076, 1.000000000000000000, 0.8660254037844387076, 1.000000000000000000, 0.8660254037844387076, 1.000000000000000000, 0.8660254037844387076, 1.000000000000000000, 0.8660254037844387076, 1.000000000000000000, 0.8660254037844387076, 1.000000000000000000, 0.8660254037844387076, 1.000000000000000000, 0.8660254037844387076, 1.000000000000000000, 0.8660254037844387076, 1.000000000000000000, 0.8660254037844387076, 1.000000000000000000, 0.8660254037844387076, 1.000000000000000000, 0.8660254037844387076, 1.000000000000000000, 0.8660254037844387076, 1.000000000000000000, 0.8660254037844387076, 1.000000000000000000, 0.8660254037844387076, 1.000000000000000000, 0.8660254037844387076, 1.000000000000000000, 0.8660254037844387076, 1.000000000000000000, 0.8660254037844387076, 1.000000000000000000, 0.8660254037844387076, 1.000000000000000000, 0.8660254037844387076, 1.000000000000000000, 0.8660254037844387076, 1.000000000000000000, 0.8660254037844387076, 1.000000000000000000, 0.8660254037844387076, 1.000000000000000000, 0.8660254037844387076, 1.000000000000000000, 0.8660254037844387076, 1.000000000000000000, 0.8660254037844387076, 1.000000000000000000, 0.8660254037844387076, 1.000000000000000000, 0.8660254037844387076, 1.000000000000000000, 0.8660254037844387076, 1.000000000000000000, 0.8660254037844387076, 1.000000000000000000, 0.8660254037844387076, 1.000000000000000000, 0.8660254037844387076, 1.000000000000000000, 0.8660254037844387076, 1.000000000000000000, 0.8660254037844387076, 1.000000000000000000, 0.8660254037844387076, 1.000000000000000000, 0.8660254037844387076, 1.000000000000000000, 0.8660254037844387076, 1.000000000000000000, 0.8660254037844387076, 1.000000000000000000, 0.8660254037844387076, 1.000000000000000000, 0.8660254037844387076, 1.000000000000000000, 0.8660254037844387076, 1.000000000000000000, 0.8660254037844387076, 1.000000000000000000, 0.8660254037844387076, 1.000000000000000000, 0.8660254037844387076, 1.000000000000000000, 0.8660254037844387076, 1.000000000000000000, 0.8660254037844387076, 1.000000000000000000, 0.8660254037844387076, 1.000000000000000000, 0.8660254037844387076, 1.000000000000000000, 0.8660254037844387076, 1.000000000000000000, 0.8660254037844387076, 1.000000000000000000, 0.8660254037844387076, 1.000000000000000000, 0.8660254037844387076, 1.000000000000000000, 0.8660254037844387076, 1.000000000000000000, 0.8660254037844387076, 1.000000000000000000, 0.8660254037844387076, 1.000000000000000000, 0.8660254037844387076, 1.000000000000000000, 0.8660254037844387076, 1.000000000000000000, 0.8660254037844387076, 1.000000000000000000, 0.8660254037844387076, 1.000000000000000000, 0.8660254037844387076, 1.000000000000000000, 0.8660254037844387076, 1.000000000000000000, 0.8660254037844387076, 1.000000000000000000, 0.8660254037844387076, 1.000000000000000000, 0.8660254037844387076, 1.000000000000000000, 0.8660254037844387076, 1.000000000000000000, 0.8660254037844387076, 1.000000000000000000, 0.8660254037844387076, 1.000000000000000000, 0.8660254037844387076, 1.000000000000000000, 0.8660254037844387076, 1.000000000000000000, 0.8660254037844387076, 1.000000000000000000, 0.8660254037844387076, 1.000000000000000000, 0.8660254037844387076, 1.000000000000000000, 0.8660254037844387076, 1.000000000000000000, 0.8660254037844387076, 1.000000000000000000, 0.8660254037844387076, 1.000000000000000000, 0.8660254037844387076, 1.000000000000000000, 0.8660254037844387076, 1.000000000000000000, 0.8660254037844387076, 1.000000000000000000, 0.8660254037844387076, 1.000000000000000000, 0.8660254037844387076, 1.000000000000000000, 0.8660254037844387076, 1.000000000000000000, 0.8660254037844387076, 1.000000000000000000, 0.8660254037844387076, 1.000000000000000000, 0.8660254037844387076, 1.000000000000000000, 0.8660254037844387076, 1.000000000000000000, 0.8660254037844387076, 1.000000000000000000, 0.8660254037844387076, 1.000000000000000000, 0.8660254037844387076, 1.000000000000000000, 0.8660254037844387076, 1.000000000000000000, 0.8660254037844387076, 1.000000000000000000, 0.8660254037844387076, 1.000000000000000000, 0.8660254037844387076, 1.000000000000000000, 0.8660254037844387076, 1.000000000000000000, 0.8660254037844387076, 1.000000000000000000, 0.8660254037844387076, 1.000000000000000000, 0.8660254037844387076, 1.000000000000000000, 0.8660254037844387076, 1.000000000000000000, 0.8660254037844387076, 1.000000000000000000, 0.8660254037844387076, 1.000000000000000000, 0.8660254037844387076, 1.000000000000000000, 0.8660254037844387076, 1.000000000000000000, 0.8660254037844387076, 1.000000000000000000, 0.8660254037844387076, 1.000000000000000000, 0.8660254037844387076, 1.000000000000000000, 0.8660254037844387076, 1.000000000000000000, 0.8660254037844387076, 1.000000000000000000, 0.8660254037844387076, 1.000000000000000000, 0.8660254037844387076, 1.000000000000000000, 0.8660254037844387076, 1.000000000000000000, 0.8660254037844387076, 1.000000000000000000, 0.8660254037844387076, 1.000000000000000000, 0.8660254037844387076, 1.000000000000000000, 0.8660254037844387076, 1.000000000000000000, 0.8660254037844387076, 1.000000000000000000, 0.8660254037844387076, 1.000000000000000000, 0.8660254037844387076, 1.000000000000000000, 0.8660254037844387076, 1.000000000000000000, 0.8660254037844387076, 1.000000000000000000, 0.8660254037844387076, 1.000000000000000000, 0.8660254037844387076, 1.000000000000000000, 0.8660254037844387076, 1.000000000000000000, 0.8660254037844387076, 1.000000000000000000, 0.8660254037844387076, 1.000000000000000000, 0.8660254037844387076, 1.000000000000000000, 0.8660254037844387076, 1.000000000000000000, 0.8660254037844387076, 1.000000000000000000, 0.8660254037844387076, 1.000000000000000000, 0.8660254037844387076, 1.000000000000000000, 0.8660254037844387076, 1.000000000000000000, 0.8660254037844387076, 1.000000000000000000, 0.8660254037844387076, 1.000000000000000000, 0.8660254037844387076, 1.000000000000000000),
 ( 1.000000000000000000, 0.8660254037844387076, 1.000000000000000000, 0.8660254037844387076, 1.000000000000000000, 0.8660254037844387076, 1.000000000000000000, 0.8660254037844387076, 1.000000000000000000, 0.8660254037844387076, 1.000000000000000000, 0.8660254037844387076, 1.000000000000000000, 0.8660254037844387076, 1.000000000000000000, 0.8660254037844387076, 1.000000000000000000, 0.8660254037844387076, 1.000000000000000000, 0.8660254037844387076, 1.000000000000000000, 0.8660254037844387076, 1.000000000000000000, 0.8660254037844387076, 1.000000000000000000, 0.8660254037844387076, 1.000000000000000000, 0.8660254037844387076, 1.000000000000000000, 0.8660254037844387076, 1.000000000000000000, 0.8660254037844387076, 1.000000000000000000, 0.8660254037844387076, 1.000000000000000000, 0.8660254037844387076, 1.000000000000000000, 0.8660254037844387076, 1.000000000000000000, 0.8660254037844387076, 1.000000000000000000, 0.8660254037844387076, 1.000000000000000000, 0.8660254037844387076, 1.000000000000000000, 0.8660254037844387076, 1.000000000000000000, 0.8660254037844387076, 1.000000000000000000, 0.8660254037844387076, 1.000000000000000000, 0.8660254037844387076, 1.000000000000000000, 0.8660254037844387076, 1.000000000000000000, 0.8660254037844387076, 1.000000000000000000, 0.8660254037844387076, 1.000000000000000000, 0.8660254037844387076, 1.000000000000000000, 0.8660254037844387076, 1.000000000000000000, 0.8660254037844387076, 1.000000000000000000, 0.8660254037844387076, 1.000000000000000000, 0.8660254037844387076, 1.000000000000000000, 0.8660254037844387076, 1.000000000000000000, 0.8660254037844387076, 1.000000000000000000, 0.8660254037844387076, 1.000000000000000000, 0.8660254037844387076, 1.000000000000000000, 0.8660254037844387076, 1.000000000000000000, 0.8660254037844387076, 1.000000000000000000, 0.8660254037844387076, 1.000000000000000000, 0.8660254037844387076, 1.000000000000000000, 0.8660254037844387076, 1.000000000000000000, 0.8660254037844387076, 1.000000000000000000, 0.8660254037844387076, 1.000000000000000000, 0.8660254037844387076, 1.000000000000000000, 0.8660254037844387076, 1.000000000000000000, 0.8660254037844387076, 1.000000000000000000, 0.8660254037844387076, 1.000000000000000000, 0.8660254037844387076, 1.000000000000000000, 0.8660254037844387076, 1.000000000000000000, 0.8660254037844387076, 1.000000000000000000, 0.8660254037844387076, 1.000000000000000000, 0.8660254037844387076, 1.000000000000000000, 0.8660254037844387076, 1.000000000000000000, 0.8660254037844387076, 1.000000000000000000, 0.8660254037844387076, 1.000000000000000000, 0.8660254037844387076, 1.000000000000000000, 0.8660254037844387076, 1.000000000000000000, 0.8660254037844387076, 1.000000000000000000, 0.8660254037844387076, 1.000000000000000000, 0.8660254037844387076, 1.000000000000000000, 0.8660254037844387076, 1.000000000000000000, 0.8660254037844387076, 1.000000000000000000, 0.8660254037844387076, 1.000000000000000000, 0.8660254037844387076, 1.000000000000000000, 0.8660254037844387076, 1.000000000000000000, 0.8660254037844387076, 1.000000000000000000, 0.8660254037844387076, 1.000000000000000000, 0.8660254037844387076, 1.000000000000000000, 0.8660254037844387076, 1.000000000000000000, 0.8660254037844387076, 1.000000000000000000, 0.8660254037844387076, 1.000000000000000000, 0.8660254037844387076, 1.000000000000000000, 0.8660254037844387076, 1.000000000000000000, 0.8660254037844387076, 1.000000000000000000, 0.8660254037844387076, 1.000000000000000000, 0.8660254037844387076, 1.000000000000000000, 0.8660254037844387076, 1.000000000000000000, 0.8660254037844387076, 1.000000000000000000, 0.8660254037844387076, 1.000000000000000000, 0.8660254037844387076, 1.000000000000000000, 0.8660254037844387076, 1.000000000000000000, 0.8660254037844387076, 1.000000000000000000, 0.8660254037844387076, 1.000000000000000000, 0.8660254037844387076, 1.000000000000000000, 0.8660254037844387076, 1.000000000000000000, 0.8660254037844387076, 1.000000000000000000, 0.8660254037844387076, 1.000000000000000000, 0.8660254037844387076, 1.000000000000000000, 0.8660254037844387076, 1.000000000000000000, 0.8660254037844387076, 1.000000000000000000, 0.8660254037844387076, 1.000000000000000000, 0.8660254037844387076, 1.000000000000000000, 0.8660254037844387076, 1.000000000000000000, 0.8660254037844387076, 1.000000000000000000, 0.8660254037844387076, 1.000000000000000000, 0.8660254037844387076, 1.000000000000000000, 0.8660254037844387076, 1.000000000000000000, 0.8660254037844387076, 1.000000000000000000, 0.8660254037844387076, 1.000000000000000000, 0.8660254037844387076, 1.000000000000000000, 0.8660254037844387076, 1.000000000000000000, 0.8660254037844387076, 1.000000000000000000, 0.8660254037844387076, 1.000000000000000000, 0.8660254037844387076, 1.000000000000000000, 0.8660254037844387076, 1.000000000000000000, 0.8660254037844387076, 1.000000000000000000, 0.8660254037844387076, 1.000000000000000000, 0.8660254037844387076, 1.000000000000000000, 0.8660254037844387076, 1.000000000000000000, 0.8660254037844387076, 1.000000000000000000, 0.8660254037844387076, 1.000000000000000000, 0.8660254037844387076, 1.000000000000000000, 0.8660254037844387076, 1.000000000000000000, 0.8660254037844387076, 1.000000000000000000, 0.8660254037844387076, 1.000000000000000000, 0.8660254037844387076, 1.000000000000000000, 0.8660254037844387076, 1.000000000000000000, 0.8660254037844387076, 1.000000000000000000, 0.8660254037844387076, 1.000000000000000000, 0.8660254037844387076, 1.000000000000000000, 0.8660254037844387076, 1.000000000000000000, 0.8660254037844387076, 1.000000000000000000, 0.8660254037844387076, 1.000000000000000000, 0.8660254037844387076, 1.000000000000000000, 0.8660254037844387076, 1.000000000000000000, 0.8660254037844387076, 1.000000000000000000, 0.8660254037844387076, 1.000000000000000000, 0.8660254037844387076, 1.000000000000000000, 0.8660254037844387076, 1.000000000000000000, 0.8660254037844387076, 1.000000000000000000, 0.8660254037844387076, 1.000000000000000000, 0.8660254037844387076, 1.000000000000000000, 0.8660254037844387076, 1.000000000000000000, 0.8660254037844387076, 1.000000000000000000, 0.8660254037844387076, 1.000000000000000000, 0.8660254037844387076, 1.000000000000000000, 0.8660254037844387076, 1.000000000000000000, 0.8660254037844387076, 1.000000000000000000, 0.8660254037844387076, 1.000000000000000000, 0.8660254037844387076, 1.000000000000000000, 0.8660254037844387076, 1.000000000000000000, 0.8660254037844387076, 1.000000000000000000, 0.8660254037844387076, 1.000000000000000000, 0.8660254037844387076, 1.000000000000000000, 0.8660254037844387076, 1.000000000000000000, 0.8660254037844387076, 1.000000000000000000, 0.8660254037844387076, 1.000000000000000000, 0.8660254037844387076, 1.000000000000000000, 0.8660254037844387076, 1.000000000000000000, 0.8660254037844387076, 1.000000000000000000, 0.8660254037844387076, 1.000000000000000000, 0.8660254037844387076, 1.000000000000000000, 0.8660254037844387076, 1.000000000000000000, 0.8660254037844387076, 1.000000000000000000, 0.8660254037844387076, 1.000000000000000000, 0.8660254037844387076, 1.000000000000000000, 0.8660254037844387076, 1.000000000000000000, 0.8660254037844387076, 1.000000000000000000, 0.8660254037844387076, 1.000000000000000000, 0.8660254037844387076, 1.000000000000000000, 0.8660254037844387076, 1.000000000000000000, 0.8660254037844387076, 1.000000000000000000, 0.8660254037844387076, 1.000000000000000000, 0.8660254037844387076, 1.000000000000000000, 0.8660254037844387076, 1.000000000000000000, 0.8660254037844387076, 1.000000000000000000, 0.8660254037844387076, 1.000000000000000000, 0.8660254037844387076, 1.000000000000000000, 0.8660254037844387076, 1.000000000000000000, 0.8660254037844387076, 1.000000000000000000, 0.8660254037844387076, 1.000000000000000000, 0.8660254037844387076, 1.000000000000000000, 0.8660254037844387076, 1.000000000000000000, 0.8660254037844387076, 1.000000000000000000, 0.8660254037844387076, 1.000000000000000000, 0.8660254037844387076, 1.000000000000000000, 0.8660254037844387076, 1.000000000000000000, 0.8660254037844387076, 1.000000000000000000, 0.8660254037844387076, 1.000000000000000000, 0.8660254037844387076, 1.000000000000000000, 0.8660254037844387076, 1.000000000000000000, 0.8660254037844387076, 1.000000000000000000, 0.8660254037844387076, 1.000000000000000000, 0.8660254037844387076, 1.000000000000000000, 0.8660254037844387076, 1.000000000000000000, 0.8660254037844387076, 1.000000000000000000, 0.8660254037844387076, 1.000000000000000000, 0.8660254037844387076, 1.000000000000000000, 0.8660254037844387076, 1.000000000000000000, 0.8660254037844387076, 1.000000000000000000, 0.8660254037844387076, 1.000000000000000000, 0.8660254037844387076, 1.000000000000000000, 0.8660254037844387076, 1.000000000000000000, 0.8660254037844387076, 1.000000000000000000, 0.8660254037844387076, 1.000000000000000000, 0.8660254037844387076, 1.000000000000000000, 0.8660254037844387076, 1.000000000000000000, 0.8660254037844387076, 1.000000000000000000, 0.8660254037844387076, 1.000000000000000000, 0.8660254037844387076, 1.000000000000000000, 0.8660254037844387076, 1.000000000000000000, 0.8660254037844387076, 1.000000000000000000, 0.8660254037844387076, 1.000000000000000000, 0.8660254037844387076, 1.000000000000000000, 0.8660254037844387076, 1.000000000000000000, 0.8660254037844387076, 1.000000000000000000, 0.8660254037844387076, 1.000000000000000000, 0.8660254037844387076, 1.000000000000000000, 0.8660254037844387076, 1.000000000000000000, 0.8660254037844387076, 1.000000000000000000, 0.8660254037844387076, 1.000000000000000000, 0.8660254037844387076, 1.000000000000000000, 0.8660254037844387076, 1.000000000000000000, 0.8660254037844387076, 1.000000000000000000, 0.8660254037844387076, 1.000000000000000000, 0.8660254037844387076, 1.000000000000000000, 0.8660254037844387076, 1.000000000000000000, 0.8660254037844387076, 1.000000000000000000, 0.8660254037844387076, 1.000000000000000000, 0.8660254037844387076, 1.000000000000000000, 0.8660254037844387076, 1.000000000000000000, 0.8660254037844387076, 1.000000000000000000, 0.8660254037844387076, 1.000000000000000000, 0.8660254037844387076, 1.000000000000000000, 0.8660254037844387076, 1.000000000000000000, 0.8660254037844387076, 1.000000000000000000, 0.8660254037844387076, 1.000000000000000000, 0.8660254037844387076, 1.000000000000000000, 0.8660254037844387076, 1.000000000000000000, 0.8660254037844387076, 1.000000000000000000, 0.8660254037844387076, 1.000000000000000000, 0.8660254037844387076, 1.000000000000000000, 0.8660254037844387076, 1.000000000000000000, 0.8660254037844387076, 1.000000000000000000, 0.8660254037844387076, 1.000000000000000000, 0.8660254037844387076, 1.000000000000000000, 0.8660254037844387076, 1.000000000000000000, 0.8660254037844387076, 1.000000000000000000, 0.8660254037844387076, 1.000000000000000000, 0.8660254037844387076, 1.000000000000000000, 0.8660254037844387076, 1.000000000000000000, 0.8660254037844387076, 1.000000000000000000, 0.8660254037844387076, 1.000000000000000000, 0.8660254037844387076, 1.000000000000000000, 0.8660254037844387076, 1.000000000000000000, 0.8660254037844387076, 1.000000000000000000, 0.8660254037844387076, 1.000000000000000000, 0.8660254037844387076, 1.000000000000000000, 0.8660254037844387076, 1.000000000000000000, 0.8660254037844387076, 1.000000000000000000, 0.8660254037844387076, 1.000000000000000000, 0.8660254037844387076, 1.000000000000000000, 0.8660254037844387076, 1.000000000000000000, 0.8660254037844387076, 1.000000000000000000, 0.8660254037844387076, 1.000000000000000000, 0.8660254037844387076, 1.000000000000000000, 0.8660254037844387076, 1.000000000000000000, 0.8660254037844387076, 1.000000000000000000, 0.8660254037844387076, 1.000000000000000000, 0.8660254037844387076, 1.000000000000000000, 0.8660254037844387076, 1.000000000000000000, 0.8660254037844387076, 1.000000000000000000, 0.8660254037844387076, 1.000000000000000000, 0.8660254037844387076, 1.000000000000000000, 0.8660254037844387076, 1.000000000000000000, 0.8660254037844387076, 1.000000000000000000, 0.8660254037844387076, 1.000000000000000000, 0.8660254037844387076, 1.000000000000000000, 0.8660254037844387076, 1.000000000000000000, 0.8660254037844387076, 1.000000000000000000, 0.8660254037844387076, 1.000000000000000000, 0.8660254037844387076, 1.000000000000000000, 0.8660254037844387076, 1.000000000000000000, 0.8660254037844387076, 1.000000000000000000, 0.8660254037844387076, 1.000000000000000000, 0.8660254037844387076, 1.000000000000000000, 0.8660254037844387076, 1.000000000000000000, 0.8660254037844387076, 1.000000000000000000, 0.8660254037844387076, 1.000000000000000000, 0.8660254037844387076, 1.000000000000000000, 0.8660254037844387076, 1.000000000000000000, 0.8660254037844387076, 1.000000000000000000, 0.8660254037844387076, 1.000000000000000000, 0.8660254037844387076, 1.000000000000000000, 0.8660254037844387076, 1.000000000000000000, 0.8660254037844387076, 1.000000000000000000, 0.8660254037844387076, 1.000000000000000000, 0.8660254037844387076, 1.000000000000000000, 0.8660254037844387076, 1.000000000000000000, 0.8660254037844387076, 1.000000000000000000, 0.8660254037844387076, 1.000000000000000000, 0.8660254037844387076, 1.000000000000000000, 0.8660254037844387076, 1.000000000000000000, 0.8660254037844387076, 1.000000000000000000, 0.8660254037844387076, 1.000000000000000000, 0.8660254037844387076, 1.000000000000000000, 0.8660254037844387076, 1.000000000000000000, 0.8660254037844387076, 1.000000000000000000, 0.8660254037844387076, 1.000000000000000000, 0.8660254037844387076, 1.000000000000000000, 0.8660254037844387076, 1.000000000000000000, 0.8660254037844387076, 1.000000000000000000, 0.8660254037844387076, 1.000000000000000000, 0.8660254037844387076, 1.000000000000000000, 0.8660254037844387076, 1.000000000000000000, 0.8660254037844387076, 1.000000000000000000, 0.8660254037844387076, 1.000000000000000000, 0.8660254037844387076, 1.000000000000000000, 0.8660254037844387076, 1.000000000000000000, 0.8660254037844387076, 1.000000000000000000, 0.8660254037844387076, 1.000000000000000000, 0.8660254037844387076, 1.000000000000000000, 0.8660254037844387076, 1.000000000000000000, 0.8660254037844387076, 1.000000000000000000, 0.8660254037844387076, 1.000000000000000000, 0.8660254037844387076, 1.000000000000000000, 0.8660254037844387076, 1.000000000000000000, 0.8660254037844387076, 1.000000000000000000, 0.8660254037844387076, 1.000000000000000000, 0.8660254037844387076, 1.000000000000000000, 0.8660254037844387076, 1.000000000000000000, 0.8660254037844387076, 1.000000000000000000, 0.8660254037844387076, 1.000000000000000000, 0.8660254037844387076, 1.000000000000000000, 0.8660254037844387076, 1.000000000000000000, 0.8660254037844387076, 1.000000000000000000, 0.8660254037844387076, 1.000000000000000000, 0.8660254037844387076, 1.000000000000000000, 0.8660254037844387076, 1.000000000000000000, 0.8660254037844387076, 1.000000000000000000, 0.8660254037844387076, 1.000000000000000000, 0.8660254037844387076, 1.000000000000000000, 0.8660254037844387076, 1.000000000000000000, 0.8660254037844387076, 1.000000000000000000, 0.8660254037844387076, 1.000000000000000000, 0.8660254037844387076, 1.000000000000000000, 0.8660254037844387076, 1.000000000000000000, 0.8660254037844387076, 1.000000000000000000, 0.8660254037844387076, 1.000000000000000000, 0.8660254037844387076, 1.000000000000000000, 0.8660254037844387076, 1.000000000000000000, 0.8660254037844387076, 1.000000000000000000, 0.8660254037844387076, 1.000000000000000000, 0.8660254037844387076, 1.000000000000000000, 0.8660254037844387076, 1.000000000000000000, 0.8660254037844387076, 1.000000000000000000, 0.8660254037844387076, 1.000000000000000000, 0.8660254037844387076, 1.000000000000000000, 0.8660254037844387076, 1.000000000000000000, 0.8660254037844387076, 1.000000000000000000, 0.8660254037844387076, 1.000000000000000000, 0.8660254037844387076, 1.000000000000000000, 0.8660254037844387076, 1.000000000000000000, 0.8660254037844387076, 1.000000000000000000, 0.8660254037844387076, 1.000000000000000000, 0.8660254037844387076, 1.000000000000000000, 0.8660254037844387076, 1.000000000000000000, 0.8660254037844387076, 1.000000000000000000, 0.8660254037844387076, 1.000000000000000000, 0.8660254037844387076, 1.000000000000000000, 0.8660254037844387076, 1.000000000000000000, 0.8660254037844387076, 1.000000000000000000, 0.8660254037844387076, 1.000000000000000000, 0.8660254037844387076, 1.000000000000000000, 0.8660254037844387076, 1.000000000000000000, 0.8660254037844387076, 1.000000000000000000, 0.8660254037844387076, 1.000000000000000000, 0.8660254037844387076, 1.000000000000000000, 0.8660254037844387076, 1.000000000000000000, 0.8660254037844387076, 1.000000000000000000, 0.8660254037844387076, 1.000000000000000000, 0.8660254037844387076, 1.000000000000000000, 0.8660254037844387076, 1.000000000000000000, 0.8660254037844387076, 1.000000000000000000, 0.8660254037844387076, 1.000000000000000000, 0.8660254037844387076, 1.000000000000000000, 0.8660254037844387076, 1.000000000000000000, 0.8660254037844387076, 1.000000000000000000, 0.8660254037844387076, 1.000000000000000000, 0.8660254037844387076, 1.000000000000000000, 0.8660254037844387076, 1.000000000000000000, 0.8660254037844387076, 1.000000000000000000, 0.8660254037844387076, 1.000000000000000000, 0.8660254037844387076, 1.000000000000000000, 0.8660254037844387076, 1.000000000000000000, 0.8660254037844387076, 1.000000000000000000, 0.8660254037844387076, 1.000000000000000000, 0.8660254037844387076, 1.000000000000000000, 0.8660254037844387076, 1.000000000000000000, 0.8660254037844387076, 1.000000000000000000, 0.8660254037844387076, 1.000000000000000000, 0.8660254037844387076, 1.000000000000000000, 0.8660254037844387076, 1.000000000000000000, 0.8660254037844387076, 1.000000000000000000, 0.8660254037844387076, 1.000000000000000000, 0.8660254037844387076, 1.000000000000000000, 0.8660254037844387076, 1.000000000000000000, 0.8660254037844387076, 1.000000000000000000, 0.8660254037844387076, 1.000000000000000000, 0.8660254037844387076, 1.000000000000000000, 0.8660254037844387076, 1.000000000000000000, 0.8660254037844387076, 1.000000000000000000, 0.8660254037844387076, 1.000000000000000000, 0.8660254037844387076, 1.000000000000000000, 0.8660254037844387076, 1.000000000000000000, 0.8660254037844387076, 1.000000000000000000, 0.8660254037844387076, 1.000000000000000000, 0.8660254037844387076, 1.000000000000000000, 0.8660254037844387076, 1.000000000000000000, 0.8660254037844387076, 1.000000000000000000, 0.8660254037844387076, 1.000000000000000000, 0.8660254037844387076, 1.000000000000000000, 0.8660254037844387076, 1.000000000000000000, 0.8660254037844387076, 1.000000000000000000, 0.8660254037844387076, 1.000000000000000000, 0.8660254037844387076, 1.000000000000000000, 0.8660254037844387076, 1.000000000000000000, 0.8660254037844387076, 1.000000000000000000, 0.8660254037844387076, 1.000000000000000000, 0.8660254037844387076, 1.000000000000000000, 0.8660254037844387076, 1.000000000000000000, 0.8660254037844387076, 1.000000000000000000, 0.8660254037844387076, 1.000000000000000000, 0.8660254037844387076, 1.000000000000000000, 0.8660254037844387076, 1.000000000000000000, 0.8660254037844387076, 1.000000000000000000, 0.8660254037844387076, 1.000000000000000000, 0.8660254037844387076, 1.000000000000000000, 0.8660254037844387076, 1.000000000000000000, 0.8660254037844387076, 1.000000000000000000, 0.8660254037844387076, 1.000000000000000000, 0.8660254037844387076, 1.000000000000000000, 0.8660254037844387076, 1.000000000000000000, 0.8660254037844387076, 1.000000000000000000, 0.8660254037844387076, 1.000000000000000000, 0.8660254037844387076, 1.000000000000000000, 0.8660254037844387076, 1.000000000000000000, 0.8660254037844387076, 1.000000000000000000, 0.8660254037844387076, 1.000000000000000000, 0.8660254037844387076, 1.000000000000000000, 0.8660254037844387076, 1.000000000000000000, 0.8660254037844387076, 1.000000000000000000, 0.8660254037844387076, 1.000000000000000000, 0.8660254037844387076, 1.000000000000000000, 0.8660254037844387076, 1.000000000000000000, 0.8660254037844387076, 1.000000000000000000, 0.8660254037844387076, 1.000000000000000000, 0.8660254037844387076, 1.000000000000000000, 0.8660254037844387076, 1.000000000000000000, 0.8660254037844387076, 1.000000000000000000, 0.8660254037844387076, 1.000000000000000000, 0.8660254037844387076, 1.000000000000000000, 0.8660254037844387076, 1.000000000000000000, 0.8660254037844387076, 1.000000000000000000, 0.8660254037844387076, 1.000000000000000000, 0.8660254037844387076, 1.000000000000000000, 0.8660254037844387076, 1.000000000000000000, 0.8660254037844387076, 1.000000000000000000, 0.8660254037844387076, 1.000000000000000000, 0.8660254037844387076, 1.000000000000000000, 0.8660254037844387076, 1.000000000000000000, 0.8660254037844387076, 1.000000000000000000, 0.8660254037844387076, 1.000000000000000000, 0.8660254037844387076, 1.000000000000000000, 0.8660254037844387076, 1.000000000000000000, 0.8660254037844387076, 1.000000000000000000, 0.8660254037844387076, 1.000000000000000000, 0.8660254037844387076, 1.000000000000000000, 0.8660254037844387076, 1.000000000000000000, 0.8660254037844387076, 1.000000000000000000, 0.8660254037844387076, 1.000000000000000000, 0.8660254037844387076, 1.000000000000000000, 0.8660254037844387076, 1.000000000000000000, 0.8660254037844387076, 1.000000000000000000, 0.8660254037844387076, 1.000000000000000000, 0.8660254037844387076, 1.000000000000000000, 0.8660254037844387076, 1.000000000000000000, 0.8660254037844387076, 1.000000000000000000, 0.8660254037844387076, 1.000000000000000000, 0.8660254037844387076, 1.000000000000000000, 0.8660254037844387076, 1.000000000000000000, 0.8660254037844387076, 1.000000000000000000, 0.8660254037844387076, 1.000000000000000000, 0.8660254037844387076, 1.000000000000000000, 0.8660254037844387076, 1.000000000000000000, 0.8660254037844387076, 1.000000000000000000, 0.8660254037844387076, 1.000000000000000000, 0.8660254037844387076, 1.000000000000000000, 0.8660254037844387076, 1.000000000000000000, 0.8660254037844387076, 1.000000000000000000, 0.8660254037844387076, 1.000000000000000000, 0.8660254037844387076, 1.000000000000000000, 0.8660254037844387076, 1.000000000000000000, 0.8660254037844387076, 1.000000000000000000, 0.8660254037844387076, 1.000000000000000000, 0.8660254037844387076, 1.000000000000000000, 0.8660254037844387076, 1.000000000000000000, 0.8660254037844387076, 1.000000000000000000, 0.8660254037844387076, 1.000000000000000000, 0.8660254037844387076, 1.000000000000000000, 0.8660254037844387076, 1.000000000000000000, 0.8660254037844387076, 1.000000000000000000, 0.8660254037844387076, 1.000000000000000000, 0.8660254037844387076, 1.000000000000000000, 0.8660254037844387076, 1.000000000000000000, 0.8660254037844387076, 1.000000000000000000, 0.8660254037844387076, 1.000000000000000000, 0.8660254037844387076, 1.000000000000000000, 0.8660254037844387076, 1.000000000000000000, 0.8660254037844387076, 1.000000000000000000, 0.8660254037844387076, 1.000000000000000000, 0.8660254037844387076, 1.000000000000000000, 0.8660254037844387076, 1.000000000000000000, 0.8660254037844387076, 1.000000000000000000, 0.8660254037844387076, 1.000000000000000000, 0.8660254037844387076, 1.000000000000000000, 0.8660254037844387076, 1.000000000000000000, 0.8660254037844387076, 1.000000000000000000, 0.8660254037844387076, 1.000000000000000000, 0.8660254037844387076, 1.000000000000000000, 0.8660254037844387076, 1.000000000000000000, 0.8660254037844387076, 1.000000000000000000, 0.8660254037844387076, 1.000000000000000000, 0.8660254037844387076, 1.000000000000000000, 0.8660254037844387076, 1.000000000000000000, 0.8660254037844387076, 1.000000000000000000, 0.8660254037844387076, 1.000000000000000000, 0.8660254037844387076, 1.000000000000000000, 0.8660254037844387076, 1.000000000000000000, 0.8660254037844387076, 1.000000000000000000, 0.8660254037844387076, 1.000000000000000000, 0.8660254037844387076, 1.000000000000000000, 0.8660254037844387076, 1.000000000000000000, 0.8660254037844387076, 1.000000000000000000, 0.8660254037844387076, 1.000000000000000000, 0.8660254037844387076, 1.000000000000000000, 0.8660254037844387076, 1.000000000000000000, 0.8660254037844387076, 1.000000000000000000, 0.8660254037844387076, 1.000000000000000000, 0.8660254037844387076, 1.000000000000000000, 0.8660254037844387076, 1.000000000000000000, 0.8660254037844387076, 1.000000000000000000, 0.8660254037844387076, 1.000000000000000000, 0.8660254037844387076, 1.000000000000000000, 0.8660254037844387076, 1.000000000000000000, 0.8660254037844387076, 1.000000000000000000, 0.8660254037844387076, 1.000000000000000000, 0.8660254037844387076, 1.000000000000000000, 0.8660254037844387076, 1.000000000000000000, 0.8660254037844387076, 1.000000000000000000, 0.8660254037844387076, 1.000000000000000000, 0.8660254037844387076, 1.000000000000000000, 0.8660254037844387076, 1.000000000000000000, 0.8660254037844387076, 1.000000000000000000, 0.8660254037844387076, 1.000000000000000000, 0.8660254037844387076, 1.000000000000000000, 0.8660254037844387076, 1.000000000000000000, 0.8660254037844387076, 1.000000000000000000, 0.8660254037844387076, 1.000000000000000000, 0.8660254037844387076, 1.000000000000000000, 0.8660254037844387076, 1.000000000000000000, 0.8660254037844387076, 1.000000000000000000, 0.8660254037844387076, 1.000000000000000000, 0.8660254037844387076, 1.000000000000000000, 0.8660254037844387076, 1.000000000000000000, 0.8660254037844387076, 1.000000000000000000, 0.8660254037844387076, 1.000000000000000000, 0.8660254037844387076, 1.000000000000000000, 0.8660254037844387076, 1.000000000000000000, 0.8660254037844387076, 1.000000000000000000, 0.8660254037844387076, 1.000000000000000000, 0.8660254037844387076, 1.000000000000000000, 0.8660254037844387076, 1.000000000000000000, 0.8660254037844387076, 1.000000000000000000, 0.8660254037844387076, 1.000000000000000000, 0.8660254037844387076, 1.000000000000000000, 0.8660254037844387076, 1.000000000000000000, 0.8660254037844387076, 1.000000000000000000, 0.8660254037844387076, 1.000000000000000000, 0.8660254037844387076, 1.000000000000000000, 0.8660254037844387076, 1.000000000000000000, 0.8660254037844387076, 1.000000000000000000, 0.8660254037844387076, 1.000000000000000000, 0.8660254037844387076, 1.000000000000000000, 0.8660254037844387076, 1.000000000000000000, 0.8660254037844387076, 1.000000000000000000, 0.8660254037844387076, 1.000000000000000000, 0.8660254037844387076, 1.000000000000000000, 0.8660254037844387076, 1.000000000000000000, 0.8660254037844387076, 1.000000000000000000, 0.8660254037844387076, 1.000000000000000000, 0.8660254037844387076, 1.000000000000000000, 0.8660254037844387076, 1.000000000000000000, 0.8660254037844387076, 1.000000000000000000, 0.8660254037844387076, 1.000000000000000000, 0.8660254037844387076, 1.000000000000000000, 0.8660254037844387076, 1.000000000000000000, 0.8660254037844387076, 1.000000000000000000, 0.8660254037844387076, 1.000000000000000000, 0.8660254037844387076, 1.000000000000000000, 0.8660254037844387076, 1.000000000000000000, 0.8660254037844387076, 1.000000000000000000, 0.8660254037844387076, 1.000000000000000000, 0.8660254037844387076, 1.000000000000000000, 0.8660254037844387076, 1.000000000000000000, 0.8660254037844387076, 1.000000000000000000, 0.8660254037844387076, 1.000000000000000000, 0.8660254037844387076, 1.000000000000000000, 0.8660254037844387076, 1.000000000000000000, 0.8660254037844387076, 1.000000000000000000, 0.8660254037844387076, 1.000000000000000000, 0.8660254037844387076, 1.000000000000000000, 0.8660254037844387076, 1.000000000000000000, 0.8660254037844387076, 1.000000000000000000, 0.8660254037844387076, 1.000000000000000000, 0.8660254037844387076, 1.000000000000000000, 0.8660254037844387076, 1.000000000000000000, 0.8660254037844387076, 1.000000000000000000, 0.8660254037844387076, 1.000000000000000000, 0.8660254037844387076, 1.000000000000000000, 0.8660254037844387076, 1.000000000000000000, 0.8660254037844387076, 1.000000000000000000, 0.8660254037844387076, 1.000000000000000000, 0.8660254037844387076, 1.000000000000000000, 0.8660254037844387076, 1.000000000000000000, 0.8660254037844387076, 1.000000000000000000, 0.8660254037844387076, 1.000000000000000000, 0.8660254037844387076, 1.000000000000000000, 0.8660254037844387076, 1.000000000000000000, 0.8660254037844387076, 1.000000000000000000, 0.8660254037844387076, 1.000000000000000000, 0.8660254037844387076, 1.000000000000000000, 0.8660254037844387076, 1.000000000000000000, 0.8660254037844387076, 1.000000000000000000, 0.8660254037844387076, 1.000000000000000000, 0.8660254037844387076, 1.000000000000000000, 0.8660254037844387076, 1.000000000000000000, 0.8660254037844387076, 1.000000000000000000, 0.8660254037844387076, 1.000000000000000000, 0.8660254037844387076, 1.000000000000000000, 0.8660254037844387076, 1.000000000000000000, 0.8660254037844387076, 1.000000000000000000, 0.8660254037844387076, 1.000000000000000000, 0.8660254037844387076, 1.000000000000000000, 0.8660254037844387076, 1.000000000000000000, 0.8660254037844387076, 1.000000000000000000, 0.8660254037844387076, 1.000000000000000000, 0.8660254037844387076, 1.000000000000000000, 0.8660254037844387076, 1.000000000000000000, 0.8660254037844387076, 1.000000000000000000, 0.8660254037844387076, 1.000000000000000000, 0.8660254037844387076, 1.000000000000000000, 0.8660254037844387076, 1.000000000000000000, 0.8660254037844387076, 1.000000000000000000, 0.8660254037844387076, 1.000000000000000000, 0.8660254037844387076, 1.000000000000000000, 0.8660254037844387076, 1.000000000000000000, 0.8660254037844387076, 1.000000000000000000, 0.8660254037844387076, 1.000000000000000000, 0.8660254037844387076, 1.000000000000000000, 0.8660254037844387076, 1.000000000000000000, 0.8660254037844387076, 1.000000000000000000, 0.8660254037844387076, 1.000000000000000000, 0.8660254037844387076, 1.000000000000000000, 0.8660254037844387076, 1.000000000000000000, 0.8660254037844387076, 1.000000000000000000, 0.8660254037844387076, 1.000000000000000000, 0.8660254037844387076, 1.000000000000000000, 0.8660254037844387076, 1.000000000000000000, 0.8660254037844387076, 1.000000000000000000, 0.8660254037844387076, 1.000000000000000000, 0.8660254037844387076, 1.000000000000000000, 0.8660254037844387076, 1.000000000000000000, 0.8660254037844387076, 1.000000000000000000, 0.8660254037844387076, 1.000000000000000000, 0.8660254037844387076, 1.000000000000000000, 0.8660254037844387076, 1.000000000000000000, 0.8660254037844387076, 1.000000000000000000, 0.8660254037844387076, 1.000000000000000000, 0.8660254037844387076, 1.000000000000000000, 0.8660254037844387076, 1.000000000000000000, 0.8660254037844387076, 1.000000000000000000, 0.8660254037844387076, 1.000000000000000000, 0.8660254037844387076, 1.000000000000000000, 0.8660254037844387076, 1.000000000000000000, 0.8660254037844387076, 1.000000000000000000, 0.8660254037844387076, 1.000000000000000000, 0.8660254037844387076, 1.000000000000000000, 0.8660254037844387076, 1.000000000000000000, 0.8660254037844387076, 1.000000000000000000, 0.8660254037844387076, 1.000000000000000000, 0.8660254037844387076, 1.000000000000000000, 0.8660254037844387076, 1.000000000000000000, 0.8660254037844387076, 1.000000000000000000, 0.8660254037844387076, 1.000000000000000000, 0.8660254037844387076, 1.000000000000000000, 0.8660254037844387076, 1.000000000000000000, 0.8660254037844387076, 1.000000000000000000, 0.8660254037844387076, 1.000000000000000000, 0.8660254037844387076, 1.000000000000000000, 0.8660254037844387076, 1.000000000000000000, 0.8660254037844387076, 1.000000000000000000, 0.8660254037844387076, 1.000000000000000000, 0.8660254037844387076, 1.000000000000000000, 0.8660254037844387076, 1.000000000000000000, 0.8660254037844387076, 1.000000000000000000, 0.8660254037844387076, 1.000000000000000000, 0.8660254037844387076, 1.000000000000000000, 0.8660254037844387076, 1.000000000000000000, 0.8660254037844387076, 1.000000000000000000, 0.8660254037844387076, 1.000000000000000000, 0.8660254037844387076, 1.000000000000000000, 0.8660254037844387076, 1.000000000000000000, 0.8660254037844387076, 1.000000000000000000, 0.8660254037844387076, 1.000000000000000000, 0.8660254037844387076, 1.000000000000000000, 0.8660254037844387076, 1.000000000000000000, 0.8660254037844387076, 1.000000000000000000) ) ) 
 REPRESENTATION_ITEM ( '' )  SURFACE ( )  );
#20398=CARTESIAN_POINT ( 'NONE',  ( 1.749999999999998224, 14.46891108675447768, -55.62764746908817415 ) ) ;
#20399=CARTESIAN_POINT ( 'NONE',  ( 0.000000000000000000, 17.50000000000002487, -149.5231586289125687 ) ) ;
#20400=CARTESIAN_POINT ( 'NONE',  ( -3.500000000000000000, 19.52072594216370405, -25.04431413575484910 ) ) ;
#20401=ORIENTED_EDGE ( 'NONE', *, *, #24609, .T. ) ;
#20402=EDGE_CURVE ( 'NONE', #8868, #33770, #26284, .T. ) ;
#20403=CARTESIAN_POINT ( 'NONE',  ( -3.500000000000002220, 15.47927405783632260, -45.57139747004410424 ) ) ;
#20405=CARTESIAN_POINT ( 'NONE',  ( -3.310556943750001313, 17.50000000000001066, -29.85160580289947063 ) ) ;
#20406=CARTESIAN_POINT ( 'NONE',  ( 4.648177544792955347E-16, 21.00000000000001776, -80.90473080337743284 ) ) ;
#20407=CARTESIAN_POINT ( 'NONE',  ( -3.500000000000002220, 15.47927405783632615, -56.87764746908817415 ) ) ;
#20409=CARTESIAN_POINT ( 'NONE',  ( 4.648177544792955347E-16, 21.00000000000002132, -119.9047308033774328 ) ) ;
#20411=CARTESIAN_POINT ( 'NONE',  ( -7.022189441860112050E-16, 13.67729811471672186, -74.51410580289947916 ) ) ;
#20412=CARTESIAN_POINT ( 'NONE',  ( 3.500000000000001332, 17.50000000000002132, -116.1547308033774328 ) ) ;
#20413=VECTOR ( 'NONE', #5644, 1000.000000000000000 ) ;
#20415=LINE ( 'NONE', #26585, #5723 ) ;
#20416=CARTESIAN_POINT ( 'NONE',  ( -3.500000000000001332, 17.50000000000001421, -54.65473080337743284 ) ) ;
#20419=CARTESIAN_POINT ( 'NONE',  ( 3.310556943750001313, 17.50000000000001776, -82.26410580289947916 ) ) ;
#20422=ORIENTED_EDGE ( 'NONE', *, *, #6889, .F. ) ;
#20423=AXIS2_PLACEMENT_3D ( 'NONE', #6238, #32391, #6026 ) ;
#20426=CARTESIAN_POINT ( 'NONE',  ( 0.9378221735089281585, 14.00000000000002132, -115.6663226036829997 ) ) ;
#20428=CARTESIAN_POINT ( 'NONE',  ( 1.655278471874998436, 14.63297358603755072, -124.4307724695661364 ) ) ;
#20429=CARTESIAN_POINT ( 'NONE',  ( 4.648177544792955347E-16, 21.00000000000001776, -95.21098080242150274 ) ) ;
#20430=CARTESIAN_POINT ( 'NONE',  ( -7.022189441860112050E-16, 13.67729811471671830, -55.60160580289947063 ) ) ;
#20431=CARTESIAN_POINT ( 'NONE',  ( -1.655278471875002211, 14.63297358603755072, -112.6849391362327992 ) ) ;
#20433=VERTEX_POINT ( 'NONE', #18868 ) ;
#20434=CARTESIAN_POINT ( 'NONE',  ( 3.500000000000001332, 17.50000000000002132, -124.1547308033774186 ) ) ;
#20435=CARTESIAN_POINT ( 'NONE',  ( -1.655278471874999990, 20.36702641396248481, -40.93077246956614346 ) ) ;
#20436=CARTESIAN_POINT ( 'NONE',  ( 3.310556943750001313, 17.50000000000001421, -68.35160580289947063 ) ) ;
#20437=CARTESIAN_POINT ( 'NONE',  ( 1.749999999999998224, 14.46891108675448478, -118.6276474690881741 ) ) ;
#20438=CARTESIAN_POINT ( 'NONE',  ( -1.655278471874999990, 20.36702641396249547, -103.9307724695661364 ) ) ;
#20439=CARTESIAN_POINT ( 'NONE',  ( -0.9378221735089310451, 14.00000000000001066, -47.44938900211595012 ) ) ;
#20442=CARTESIAN_POINT ( 'NONE',  ( 1.750000000000001110, 20.53108891324555074, -67.29431413575484555 ) ) ;
#20444=CARTESIAN_POINT ( 'NONE',  ( -1.655278471874999990, 20.36702641396248481, -35.93077246956613635 ) ) ;
#20445=( BOUNDED_CURVE ( )  B_SPLINE_CURVE ( 2, ( #18239, #36987, #33790, #1044, #33994, #21225, #34196, #5056, #18035 ),
 .UNSPECIFIED., .F., .T. ) 
 B_SPLINE_CURVE_WITH_KNOTS ( ( 3, 2, 2, 2, 3 ),
 ( 0.6770833333333333703, 0.6777777777777778123, 0.6791666666666666963, 0.6805555555555555802, 0.6812500000000000222 ),
 .UNSPECIFIED. ) 
 CURVE ( )  GEOMETRIC_REPRESENTATION_ITEM ( )  RATIONAL_B_SPLINE_CURVE ( ( 0.9330127018922194093, 0.9330127018922194093, 1.000000000000000000, 0.8660254037844387076, 1.000000000000000000, 0.8660254037844387076, 1.000000000000000000, 0.9330127018922194093, 0.9330127018922194093 ) ) 
 REPRESENTATION_ITEM ( '' )  );
#20447=CARTESIAN_POINT ( 'NONE',  ( 1.655278471875001101, 20.36702641396249192, -95.18493913623279923 ) ) ;
#20448=CARTESIAN_POINT ( 'NONE',  ( -7.424026671074350129E-16, 13.45854811567263454, -61.40473080337741862 ) ) ;
#20450=CARTESIAN_POINT ( 'NONE',  ( -7.022189441860112050E-16, 13.67729811471672896, -111.6016058028994706 ) ) ;
#20451=CARTESIAN_POINT ( 'NONE',  ( -1.655278471874999990, 20.36702641396248481, -41.01827246956612782 ) ) ;
#20458=CARTESIAN_POINT ( 'NONE',  ( -7.022189441860112050E-16, 13.67729811471672541, -95.51410580289945074 ) ) ;
#20459=CARTESIAN_POINT ( 'NONE',  ( 3.500000000000001332, 17.50000000000001066, -39.15473080337743284 ) ) ;
#20461=VERTEX_POINT ( 'NONE', #2703 ) ;
#20462=DIRECTION ( 'NONE',  ( 0.000000000000000000, 1.000000000000000000, 0.000000000000000000 ) ) ;
#20466=EDGE_CURVE ( 'NONE', #22382, #8132, #260, .T. ) ;
#20470=CARTESIAN_POINT ( 'NONE',  ( 3.310556943750001313, 17.50000000000001066, -30.26410580289948271 ) ) ;
#20480=AXIS2_PLACEMENT_3D ( 'NONE', #40940, #15633, #1812 ) ;
#20482=EDGE_CURVE ( 'NONE', #32798, #7014, #7276, .T. ) ;
#20483=CARTESIAN_POINT ( 'NONE',  ( 3.310556943750001313, 19.41135094264167549, -141.1807724695661648 ) ) ;
#20484=CARTESIAN_POINT ( 'NONE',  ( 0.000000000000000000, 21.00000000000002487, -149.5231586289125687 ) ) ;
#20485=CARTESIAN_POINT ( 'NONE',  ( -1.655278471874999990, 20.36702641396249902, -131.0182724695661136 ) ) ;
#20486=CARTESIAN_POINT ( 'NONE',  ( 3.500000000000000000, 15.47927405783632082, -26.54431413575483845 ) ) ;
#20488=CARTESIAN_POINT ( 'NONE',  ( 3.500000000000000000, 15.47927405783632082, -43.23806413671076143 ) ) ;
#20490=CARTESIAN_POINT ( 'NONE',  ( 1.750000000000001110, 20.53108891324556140, -132.2943141357548598 ) ) ;
#20491=CARTESIAN_POINT ( 'NONE',  ( -1.655278471874999990, 20.36702641396249547, -115.9307724695661364 ) ) ;
#20494=CARTESIAN_POINT ( 'NONE',  ( 1.749999999999998224, 14.46891108675448123, -87.62764746908817415 ) ) ;
#20495=CARTESIAN_POINT ( 'NONE',  ( -0.9378221735089310451, 14.00000000000002132, -92.44938900211593591 ) ) ;
#20496=CARTESIAN_POINT ( 'NONE',  ( 3.310556943749999981, 15.58864905735836537, -55.34743913623281486 ) ) ;
#20497=CARTESIAN_POINT ( 'NONE',  ( -3.310556943750002645, 15.58864905735837780, -110.7682724695661420 ) ) ;
#20498=CARTESIAN_POINT ( 'NONE',  ( -1.394453263437886604E-15, 14.00000000000001776, -85.71098080242151696 ) ) ;
#20500=CARTESIAN_POINT ( 'NONE',  ( 1.655278471874998436, 14.63297358603755072, -129.5182724695661136 ) ) ;
#20503=CARTESIAN_POINT ( 'NONE',  ( 0.9378221735089281585, 14.00000000000002309, -124.3600726046389155 ) ) ;
#20505=CARTESIAN_POINT ( 'NONE',  ( -1.655278471875002211, 14.63297358603754361, -66.68493913623279923 ) ) ;
#20509=CARTESIAN_POINT ( 'NONE',  ( 2.340729813953370519E-16, 21.32270188528331190, -78.10160580289944221 ) ) ;
#20514=CARTESIAN_POINT ( 'NONE',  ( 1.655278471874998436, 14.63297358603754006, -43.43077246956614346 ) ) ;
#20515=CARTESIAN_POINT ( 'NONE',  ( 1.655278471874998436, 14.63297358603754716, -99.43077246956613635 ) ) ;
#20516=DIRECTION ( 'NONE',  ( 0.000000000000000000, 1.000000000000000000, 0.000000000000000000 ) ) ;
#20519=ORIENTED_EDGE ( 'NONE', *, *, #36536, .F. ) ;
#20521=EDGE_CURVE ( 'NONE', #14839, #5239, #27962, .T. ) ;
#20523=CARTESIAN_POINT ( 'NONE',  ( 1.655278471874998436, 14.63297358603754184, -54.43077246956613635 ) ) ;
#20524=ORIENTED_EDGE ( 'NONE', *, *, #37617, .F. ) ;
#20526=ORIENTED_EDGE ( 'NONE', *, *, #29744, .T. ) ;
#20527=CARTESIAN_POINT ( 'NONE',  ( -3.500000000000001332, 17.50000000000001776, -98.65473080337743284 ) ) ;
#20528=CARTESIAN_POINT ( 'NONE',  ( 4.648177544792955347E-16, 21.00000000000001421, -51.90473080337743284 ) ) ;
#20530=DIRECTION ( 'NONE',  ( -0.000000000000000000, 1.259100132267607459E-16, -1.000000000000000000 ) ) ;
#20531=ORIENTED_EDGE ( 'NONE', *, *, #8557, .F. ) ;
#20532=CARTESIAN_POINT ( 'NONE',  ( 3.500000000000001776, 19.52072594216370405, -44.37764746908817415 ) ) ;
#20536=CARTESIAN_POINT ( 'NONE',  ( 1.655278471875001101, 20.36702641396248481, -27.18493913623279568 ) ) ;
#20537=CARTESIAN_POINT ( 'NONE',  ( -3.310556943750001313, 17.50000000000001066, -23.85160580289946708 ) ) ;
#20538=CARTESIAN_POINT ( 'NONE',  ( -3.310556943750000425, 19.41135094264166483, -80.93493913623279923 ) ) ;
#20539=CARTESIAN_POINT ( 'NONE',  ( 3.310556943749999981, 15.58864905735837425, -135.3474391362328220 ) ) ;
#20544=CARTESIAN_POINT ( 'NONE',  ( 3.310556943750001313, 19.41135094264166838, -127.2682724695661136 ) ) ;
#20545=CARTESIAN_POINT ( 'NONE',  ( 0.000000000000000000, 21.00000000000002487, -149.5231586289125687 ) ) ;
#20546=CARTESIAN_POINT ( 'NONE',  ( -1.655278471875002211, 14.63297358603754716, -85.59743913623279354 ) ) ;
#20549=CARTESIAN_POINT ( 'NONE',  ( 4.648177544792955347E-16, 21.00000000000001776, -88.90473080337740441 ) ) ;
#20551=CARTESIAN_POINT ( 'NONE',  ( -1.750000000000002220, 14.46891108675448123, -70.48806413671076143 ) ) ;
#20552=CARTESIAN_POINT ( 'NONE',  ( 2.340729813953370519E-16, 21.32270188528331190, -53.10160580289946353 ) ) ;
#20554=CARTESIAN_POINT ( 'NONE',  ( -0.9378221735089291577, 21.00000000000001421, -67.86007260463890134 ) ) ;
#20557=CARTESIAN_POINT ( 'NONE',  ( -3.310556943750000425, 19.41135094264166483, -79.93493913623281344 ) ) ;
#20558=CARTESIAN_POINT ( 'NONE',  ( 3.310556943750001313, 17.50000000000002487, -142.3516058028994564 ) ) ;
#20560=CARTESIAN_POINT ( 'NONE',  ( -1.655278471874999990, 20.36702641396249547, -106.9307724695661364 ) ) ;
#20561=CARTESIAN_POINT ( 'NONE',  ( -1.655278471874999990, 20.36702641396248836, -72.93077246956613635 ) ) ;
#20562=CARTESIAN_POINT ( 'NONE',  ( -1.750000000000002220, 14.46891108675448478, -100.7943141357548456 ) ) ;
#20564=CARTESIAN_POINT ( 'NONE',  ( 3.310556943749999981, 15.58864905735836892, -94.43493913623279923 ) ) ;
#20565=CARTESIAN_POINT ( 'NONE',  ( 2.474675557024783212E-16, 21.54145188432739744, -99.90473080337746126 ) ) ;
#20569=CARTESIAN_POINT ( 'NONE',  ( -3.310556943750000425, 19.41135094264166483, -59.84743913623280775 ) ) ;
#20571=CARTESIAN_POINT ( 'NONE',  ( 1.655278471875001101, 20.36702641396249547, -116.0974391362327935 ) ) ;
#20572=DIRECTION ( 'NONE',  ( -0.000000000000000000, 1.259100132267607459E-16, -1.000000000000000000 ) ) ;
#20573=( BOUNDED_CURVE ( )  B_SPLINE_CURVE ( 2, ( #4241, #10630, #36356, #17225, #33158, #19766, #29969, #32949, #412 ),
 .UNSPECIFIED., .F., .F. ) 
 B_SPLINE_CURVE_WITH_KNOTS ( ( 3, 2, 2, 2, 3 ),
 ( 0.9104166666666666519, 0.9111111111111110938, 0.9124999999999999778, 0.9138888888888888618, 0.9145833333333333037 ),
 .UNSPECIFIED. ) 
 CURVE ( )  GEOMETRIC_REPRESENTATION_ITEM ( )  RATIONAL_B_SPLINE_CURVE ( ( 0.9330127018922194093, 0.9330127018922194093, 1.000000000000000000, 0.8660254037844387076, 1.000000000000000000, 0.8660254037844387076, 1.000000000000000000, 0.9330127018922194093, 0.9330127018922194093 ) ) 
 REPRESENTATION_ITEM ( '' )  );
#20576=( BOUNDED_CURVE ( )  B_SPLINE_CURVE ( 2, ( #35944, #40771, #6809, #5040, #18018, #14831, #19783, #37178, #3616 ),
 .UNSPECIFIED., .F., .T. ) 
 B_SPLINE_CURVE_WITH_KNOTS ( ( 3, 2, 2, 2, 3 ),
 ( 0.002083333333333334605, 0.002777777777777777884, 0.004166666666666666609, 0.005555555555555555768, 0.006250000000000000347 ),
 .UNSPECIFIED. ) 
 CURVE ( )  GEOMETRIC_REPRESENTATION_ITEM ( )  RATIONAL_B_SPLINE_CURVE ( ( 0.9330127018922192983, 0.9330127018922194093, 1.000000000000000000, 0.8660254037844387076, 1.000000000000000000, 0.8660254037844387076, 1.000000000000000000, 0.9330127018922192983, 0.9330127018922194093 ) ) 
 REPRESENTATION_ITEM ( '' )  );
#20577=ORIENTED_EDGE ( 'NONE', *, *, #4550, .T. ) ;
#20581=ADVANCED_FACE ( 'NONE', ( #29262 ), #38438, .T. ) ;
#20582=CARTESIAN_POINT ( 'NONE',  ( -1.655278471874999990, 20.36702641396248836, -68.93077246956613635 ) ) ;
#20584=ORIENTED_EDGE ( 'NONE', *, *, #38832, .F. ) ;
#20585=DIRECTION ( 'NONE',  ( 0.000000000000000000, 1.000000000000000000, 0.000000000000000000 ) ) ;
#20586=CARTESIAN_POINT ( 'NONE',  ( 0.000000000000000000, 17.50000000000002487, -149.5231586289125687 ) ) ;
#20588=CARTESIAN_POINT ( 'NONE',  ( 4.648177544792955347E-16, 21.00000000000001776, -84.21098080242150274 ) ) ;
#20589=VECTOR ( 'NONE', #21282, 1000.000000000000000 ) ;
#20592=CARTESIAN_POINT ( 'NONE',  ( 2.340729813953370519E-16, 21.32270188528332255, -134.0141058028994507 ) ) ;
#20594=CARTESIAN_POINT ( 'NONE',  ( -3.310556943750000425, 19.41135094264165772, -44.93493913623280633 ) ) ;
#20596=CARTESIAN_POINT ( 'NONE',  ( -3.310556943750001313, 17.50000000000001066, -40.85160580289947063 ) ) ;
#20597=CARTESIAN_POINT ( 'NONE',  ( -3.310556943750000425, 19.41135094264166483, -97.93493913623278502 ) ) ;
#20599=CARTESIAN_POINT ( 'NONE',  ( 3.310556943749999981, 15.58864905735836004, -23.34743913623281486 ) ) ;
#20600=CARTESIAN_POINT ( 'NONE',  ( 4.648177544792955347E-16, 21.00000000000002132, -110.9047308033774186 ) ) ;
#20601=CARTESIAN_POINT ( 'NONE',  ( -3.500000000000000888, 19.52072594216371115, -95.04431413575484555 ) ) ;
#20602=CARTESIAN_POINT ( 'NONE',  ( 0.000000000000000000, 21.00000000000002487, -149.5231586289125687 ) ) ;
#20603=CARTESIAN_POINT ( 'NONE',  ( 1.749999999999998224, 14.46891108675448123, -85.32139747004409003 ) ) ;
#20604=CARTESIAN_POINT ( 'NONE',  ( -3.310556943750002201, 15.58864905735837070, -67.76827246956612782 ) ) ;
#20608=CARTESIAN_POINT ( 'NONE',  ( 4.648177544792955347E-16, 21.00000000000001421, -66.90473080337743284 ) ) ;
#20609=CARTESIAN_POINT ( 'NONE',  ( 3.500000000000001776, 19.52072594216370760, -52.37764746908817415 ) ) ;
#20612=CARTESIAN_POINT ( 'NONE',  ( -0.9378221735089310451, 14.00000000000001066, -34.75563900116002714 ) ) ;
#20614=CARTESIAN_POINT ( 'NONE',  ( -1.749999999999999778, 20.53108891324554719, -44.82139747004409713 ) ) ;
#20616=CARTESIAN_POINT ( 'NONE',  ( -1.655278471874999990, 20.36702641396248481, -28.01827246956613138 ) ) ;
#20617=CARTESIAN_POINT ( 'NONE',  ( 1.749999999999998224, 14.46891108675447946, -76.32139747004410424 ) ) ;
#20618=CARTESIAN_POINT ( 'NONE',  ( -3.500000000000000000, 19.52072594216370760, -57.04431413575483845 ) ) ;
#20621=CARTESIAN_POINT ( 'NONE',  ( 4.648177544792955347E-16, 21.00000000000002132, -121.2109808024215170 ) ) ;
#20623=CARTESIAN_POINT ( 'NONE',  ( -3.310556943750000425, 19.41135094264166838, -78.84743913623279354 ) ) ;
#20625=ORIENTED_EDGE ( 'NONE', *, *, #15825, .T. ) ;
#20627=CARTESIAN_POINT ( 'NONE',  ( 4.648177544792955347E-16, 21.00000000000001421, -60.90473080337742573 ) ) ;
#20628=ORIENTED_EDGE ( 'NONE', *, *, #872, .T. ) ;
#20631=CARTESIAN_POINT ( 'NONE',  ( 3.310556943750001313, 19.41135094264166483, -86.18077246956613635 ) ) ;
#20632=ORIENTED_EDGE ( 'NONE', *, *, #2271, .F. ) ;
#20635=ADVANCED_FACE ( 'NONE', ( #22265 ), #35863, .T. ) ;
#20637=CARTESIAN_POINT ( 'NONE',  ( -1.394453263437886604E-15, 14.00000000000001066, -53.40473080337743284 ) ) ;
#20638=EDGE_CURVE ( 'NONE', #40349, #26292, #39057, .T. ) ;
#20639=CARTESIAN_POINT ( 'NONE',  ( 3.310556943750001313, 19.41135094264166838, -127.1807724695661364 ) ) ;
#20642=CARTESIAN_POINT ( 'NONE',  ( 3.310556943750001313, 17.50000000000001421, -53.35160580289946353 ) ) ;
#20643=CARTESIAN_POINT ( 'NONE',  ( 3.310556943749999981, 15.58864905735837247, -114.4349391362327850 ) ) ;
#20645=( BOUNDED_CURVE ( )  B_SPLINE_CURVE ( 2, ( #30850, #14693, #11480, #7416, #24015, #16989, #33993, #17204, #27609 ),
 .UNSPECIFIED., .F., .T. ) 
 B_SPLINE_CURVE_WITH_KNOTS ( ( 3, 2, 2, 2, 3 ),
 ( 0.1562500000000000000, 0.1569444444444444420, 0.1583333333333333259, 0.1597222222222222099, 0.1604166666666666796 ),
 .UNSPECIFIED. ) 
 CURVE ( )  GEOMETRIC_REPRESENTATION_ITEM ( )  RATIONAL_B_SPLINE_CURVE ( ( 0.9330127018922194093, 0.9330127018922194093, 1.000000000000000000, 0.8660254037844387076, 1.000000000000000000, 0.8660254037844387076, 1.000000000000000000, 0.9330127018922180770, 0.9330127018922194093 ) ) 
 REPRESENTATION_ITEM ( '' )  );
#20646=CARTESIAN_POINT ( 'NONE',  ( 1.749999999999998224, 14.46891108675448656, -123.3213974700441042 ) ) ;
#20647=CARTESIAN_POINT ( 'NONE',  ( -3.310556943750000425, 19.41135094264165772, -40.84743913623280775 ) ) ;
#20649=CARTESIAN_POINT ( 'NONE',  ( -3.310556943750000425, 19.41135094264166128, -67.93493913623281344 ) ) ;
#20650=CARTESIAN_POINT ( 'NONE',  ( -3.500000000000001332, 17.50000000000002132, -117.9609808024215170 ) ) ;
#20651=CARTESIAN_POINT ( 'NONE',  ( -3.310556943750001313, 17.50000000000001776, -97.76410580289947916 ) ) ;
#20653=DIRECTION ( 'NONE',  ( -0.000000000000000000, 1.259100132267607459E-16, -1.000000000000000000 ) ) ;
#20656=CARTESIAN_POINT ( 'NONE',  ( 3.500000000000001776, 19.52072594216370760, -69.37764746908817415 ) ) ;
#20657=CARTESIAN_POINT ( 'NONE',  ( 4.648177544792955347E-16, 21.00000000000001066, -44.21098080242150985 ) ) ;
#20658=CARTESIAN_POINT ( 'NONE',  ( -3.310556943750002645, 15.58864905735836537, -31.68077246956614701 ) ) ;
#20659=CARTESIAN_POINT ( 'NONE',  ( 3.310556943750001313, 19.41135094264166483, -91.26827246956614204 ) ) ;
#20660=CARTESIAN_POINT ( 'NONE',  ( 2.474675557024783212E-16, 21.54145188432739388, -61.90473080337742573 ) ) ;
#20661=CARTESIAN_POINT ( 'NONE',  ( 7.785697387528201340E-15, 14.00000000000002487, -137.7109808024215170 ) ) ;
#20662=CARTESIAN_POINT ( 'NONE',  ( 1.655278471875001101, 20.36702641396249547, -111.1849391362327992 ) ) ;
#20663=CARTESIAN_POINT ( 'NONE',  ( -3.310556943750002201, 15.58864905735836714, -45.76827246956613493 ) ) ;
#20670=EDGE_CURVE ( 'NONE', #38828, #12815, #32880, .T. ) ;
#20671=CARTESIAN_POINT ( 'NONE',  ( 2.340729813953370519E-16, 21.32270188528331190, -91.01410580289947916 ) ) ;
#20672=CARTESIAN_POINT ( 'NONE',  ( -1.394453263437886604E-15, 14.00000000000001066, -36.40473080337743284 ) ) ;
#20674=EDGE_LOOP ( 'NONE', ( #5093, #7136, #28239, #27835 ) ) ;
#20675=CARTESIAN_POINT ( 'NONE',  ( 0.000000000000000000, 17.50000000000002487, -149.5231586289125687 ) ) ;
#20678=AXIS2_PLACEMENT_3D ( 'NONE', #23398, #23826, #4464 ) ;
#20679=FACE_OUTER_BOUND ( 'NONE', #19406, .T. ) ;
#20683=ORIENTED_EDGE ( 'NONE', *, *, #20670, .F. ) ;
#20684=CARTESIAN_POINT ( 'NONE',  ( 4.648177544792955347E-16, 21.00000000000002487, -131.2109808024214885 ) ) ;
#20690=EDGE_CURVE ( 'NONE', #5144, #14962, #33933, .T. ) ;
#20693=CARTESIAN_POINT ( 'NONE',  ( 3.310556943749999981, 15.58864905735837780, -141.3474391362327935 ) ) ;
#20694=CARTESIAN_POINT ( 'NONE',  ( 1.750000000000001110, 20.53108891324555785, -109.9880641367107614 ) ) ;
#20695=CYLINDRICAL_SURFACE ( 'NONE', #28834, 3.499999999999999556 ) ;
#20696=CARTESIAN_POINT ( 'NONE',  ( -3.310556943750001313, 17.50000000000002487, -132.8516058028994564 ) ) ;
#20697=CARTESIAN_POINT ( 'NONE',  ( -3.500000000000001332, 17.50000000000001066, -29.96098080242151696 ) ) ;
#20699=CARTESIAN_POINT ( 'NONE',  ( 3.500000000000000000, 15.47927405783633503, -141.2380641367107614 ) ) ;
#20700=( BOUNDED_CURVE ( )  B_SPLINE_CURVE ( 2, ( #22311, #9561, #35502, #36338, #26150, #396, #20180, #4005, #32933 ),
 .UNSPECIFIED., .F., .T. ) 
 B_SPLINE_CURVE_WITH_KNOTS ( ( 3, 2, 2, 2, 3 ),
 ( 0.006250000000000000347, 0.006944444444444444059, 0.008333333333333333218, 0.009722222222222222376, 0.01041666666666666782 ),
 .UNSPECIFIED. ) 
 CURVE ( )  GEOMETRIC_REPRESENTATION_ITEM ( )  RATIONAL_B_SPLINE_CURVE ( ( 0.9330127018922194093, 0.9330127018922194093, 1.000000000000000000, 0.8660254037844387076, 1.000000000000000000, 0.8660254037844387076, 1.000000000000000000, 0.9330127018922191873, 0.9330127018922192983 ) ) 
 REPRESENTATION_ITEM ( '' )  );
#20702=CARTESIAN_POINT ( 'NONE',  ( 4.648177544792955347E-16, 21.00000000000002132, -123.2109808024214885 ) ) ;
#20704=CARTESIAN_POINT ( 'NONE',  ( 2.474675557024783212E-16, 21.54145188432740810, -134.2109808024214885 ) ) ;
#20705=CARTESIAN_POINT ( 'NONE',  ( -3.310556943750000425, 19.41135094264166838, -118.8474391362327935 ) ) ;
#20708=CARTESIAN_POINT ( 'NONE',  ( 1.750000000000001110, 20.53108891324555429, -86.29431413575483134 ) ) ;
#20711=CARTESIAN_POINT ( 'NONE',  ( 2.340729813953370519E-16, 21.32270188528330834, -52.01410580289947205 ) ) ;
#20712=CARTESIAN_POINT ( 'NONE',  ( 2.340729813953370519E-16, 21.32270188528331900, -104.1016058028994422 ) ) ;
#20713=CARTESIAN_POINT ( 'NONE',  ( -0.9378221735088960731, 14.00000000000000000, -93.75563900116003424 ) ) ;
#20714=CARTESIAN_POINT ( 'NONE',  ( -0.9378221735089310451, 14.00000000000001599, -79.75563900116002003 ) ) ;
#20717=CARTESIAN_POINT ( 'NONE',  ( 3.310556943750001313, 17.50000000000002487, -130.3516058028994564 ) ) ;
#20720=CARTESIAN_POINT ( 'NONE',  ( 4.286263797015737581E-16, 14.00000000000002487, -149.5231586289125687 ) ) ;
#20721=CARTESIAN_POINT ( 'NONE',  ( 3.500000000000001332, 17.50000000000001421, -58.46098080242151696 ) ) ;
#20723=CARTESIAN_POINT ( 'NONE',  ( 1.655278471875001101, 20.36702641396248836, -63.18493913623279923 ) ) ;
#20724=ORIENTED_EDGE ( 'NONE', *, *, #6590, .F. ) ;
#20725=CARTESIAN_POINT ( 'NONE',  ( -3.310556943750002201, 15.58864905735837247, -81.76827246956614204 ) ) ;
#20728=CARTESIAN_POINT ( 'NONE',  ( 0.9378221735089281585, 14.00000000000001066, -44.66632260368299256 ) ) ;
#20731=CARTESIAN_POINT ( 'NONE',  ( 3.310556943750001313, 19.41135094264166128, -37.18077246956613635 ) ) ;
#20732=CARTESIAN_POINT ( 'NONE',  ( -7.022189441860112050E-16, 13.67729811471672541, -102.5141058028994649 ) ) ;
#20735=ORIENTED_EDGE ( 'NONE', *, *, #32932, .F. ) ;
#20737=VERTEX_POINT ( 'NONE', #39899 ) ;
#20739=CARTESIAN_POINT ( 'NONE',  ( -3.310556943750001313, 17.50000000000001421, -51.76410580289947205 ) ) ;
#20740=EDGE_LOOP ( 'NONE', ( #19013, #25693, #10936, #18640 ) ) ;
#20741=ORIENTED_EDGE ( 'NONE', *, *, #7117, .F. ) ;
#20742=CARTESIAN_POINT ( 'NONE',  ( -1.749999999999999778, 20.53108891324554719, -43.82139747004409713 ) ) ;
#20743=CARTESIAN_POINT ( 'NONE',  ( -1.750000000000002220, 14.46891108675448301, -91.48806413671076143 ) ) ;
#20745=DIRECTION ( 'NONE',  ( 0.000000000000000000, 1.000000000000000000, 0.000000000000000000 ) ) ;
#20750=CARTESIAN_POINT ( 'NONE',  ( -7.424026671074350129E-16, 13.45854811567263276, -44.71098080242151696 ) ) ;
#20753=EDGE_CURVE ( 'NONE', #18164, #41382, #33089, .T. ) ;
#20755=CARTESIAN_POINT ( 'NONE',  ( -1.655278471874999990, 20.36702641396248481, -30.01827246956613493 ) ) ;
#20758=CARTESIAN_POINT ( 'NONE',  ( 3.310556943749999981, 15.58864905735836892, -84.43493913623278502 ) ) ;
#20759=CARTESIAN_POINT ( 'NONE',  ( 1.655278471874998436, 14.63297358603755072, -131.4307724695661364 ) ) ;
#20762=CARTESIAN_POINT ( 'NONE',  ( 1.749999999999998224, 14.46891108675447235, -24.32139747004409713 ) ) ;
#20763=CARTESIAN_POINT ( 'NONE',  ( 3.310556943749999981, 15.58864905735837247, -120.4349391362327850 ) ) ;
#20764=CYLINDRICAL_SURFACE ( 'NONE', #26179, 3.499999999999999556 ) ;
#20765=CARTESIAN_POINT ( 'NONE',  ( -3.310556943750002645, 15.58864905735837247, -85.68077246956613635 ) ) ;
#20766=FACE_OUTER_BOUND ( 'NONE', #39723, .T. ) ;
#20767=CARTESIAN_POINT ( 'NONE',  ( 4.648177544792955347E-16, 21.00000000000002132, -114.9047308033774186 ) ) ;
#20768=CARTESIAN_POINT ( 'NONE',  ( -3.695301148110399846E-14, 21.00000000000002132, -123.9047308033773902 ) ) ;
#20769=CARTESIAN_POINT ( 'NONE',  ( -7.424026671074350129E-16, 13.45854811567263454, -70.40473080337743284 ) ) ;
#20771=CARTESIAN_POINT ( 'NONE',  ( -1.655278471874999990, 20.36702641396248836, -55.01827246956612782 ) ) ;
#20773=CYLINDRICAL_SURFACE ( 'NONE', #35334, 3.499999999999999556 ) ;
#20774=CARTESIAN_POINT ( 'NONE',  ( -1.394453263437886604E-15, 14.00000000000001066, -48.71098080242150985 ) ) ;
#20775=CARTESIAN_POINT ( 'NONE',  ( -3.310556943750002645, 15.58864905735837247, -81.76827246956614204 ) ) ;
#20776=CARTESIAN_POINT ( 'NONE',  ( 2.340729813953370519E-16, 21.32270188528332255, -141.1016058028994564 ) ) ;
#20778=CARTESIAN_POINT ( 'NONE',  ( 1.655278471874998436, 14.63297358603754716, -104.4307724695661364 ) ) ;
#20779=CARTESIAN_POINT ( 'NONE',  ( -3.310556943750000425, 19.41135094264166483, -77.84743913623280775 ) ) ;
#20780=CARTESIAN_POINT ( 'NONE',  ( 4.648177544792955347E-16, 21.00000000000001776, -97.21098080242148853 ) ) ;
#20782=CARTESIAN_POINT ( 'NONE',  ( 3.310556943750001313, 17.50000000000001776, -96.35160580289945642 ) ) ;
#20785=CARTESIAN_POINT ( 'NONE',  ( 0.9378221735089281585, 14.00000000000001776, -91.66632260368298546 ) ) ;
#20788=CARTESIAN_POINT ( 'NONE',  ( -7.022189441860112050E-16, 13.67729811471672186, -61.51410580289947205 ) ) ;
#20790=CARTESIAN_POINT ( 'NONE',  ( -7.022189441860112050E-16, 13.67729811471672718, -115.5141058028994792 ) ) ;
#20791=CARTESIAN_POINT ( 'NONE',  ( 4.286263797015737581E-16, 14.00000000000002487, -149.5231586289125687 ) ) ;
#20793=ORIENTED_EDGE ( 'NONE', *, *, #38428, .T. ) ;
#20795=ORIENTED_EDGE ( 'NONE', *, *, #30881, .F. ) ;
#20797=CARTESIAN_POINT ( 'NONE',  ( -1.655278471875002211, 14.63297358603754539, -68.59743913623280775 ) ) ;
#20804=CARTESIAN_POINT ( 'NONE',  ( 3.310556943750001313, 19.41135094264167549, -134.1807724695661364 ) ) ;
#20807=CARTESIAN_POINT ( 'NONE',  ( 2.340729813953370519E-16, 21.32270188528330479, -43.10160580289947063 ) ) ;
#20809=CARTESIAN_POINT ( 'NONE',  ( 3.310556943750001313, 17.50000000000001066, -34.35160580289946353 ) ) ;
#20810=CARTESIAN_POINT ( 'NONE',  ( 2.340729813953370519E-16, 21.32270188528331190, -98.10160580289947063 ) ) ;
#20813=CARTESIAN_POINT ( 'NONE',  ( -3.310556943750002645, 15.58864905735837958, -141.7682724695661420 ) ) ;
#20815=CARTESIAN_POINT ( 'NONE',  ( -1.749999999999999778, 20.53108891324555429, -94.12764746908815994 ) ) ;
#20817=CARTESIAN_POINT ( 'NONE',  ( 0.000000000000000000, 17.50000000000002487, -149.5231586289125687 ) ) ;
#20818=CARTESIAN_POINT ( 'NONE',  ( -3.500000000000002220, 15.47927405783632793, -83.57139747004411845 ) ) ;
#20819=EDGE_CURVE ( 'NONE', #14962, #10652, #38266, .T. ) ;
#20820=CARTESIAN_POINT ( 'NONE',  ( 2.340729813953370519E-16, 21.32270188528331190, -72.10160580289947063 ) ) ;
#20825=CARTESIAN_POINT ( 'NONE',  ( 1.749999999999998224, 14.46891108675447590, -47.62764746908818125 ) ) ;
#20826=CARTESIAN_POINT ( 'NONE',  ( 0.000000000000000000, 21.00000000000002487, -149.5231586289125687 ) ) ;
#20827=DIRECTION ( 'NONE',  ( -0.000000000000000000, 1.259100132267607459E-16, -1.000000000000000000 ) ) ;
#20828=( BOUNDED_CURVE ( )  B_SPLINE_CURVE ( 2, ( #10118, #3935, #3314, #29669, #16102, #9710, #22671, #3724, #3515 ),
 .UNSPECIFIED., .F., .F. ) 
 B_SPLINE_CURVE_WITH_KNOTS ( ( 3, 2, 2, 2, 3 ),
 ( 0.01874999999999999931, 0.01944444444444444475, 0.02083333333333333218, 0.02222222222222222307, 0.02291666666666666852 ),
 .UNSPECIFIED. ) 
 CURVE ( )  GEOMETRIC_REPRESENTATION_ITEM ( )  RATIONAL_B_SPLINE_CURVE ( ( 0.9330127018922194093, 0.9330127018922194093, 1.000000000000000000, 0.8660254037844387076, 1.000000000000000000, 0.8660254037844387076, 1.000000000000000000, 0.9330127018922191873, 0.9330127018922194093 ) ) 
 REPRESENTATION_ITEM ( '' )  );
#20829=CARTESIAN_POINT ( 'NONE',  ( 0.9378221735089300459, 21.00000000000001776, -95.25563900116003424 ) ) ;
#20830=VERTEX_POINT ( 'NONE', #30535 ) ;
#20831=CARTESIAN_POINT ( 'NONE',  ( -1.749999999999999778, 20.53108891324555785, -115.8213974700440900 ) ) ;
#20836=CARTESIAN_POINT ( 'NONE',  ( 3.310556943750001313, 19.41135094264166838, -75.18077246956613635 ) ) ;
#20837=CARTESIAN_POINT ( 'NONE',  ( 1.750000000000001110, 20.53108891324555429, -98.29431413575484555 ) ) ;
#20841=CARTESIAN_POINT ( 'NONE',  ( 2.340729813953370519E-16, 21.32270188528331190, -85.01410580289949337 ) ) ;
#20847=ORIENTED_EDGE ( 'NONE', *, *, #9770, .F. ) ;
#20848=PLANE ( 'NONE',  #323 ) ;
#20849=CARTESIAN_POINT ( 'NONE',  ( -1.655278471874999990, 20.36702641396248836, -53.01827246956612782 ) ) ;
#20850=CARTESIAN_POINT ( 'NONE',  ( 1.655278471874998436, 14.63297358603754894, -115.5182724695661278 ) ) ;
#20851=ORIENTED_EDGE ( 'NONE', *, *, #28767, .F. ) ;
#20852=CARTESIAN_POINT ( 'NONE',  ( -1.749999999999999778, 20.53108891324555785, -123.8213974700440900 ) ) ;
#20853=CARTESIAN_POINT ( 'NONE',  ( -1.655278471875002211, 14.63297358603754184, -40.59743913623280065 ) ) ;
#20854=CARTESIAN_POINT ( 'NONE',  ( -7.022189441860112050E-16, 13.67729811471671830, -65.60160580289945642 ) ) ;
#20855=CARTESIAN_POINT ( 'NONE',  ( -1.749999999999999778, 20.53108891324555785, -111.1276474690881741 ) ) ;
#20857=CARTESIAN_POINT ( 'NONE',  ( -1.655278471875002211, 14.63297358603754894, -95.59743913623280775 ) ) ;
#20858=CARTESIAN_POINT ( 'NONE',  ( -3.500000000000002220, 15.47927405783632437, -47.57139747004410424 ) ) ;
#20859=EDGE_CURVE ( 'NONE', #5960, #41241, #4868, .T. ) ;
#20863=CARTESIAN_POINT ( 'NONE',  ( -1.749999999999999778, 20.53108891324555074, -62.12764746908818125 ) ) ;
#20864=DIRECTION ( 'NONE',  ( -0.000000000000000000, 1.259100132267607459E-16, -1.000000000000000000 ) ) ;
#20865=CARTESIAN_POINT ( 'NONE',  ( -7.022189441860112050E-16, 13.67729811471671475, -31.51410580289946850 ) ) ;
#20866=ADVANCED_FACE ( 'NONE', ( #17150 ), #24614, .T. ) ;
#20867=CARTESIAN_POINT ( 'NONE',  ( 3.310556943750001313, 17.50000000000001776, -89.35160580289947063 ) ) ;
#20868=CARTESIAN_POINT ( 'NONE',  ( -7.424026671074350129E-16, 13.45854811567263276, -51.40473080337742573 ) ) ;
#20869=DIRECTION ( 'NONE',  ( 0.000000000000000000, 1.000000000000000000, 0.000000000000000000 ) ) ;
#20870=CARTESIAN_POINT ( 'NONE',  ( 1.655278471875001101, 20.36702641396249547, -110.1849391362327992 ) ) ;
#20871=CARTESIAN_POINT ( 'NONE',  ( -3.310556943750001313, 17.50000000000001066, -35.85160580289946353 ) ) ;
#20877=CARTESIAN_POINT ( 'NONE',  ( 2.340729813953370519E-16, 21.32270188528331190, -95.01410580289946495 ) ) ;
#20880=VERTEX_POINT ( 'NONE', #17777 ) ;
#20881=CARTESIAN_POINT ( 'NONE',  ( 0.9378221735089300459, 21.00000000000001421, -57.25563900116002714 ) ) ;
#20883=CARTESIAN_POINT ( 'NONE',  ( 0.000000000000000000, 21.00000000000002487, -149.5231586289125687 ) ) ;
#20889=DIRECTION ( 'NONE',  ( -0.000000000000000000, 1.259100132267607459E-16, -1.000000000000000000 ) ) ;
#20893=ORIENTED_EDGE ( 'NONE', *, *, #24616, .T. ) ;
#20894=FACE_OUTER_BOUND ( 'NONE', #15508, .T. ) ;
#20896=CARTESIAN_POINT ( 'NONE',  ( 2.340729813953370519E-16, 21.32270188528332255, -143.0141058028994792 ) ) ;
#20897=CYLINDRICAL_SURFACE ( 'NONE', #27127, 3.499999999999999556 ) ;
#20898=CARTESIAN_POINT ( 'NONE',  ( -3.500000000000002220, 15.47927405783632615, -63.57139747004410424 ) ) ;
#20899=CARTESIAN_POINT ( 'NONE',  ( -1.655278471874999990, 20.36702641396249902, -130.0182724695661136 ) ) ;
#20900=CARTESIAN_POINT ( 'NONE',  ( -1.655278471875002211, 14.63297358603754361, -55.68493913623279212 ) ) ;
#20901=ORIENTED_EDGE ( 'NONE', *, *, #34340, .T. ) ;
#20905=CARTESIAN_POINT ( 'NONE',  ( 1.750000000000001110, 20.53108891324555785, -123.2943141357548456 ) ) ;
#20907=CARTESIAN_POINT ( 'NONE',  ( -3.500000000000000888, 19.52072594216372181, -131.0443141357548313 ) ) ;
#20908=CARTESIAN_POINT ( 'NONE',  ( 1.655278471874998436, 14.63297358603754894, -112.4307724695661506 ) ) ;
#20911=CARTESIAN_POINT ( 'NONE',  ( 1.750000000000001110, 20.53108891324555429, -87.29431413575483134 ) ) ;
#20913=CARTESIAN_POINT ( 'NONE',  ( -3.310556943750001313, 17.50000000000001421, -48.76410580289947205 ) ) ;
#20914=CARTESIAN_POINT ( 'NONE',  ( -1.655278471874999990, 20.36702641396249547, -107.0182724695661278 ) ) ;
#20915=CARTESIAN_POINT ( 'NONE',  ( -3.500000000000001332, 17.50000000000002487, -129.9609808024214885 ) ) ;
#20916=CARTESIAN_POINT ( 'NONE',  ( -3.500000000000001332, 17.50000000000001776, -79.96098080242150274 ) ) ;
#20919=CARTESIAN_POINT ( 'NONE',  ( -3.310556943750002201, 15.58864905735837780, -130.7682724695661136 ) ) ;
#20922=CARTESIAN_POINT ( 'NONE',  ( -3.500000000000002220, 15.47927405783633503, -116.8776474690881741 ) ) ;
#20923=DIRECTION ( 'NONE',  ( -0.000000000000000000, 1.259100132267607459E-16, -1.000000000000000000 ) ) ;
#20924=CARTESIAN_POINT ( 'NONE',  ( -3.310556943750001313, 17.50000000000001421, -59.85160580289947063 ) ) ;
#20927=ORIENTED_EDGE ( 'NONE', *, *, #7989, .F. ) ;
#20928=CARTESIAN_POINT ( 'NONE',  ( 1.655278471875001101, 20.36702641396249192, -82.18493913623278502 ) ) ;
#20929=ADVANCED_FACE ( 'NONE', ( #40108 ), #17365, .T. ) ;
#20930=CARTESIAN_POINT ( 'NONE',  ( 3.500000000000001332, 17.50000000000001066, -30.15473080337743994 ) ) ;
#20934=CARTESIAN_POINT ( 'NONE',  ( -1.655278471874999990, 20.36702641396248481, -40.93077246956614346 ) ) ;
#20935=CARTESIAN_POINT ( 'NONE',  ( -3.310556943750001313, 17.50000000000001776, -92.76410580289947916 ) ) ;
#20940=CARTESIAN_POINT ( 'NONE',  ( -3.310556943750001313, 17.50000000000001421, -50.76410580289947205 ) ) ;
#20941=ORIENTED_EDGE ( 'NONE', *, *, #13644, .T. ) ;
#20942=VERTEX_POINT ( 'NONE', #20767 ) ;
#20944=( BOUNDED_CURVE ( )  B_SPLINE_CURVE ( 2, ( #1671, #33800, #37403, #21235, #10826, #33365, #4858, #20612, #4233 ),
 .UNSPECIFIED., .F., .T. ) 
 B_SPLINE_CURVE_WITH_KNOTS ( ( 3, 2, 2, 2, 3 ),
 ( 0.9020833333333333481, 0.9027777777777777901, 0.9041666666666666741, 0.9055555555555555580, 0.9062500000000000000 ),
 .UNSPECIFIED. ) 
 CURVE ( )  GEOMETRIC_REPRESENTATION_ITEM ( )  RATIONAL_B_SPLINE_CURVE ( ( 0.9330127018922194093, 0.9330127018922194093, 1.000000000000000000, 0.8660254037844387076, 1.000000000000000000, 0.8660254037844387076, 1.000000000000000000, 0.9330127018922194093, 0.9330127018922194093 ) ) 
 REPRESENTATION_ITEM ( '' )  );
#20945=CARTESIAN_POINT ( 'NONE',  ( 1.750000000000001110, 20.53108891324555785, -124.9880641367107614 ) ) ;
#20950=CARTESIAN_POINT ( 'NONE',  ( 3.500000000000001332, 17.50000000000001066, -40.46098080242150985 ) ) ;
#20951=EDGE_CURVE ( 'NONE', #29973, #21640, #9215, .T. ) ;
#20953=CARTESIAN_POINT ( 'NONE',  ( 3.500000000000001332, 19.52072594216371826, -119.0713974700441042 ) ) ;
#20957=CARTESIAN_POINT ( 'NONE',  ( -7.022189441860112050E-16, 13.67729811471671475, -30.60160580289945997 ) ) ;
#20959=CARTESIAN_POINT ( 'NONE',  ( 1.655278471874998436, 14.63297358603755072, -127.4307724695661364 ) ) ;
#20963=CARTESIAN_POINT ( 'NONE',  ( 3.310556943750001313, 17.50000000000002132, -122.3516058028994706 ) ) ;
#20965=CARTESIAN_POINT ( 'NONE',  ( 3.310556943750001313, 17.50000000000001776, -84.26410580289947916 ) ) ;
#20967=CARTESIAN_POINT ( 'NONE',  ( 0.9378221735089300459, 21.00000000000001421, -64.94938900211595012 ) ) ;
#20969=CARTESIAN_POINT ( 'NONE',  ( -3.500000000000001332, 17.50000000000001421, -70.65473080337743284 ) ) ;
#20970=CARTESIAN_POINT ( 'NONE',  ( -3.310556943750002201, 15.58864905735836892, -55.76827246956612782 ) ) ;
#20972=CARTESIAN_POINT ( 'NONE',  ( -0.9378221735089310451, 14.00000000000002132, -98.75563900116003424 ) ) ;
#20973=CARTESIAN_POINT ( 'NONE',  ( 3.310556943750001313, 17.50000000000001421, -74.35160580289947063 ) ) ;
#20974=CARTESIAN_POINT ( 'NONE',  ( 3.310556943749999981, 15.58864905735837780, -139.4349391362327708 ) ) ;
#20976=CARTESIAN_POINT ( 'NONE',  ( 3.310556943749999981, 15.58864905735837070, -101.3474391362328220 ) ) ;
#20977=CARTESIAN_POINT ( 'NONE',  ( 1.655278471874998436, 14.63297358603754361, -73.43077246956613635 ) ) ;
#20979=CARTESIAN_POINT ( 'NONE',  ( 3.310556943750001313, 17.50000000000001776, -94.35160580289947063 ) ) ;
#20982=CARTESIAN_POINT ( 'NONE',  ( -1.749999999999999778, 20.53108891324555429, -81.82139747004410424 ) ) ;
#20983=CARTESIAN_POINT ( 'NONE',  ( -1.394453263437886604E-15, 14.00000000000001066, -47.71098080242150274 ) ) ;
#20984=CARTESIAN_POINT ( 'NONE',  ( 3.310556943750001313, 17.50000000000001421, -53.26410580289947205 ) ) ;
#20985=CARTESIAN_POINT ( 'NONE',  ( -3.500000000000001332, 17.50000000000001421, -68.65473080337743284 ) ) ;
#20986=CARTESIAN_POINT ( 'NONE',  ( 3.310556943749999981, 15.58864905735837247, -115.3474391362327935 ) ) ;
#20987=VECTOR ( 'NONE', #20572, 1000.000000000000000 ) ;
#20988=EDGE_CURVE ( 'NONE', #25124, #37987, #17663, .T. ) ;
#20990=ORIENTED_EDGE ( 'NONE', *, *, #34732, .T. ) ;
#20991=VERTEX_POINT ( 'NONE', #5216 ) ;
#20995=CARTESIAN_POINT ( 'NONE',  ( -3.500000000000000000, 19.52072594216371826, -110.0443141357548456 ) ) ;
#20996=CARTESIAN_POINT ( 'NONE',  ( 3.310556943749999981, 15.58864905735836537, -67.34743913623280775 ) ) ;
#20999=CARTESIAN_POINT ( 'NONE',  ( 0.000000000000000000, 17.50000000000002487, -149.5231586289125687 ) ) ;
#21002=ADVANCED_FACE ( 'NONE', ( #34769 ), #21379, .T. ) ;
#21003=ORIENTED_EDGE ( 'NONE', *, *, #14627, .T. ) ;
#21004=DIRECTION ( 'NONE',  ( -0.000000000000000000, 1.259100132267607459E-16, -1.000000000000000000 ) ) ;
#21005=CARTESIAN_POINT ( 'NONE',  ( 1.655278471875001101, 20.36702641396249902, -134.0974391362328220 ) ) ;
#21006=CARTESIAN_POINT ( 'NONE',  ( -1.394453263437886604E-15, 14.00000000000002132, -119.7109808024215170 ) ) ;
#21008=CARTESIAN_POINT ( 'NONE',  ( -3.310556943750000425, 19.41135094264165772, -45.93493913623279923 ) ) ;
#21009=CARTESIAN_POINT ( 'NONE',  ( -7.022189441860112050E-16, 13.67729811471671475, -32.60160580289946353 ) ) ;
#21010=CARTESIAN_POINT ( 'NONE',  ( -3.310556943750001313, 17.50000000000001776, -97.85160580289945642 ) ) ;
#21011=( BOUNDED_CURVE ( )  B_SPLINE_CURVE ( 2, ( #17687, #23440, #36619, #7483, #4288, #7052, #20032, #1313, #32997 ),
 .UNSPECIFIED., .F., .T. ) 
 B_SPLINE_CURVE_WITH_KNOTS ( ( 3, 2, 2, 2, 3 ),
 ( 0.6812500000000000222, 0.6819444444444444642, 0.6833333333333333481, 0.6847222222222222321, 0.6854166666666666741 ),
 .UNSPECIFIED. ) 
 CURVE ( )  GEOMETRIC_REPRESENTATION_ITEM ( )  RATIONAL_B_SPLINE_CURVE ( ( 0.9330127018922194093, 0.9330127018922194093, 1.000000000000000000, 0.8660254037844387076, 1.000000000000000000, 0.8660254037844387076, 1.000000000000000000, 0.9330127018922194093, 0.9330127018922194093 ) ) 
 REPRESENTATION_ITEM ( '' )  );
#21014=CARTESIAN_POINT ( 'NONE',  ( 1.655278471875001101, 20.36702641396249902, -136.1849391362327992 ) ) ;
#21015=CARTESIAN_POINT ( 'NONE',  ( 0.000000000000000000, 21.00000000000002487, -149.5231586289125687 ) ) ;
#21016=CARTESIAN_POINT ( 'NONE',  ( -1.749999999999999778, 20.53108891324555429, -98.12764746908817415 ) ) ;
#21019=CARTESIAN_POINT ( 'NONE',  ( -7.424026671074350129E-16, 13.45854811567263631, -85.40473080337743284 ) ) ;
#21020=CARTESIAN_POINT ( 'NONE',  ( 3.310556943750001313, 19.41135094264166483, -69.26827246956612782 ) ) ;
#21025=CARTESIAN_POINT ( 'NONE',  ( -3.500000000000002220, 15.47927405783632260, -49.87764746908817415 ) ) ;
#21026=CARTESIAN_POINT ( 'NONE',  ( -7.022189441860112050E-16, 13.67729811471672896, -119.5141058028994934 ) ) ;
#21027=DIRECTION ( 'NONE',  ( 0.000000000000000000, 1.000000000000000000, 0.000000000000000000 ) ) ;
#21029=EDGE_LOOP ( 'NONE', ( #9492, #39440, #8802, #12032, #6024, #15300, #27176, #17233 ) ) ;
#21031=CARTESIAN_POINT ( 'NONE',  ( 2.474675557024783212E-16, 21.54145188432740099, -114.9047308033774186 ) ) ;
#21032=CARTESIAN_POINT ( 'NONE',  ( 1.750000000000001110, 20.53108891324555074, -54.98806413671076854 ) ) ;
#21034=CARTESIAN_POINT ( 'NONE',  ( 1.750000000000001110, 20.53108891324555074, -60.98806413671076143 ) ) ;
#21037=CARTESIAN_POINT ( 'NONE',  ( -3.310556943750002201, 15.58864905735837070, -69.68077246956613635 ) ) ;
#21039=LINE ( 'NONE', #34017, #38679 ) ;
#21041=EDGE_CURVE ( 'NONE', #37987, #39141, #33322, .T. ) ;
#21042=CARTESIAN_POINT ( 'NONE',  ( -0.9378221735089310451, 14.00000000000001599, -63.75563900116003424 ) ) ;
#21043=CARTESIAN_POINT ( 'NONE',  ( -3.310556943750000425, 19.41135094264166483, -85.84743913623279354 ) ) ;
#21044=EDGE_LOOP ( 'NONE', ( #10574, #17491, #21824, #33497 ) ) ;
#21045=ORIENTED_EDGE ( 'NONE', *, *, #14627, .F. ) ;
#21047=VECTOR ( 'NONE', #23449, 1000.000000000000000 ) ;
#21054=CARTESIAN_POINT ( 'NONE',  ( -1.655278471874999990, 20.36702641396248836, -51.01827246956612782 ) ) ;
#21055=CARTESIAN_POINT ( 'NONE',  ( -3.310556943750000425, 19.41135094264166838, -112.9349391362327992 ) ) ;
#21056=VERTEX_POINT ( 'NONE', #29924 ) ;
#21057=CARTESIAN_POINT ( 'NONE',  ( 1.749999999999998224, 14.46891108675448478, -122.3213974700441042 ) ) ;
#21058=( BOUNDED_CURVE ( )  B_SPLINE_CURVE ( 2, ( #41439, #15498, #25272, #38241, #12289, #35051, #9748, #21864, #3150 ),
 .UNSPECIFIED., .F., .T. ) 
 B_SPLINE_CURVE_WITH_KNOTS ( ( 3, 2, 2, 2, 3 ),
 ( 0.9187499999999999556, 0.9194444444444443976, 0.9208333333333332815, 0.9222222222222222765, 0.9229166666666667185 ),
 .UNSPECIFIED. ) 
 CURVE ( )  GEOMETRIC_REPRESENTATION_ITEM ( )  RATIONAL_B_SPLINE_CURVE ( ( 0.9330127018922194093, 0.9330127018922194093, 1.000000000000000000, 0.8660254037844387076, 1.000000000000000000, 0.8660254037844387076, 1.000000000000000000, 0.9330127018922194093, 0.9330127018922194093 ) ) 
 REPRESENTATION_ITEM ( '' )  );
#21059=CARTESIAN_POINT ( 'NONE',  ( 2.340729813953370519E-16, 21.32270188528330479, -34.01410580289947205 ) ) ;
#21060=CARTESIAN_POINT ( 'NONE',  ( 1.655278471875001101, 20.36702641396248836, -69.18493913623279923 ) ) ;
#21061=CARTESIAN_POINT ( 'NONE',  ( -3.500000000000000888, 19.52072594216371826, -110.0443141357548456 ) ) ;
#21063=CARTESIAN_POINT ( 'NONE',  ( 1.655278471875001101, 20.36702641396249192, -98.09743913623280775 ) ) ;
#21065=CYLINDRICAL_SURFACE ( 'NONE', #13923, 3.499999999999999556 ) ;
#21068=CARTESIAN_POINT ( 'NONE',  ( 1.749999999999998224, 14.46891108675447768, -66.62764746908817415 ) ) ;
#21071=CARTESIAN_POINT ( 'NONE',  ( 3.310556943750001313, 17.50000000000001066, -33.26410580289947205 ) ) ;
#21072=CARTESIAN_POINT ( 'NONE',  ( -3.310556943750002645, 15.58864905735837247, -88.76827246956612782 ) ) ;
#21073=CARTESIAN_POINT ( 'NONE',  ( -1.750000000000002220, 14.46891108675447768, -52.48806413671076854 ) ) ;
#21074=CARTESIAN_POINT ( 'NONE',  ( 4.648177544792955347E-16, 21.00000000000001776, -92.21098080242150274 ) ) ;
#21075=CARTESIAN_POINT ( 'NONE',  ( -1.655278471875002211, 14.63297358603754894, -105.6849391362327992 ) ) ;
#21076=CARTESIAN_POINT ( 'NONE',  ( -1.655278471875002211, 14.63297358603754006, -39.68493913623280633 ) ) ;
#21082=CARTESIAN_POINT ( 'NONE',  ( -0.9378221735089310451, 14.00000000000001066, -49.75563900116002714 ) ) ;
#21083=CARTESIAN_POINT ( 'NONE',  ( 1.655278471875001101, 20.36702641396249192, -92.09743913623280775 ) ) ;
#21087=CARTESIAN_POINT ( 'NONE',  ( 4.648177544792955347E-16, 21.00000000000001421, -57.21098080242150274 ) ) ;
#21090=ORIENTED_EDGE ( 'NONE', *, *, #19329, .F. ) ;
#21095=CARTESIAN_POINT ( 'NONE',  ( 1.750000000000001110, 20.53108891324555429, -81.98806413671074722 ) ) ;
#21098=LINE ( 'NONE', #34071, #12923 ) ;
#21102=ORIENTED_EDGE ( 'NONE', *, *, #25102, .T. ) ;
#21103=AXIS2_PLACEMENT_3D ( 'NONE', #12872, #22653, #3092 ) ;
#21104=CARTESIAN_POINT ( 'NONE',  ( -3.500000000000001332, 17.50000000000001066, -27.65473080337743639 ) ) ;
#21105=CARTESIAN_POINT ( 'NONE',  ( -4.299564228933483745E-15, 21.00000000000002842, -139.9047308033774186 ) ) ;
#21106=CARTESIAN_POINT ( 'NONE',  ( 1.655278471874998436, 14.63297358603755249, -139.4307724695661364 ) ) ;
#21107=CARTESIAN_POINT ( 'NONE',  ( -3.500000000000002220, 15.47927405783633503, -132.5713974700441042 ) ) ;
#21108=CARTESIAN_POINT ( 'NONE',  ( 4.648177544792955347E-16, 21.00000000000001066, -26.90473080337742928 ) ) ;
#21109=CARTESIAN_POINT ( 'NONE',  ( 3.310556943749999981, 15.58864905735837425, -129.4349391362327992 ) ) ;
#21110=CARTESIAN_POINT ( 'NONE',  ( 1.655278471874998436, 14.63297358603754184, -57.51827246956612782 ) ) ;
#21111=VERTEX_POINT ( 'NONE', #36950 ) ;
#21113=CARTESIAN_POINT ( 'NONE',  ( -3.500000000000001332, 17.50000000000002487, -138.6547308033774186 ) ) ;
#21116=CARTESIAN_POINT ( 'NONE',  ( 3.500000000000000000, 15.47927405783633503, -126.5443141357548456 ) ) ;
#21117=CARTESIAN_POINT ( 'NONE',  ( -3.310556943750002645, 15.58864905735837780, -113.6807724695661364 ) ) ;
#21120=CARTESIAN_POINT ( 'NONE',  ( 1.749999999999998224, 14.46891108675447946, -79.62764746908817415 ) ) ;
#21121=CARTESIAN_POINT ( 'NONE',  ( -0.9378221735089291577, 21.00000000000001421, -69.86007260463891555 ) ) ;
#21122=CARTESIAN_POINT ( 'NONE',  ( 3.310556943750001313, 17.50000000000001421, -47.26410580289947205 ) ) ;
#21123=CARTESIAN_POINT ( 'NONE',  ( -3.310556943750001313, 17.50000000000002132, -106.8516058028994564 ) ) ;
#21124=CARTESIAN_POINT ( 'NONE',  ( -1.750000000000002220, 14.46891108675448834, -130.4880641367107614 ) ) ;
#21125=CARTESIAN_POINT ( 'NONE',  ( -0.9378221735089310451, 14.00000000000002132, -99.44938900211596433 ) ) ;
#21126=CARTESIAN_POINT ( 'NONE',  ( -1.750000000000002220, 14.46891108675448301, -88.79431413575483134 ) ) ;
#21127=CARTESIAN_POINT ( 'NONE',  ( -3.310556943750000425, 19.41135094264166838, -128.9349391362327992 ) ) ;
#21130=CYLINDRICAL_SURFACE ( 'NONE', #16374, 3.499999999999999556 ) ;
#21131=CARTESIAN_POINT ( 'NONE',  ( 1.655278471875001101, 20.36702641396248836, -59.18493913623279212 ) ) ;
#21132=VECTOR ( 'NONE', #38090, 1000.000000000000000 ) ;
#21133=VERTEX_POINT ( 'NONE', #4406 ) ;
#21134=CARTESIAN_POINT ( 'NONE',  ( -3.310556943750000425, 19.41135094264166838, -80.93493913623279923 ) ) ;
#21135=CARTESIAN_POINT ( 'NONE',  ( 3.602337597214540226E-14, 14.00000000000002132, -117.7109808024215027 ) ) ;
#21137=CYLINDRICAL_SURFACE ( 'NONE', #23937, 3.499999999999999556 ) ;
#21141=CARTESIAN_POINT ( 'NONE',  ( -1.655278471875002211, 14.63297358603754006, -39.59743913623281486 ) ) ;
#21144=EDGE_LOOP ( 'NONE', ( #24628, #38235, #14721, #40025 ) ) ;
#21146=CARTESIAN_POINT ( 'NONE',  ( -3.310556943750000425, 19.41135094264165772, -45.84743913623280775 ) ) ;
#21147=ORIENTED_EDGE ( 'NONE', *, *, #6716, .F. ) ;
#21149=FACE_OUTER_BOUND ( 'NONE', #37781, .T. ) ;
#21152=VERTEX_POINT ( 'NONE', #39493 ) ;
#21154=CARTESIAN_POINT ( 'NONE',  ( 1.750000000000001110, 20.53108891324554719, -36.29431413575484555 ) ) ;
#21157=CARTESIAN_POINT ( 'NONE',  ( -0.9378221735088960731, 14.00000000000000355, -110.4493890021159501 ) ) ;
#21160=CARTESIAN_POINT ( 'NONE',  ( -3.500000000000000888, 19.52072594216372181, -143.0443141357548313 ) ) ;
#21162=CARTESIAN_POINT ( 'NONE',  ( 1.655278471874998436, 14.63297358603755072, -129.4307724695661364 ) ) ;
#21166=CARTESIAN_POINT ( 'NONE',  ( 3.310556943750001313, 17.50000000000002132, -123.3516058028994564 ) ) ;
#21167=CARTESIAN_POINT ( 'NONE',  ( 0.000000000000000000, 21.00000000000002487, -149.5231586289125687 ) ) ;
#21168=CARTESIAN_POINT ( 'NONE',  ( 2.474675557024783212E-16, 21.54145188432739033, -39.90473080337743284 ) ) ;
#21169=CARTESIAN_POINT ( 'NONE',  ( 3.500000000000001332, 17.50000000000002132, -115.1547308033774328 ) ) ;
#21171=CARTESIAN_POINT ( 'NONE',  ( 1.655278471875001101, 20.36702641396249902, -143.1849391362327992 ) ) ;
#21172=CARTESIAN_POINT ( 'NONE',  ( -7.424026671074350129E-16, 13.45854811567263454, -71.40473080337743284 ) ) ;
#21173=CARTESIAN_POINT ( 'NONE',  ( -1.655278471874999990, 20.36702641396248836, -52.01827246956612782 ) ) ;
#21176=CARTESIAN_POINT ( 'NONE',  ( 3.310556943750001313, 17.50000000000001776, -77.35160580289945642 ) ) ;
#21178=CARTESIAN_POINT ( 'NONE',  ( 1.655278471875001101, 20.36702641396249192, -101.0974391362328078 ) ) ;
#21179=CARTESIAN_POINT ( 'NONE',  ( -3.310556943750000425, 19.41135094264166483, -75.84743913623279354 ) ) ;
#21181=CARTESIAN_POINT ( 'NONE',  ( -3.310556943750000425, 19.41135094264166838, -97.93493913623278502 ) ) ;
#21182=( BOUNDED_CURVE ( )  B_SPLINE_CURVE ( 2, ( #18457, #5271, #11855, #37811, #31424, #15275, #28234, #12916, #36290 ),
 .UNSPECIFIED., .F., .T. ) 
 B_SPLINE_CURVE_WITH_KNOTS ( ( 3, 2, 2, 2, 3 ),
 ( 0.4354166666666666741, 0.4361111111111111160, 0.4375000000000000000, 0.4388888888888888840, 0.4395833333333333259 ),
 .UNSPECIFIED. ) 
 CURVE ( )  GEOMETRIC_REPRESENTATION_ITEM ( )  RATIONAL_B_SPLINE_CURVE ( ( 0.9330127018922194093, 0.9330127018922194093, 1.000000000000000000, 0.8660254037844387076, 1.000000000000000000, 0.8660254037844387076, 1.000000000000000000, 0.9330127018922194093, 0.9330127018922194093 ) ) 
 REPRESENTATION_ITEM ( '' )  );
#21184=CARTESIAN_POINT ( 'NONE',  ( -3.500000000000000000, 19.52072594216370405, -33.04431413575484555 ) ) ;
#21187=CARTESIAN_POINT ( 'NONE',  ( 2.340729813953370519E-16, 21.32270188528331190, -58.01410580289949337 ) ) ;
#21188=EDGE_CURVE ( 'NONE', #28293, #745, #4610, .T. ) ;
#21189=LINE ( 'NONE', #24391, #29336 ) ;
#21190=CARTESIAN_POINT ( 'NONE',  ( -1.655278471875002211, 14.63297358603755072, -109.5974391362328078 ) ) ;
#21191=CARTESIAN_POINT ( 'NONE',  ( 1.750000000000001110, 20.53108891324555429, -84.29431413575483134 ) ) ;
#21192=( BOUNDED_CURVE ( )  B_SPLINE_CURVE ( 2, ( #26110, #146, #26320, #6325, #35465, #29273, #3344, #19300, #10359 ),
 .UNSPECIFIED., .F., .F. ) 
 B_SPLINE_CURVE_WITH_KNOTS ( ( 3, 2, 2, 2, 3 ),
 ( 0.3854166666666666852, 0.3861111111111111271, 0.3875000000000000111, 0.3888888888888888951, 0.3895833333333333370 ),
 .UNSPECIFIED. ) 
 CURVE ( )  GEOMETRIC_REPRESENTATION_ITEM ( )  RATIONAL_B_SPLINE_CURVE ( ( 0.9330127018922194093, 0.9330127018922194093, 1.000000000000000000, 0.8660254037844387076, 1.000000000000000000, 0.8660254037844387076, 1.000000000000000000, 0.9330127018922194093, 0.9330127018922194093 ) ) 
 REPRESENTATION_ITEM ( '' )  );
#21195=VERTEX_POINT ( 'NONE', #37358 ) ;
#21198=VERTEX_POINT ( 'NONE', #27984 ) ;
#21199=CARTESIAN_POINT ( 'NONE',  ( 4.648177544792955347E-16, 21.00000000000001066, -33.21098080242150274 ) ) ;
#21200=CARTESIAN_POINT ( 'NONE',  ( -7.022189441860112050E-16, 13.67729811471672186, -67.51410580289946495 ) ) ;
#21203=CARTESIAN_POINT ( 'NONE',  ( -3.500000000000002220, 15.47927405783633503, -130.8776474690881741 ) ) ;
#21210=CARTESIAN_POINT ( 'NONE',  ( -3.310556943750000425, 19.41135094264167549, -131.8474391362328220 ) ) ;
#21212=ADVANCED_FACE ( 'NONE', ( #24598 ), #27780, .T. ) ;
#21213=CARTESIAN_POINT ( 'NONE',  ( -3.310556943750002645, 15.58864905735836537, -37.76827246956612782 ) ) ;
#21214=CARTESIAN_POINT ( 'NONE',  ( -3.310556943750000425, 19.41135094264165772, -32.93493913623279923 ) ) ;
#21216=CARTESIAN_POINT ( 'NONE',  ( 3.310556943750001313, 19.41135094264166483, -92.26827246956612782 ) ) ;
#21217=CARTESIAN_POINT ( 'NONE',  ( -1.750000000000002220, 14.46891108675447413, -23.48806413671077209 ) ) ;
#21221=CARTESIAN_POINT ( 'NONE',  ( 1.655278471874998436, 14.63297358603755249, -140.5182724695661420 ) ) ;
#21222=CARTESIAN_POINT ( 'NONE',  ( 4.648177544792955347E-16, 21.00000000000002132, -126.2109808024214885 ) ) ;
#21223=CARTESIAN_POINT ( 'NONE',  ( -1.749999999999999778, 20.53108891324555429, -95.12764746908815994 ) ) ;
#21225=CARTESIAN_POINT ( 'NONE',  ( -3.500000000000002220, 15.47927405783632615, -61.57139747004410424 ) ) ;
#21226=CARTESIAN_POINT ( 'NONE',  ( -1.750000000000002220, 14.46891108675448301, -86.48806413671076143 ) ) ;
#21227=CARTESIAN_POINT ( 'NONE',  ( 2.340729813953370519E-16, 21.32270188528331190, -70.10160580289947063 ) ) ;
#21231=DIRECTION ( 'NONE',  ( -0.000000000000000000, 1.259100132267607459E-16, -1.000000000000000000 ) ) ;
#21232=CARTESIAN_POINT ( 'NONE',  ( 1.750000000000001110, 20.53108891324555074, -50.29431413575484555 ) ) ;
#21233=CARTESIAN_POINT ( 'NONE',  ( 1.655278471874998436, 14.63297358603754894, -117.4307724695661364 ) ) ;
#21234=LINE ( 'NONE', #8669, #12889 ) ;
#21235=CARTESIAN_POINT ( 'NONE',  ( -3.500000000000000000, 19.52072594216370405, -35.04431413575484555 ) ) ;
#21237=CARTESIAN_POINT ( 'NONE',  ( -3.500000000000002220, 15.47927405783633503, -113.5713974700440900 ) ) ;
#21239=CARTESIAN_POINT ( 'NONE',  ( -0.9378221735089310451, 14.00000000000002132, -83.44938900211595012 ) ) ;
#21243=CARTESIAN_POINT ( 'NONE',  ( -7.022189441860112050E-16, 13.67729811471672186, -72.51410580289946495 ) ) ;
#21245=CARTESIAN_POINT ( 'NONE',  ( -0.9378221735089310451, 14.00000000000002132, -96.75563900116003424 ) ) ;
#21246=EDGE_CURVE ( 'NONE', #25967, #18164, #17910, .T. ) ;
#21248=VECTOR ( 'NONE', #11086, 1000.000000000000000 ) ;
#21249=ORIENTED_EDGE ( 'NONE', *, *, #38085, .T. ) ;
#21250=CARTESIAN_POINT ( 'NONE',  ( 2.340729813953370519E-16, 21.32270188528330834, -26.01410580289947916 ) ) ;
#21251=CARTESIAN_POINT ( 'NONE',  ( 0.9378221735089300459, 21.00000000000001066, -25.25563900116003424 ) ) ;
#21252=CARTESIAN_POINT ( 'NONE',  ( 3.310556943750001313, 17.50000000000001776, -84.26410580289947916 ) ) ;
#21257=( BOUNDED_CURVE ( )  B_SPLINE_CURVE ( 2, ( #37048, #14287, #13643, #36836, #26626, #36405, #1521, #14499, #27470 ),
 .UNSPECIFIED., .F., .T. ) 
 B_SPLINE_CURVE_WITH_KNOTS ( ( 3, 2, 2, 2, 3 ),
 ( 0.9937500000000000222, 0.9944444444444444642, 0.9958333333333333481, 0.9972222222222222321, 0.9979166666666666741 ),
 .UNSPECIFIED. ) 
 CURVE ( )  GEOMETRIC_REPRESENTATION_ITEM ( )  RATIONAL_B_SPLINE_CURVE ( ( 0.9330127018922194093, 0.9330127018922194093, 1.000000000000000000, 0.8660254037844387076, 1.000000000000000000, 0.8660254037844387076, 1.000000000000000000, 0.9330127018922194093, 0.9330127018922194093 ) ) 
 REPRESENTATION_ITEM ( '' )  );
#21261=CARTESIAN_POINT ( 'NONE',  ( 1.655278471874998436, 14.63297358603754006, -47.51827246956613493 ) ) ;
#21262=CARTESIAN_POINT ( 'NONE',  ( 3.310556943750001313, 19.41135094264166838, -109.2682724695661278 ) ) ;
#21265=CARTESIAN_POINT ( 'NONE',  ( 3.310556943749999981, 15.58864905735836182, -36.34743913623281486 ) ) ;
#21266=CARTESIAN_POINT ( 'NONE',  ( 2.340729813953370519E-16, 21.32270188528330834, -67.10160580289945642 ) ) ;
#21267=CARTESIAN_POINT ( 'NONE',  ( 3.500000000000000000, 15.47927405783632970, -114.5443141357548171 ) ) ;
#21268=EDGE_CURVE ( 'NONE', #2767, #10325, #40345, .T. ) ;
#21270=CARTESIAN_POINT ( 'NONE',  ( 3.310556943750001313, 17.50000000000001776, -95.26410580289946495 ) ) ;
#21271=AXIS2_PLACEMENT_3D ( 'NONE', #31778, #41798, #35185 ) ;
#21272=CARTESIAN_POINT ( 'NONE',  ( 4.648177544792955347E-16, 21.00000000000002132, -122.2109808024215170 ) ) ;
#21273=CARTESIAN_POINT ( 'NONE',  ( 1.749999999999998224, 14.46891108675447590, -52.32139747004409003 ) ) ;
#21277=CARTESIAN_POINT ( 'NONE',  ( -1.750000000000002220, 14.46891108675447946, -63.79431413575484555 ) ) ;
#21278=CARTESIAN_POINT ( 'NONE',  ( -0.9378221735089310451, 14.00000000000001599, -71.75563900116002003 ) ) ;
#21279=CARTESIAN_POINT ( 'NONE',  ( -3.310556943750000425, 19.41135094264165772, -33.84743913623280775 ) ) ;
#21280=CARTESIAN_POINT ( 'NONE',  ( 3.310556943750001313, 17.50000000000001776, -93.35160580289947063 ) ) ;
#21281=CARTESIAN_POINT ( 'NONE',  ( -1.749999999999999778, 20.53108891324555074, -53.82139747004409713 ) ) ;
#21282=DIRECTION ( 'NONE',  ( -0.000000000000000000, 1.259100132267607459E-16, -1.000000000000000000 ) ) ;
#21283=CARTESIAN_POINT ( 'NONE',  ( 1.655278471875001101, 20.36702641396249547, -106.1849391362327992 ) ) ;
#21284=CARTESIAN_POINT ( 'NONE',  ( 2.340729813953370519E-16, 21.32270188528330834, -37.10160580289946353 ) ) ;
#21286=CARTESIAN_POINT ( 'NONE',  ( 3.500000000000000000, 15.47927405783632082, -53.54431413575483845 ) ) ;
#21293=CARTESIAN_POINT ( 'NONE',  ( 1.655278471875001101, 20.36702641396249192, -86.09743913623279354 ) ) ;
#21294=FACE_OUTER_BOUND ( 'NONE', #18673, .T. ) ;
#21298=CARTESIAN_POINT ( 'NONE',  ( 0.9378221735089281585, 14.00000000000001599, -74.66632260368299967 ) ) ;
#21303=ORIENTED_EDGE ( 'NONE', *, *, #17697, .T. ) ;
#21305=LINE ( 'NONE', #5342, #16333 ) ;
#21309=CARTESIAN_POINT ( 'NONE',  ( 0.9378221735089281585, 14.00000000000002132, -109.3600726046389013 ) ) ;
#21310=( BOUNDED_CURVE ( )  B_SPLINE_CURVE ( 2, ( #24124, #14328, #37094, #7950, #20916, #40273, #21543, #20714, #14954 ),
 .UNSPECIFIED., .F., .T. ) 
 B_SPLINE_CURVE_WITH_KNOTS ( ( 3, 2, 2, 2, 3 ),
 ( 0.5270833333333333481, 0.5277777777777777901, 0.5291666666666666741, 0.5305555555555555580, 0.5312500000000000000 ),
 .UNSPECIFIED. ) 
 CURVE ( )  GEOMETRIC_REPRESENTATION_ITEM ( )  RATIONAL_B_SPLINE_CURVE ( ( 0.9330127018922194093, 0.9330127018922194093, 1.000000000000000000, 0.8660254037844387076, 1.000000000000000000, 0.8660254037844387076, 1.000000000000000000, 0.9330127018922194093, 0.9330127018922194093 ) ) 
 REPRESENTATION_ITEM ( '' )  );
#21311=DIRECTION ( 'NONE',  ( -0.000000000000000000, 1.259100132267607459E-16, -1.000000000000000000 ) ) ;
#21312=CARTESIAN_POINT ( 'NONE',  ( 2.340729813953370519E-16, 21.32270188528332255, -135.0141058028994507 ) ) ;
#21313=VECTOR ( 'NONE', #27999, 1000.000000000000000 ) ;
#21314=CARTESIAN_POINT ( 'NONE',  ( 3.500000000000001332, 19.52072594216370405, -38.07139747004409713 ) ) ;
#21316=CARTESIAN_POINT ( 'NONE',  ( 0.000000000000000000, 17.50000000000002487, -143.4609808024215170 ) ) ;
#21317=CARTESIAN_POINT ( 'NONE',  ( -3.310556943750002645, 15.58864905735837780, -127.7682724695661136 ) ) ;
#21318=CARTESIAN_POINT ( 'NONE',  ( -7.022189441860112050E-16, 13.67729811471671653, -53.60160580289946353 ) ) ;
#21321=CARTESIAN_POINT ( 'NONE',  ( -1.750000000000002220, 14.46891108675449011, -138.4880641367107614 ) ) ;
#21323=CARTESIAN_POINT ( 'NONE',  ( 1.749999999999998224, 14.46891108675448656, -128.6276474690881741 ) ) ;
#21324=CARTESIAN_POINT ( 'NONE',  ( 1.655278471875001101, 20.36702641396249547, -115.0974391362327935 ) ) ;
#21328=CARTESIAN_POINT ( 'NONE',  ( -3.500000000000000888, 19.52072594216371115, -81.04431413575484555 ) ) ;
#21329=CARTESIAN_POINT ( 'NONE',  ( 4.648177544792955347E-16, 21.00000000000001421, -62.21098080242150274 ) ) ;
#21330=CARTESIAN_POINT ( 'NONE',  ( 1.655278471875001101, 20.36702641396248481, -46.09743913623280775 ) ) ;
#21331=CARTESIAN_POINT ( 'NONE',  ( -3.310556943750002645, 15.58864905735837425, -107.7682724695661420 ) ) ;
#21332=FACE_OUTER_BOUND ( 'NONE', #6756, .T. ) ;
#21334=CARTESIAN_POINT ( 'NONE',  ( -3.500000000000001332, 17.50000000000001066, -42.65473080337743284 ) ) ;
#21336=CARTESIAN_POINT ( 'NONE',  ( 1.655278471875001101, 20.36702641396249547, -123.1849391362327992 ) ) ;
#21340=CARTESIAN_POINT ( 'NONE',  ( 1.749999999999998224, 14.46891108675447413, -27.62764746908817770 ) ) ;
#21342=CARTESIAN_POINT ( 'NONE',  ( -3.310556943750002645, 15.58864905735836892, -57.76827246956613493 ) ) ;
#21344=CARTESIAN_POINT ( 'NONE',  ( 3.310556943749999981, 15.58864905735836714, -74.43493913623279923 ) ) ;
#21345=CARTESIAN_POINT ( 'NONE',  ( 4.648177544792955347E-16, 21.00000000000002132, -104.2109808024215027 ) ) ;
#21347=CARTESIAN_POINT ( 'NONE',  ( 3.500000000000000000, 15.47927405783632082, -30.23806413671076143 ) ) ;
#21350=CARTESIAN_POINT ( 'NONE',  ( 3.500000000000000000, 15.47927405783632615, -74.23806413671076143 ) ) ;
#21352=CARTESIAN_POINT ( 'NONE',  ( 3.310556943750001313, 19.41135094264166128, -38.18077246956613635 ) ) ;
#21357=CARTESIAN_POINT ( 'NONE',  ( 3.310556943749999981, 15.58864905735836182, -46.34743913623280775 ) ) ;
#21358=VERTEX_POINT ( 'NONE', #37160 ) ;
#21359=ORIENTED_EDGE ( 'NONE', *, *, #4786, .T. ) ;
#21361=CARTESIAN_POINT ( 'NONE',  ( 3.500000000000001332, 17.50000000000001066, -24.46098080242150985 ) ) ;
#21364=CARTESIAN_POINT ( 'NONE',  ( 3.500000000000001332, 19.52072594216371115, -97.37764746908817415 ) ) ;
#21365=CARTESIAN_POINT ( 'NONE',  ( 0.9378221735089300459, 21.00000000000001066, -43.25563900116002714 ) ) ;
#21366=CARTESIAN_POINT ( 'NONE',  ( -3.500000000000000888, 19.52072594216370405, -38.04431413575485266 ) ) ;
#21367=CARTESIAN_POINT ( 'NONE',  ( -1.750000000000002220, 14.46891108675447946, -64.48806413671076143 ) ) ;
#21369=CARTESIAN_POINT ( 'NONE',  ( 3.500000000000001776, 19.52072594216372181, -143.3776474690881741 ) ) ;
#21370=CARTESIAN_POINT ( 'NONE',  ( -1.750000000000002220, 14.46891108675447946, -59.48806413671076143 ) ) ;
#21371=CARTESIAN_POINT ( 'NONE',  ( -3.310556943750002645, 15.58864905735837780, -129.6807724695661364 ) ) ;
#21374=CARTESIAN_POINT ( 'NONE',  ( 3.500000000000001332, 17.50000000000001066, -24.15473080337743284 ) ) ;
#21375=CARTESIAN_POINT ( 'NONE',  ( 3.310556943750001313, 17.50000000000002132, -121.3516058028994706 ) ) ;
#21377=CARTESIAN_POINT ( 'NONE',  ( -1.750000000000002220, 14.46891108675447590, -38.48806413671076854 ) ) ;
#21378=CARTESIAN_POINT ( 'NONE',  ( 3.500000000000001332, 19.52072594216371826, -115.0713974700440758 ) ) ;
#21379=CYLINDRICAL_SURFACE ( 'NONE', #23920, 3.499999999999999556 ) ;
#21380=CARTESIAN_POINT ( 'NONE',  ( 3.310556943749999981, 15.58864905735837780, -140.4349391362327708 ) ) ;
#21381=CARTESIAN_POINT ( 'NONE',  ( -7.424026671074350129E-16, 13.45854811567263454, -67.40473080337743284 ) ) ;
#21383=CARTESIAN_POINT ( 'NONE',  ( -3.310556943750002201, 15.58864905735836714, -48.76827246956613493 ) ) ;
#21385=CARTESIAN_POINT ( 'NONE',  ( 3.310556943749999981, 15.58864905735836714, -76.43493913623278502 ) ) ;
#21387=CARTESIAN_POINT ( 'NONE',  ( 3.310556943749999981, 15.58864905735837070, -105.3474391362328078 ) ) ;
#21388=CARTESIAN_POINT ( 'NONE',  ( -3.310556943750000425, 19.41135094264166128, -68.84743913623280775 ) ) ;
#21390=CARTESIAN_POINT ( 'NONE',  ( 3.310556943749999981, 15.58864905735837070, -97.43493913623281344 ) ) ;
#21394=CARTESIAN_POINT ( 'NONE',  ( 0.000000000000000000, 21.00000000000002487, -149.5231586289125687 ) ) ;
#21395=CARTESIAN_POINT ( 'NONE',  ( 3.500000000000000000, 15.47927405783633326, -117.5443141357548171 ) ) ;
#21396=CARTESIAN_POINT ( 'NONE',  ( 3.310556943750001313, 19.41135094264166483, -54.18077246956613635 ) ) ;
#21397=CARTESIAN_POINT ( 'NONE',  ( 4.286263797015737581E-16, 14.00000000000002487, -149.5231586289125687 ) ) ;
#21398=CARTESIAN_POINT ( 'NONE',  ( 3.310556943749999981, 15.58864905735837247, -111.3474391362328078 ) ) ;
#21399=AXIS2_PLACEMENT_3D ( 'NONE', #30417, #40822, #17659 ) ;
#21400=ORIENTED_EDGE ( 'NONE', *, *, #24842, .F. ) ;
#21404=EDGE_LOOP ( 'NONE', ( #22341, #25279, #36153, #4916 ) ) ;
#21406=CARTESIAN_POINT ( 'NONE',  ( -3.310556943750001313, 17.50000000000001421, -61.76410580289947205 ) ) ;
#21407=VERTEX_POINT ( 'NONE', #20983 ) ;
#21408=ORIENTED_EDGE ( 'NONE', *, *, #32428, .T. ) ;
#21415=CARTESIAN_POINT ( 'NONE',  ( -3.310556943750000425, 19.41135094264167549, -130.8474391362328220 ) ) ;
#21418=CARTESIAN_POINT ( 'NONE',  ( 2.340729813953370519E-16, 21.32270188528330479, -41.10160580289946353 ) ) ;
#21419=CARTESIAN_POINT ( 'NONE',  ( 3.310556943750001313, 17.50000000000001066, -32.35160580289946353 ) ) ;
#21420=CARTESIAN_POINT ( 'NONE',  ( -3.310556943750000425, 19.41135094264166483, -91.93493913623278502 ) ) ;
#21421=CARTESIAN_POINT ( 'NONE',  ( 1.749999999999998224, 14.46891108675447235, -25.32139747004409713 ) ) ;
#21422=VERTEX_POINT ( 'NONE', #18835 ) ;
#21423=EDGE_CURVE ( 'NONE', #25228, #22103, #29313, .T. ) ;
#21425=CARTESIAN_POINT ( 'NONE',  ( 3.310556943749999981, 15.58864905735836892, -84.34743913623280775 ) ) ;
#21427=( BOUNDED_CURVE ( )  B_SPLINE_CURVE ( 2, ( #41301, #33871, #8129, #11321, #21727, #37077, #28108, #27498, #31097 ),
 .UNSPECIFIED., .F., .T. ) 
 B_SPLINE_CURVE_WITH_KNOTS ( ( 3, 2, 2, 2, 3 ),
 ( 0.3479166666666666519, 0.3486111111111110938, 0.3499999999999999778, 0.3513888888888888618, 0.3520833333333333592 ),
 .UNSPECIFIED. ) 
 CURVE ( )  GEOMETRIC_REPRESENTATION_ITEM ( )  RATIONAL_B_SPLINE_CURVE ( ( 0.9330127018922194093, 0.9330127018922194093, 1.000000000000000000, 0.8660254037844387076, 1.000000000000000000, 0.8660254037844387076, 1.000000000000000000, 0.9330127018922167448, 0.9330127018922194093 ) ) 
 REPRESENTATION_ITEM ( '' )  );
#21428=CARTESIAN_POINT ( 'NONE',  ( 3.310556943750001313, 17.50000000000002487, -139.3516058028994564 ) ) ;
#21431=CARTESIAN_POINT ( 'NONE',  ( -3.500000000000000888, 19.52072594216371115, -97.04431413575484555 ) ) ;
#21432=CARTESIAN_POINT ( 'NONE',  ( 1.655278471874998436, 14.63297358603754184, -57.43077246956614346 ) ) ;
#21433=CARTESIAN_POINT ( 'NONE',  ( 3.500000000000000000, 15.47927405783632437, -64.54431413575484555 ) ) ;
#21434=CARTESIAN_POINT ( 'NONE',  ( -7.424026671074350129E-16, 13.45854811567263631, -88.40473080337743284 ) ) ;
#21435=CARTESIAN_POINT ( 'NONE',  ( 3.310556943749999981, 15.58864905735836714, -70.43493913623279923 ) ) ;
#21438=CARTESIAN_POINT ( 'NONE',  ( -3.500000000000002220, 15.47927405783633503, -116.5713974700440900 ) ) ;
#21439=CARTESIAN_POINT ( 'NONE',  ( -3.500000000000000888, 19.52072594216370760, -50.04431413575484555 ) ) ;
#21440=CARTESIAN_POINT ( 'NONE',  ( 2.340729813953370519E-16, 21.32270188528331900, -120.0141058028994649 ) ) ;
#21442=CARTESIAN_POINT ( 'NONE',  ( 4.648177544792955347E-16, 21.00000000000001421, -72.90473080337743284 ) ) ;
#21444=CARTESIAN_POINT ( 'NONE',  ( -1.749999999999999778, 20.53108891324555785, -111.8213974700441042 ) ) ;
#21446=CARTESIAN_POINT ( 'NONE',  ( 4.648177544792955347E-16, 21.00000000000001776, -83.90473080337743284 ) ) ;
#21447=CARTESIAN_POINT ( 'NONE',  ( 1.749999999999998224, 14.46891108675447413, -37.62764746908817415 ) ) ;
#21450=CARTESIAN_POINT ( 'NONE',  ( 1.655278471874998436, 14.63297358603754361, -70.43077246956613635 ) ) ;
#21452=EDGE_CURVE ( 'NONE', #7014, #2470, #9265, .T. ) ;
#21453=CARTESIAN_POINT ( 'NONE',  ( 1.749999999999998224, 14.46891108675447946, -72.62764746908817415 ) ) ;
#21454=EDGE_CURVE ( 'NONE', #25342, #3618, #15654, .T. ) ;
#21455=VERTEX_POINT ( 'NONE', #42024 ) ;
#21456=CARTESIAN_POINT ( 'NONE',  ( 2.340729813953370519E-16, 21.32270188528330834, -24.01410580289947205 ) ) ;
#21457=CARTESIAN_POINT ( 'NONE',  ( 1.750000000000001110, 20.53108891324555429, -88.29431413575483134 ) ) ;
#21458=CARTESIAN_POINT ( 'NONE',  ( -3.310556943750002645, 15.58864905735837070, -76.68077246956615056 ) ) ;
#21460=ORIENTED_EDGE ( 'NONE', *, *, #37133, .T. ) ;
#21461=AXIS2_PLACEMENT_3D ( 'NONE', #27183, #21004, #11625 ) ;
#21466=CARTESIAN_POINT ( 'NONE',  ( 1.655278471874998436, 14.63297358603754006, -50.51827246956612782 ) ) ;
#21467=CARTESIAN_POINT ( 'NONE',  ( -1.655278471875002211, 14.63297358603754894, -107.6849391362327992 ) ) ;
#21468=EDGE_LOOP ( 'NONE', ( #31182, #22351, #2502, #15829 ) ) ;
#21469=EDGE_CURVE ( 'NONE', #21133, #29815, #22251, .T. ) ;
#21471=ADVANCED_FACE ( 'NONE', ( #32431 ), #3295, .T. ) ;
#21472=CARTESIAN_POINT ( 'NONE',  ( -3.310556943750001313, 17.50000000000001066, -35.76410580289947205 ) ) ;
#21473=CARTESIAN_POINT ( 'NONE',  ( 3.310556943750001313, 17.50000000000001421, -62.35160580289945642 ) ) ;
#21474=CARTESIAN_POINT ( 'NONE',  ( 3.500000000000000000, 15.47927405783632970, -113.5443141357548456 ) ) ;
#21476=CARTESIAN_POINT ( 'NONE',  ( 3.310556943749999981, 15.58864905735837070, -95.34743913623282197 ) ) ;
#21477=CARTESIAN_POINT ( 'NONE',  ( -1.394453263437886604E-15, 14.00000000000001066, -42.71098080242150274 ) ) ;
#21478=CARTESIAN_POINT ( 'NONE',  ( -3.500000000000002220, 15.47927405783632615, -56.57139747004409713 ) ) ;
#21480=CARTESIAN_POINT ( 'NONE',  ( -3.500000000000000888, 19.52072594216370760, -65.04431413575484555 ) ) ;
#21482=CARTESIAN_POINT ( 'NONE',  ( -1.655278471875002211, 14.63297358603754006, -31.59743913623280775 ) ) ;
#21483=CARTESIAN_POINT ( 'NONE',  ( 2.474675557024783212E-16, 21.54145188432739388, -54.90473080337743284 ) ) ;
#21486=CARTESIAN_POINT ( 'NONE',  ( 1.655278471874998436, 14.63297358603754716, -107.5182724695661278 ) ) ;
#21487=CARTESIAN_POINT ( 'NONE',  ( 3.310556943749999981, 15.58864905735836182, -36.43493913623279923 ) ) ;
#21489=CARTESIAN_POINT ( 'NONE',  ( 1.749999999999998224, 14.46891108675447590, -53.62764746908817415 ) ) ;
#21496=CARTESIAN_POINT ( 'NONE',  ( -1.655278471874999990, 20.36702641396249192, -86.93077246956613635 ) ) ;
#21497=CARTESIAN_POINT ( 'NONE',  ( 0.000000000000000000, 17.50000000000002487, -149.5231586289125687 ) ) ;
#21501=CARTESIAN_POINT ( 'NONE',  ( 0.9378221735089300459, 21.00000000000002487, -132.9493890021159359 ) ) ;
#21506=( BOUNDED_CURVE ( )  B_SPLINE_CURVE ( 2, ( #13593, #26577, #410, #32947, #3814, #1058, #39317, #36132, #32731 ),
 .UNSPECIFIED., .F., .F. ) 
 B_SPLINE_CURVE_WITH_KNOTS ( ( 3, 2, 2, 2, 3 ),
 ( 0.6854166666666666741, 0.6861111111111111160, 0.6875000000000000000, 0.6888888888888888840, 0.6895833333333333259 ),
 .UNSPECIFIED. ) 
 CURVE ( )  GEOMETRIC_REPRESENTATION_ITEM ( )  RATIONAL_B_SPLINE_CURVE ( ( 0.9330127018922194093, 0.9330127018922194093, 1.000000000000000000, 0.8660254037844387076, 1.000000000000000000, 0.8660254037844387076, 1.000000000000000000, 0.9330127018922194093, 0.9330127018922194093 ) ) 
 REPRESENTATION_ITEM ( '' )  );
#21507=ORIENTED_EDGE ( 'NONE', *, *, #17697, .F. ) ;
#21509=ORIENTED_EDGE ( 'NONE', *, *, #13910, .T. ) ;
#21511=EDGE_CURVE ( 'NONE', #29443, #37080, #22004, .T. ) ;
#21517=EDGE_LOOP ( 'NONE', ( #25234, #30190, #34316, #30365 ) ) ;
#21519=CARTESIAN_POINT ( 'NONE',  ( 0.000000000000000000, 17.50000000000002487, -149.5231586289125687 ) ) ;
#21520=CARTESIAN_POINT ( 'NONE',  ( -3.310556943750001313, 17.50000000000002487, -138.7641058028994792 ) ) ;
#21521=CARTESIAN_POINT ( 'NONE',  ( 1.750000000000001110, 20.53108891324555785, -103.9880641367107756 ) ) ;
#21522=VERTEX_POINT ( 'NONE', #16087 ) ;
#21525=CARTESIAN_POINT ( 'NONE',  ( -3.310556943750000425, 19.41135094264166838, -123.9349391362327992 ) ) ;
#21526=CARTESIAN_POINT ( 'NONE',  ( 3.310556943749999981, 15.58864905735836537, -56.43493913623279212 ) ) ;
#21529=CARTESIAN_POINT ( 'NONE',  ( 1.750000000000001110, 20.53108891324556140, -136.9880641367107614 ) ) ;
#21532=CARTESIAN_POINT ( 'NONE',  ( -1.655278471875002211, 14.63297358603754539, -75.68493913623279923 ) ) ;
#21533=CARTESIAN_POINT ( 'NONE',  ( -3.500000000000000888, 19.52072594216371826, -126.0443141357548313 ) ) ;
#21534=CARTESIAN_POINT ( 'NONE',  ( 3.310556943750001313, 19.41135094264166838, -113.1807724695661221 ) ) ;
#21538=CARTESIAN_POINT ( 'NONE',  ( 2.474675557024783212E-16, 21.54145188432739744, -78.21098080242151696 ) ) ;
#21539=CARTESIAN_POINT ( 'NONE',  ( 4.648177544792955347E-16, 21.00000000000001421, -60.21098080242150274 ) ) ;
#21540=CARTESIAN_POINT ( 'NONE',  ( -1.655278471874999990, 20.36702641396248836, -49.93077246956615056 ) ) ;
#21541=CARTESIAN_POINT ( 'NONE',  ( 1.655278471874998436, 14.63297358603754716, -104.5182724695661278 ) ) ;
#21543=CARTESIAN_POINT ( 'NONE',  ( -1.750000000000002220, 14.46891108675448123, -79.79431413575484555 ) ) ;
#21544=CARTESIAN_POINT ( 'NONE',  ( 1.655278471874998436, 14.63297358603754894, -122.5182724695661278 ) ) ;
#21547=CARTESIAN_POINT ( 'NONE',  ( 1.749999999999998224, 14.46891108675447590, -50.62764746908816704 ) ) ;
#21548=CARTESIAN_POINT ( 'NONE',  ( 0.000000000000000000, 17.49999999999990052, 850.4768413710875166 ) ) ;
#21549=CARTESIAN_POINT ( 'NONE',  ( -3.310556943750001313, 17.50000000000001421, -57.85160580289947063 ) ) ;
#21551=CARTESIAN_POINT ( 'NONE',  ( -3.310556943750000425, 19.41135094264166838, -74.93493913623279923 ) ) ;
#21557=CARTESIAN_POINT ( 'NONE',  ( 1.655278471874998436, 14.63297358603754006, -41.43077246956614346 ) ) ;
#21559=( BOUNDED_CURVE ( )  B_SPLINE_CURVE ( 2, ( #32292, #3158, #6972, #22719, #19946, #35697, #379, #32912, #3776 ),
 .UNSPECIFIED., .F., .F. ) 
 B_SPLINE_CURVE_WITH_KNOTS ( ( 3, 2, 2, 2, 3 ),
 ( 0.5312500000000000000, 0.5319444444444444420, 0.5333333333333333259, 0.5347222222222222099, 0.5354166666666666519 ),
 .UNSPECIFIED. ) 
 CURVE ( )  GEOMETRIC_REPRESENTATION_ITEM ( )  RATIONAL_B_SPLINE_CURVE ( ( 0.9330127018922194093, 0.9330127018922194093, 1.000000000000000000, 0.8660254037844387076, 1.000000000000000000, 0.8660254037844387076, 1.000000000000000000, 0.9330127018922194093, 0.9330127018922194093 ) ) 
 REPRESENTATION_ITEM ( '' )  );
#21561=ORIENTED_EDGE ( 'NONE', *, *, #27246, .T. ) ;
#21563=CARTESIAN_POINT ( 'NONE',  ( 1.655278471874998436, 14.63297358603754006, -47.43077246956614346 ) ) ;
#21564=ORIENTED_EDGE ( 'NONE', *, *, #20165, .T. ) ;
#21568=CARTESIAN_POINT ( 'NONE',  ( -3.500000000000002220, 15.47927405783632082, -24.87764746908817060 ) ) ;
#21570=CARTESIAN_POINT ( 'NONE',  ( 0.9378221735089281585, 14.00000000000001243, -63.36007260463891555 ) ) ;
#21572=CARTESIAN_POINT ( 'NONE',  ( 3.500000000000000000, 15.47927405783632793, -89.54431413575483134 ) ) ;
#21573=CARTESIAN_POINT ( 'NONE',  ( 3.500000000000000000, 15.47927405783632082, -37.54431413575484555 ) ) ;
#21575=DIRECTION ( 'NONE',  ( -0.000000000000000000, 1.259100132267607459E-16, -1.000000000000000000 ) ) ;
#21577=CARTESIAN_POINT ( 'NONE',  ( 2.340729813953370519E-16, 21.32270188528330479, -24.10160580289947063 ) ) ;
#21579=CARTESIAN_POINT ( 'NONE',  ( 3.310556943750001313, 19.41135094264167549, -130.1807724695661364 ) ) ;
#21582=CARTESIAN_POINT ( 'NONE',  ( 0.9378221735089300459, 21.00000000000001776, -93.94938900211595012 ) ) ;
#21583=CARTESIAN_POINT ( 'NONE',  ( -1.655278471874999990, 20.36702641396249547, -123.0182724695661278 ) ) ;
#21584=CARTESIAN_POINT ( 'NONE',  ( 3.500000000000000000, 15.47927405783633503, -134.2380641367107614 ) ) ;
#21585=CARTESIAN_POINT ( 'NONE',  ( -7.424026671074350129E-16, 13.45854811567263098, -36.40473080337743284 ) ) ;
#21588=CARTESIAN_POINT ( 'NONE',  ( -3.310556943750002201, 15.58864905735837958, -138.7682724695661420 ) ) ;
#21590=CARTESIAN_POINT ( 'NONE',  ( 3.310556943750001313, 19.41135094264166483, -47.26827246956613493 ) ) ;
#21592=CARTESIAN_POINT ( 'NONE',  ( 1.749999999999998224, 14.46891108675448301, -104.6276474690881741 ) ) ;
#21593=CARTESIAN_POINT ( 'NONE',  ( -3.310556943750001313, 17.50000000000001776, -74.85160580289947063 ) ) ;
#21595=CARTESIAN_POINT ( 'NONE',  ( -7.022189441860112050E-16, 13.67729811471672541, -104.5141058028994792 ) ) ;
#21596=CARTESIAN_POINT ( 'NONE',  ( 3.310556943750001313, 19.41135094264166128, -69.18077246956613635 ) ) ;
#21598=CARTESIAN_POINT ( 'NONE',  ( -3.310556943750001313, 17.50000000000001776, -93.85160580289947063 ) ) ;
#21600=CARTESIAN_POINT ( 'NONE',  ( 3.500000000000000000, 15.47927405783632437, -67.54431413575484555 ) ) ;
#21601=EDGE_CURVE ( 'NONE', #28293, #6435, #35290, .T. ) ;
#21604=CARTESIAN_POINT ( 'NONE',  ( -7.022189441860112050E-16, 13.67729811471672186, -55.51410580289947916 ) ) ;
#21605=CARTESIAN_POINT ( 'NONE',  ( -1.655278471875002211, 14.63297358603755072, -111.5974391362328078 ) ) ;
#21606=CARTESIAN_POINT ( 'NONE',  ( -0.9378221735089291577, 21.00000000000001776, -101.8600726046389013 ) ) ;
#21608=ORIENTED_EDGE ( 'NONE', *, *, #33482, .T. ) ;
#21610=VERTEX_POINT ( 'NONE', #17077 ) ;
#21612=CARTESIAN_POINT ( 'NONE',  ( 3.310556943749999981, 15.58864905735836537, -63.34743913623281486 ) ) ;
#21613=ORIENTED_EDGE ( 'NONE', *, *, #38381, .F. ) ;
#21614=ORIENTED_EDGE ( 'NONE', *, *, #37020, .F. ) ;
#21615=CYLINDRICAL_SURFACE ( 'NONE', #32765, 3.499999999999999556 ) ;
#21621=CARTESIAN_POINT ( 'NONE',  ( 2.340729813953370519E-16, 21.32270188528332255, -130.0141058028994507 ) ) ;
#21622=CARTESIAN_POINT ( 'NONE',  ( -1.749999999999999778, 20.53108891324555785, -103.1276474690881741 ) ) ;
#21623=CARTESIAN_POINT ( 'NONE',  ( 2.340729813953370519E-16, 21.32270188528330479, -42.10160580289947063 ) ) ;
#21624=CARTESIAN_POINT ( 'NONE',  ( 3.310556943750001313, 19.41135094264165772, -33.26827246956613493 ) ) ;
#21625=CARTESIAN_POINT ( 'NONE',  ( -7.022189441860112050E-16, 13.67729811471672363, -94.60160580289945642 ) ) ;
#21626=CARTESIAN_POINT ( 'NONE',  ( -3.500000000000001332, 17.50000000000001066, -23.65473080337743284 ) ) ;
#21629=CARTESIAN_POINT ( 'NONE',  ( -3.310556943750002645, 15.58864905735837958, -136.7682724695661420 ) ) ;
#21631=CARTESIAN_POINT ( 'NONE',  ( 1.749999999999998224, 14.46891108675448834, -136.3213974700441042 ) ) ;
#21632=CARTESIAN_POINT ( 'NONE',  ( 1.655278471874998436, 14.63297358603754184, -60.43077246956614346 ) ) ;
#21633=CARTESIAN_POINT ( 'NONE',  ( 0.9378221735089281585, 14.00000000000002309, -132.3600726046389013 ) ) ;
#21634=CARTESIAN_POINT ( 'NONE',  ( -1.749999999999999778, 20.53108891324555429, -81.82139747004410424 ) ) ;
#21635=CARTESIAN_POINT ( 'NONE',  ( -1.655278471874999990, 20.36702641396248836, -67.01827246956612782 ) ) ;
#21637=CARTESIAN_POINT ( 'NONE',  ( -8.715332896486792803E-15, 21.00000000000002842, -137.2109808024214885 ) ) ;
#21640=VERTEX_POINT ( 'NONE', #33671 ) ;
#21642=CARTESIAN_POINT ( 'NONE',  ( -3.310556943750002201, 15.58864905735837780, -119.6807724695661364 ) ) ;
#21645=ORIENTED_EDGE ( 'NONE', *, *, #8959, .F. ) ;
#21646=CARTESIAN_POINT ( 'NONE',  ( 1.750000000000001110, 20.53108891324555785, -115.9880641367107614 ) ) ;
#21647=CARTESIAN_POINT ( 'NONE',  ( 3.369928719974892676E-15, 14.00000000000002309, -139.7109808024214885 ) ) ;
#21652=CARTESIAN_POINT ( 'NONE',  ( 1.655278471875001101, 20.36702641396248836, -69.09743913623280775 ) ) ;
#21654=CARTESIAN_POINT ( 'NONE',  ( -1.749999999999999778, 20.53108891324555429, -79.12764746908817415 ) ) ;
#21656=ORIENTED_EDGE ( 'NONE', *, *, #40455, .T. ) ;
#21657=CARTESIAN_POINT ( 'NONE',  ( -1.655278471874999990, 20.36702641396248481, -24.93077246956613990 ) ) ;
#21659=CARTESIAN_POINT ( 'NONE',  ( 2.340729813953370519E-16, 21.32270188528331190, -80.01410580289946495 ) ) ;
#21662=VERTEX_POINT ( 'NONE', #1337 ) ;
#21663=CARTESIAN_POINT ( 'NONE',  ( -3.500000000000000000, 19.52072594216371826, -128.0443141357548313 ) ) ;
#21665=CARTESIAN_POINT ( 'NONE',  ( 3.500000000000001332, 17.50000000000002132, -102.4609808024215027 ) ) ;
#21666=AXIS2_PLACEMENT_3D ( 'NONE', #1455, #4220, #1657 ) ;
#21667=( BOUNDED_SURFACE ( )  B_SPLINE_SURFACE ( 1, 2, ( 
 ( #29069, #9738, #25896, #12918, #22698, #6539, #3340, #16328, #10770, #23973, #783, #7583, #20558, #7801, #3964, #33310, #4395, #23753, #10569, #33533, #39908, #36508, #13967, #17373, #13757, #7370, #8004, #20776, #4600, #40116, #26736, #30333, #30543, #17579, #1206, #1412, #33746, #20343, #14386, #14173, #27363, #40335, #4177, #37152, #16944, #11198, #36718, #20974, #33947, #27149, #10985, #36939, #17161, #30123, #23549, #24182, #4806, #33097, #29912, #39696, #999, #26946, #4096, #29619, #41987, #29833, #35798, #700, #7080, #26440, #10272, #23240, #36208, #38784, #13255, #19428, #13671, #6660, #33233, #39612, #23030, #20058, #26241, #9657, #39396, #486, #39190, #20266, #29404, #22617, #35596, #33022, #36431, #12836, #3464, #16247, #19625, #19837, #10483, #3888, #16869, #23468, #26653, #29189, #67, #7296, #28990, #32805, #6458, #273, #35999, #6865, #32397, #25820, #3263, #13046, #26027, #3674, #10067, #13456, #38991, #9874, #22829, #32598, #16454, #16660, #20696, #4315, #11125, #1132, #23897, #40042, #14735, #7933, #14527, #40467, #33673, #17506, #27499, #39837, #26865, #30469, #24106, #37078, #23682, #30044, #11322, #24308, #20485, #33872, #1339, #30681, #33451, #13885, #17710, #37277, #1546, #10697, #4525, #17296, #20899, #14103, #36865, #10911, #27694, #4732, #8130, #21109, #14312, #27291, #34081, #36644, #40256, #4938, #917, #27076, #17918, #30895, #30260, #1755, #40664, #7724, #11521, #24514, #7509, #37483, #8337, #21317, #34287, #17079, #27901, #12149, #22151, #38310, #38106, #9175, #28526, #31300, #5986, #41302, #12367, #2796, #2159, #41724, #1952, #35122, #21728, #12578, #38524, #21935, #5567, #28316, #34494, #28109, #8547, #41516, #22353, #9390, #18128, #15780, #28728, #25563, #31098, #5780, #14933, #18960, #11942, #40876, #25351, #2583, #11730, #24727, #37690, #21525, #31510, #5352, #18329, #24937, #15145, #41093, #25141, #37895, #2379, #8754, #15568, #18756, #15368, #18541, #34912, #31715, #41936, #39342, #643, #19170, #9820, #22565, #25978, #26190, #3838, #13407, #434, #16816, #23191, #35542, #6406, #29781, #10220, #39140, #16199, #32971, #10020, #32754, #16611, #38942, #35751, #3622, #15998, #32550, #29571, #6195, #32350, #29351, #22780, #38733, #3417, #6614, #19377, #19577, #16408, #28939, #3214, #13617, #26390, #36156, #35950, #12784, #222, #7029, #20007, #22983, #26600, #39559, #29142, #10437, #13204, #35330, #32142, #18, #3006, #25767, #9604, #6814, #12999, #19788, #14260, #10857, #4478, #10650, #4261, #26817, #4682, #40612, #14680, #27642, #34031, #4884, #17865, #23414, #24054, #36379, #24254, #30207, #37224, #1492, #20850, #17661, #30626, #14469, #33179, #7669, #13835, #8078, #1084, #7246, #30836, #17460, #27444, #20643, #4045, #33824, #37024, #33622, #20219, #23841, #17027, #29991, #40411, #1701, #863, #39990, #23628, #14055, #27238, #39785, #11271, #21055, #36592, #7455, #20431, #33395, #17245, #27027, #40200, #36809, #30419, #1289, #11071, #7882, #24462, #5727, #18705, #14879, #28265, #37841, #25086, #27848, #8286, #12092, #31664, #38049, #5092, #15094, #40825, #5513, #37635, #18275, #34234, #15515, #28470, #11889, #2741, #8698, #2530, #41461, #41037, #24881, #21671, #31248, #1898, #21262, #8492, #28679, #31044, #18073, #15312, #11676, #34858, #2109, #25295, #34648, #18487, #31456, #24675, #28055, #35073, #15726, #12310, #2325, #21467, #41249, #5933, #8910, #34442, #21882, #38258, #9121, #22102, #18905, #31872, #5301, #11470, #37430, #16568, #29523, #22730, #29305, #174, #38682, #32302, #26143, #16774, #6355, #41672, #39296, #6771, #29098, #9773, #39095, #35707, #22304, #6570, #12528, #389, #13366, #10178, #15945, #3168, #6142, #19121, #6986, #22512, #19745, #9340, #19535, #32924, #16159, #35496, #42097, #26347, #19961, #12951, #19327, #2954, #23146, #32088, #13156, #32506, #3575, #36114, #32712, #35278, #25719, #28895, #3791, #25512, #38477, #41889, #3376, #25930, #12740, #9554, #16362, #38894, #9975, #22938, #35904, #24215, #4216, #7621, #17199, #597, #26981, #36980, #33572, #4433, #13573, #11231, #14423, #27190, #20382, #30160, #33985, #26557, #8038, #4842, #27400, #7840, #1037, #39944, #14212, #23792, #10393, #36759, #39514, #17618, #4640, #40370, #3998, #33348, #36330, #7202, #37183, #10607, #20810, #23367, #20597, #21010, #14010, #23585, #10808, #1452, #29734, #17414, #36544, #33134, #20175, #16982, #30373, #1244, #33784, #29946, #30582, #819, #13793, #26773, #39736, #7408, #40156, #11024, #24010, #11631, #27604, #1652, #11841, #37591, #21841, #25042, #25248, #12263, #34397, #37797, #5257, #30791, #15047, #38005, #21625, #34602, #14637, #41414, #2487, #15262, #8443, #18232, #22053, #40571, #38214, #11426, #34814, #5683, #31202, #9077, #2062, #8866, #18657, #28012, #40992, #24839, #24626, #8241, #24417, #14837, #35026, #37384, #21216, #5465, #34187, #41208, #21420, #31622, #8653, #18443, #31412, #18024, #2279, #17818, #5045, #15471, #28220, #1857, #12049, #31003, #28425, #27805, #40778, #22681, #3120, #12694, #25674, #16311, #25465, #6718, #35444, #22888, #35854, #29053, #35657, #6520, #2908, #38634, #32457, #23093, #9501, #19690, #32660, #3523, #22258, #22463, #12480, #38429, #13314, #28843, #26089, #15680, #12901, #39245, #6304, #41842, #19281, #16517, #26300, #32254, #16111, #9292, #29466, #35231, #19488, #42049, #9931, #335, #39047, #28638, #32040, #6092, #10126, #18861, #5888, #19070, #25880, #38842, #41625, #31822, #9719, #3323, #2693, #13104, #15899, #29251, #125, #13949, #23530, #6929, #33291, #1185, #39890, #10751, #19904, #17561, #20758, #33512, #26714, #10548, #40882, #32871, #14940, #16720, #40099, #10966, #36490, #27909, #20324, #14155, #23953, #7352, #4157, #17140, #762, #26504, #3734, #33080, #11738, #13517, #546, #23736, #39462, #17354, #13737, #7783, #30103, #979, #26926, #36274, #39679, #30526, #36061, #36919, #36700, #20117, #7564, #1394, #20538, #23312, #4376, #30316, #27131, #33729, #4582, #29680, #10336, #7147, #3945, #16927, #29893, #5788, #12372, #25358, #21735, #15376, #9181, #41942, #31517, #24733, #22358, #31931, #12157, #34918, #22159, #18761, #5358, #31720, #37698, #2589, #15573, #24943, #28323, #6201, #16003, #12584, #28532, #8761, #2386, #19176, #41522, #11950, #41309, #38316, #21942, #25148, #38113, #35128, #2167, #25568, #8970, #41729, #38530, #5991, #18965, #2804, #34709, #15785, #28734, #8554, #9396, #21532, #35336, #32148, #3012, #28945, #34500, #18336, #31308, #15152, #28116, #41100, #37905, #5574, #18549, #16413, #19382, #32355, #20223, #35758, #32976, #22571, #19793, #4050, #3420, #6617, #227, #26606, #33186, #29357, #19580, #16203, #23419, #3218, #440, #22987, #16823, #39565, #3843, #35549, #38949, #23, #10443, #25772, #29786, #29146, #32759, #32553, #6411, #38738, #6819, #13208, #650, #20011, #17035, #7251, #26196, #3628, #39144, #9610, #10026, #13623, #16615, #29575, #13004, #36384, #29998, #10225, #35955, #13411, #12790, #25983, #9826, #22784, #26396, #39346, #23196, #36161, #7034, #21060, #30844, #30423, #14265, #27243, #7675, #33403, #10655, #39995, #18077, #20436, #7462, #4686, #4266, #24258, #20649, #14687, #11075, #23634, #7886, #34238, #33626, #23850, #1293, #27645, #21266, #4482, #36815, #17250, #11473, #30212, #30632, #24062, #4890, #40615, #34036, #36597, #27033, #1089, #24465, #13841, #17869, #14060, #20854, #17464, #10862, #26822, #37028, #40207, #1705, #8083, #8290, #37435, #33828, #17666, #1497, #39790, #14476, #5098, #27449, #40417, #11275, #869, #37228, #28475, #21678, #5518, #35283, #14883, #9343, #11680, #35076, #5936, #31459, #22308, #15315, #9126, #18909, #18490, #2328, #28270, #37847, #21473, #40828, #28059, #6146, #8495, #37639, #34861, #34445, #12315, #8702, #2746, #41252, #38054, #25090, #31251, #34651, #12531, #31049, #31876, #21885, #15098, #12098, #25515, #8913, #18279, #5732, #18708, #31667, #2534, #15518, #41464, #5306, #15729, #25298, #28684, #41676, #38261, #22105, #38480, #41041, #1901, #27851, #24678, #2113, #11893, #24884, #24728, #4939, #27695, #1953, #11522, #40257, #24515, #30470, #5353, #34495, #15146, #33873, #21110, #24107, #37079, #24938, #40468, #37691, #18330, #37484, #8548, #2160, #1547, #11943, #14313, #21526, #34082, #37896, #8755, #8338, #17919, #40665, #4733, #11323, #20900, #40877, #34703, #21729, #17507, #28110, #41094, #1340, #27292, #18129, #11126, #31301, #24309, #7934, #17711, #14934, #11731, #30682, #14528, #27500, #1756, #37278, #8131, #30896, #14736, #21318, #34288, #5152, #31099, #27902, #3007, #19171, #2797, #38943, #5987, #15369, #12150, #9605, #13000, #31511, #22152, #34913, #38311, #38525, #16200, #25768, #12785, #29143, #35543, #5781, #18757, #19, #22566, #9391, #28317, #18961, #12579, #25564, #25142, #18542, #41937, #38734, #8964, #22354, #31926, #32143, #21936, #2380, #6196, #6407, #15999, #41303, #9176, #31716, #41725, #2584, #12368, #28527, #3215, #35331, #28940, #19378, #35123, #15781, #32351, #38107, #28729, #25979, #15569, #41517, #9821, #22781, #25352, #5568, #39942, #36541, #26979, #33569, #16979, #23582, #1650, #14419, #27397, #36977, #29943, #1241, #11229, #40368, #27187, #24213, #17615, #20380, #37181, #40153, #11020, #20172, #30789, #21008, #33780, #10805, #23789, #11424, #33131, #14635, #817, #8035, #33983, #36756, #27602, #20594, #4840, #35752, #7617, #4430, #17410, #1034, #26769, #3996, #33345, #7199, #13790, #39733, #24007, #10605, #30579, #14007, #7406, #30370, #14209, #7837, #4213, #20807, #17196, #30157, #4637, #15260, #8441, #31199, #18859, #18440, #11630, #40990, #41206, #21623, #2060, #15045, #34810, #1855, #25246, #11839, #41412, #12261, #5462, #12047, #25040, #21418, #28009, #8864, #41622, #24837, #24414, #22050, #31620, #37795, #34600, #21838, #31408, #5043, #2277, #37382, #38210, #9074, #35024, #40775, #8651, #31001, #14835, #31820, #5255, #2485, #34185, #28218, #15678, #38003, #18230, #5680, #5886, #2691, #18656, #15469, #27803, #28636, #24623, #28423, #8239, #21213, #18022, #37589, #34395, #38632, #41839, #10124, #25462, #16514, #15897, #19486, #6302, #22256, #38426, #6518, #32252, #29464, #19687, #19902, #6927, #29050, #32454, #42047, #9290, #9716, #3320, #9499, #19279, #35442, #23090, #16309, #9929, #35852, #16108, #12899, #22886, #35229, #22679, #32658, #6090, #22461, #29249, #25878, #28840, #35655, #38840, #12691, #3117, #123, #19068, #25672, #32869, #3521, #333, #13101, #32038, #26087, #13313, #26298, #39045, #39243, #36058, #3732, #16718, #29678, #12477, #2905, #26711, #37132, #39459, #33727, #17138, #7985, #33928, #33509, #30099, #23734, #29891, #23528, #3943, #23951, #17766, #4788, #544, #11180, #24163, #20957, #13515, #1183, #26502, #1392, #7350, #14367, #20755, #40097, #36916, #7781, #4580, #10334, #26924, #33078, #27341, #20322, #23308, #36272, #36698, #17559, #39888, #7145, #10964, #14153, #10749, #20115, #977, #16925, #760, #30524, #13734, #39677, #13947, #10546, #33289, #4373, #36488, #40313, #4155, #7562, #20536, #17352, #30314, #27129, #5626, #34551, #40522, #2009, #37747, #8604, #37333, #1601, #24991, #37955, #34133, #5412, #14992, #2224, #4993, #27556, #31358, #8816, #15203, #24362, #34346, #17973, #28168, #21786, #41154, #8186, #5206, #30950, #24786, #14787, #37535, #11577, #28373, #21577, #12001, #34758, #18181, #31150, #18604, #11379, #27957, #31567, #14582 ),
 ( #9021, #21369, #24570, #1807, #41359, #21160, #18390, #40934, #2436, #15420, #12210, #27750, #40720, #8390, #25200, #11790, #38161, #21998, #34974, #5837, #30738, #2640, #12843, #38578, #22835, #26035, #26247, #13263, #35388, #38791, #6252, #31768, #16056, #38997, #22625, #35604, #15627, #280, #3470, #16256, #9443, #19228, #23037, #28584, #39195, #41571, #35803, #6665, #32200, #10072, #3064, #9880, #19633, #28997, #41995, #25827, #25619, #9238, #12425, #15842, #36006, #38372, #25409, #6466, #22206, #73, #22411, #32607, #9663, #19434, #32403, #19018, #3269, #18808, #35175, #16461, #29195, #2852, #13052, #6041, #29411, #31986, #28786, #41784, #12637, #13678, #26658, #17302, #26447, #7730, #36437, #23902, #36870, #30051, #36652, #7516, #3893, #39619, #33458, #24114, #10490, #6873, #4531, #14109, #7301, #17087, #4321, #925, #29626, #13892, #19844, #20704, #33680, #17511, #23249, #23475, #13461, #39402, #14319, #29839, #27082, #16668, #26872, #40263, #20272, #706, #33239, #30476, #27298, #4103, #39842, #10278, #1346, #36214, #20490, #10704, #10918, #11133, #40049, #492, #33028, #7088, #32811, #3682, #20066, #16875, #23688, #30267, #1138, #20907, #31104, #14743, #41101, #2168, #2387, #31518, #11529, #14941, #24521, #7939, #34295, #15153, #40883, #11739, #33879, #18550, #21736, #34501, #27700, #37489, #41310, #4740, #15377, #17718, #11951, #24944, #8344, #28324, #21323, #28117, #37906, #5160, #18134, #1958, #1762, #27506, #30688, #34087, #12158, #14534, #1554, #24734, #40474, #18337, #40670, #8762, #27910, #5575, #34710, #37085, #11329, #37284, #8139, #21116, #4945, #17925, #37699, #30902, #8555, #21533, #5359, #31309, #38114, #19383, #32356, #28533, #41943, #9397, #38739, #41523, #21943, #25773, #3219, #9611, #18762, #28735, #12373, #19177, #9182, #31932, #5992, #22785, #16004, #22572, #6412, #41730, #25569, #35550, #5789, #22359, #16204, #8971, #22160, #32149, #12585, #25359, #35337, #38531, #38317, #15786, #6202, #31721, #35129, #32554, #29147, #24, #13005, #2590, #3013, #25984, #38950, #28946, #9827, #35759, #18966, #6618, #12791, #19581, #3421, #2805, #16414, #34919, #29358, #228, #25149, #15574, #4051, #651, #36385, #441, #36162, #16616, #36598, #30424, #4483, #17465, #23851, #36816, #7676, #13209, #13842, #26197, #14061, #20012, #27034, #33404, #10656, #7463, #20437, #4267, #22988, #39566, #3629, #39996, #32977, #39145, #20650, #7252, #17251, #10444, #35956, #23635, #26823, #23420, #10027, #13624, #6820, #19794, #30213, #33627, #32760, #29787, #13412, #3844, #26607, #29576, #26397, #1090, #39347, #10226, #20224, #23197, #16824, #17036, #7035, #10863, #33187, #29999, #870, #39791, #1498, #37848, #18280, #5099, #11076, #14688, #8291, #21267, #7887, #14266, #37640, #8496, #4687, #18078, #27646, #14884, #17667, #40208, #1902, #21474, #27852, #37029, #4891, #30633, #37436, #27450, #8084, #24259, #41042, #34239, #40829, #24679, #17870, #1706, #11681, #24063, #40616, #34446, #27244, #40418, #31050, #30845, #14477, #11474, #24466, #11276, #34037, #5307, #20855, #37229, #8704, #31252, #2114, #15099, #33829, #28060, #11894, #24885, #21679, #34652, #5519, #21061, #18491, #1294, #38687, #16162, #15519, #25934, #28271, #22515, #5937, #38898, #22735, #22309, #18910, #12532, #18709, #12316, #34862, #12744, #6573, #35711, #31460, #42101, #12954, #9777, #2329, #32092, #15316, #32305, #38262, #3174, #9558, #28899, #25724, #35500, #6358, #41253, #15730, #21886, #29102, #9127, #12099, #25091, #25516, #19333, #28685, #38055, #41895, #2960, #41677, #8914, #31877, #5733, #31668, #38481, #19127, #15950, #28476, #22106, #2535, #41465, #35077, #25299, #2747, #9344, #35284, #6147, #4003, #13577, #180, #26561, #32509, #7415, #36548, #17203, #35909, #23149, #26148, #39098, #26986, #394, #39743, #29308, #39518, #10812, #10182, #13369, #6989, #33353, #39948, #36117, #26351, #22941, #30165, #9979, #7207, #29738, #23589, #4221, #10610, #13160, #3578, #6775, #1042, #3380, #20387, #19748, #10397, #39302, #32715, #16365, #23371, #19965, #14015, #26778, #23799, #36763, #32930, #36336, #3795, #16573, #16780, #19538, #20179, #33140, #29527, #602, #16988, #29951, #824, #13797, #12431, #33579, #28591, #30378, #11637, #24633, #8042, #41577, #33992, #27812, #37597, #37187, #21016, #4846, #14430, #40162, #17419, #4644, #25415, #27196, #14217, #11431, #11029, #31009, #27405, #21431, #17825, #14645, #1658, #7845, #40375, #31774, #7626, #8451, #40576, #33788, #11236, #2646, #27608, #36985, #24218, #24423, #30798, #37390, #8247, #18033, #24014, #34403, #21223, #20601, #18814, #34194, #40784, #5054, #1248, #1863, #14842, #5263, #4439, #15634, #20815, #17622, #30587, #1456, #22213, #12850, #25625, #29005, #29202, #6877, #16466, #3476, #19850, #26252, #38585, #9450, #32817, #13269, #78, #6047, #9670, #3276, #16262, #2858, #9243, #32612, #29416, #41792, #13058, #22633, #9885, #12645, #35181, #39003, #286, #22840, #31993, #42001, #22417, #32410, #35395, #3070, #19234, #36012, #26041, #35808, #19640, #25832, #38797, #6671, #19025, #35609, #39200, #15848, #6259, #10078, #6472, #32206, #19440, #23044, #16064, #3687, #16675, #28792, #29632, #497, #13466, #38380, #27086, #7094, #33462, #1350, #17515, #17308, #30480, #7734, #10496, #27303, #20494, #33685, #11137, #23480, #20911, #23254, #14323, #929, #33883, #17722, #30271, #13896, #7520, #13683, #7306, #29844, #20708, #1559, #30692, #26452, #37089, #7944, #4744, #39408, #40053, #10284, #40268, #33243, #24118, #4535, #23906, #36220, #20071, #33033, #3899, #10708, #16880, #711, #26663, #39624, #36443, #20277, #10922, #4108, #4325, #17091, #30055, #1143, #26877, #39846, #23692, #36657, #14113, #36874, #41316, #40676, #8978, #11333, #5582, #31109, #21949, #5794, #5364, #1963, #37704, #1767, #37494, #17931, #37910, #31726, #18768, #14538, #25154, #38119, #34924, #27510, #15158, #40478, #15382, #21328, #28330, #34714, #11956, #8767, #21740, #18554, #24320, #40889, #4949, #12163, #34302, #37289, #8144, #8561, #31523, #11744, #21120, #24950, #28122, #24739, #34091, #14947, #30907, #14748, #2392, #27705, #11534, #27915, #24527, #5165, #18342, #8349, #18139, #21538, #34506, #31316, #2175, #41108, #39150, #19587, #6417, #12380, #16009, #9616, #22580, #9187, #15579, #38956, #9832, #5997, #19389, #28952, #16208, #18971, #41528, #3225, #22790, #29152, #38323, #6208, #31938, #38745, #28740, #9402, #25574, #234, #35555, #29, #25991, #19182, #3018, #13011, #25366, #41948, #35763, #28538, #41736, #32361, #32154, #2810, #12796, #25778, #15793, #35342, #6624, #22165, #32559, #12591, #3426, #16419, #38536, #29365, #13216, #35134, #22365, #10032, #26202, #22992, #35962, #6825, #19798, #2594, #23857, #23642, #36822, #14067, #16829, #33634, #26828, #40003, #17471, #29792, #27252, #29582, #7684, #7258, #40214, #24069, #36605, #20230, #13847, #20018, #13629, #36169, #27040, #7894, #37035, #32768, #1300, #14272, #11085, #3635, #33410, #16622, #4489, #39574, #30430, #10870, #30219, #20656, #446, #13417, #26402, #17041, #23202, #39352, #10449, #10232, #7040, #39797, #32983, #30004, #3850, #1096, #4275, #877, #656, #33192, #26613, #23425, #36391, #4056, #10662, #7469, #20442, #17258, #11687, #31469, #41048, #28068, #2336, #8711, #21068, #34042, #15323, #37854, #24686, #30641, #34246, #27858, #40835, #27457, #33836, #15105, #11900, #24267, #37647, #5106, #34452, #37237, #17674, #21480, #24892, #5313, #14485, #24473, #8091, #14890, #4899, #27653, #1712, #18499, #8503, #18286, #2121, #37443, #21277, #31258, #1506, #18085, #21685, #4694, #17879, #34658, #5525, #8298, #28278, #12106, #41261, #31057, #1909, #30852, #14695, #40624, #25099, #38062, #20863, #40423, #11283, #11482, #3386, #26155, #9566, #21893, #9784, #15737, #22742, #29109, #6366, #32314, #3182, #16170, #18716, #35293, #41473, #35718, #28691, #13168, #19545, #2966, #42108, #6155, #31675, #19340, #22523, #19134, #188, #9350, #2543, #15527, #12961, #16373, #34872, #25524, #38269, #41683, #41903, #32517, #25942, #38906, #29316, #6580, #9134, #22111, #8921, #5740, #12751, #28483, #22316, #15957, #28906, #12323, #25306, #35083, #5943, #18917, #25731, #32100, #35507, #31884, #2753, #12538, #38488, #38695, #32722, #609, #26358, #33148, #23158, #3804, #19972, #36773, #29958, #36558, #20398, #13584, #39528, #7423, #19756, #36343, #33361, #9986, #36124, #4012, #26568, #402, #7216, #10405, #39309, #29746, #20188, #3586, #10188, #4449, #4230, #30175, #39751, #16581, #16996, #14024, #1051, #832, #26994, #17212, #6996, #39958, #13806, #10823, #23808, #32939, #33588, #35916, #7635, #20609, #29536, #16787, #23381, #17429, #22948, #30387, #13377, #26786, #10618, #6783, #23598, #1257, #14227, #39106, #14851, #31218, #18246, #34001, #11441, #4855, #27206, #14654, #27821, #8256, #21232, #11039, #2079, #21439, #31018, #21025, #17833, #28027, #24021, #15063, #7855, #11646, #24642, #30807, #40170, #40585, #37605, #34413, #27617, #24432, #37400, #1668, #1465, #33797, #37197, #36994, #14440, #27415, #18043, #40384, #8460, #34203, #20825, #5063, #1871, #40793, #5273, #4652, #17631, #30597, #11245, #24227, #8051, #29886, #17553, #17133, #10327, #39667, #39882, #20317, #753, #13725, #33504, #537, #23946, #10541, #40093, #10960, #4149, #10744, #23730, #20109, #26705, #7557, #40307, #23520, #23085, #20750, #30307, #36482, #33284, #20532, #30094, #3727, #972, #36052, #36912, #7775, #33723, #39452, #7345, #29672, #13509, #30518, #3938, #1180, #32861, #13940, #14363, #26920, #16920, #36694, #4574, #1387, #4366, #17348, #26497, #27337, #23300, #14148, #27123, #6918, #16711, #19896, #36265, #7138, #33072, #15415, #21781, #5202, #2218, #37528, #33923, #8599, #24779, #8385, #2430, #11572, #20950, #17762, #15197, #18596, #37128, #27744, #40516, #1802, #2004, #34752, #31353, #18384, #5621, #41148, #11374, #24357, #31559, #28159, #14988, #4781, #24566, #18177, #31146, #30733, #24159, #5406, #11995, #14577, #27952, #21366, #37742, #27552, #7981, #11783, #24986, #21573, #1597, #14783, #37327, #40927, #8182, #17968, #34129, #8809, #34544, #37948, #28367, #40715, #34342, #11175, #21154, #4988, #30946, #12205, #38365, #35383, #28780, #2633, #38573, #2847, #41566, #31978, #9438, #21992, #28579, #6661, #6459, #32398, #41988, #34963, #6246, #16248, #3264, #32194, #29190, #22618, #25403, #68, #19223, #19429, #26028, #9231, #35799, #38156, #13047, #15837, #19626, #32599, #3058, #41776, #22405, #12419, #22201, #15621, #35597, #16455, #3465, #41353, #9875, #22830, #25195, #9015, #12837, #5832, #38992, #6035, #18803, #31763, #38785, #35170, #19011, #12632, #25611, #16050, #28991, #25821, #9658, #10698, #36209, #1133, #39613, #36432, #23469, #29620, #20059, #10912, #20697, #17297, #20267, #13457, #7081, #23898, #7297, #16661, #3889, #4097, #26654, #33023, #16870, #39838, #6866, #30261, #29834, #4316, #14104, #10484, #17080, #30045, #26441, #701, #13886, #4526, #13672, #29405, #27077, #36645, #33234, #918, #26866, #23683, #10068, #7510, #274, #40043, #36866, #7725, #3675, #20486, #36000, #19838, #33674, #10273, #33452, #39191, #13256, #26242, #23031, #23241, #32806, #487, #39397, #2000, #5197, #14778, #21988, #17962, #41143, #21568, #15411, #25192, #2423, #34124, #21361, #40710, #9011, #8176, #28364, #27740, #18379, #18173, #4983, #11567, #5401, #14984, #41349 ) ),
 .UNSPECIFIED., .F., .F., .T. ) 
 B_SPLINE_SURFACE_WITH_KNOTS ( ( 2, 2 ),
 ( 3, 2, 2, 2, 2, 2, 2, 2, 2, 2, 2, 2, 2, 2, 2, 2, 2, 2, 2, 2, 2, 2, 2, 2, 2, 2, 2, 2, 2, 2, 2, 2, 2, 2, 2, 2, 2, 2, 2, 2, 2, 2, 2, 2, 2, 2, 2, 2, 2, 2, 2, 2, 2, 2, 2, 2, 2, 2, 2, 2, 2, 2, 2, 2, 2, 2, 2, 2, 2, 2, 2, 2, 2, 2, 2, 2, 2, 2, 2, 2, 2, 2, 2, 2, 2, 2, 2, 2, 2, 2, 2, 2, 2, 2, 2, 2, 2, 2, 2, 2, 2, 2, 2, 2, 2, 2, 2, 2, 2, 2, 2, 2, 2, 2, 2, 2, 2, 2, 2, 2, 2, 2, 2, 2, 2, 2, 2, 2, 2, 2, 2, 2, 2, 2, 2, 2, 2, 2, 2, 2, 2, 2, 2, 2, 2, 2, 2, 2, 2, 2, 2, 2, 2, 2, 2, 2, 2, 2, 2, 2, 2, 2, 2, 2, 2, 2, 2, 2, 2, 2, 2, 2, 2, 2, 2, 2, 2, 2, 2, 2, 2, 2, 2, 2, 2, 2, 2, 2, 2, 2, 2, 2, 2, 2, 2, 2, 2, 2, 2, 2, 2, 2, 2, 2, 2, 2, 2, 2, 2, 2, 2, 2, 2, 2, 2, 2, 2, 2, 2, 2, 2, 2, 2, 2, 2, 2, 2, 2, 2, 2, 2, 2, 2, 2, 2, 2, 2, 2, 2, 2, 2, 2, 2, 2, 2, 2, 2, 2, 2, 2, 2, 2, 2, 2, 2, 2, 2, 2, 2, 2, 2, 2, 2, 2, 2, 2, 2, 2, 2, 2, 2, 2, 2, 2, 2, 2, 2, 2, 2, 2, 2, 2, 2, 2, 2, 2, 2, 2, 2, 2, 2, 2, 2, 2, 2, 2, 2, 2, 2, 2, 2, 2, 2, 2, 2, 2, 2, 2, 2, 2, 2, 2, 2, 2, 2, 2, 2, 2, 2, 2, 2, 2, 2, 2, 2, 2, 2, 2, 2, 2, 2, 2, 2, 2, 2, 2, 2, 2, 2, 2, 2, 2, 2, 2, 2, 2, 2, 2, 2, 2, 2, 2, 2, 2, 2, 2, 2, 2, 2, 2, 2, 2, 2, 2, 2, 2, 2, 2, 2, 2, 2, 2, 2, 2, 2, 2, 2, 2, 2, 2, 2, 2, 2, 2, 2, 2, 2, 2, 2, 2, 2, 2, 2, 2, 2, 2, 2, 2, 2, 2, 2, 2, 2, 2, 2, 2, 2, 2, 2, 2, 2, 2, 2, 2, 2, 2, 2, 2, 2, 2, 2, 2, 2, 2, 2, 2, 2, 2, 2, 2, 2, 2, 2, 2, 2, 2, 2, 2, 2, 2, 2, 2, 2, 2, 2, 2, 2, 2, 2, 2, 2, 2, 2, 2, 2, 2, 2, 2, 2, 2, 2, 2, 2, 2, 2, 2, 2, 2, 2, 2, 2, 2, 2, 2, 2, 2, 2, 2, 2, 2, 2, 2, 2, 2, 2, 2, 2, 2, 2, 2, 2, 2, 2, 2, 2, 2, 2, 2, 2, 2, 2, 2, 2, 2, 2, 2, 2, 2, 2, 2, 2, 2, 2, 2, 2, 2, 2, 2, 2, 2, 2, 2, 2, 2, 2, 2, 2, 2, 2, 2, 2, 2, 2, 2, 2, 2, 2, 2, 2, 2, 2, 2, 2, 2, 2, 2, 2, 2, 2, 2, 2, 2, 2, 2, 2, 2, 2, 2, 2, 2, 2, 2, 2, 2, 2, 2, 2, 2, 2, 2, 2, 2, 2, 2, 2, 2, 2, 2, 2, 2, 2, 2, 2, 2, 2, 2, 2, 2, 2, 2, 2, 2, 2, 2, 2, 2, 2, 2, 2, 2, 2, 2, 2, 2, 2, 2, 2, 2, 2, 2, 2, 2, 2, 2, 2, 2, 2, 2, 2, 2, 2, 2, 2, 2, 2, 2, 2, 2, 2, 2, 2, 2, 2, 2, 2, 2, 2, 2, 2, 2, 2, 2, 2, 2, 2, 2, 2, 2, 2, 2, 2, 2, 2, 2, 2, 2, 2, 2, 2, 2, 2, 2, 2, 2, 2, 2, 2, 2, 2, 2, 2, 2, 2, 2, 2, 2, 2, 2, 2, 2, 2, 2, 2, 2, 2, 2, 2, 2, 2, 2, 2, 2, 2, 2, 2, 2, 2, 2, 2, 2, 2, 2, 2, 2, 2, 2, 2, 2, 2, 2, 2, 2, 2, 2, 2, 2, 2, 2, 2, 2, 3 ),
 ( 0.000000000000000000, 1.000000000000000000 ),
 ( 0.000000000000000000, 0.001388888888888888942, 0.002777777777777777884, 0.004166666666666666609, 0.005555555555555555768, 0.006944444444444444059, 0.008333333333333333218, 0.009722222222222222376, 0.01111111111111111154, 0.01250000000000000069, 0.01388888888888888812, 0.01527777777777777728, 0.01666666666666666644, 0.01805555555555555386, 0.01944444444444444475, 0.02083333333333333218, 0.02222222222222222307, 0.02361111111111111049, 0.02500000000000000139, 0.02638888888888888881, 0.02777777777777777624, 0.02916666666666666713, 0.03055555555555555455, 0.03194444444444444198, 0.03333333333333333287, 0.03472222222222222376, 0.03611111111111110772, 0.03749999999999999861, 0.03888888888888888951, 0.04027777777777778040, 0.04166666666666666435, 0.04305555555555555525, 0.04444444444444444614, 0.04583333333333333010, 0.04722222222222222099, 0.04861111111111111188, 0.05000000000000000278, 0.05138888888888888673, 0.05277777777777777762, 0.05416666666666666852, 0.05555555555555555247, 0.05694444444444444337, 0.05833333333333333426, 0.05972222222222222515, 0.06111111111111110911, 0.06250000000000000000, 0.06388888888888888395, 0.06527777777777778179, 0.06666666666666666574, 0.06805555555555554970, 0.06944444444444444753, 0.07083333333333333148, 0.07222222222222221544, 0.07361111111111111327, 0.07499999999999999722, 0.07638888888888889506, 0.07777777777777777901, 0.07916666666666666297, 0.08055555555555556080, 0.08194444444444444475, 0.08333333333333332871, 0.08472222222222222654, 0.08611111111111111049, 0.08749999999999999445, 0.08888888888888889228, 0.09027777777777777624, 0.09166666666666666019, 0.09305555555555555802, 0.09444444444444444198, 0.09583333333333333981, 0.09722222222222222376, 0.09861111111111110772, 0.1000000000000000056, 0.1013888888888888895, 0.1027777777777777735, 0.1041666666666666713, 0.1055555555555555552, 0.1069444444444444392, 0.1083333333333333370, 0.1097222222222222210, 0.1111111111111111049, 0.1125000000000000028, 0.1138888888888888867, 0.1152777777777777846, 0.1166666666666666685, 0.1180555555555555525, 0.1194444444444444503, 0.1208333333333333343, 0.1222222222222222182, 0.1236111111111111160, 0.1250000000000000000, 0.1263888888888888840, 0.1277777777777777679, 0.1291666666666666796, 0.1305555555555555636, 0.1319444444444444475, 0.1333333333333333315, 0.1347222222222222154, 0.1361111111111110994, 0.1375000000000000111, 0.1388888888888888951, 0.1402777777777777790, 0.1416666666666666630, 0.1430555555555555469, 0.1444444444444444309, 0.1458333333333333426, 0.1472222222222222265, 0.1486111111111111105, 0.1499999999999999944, 0.1513888888888888784, 0.1527777777777777901, 0.1541666666666666741, 0.1555555555555555580, 0.1569444444444444420, 0.1583333333333333259, 0.1597222222222222099, 0.1611111111111111216, 0.1625000000000000056, 0.1638888888888888895, 0.1652777777777777735, 0.1666666666666666574, 0.1680555555555555691, 0.1694444444444444531, 0.1708333333333333370, 0.1722222222222222210, 0.1736111111111111049, 0.1749999999999999889, 0.1763888888888889006, 0.1777777777777777846, 0.1791666666666666685, 0.1805555555555555525, 0.1819444444444444364, 0.1833333333333333204, 0.1847222222222222321, 0.1861111111111111160, 0.1875000000000000000, 0.1888888888888888840, 0.1902777777777777679, 0.1916666666666666796, 0.1930555555555555636, 0.1944444444444444475, 0.1958333333333333315, 0.1972222222222222154, 0.1986111111111110994, 0.2000000000000000111, 0.2013888888888888951, 0.2027777777777777790, 0.2041666666666666630, 0.2055555555555555469, 0.2069444444444444309, 0.2083333333333333426, 0.2097222222222222265, 0.2111111111111111105, 0.2124999999999999944, 0.2138888888888888784, 0.2152777777777777901, 0.2166666666666666741, 0.2180555555555555580, 0.2194444444444444420, 0.2208333333333333259, 0.2222222222222222099, 0.2236111111111111216, 0.2250000000000000056, 0.2263888888888888895, 0.2277777777777777735, 0.2291666666666666574, 0.2305555555555555691, 0.2319444444444444531, 0.2333333333333333370, 0.2347222222222222210, 0.2361111111111111049, 0.2374999999999999889, 0.2388888888888889006, 0.2402777777777777846, 0.2416666666666666685, 0.2430555555555555525, 0.2444444444444444364, 0.2458333333333333204, 0.2472222222222222321, 0.2486111111111111160, 0.2500000000000000000, 0.2513888888888888840, 0.2527777777777777679, 0.2541666666666666519, 0.2555555555555555358, 0.2569444444444444198, 0.2583333333333333592, 0.2597222222222222432, 0.2611111111111111271, 0.2625000000000000111, 0.2638888888888888951, 0.2652777777777777790, 0.2666666666666666630, 0.2680555555555555469, 0.2694444444444444309, 0.2708333333333333148, 0.2722222222222221988, 0.2736111111111111382, 0.2750000000000000222, 0.2763888888888889062, 0.2777777777777777901, 0.2791666666666666741, 0.2805555555555555580, 0.2819444444444444420, 0.2833333333333333259, 0.2847222222222222099, 0.2861111111111110938, 0.2874999999999999778, 0.2888888888888888618, 0.2902777777777778012, 0.2916666666666666852, 0.2930555555555555691, 0.2944444444444444531, 0.2958333333333333370, 0.2972222222222222210, 0.2986111111111111049, 0.2999999999999999889, 0.3013888888888888729, 0.3027777777777777568, 0.3041666666666666408, 0.3055555555555555802, 0.3069444444444444642, 0.3083333333333333481, 0.3097222222222222321, 0.3111111111111111160, 0.3125000000000000000, 0.3138888888888888840, 0.3152777777777777679, 0.3166666666666666519, 0.3180555555555555358, 0.3194444444444444198, 0.3208333333333333592, 0.3222222222222222432, 0.3236111111111111271, 0.3250000000000000111, 0.3263888888888888951, 0.3277777777777777790, 0.3291666666666666630, 0.3305555555555555469, 0.3319444444444444309, 0.3333333333333333148, 0.3347222222222221988, 0.3361111111111111382, 0.3375000000000000222, 0.3388888888888889062, 0.3402777777777777901, 0.3416666666666666741, 0.3430555555555555580, 0.3444444444444444420, 0.3458333333333333259, 0.3472222222222222099, 0.3486111111111110938, 0.3499999999999999778, 0.3513888888888888618, 0.3527777777777778012, 0.3541666666666666852, 0.3555555555555555691, 0.3569444444444444531, 0.3583333333333333370, 0.3597222222222222210, 0.3611111111111111049, 0.3624999999999999889, 0.3638888888888888729, 0.3652777777777777568, 0.3666666666666666408, 0.3680555555555555802, 0.3694444444444444642, 0.3708333333333333481, 0.3722222222222222321, 0.3736111111111111160, 0.3750000000000000000, 0.3763888888888888840, 0.3777777777777777679, 0.3791666666666666519, 0.3805555555555555358, 0.3819444444444444198, 0.3833333333333333592, 0.3847222222222222432, 0.3861111111111111271, 0.3875000000000000111, 0.3888888888888888951, 0.3902777777777777790, 0.3916666666666666630, 0.3930555555555555469, 0.3944444444444444309, 0.3958333333333333148, 0.3972222222222221988, 0.3986111111111111382, 0.4000000000000000222, 0.4013888888888889062, 0.4027777777777777901, 0.4041666666666666741, 0.4055555555555555580, 0.4069444444444444420, 0.4083333333333333259, 0.4097222222222222099, 0.4111111111111110938, 0.4124999999999999778, 0.4138888888888888618, 0.4152777777777778012, 0.4166666666666666852, 0.4180555555555555691, 0.4194444444444444531, 0.4208333333333333370, 0.4222222222222222210, 0.4236111111111111049, 0.4249999999999999889, 0.4263888888888888729, 0.4277777777777777568, 0.4291666666666666408, 0.4305555555555555802, 0.4319444444444444642, 0.4333333333333333481, 0.4347222222222222321, 0.4361111111111111160, 0.4375000000000000000, 0.4388888888888888840, 0.4402777777777777679, 0.4416666666666666519, 0.4430555555555555358, 0.4444444444444444198, 0.4458333333333333592, 0.4472222222222222432, 0.4486111111111111271, 0.4500000000000000111, 0.4513888888888888951, 0.4527777777777777790, 0.4541666666666666630, 0.4555555555555555469, 0.4569444444444444309, 0.4583333333333333148, 0.4597222222222221988, 0.4611111111111111382, 0.4625000000000000222, 0.4638888888888889062, 0.4652777777777777901, 0.4666666666666666741, 0.4680555555555555580, 0.4694444444444444420, 0.4708333333333333259, 0.4722222222222222099, 0.4736111111111110938, 0.4749999999999999778, 0.4763888888888888618, 0.4777777777777778012, 0.4791666666666666852, 0.4805555555555555691, 0.4819444444444444531, 0.4833333333333333370, 0.4847222222222222210, 0.4861111111111111049, 0.4874999999999999889, 0.4888888888888888729, 0.4902777777777777568, 0.4916666666666666408, 0.4930555555555555802, 0.4944444444444444642, 0.4958333333333333481, 0.4972222222222222321, 0.4986111111111111160, 0.5000000000000000000, 0.5013888888888888840, 0.5027777777777777679, 0.5041666666666666519, 0.5055555555555555358, 0.5069444444444444198, 0.5083333333333333037, 0.5097222222222221877, 0.5111111111111110716, 0.5124999999999999556, 0.5138888888888888395, 0.5152777777777777235, 0.5166666666666667185, 0.5180555555555556024, 0.5194444444444444864, 0.5208333333333333703, 0.5222222222222222543, 0.5236111111111111382, 0.5250000000000000222, 0.5263888888888889062, 0.5277777777777777901, 0.5291666666666666741, 0.5305555555555555580, 0.5319444444444444420, 0.5333333333333333259, 0.5347222222222222099, 0.5361111111111110938, 0.5374999999999999778, 0.5388888888888888618, 0.5402777777777777457, 0.5416666666666666297, 0.5430555555555555136, 0.5444444444444443976, 0.5458333333333332815, 0.5472222222222222765, 0.5486111111111111605, 0.5500000000000000444, 0.5513888888888889284, 0.5527777777777778123, 0.5541666666666666963, 0.5555555555555555802, 0.5569444444444444642, 0.5583333333333333481, 0.5597222222222222321, 0.5611111111111111160, 0.5625000000000000000, 0.5638888888888888840, 0.5652777777777777679, 0.5666666666666666519, 0.5680555555555555358, 0.5694444444444444198, 0.5708333333333333037, 0.5722222222222221877, 0.5736111111111110716, 0.5749999999999999556, 0.5763888888888888395, 0.5777777777777777235, 0.5791666666666667185, 0.5805555555555556024, 0.5819444444444444864, 0.5833333333333333703, 0.5847222222222222543, 0.5861111111111111382, 0.5875000000000000222, 0.5888888888888889062, 0.5902777777777777901, 0.5916666666666666741, 0.5930555555555555580, 0.5944444444444444420, 0.5958333333333333259, 0.5972222222222222099, 0.5986111111111110938, 0.5999999999999999778, 0.6013888888888888618, 0.6027777777777777457, 0.6041666666666666297, 0.6055555555555555136, 0.6069444444444443976, 0.6083333333333332815, 0.6097222222222222765, 0.6111111111111111605, 0.6125000000000000444, 0.6138888888888889284, 0.6152777777777778123, 0.6166666666666666963, 0.6180555555555555802, 0.6194444444444444642, 0.6208333333333333481, 0.6222222222222222321, 0.6236111111111111160, 0.6250000000000000000, 0.6263888888888888840, 0.6277777777777777679, 0.6291666666666666519, 0.6305555555555555358, 0.6319444444444444198, 0.6333333333333333037, 0.6347222222222221877, 0.6361111111111110716, 0.6374999999999999556, 0.6388888888888888395, 0.6402777777777777235, 0.6416666666666667185, 0.6430555555555556024, 0.6444444444444444864, 0.6458333333333333703, 0.6472222222222222543, 0.6486111111111111382, 0.6500000000000000222, 0.6513888888888889062, 0.6527777777777777901, 0.6541666666666666741, 0.6555555555555555580, 0.6569444444444444420, 0.6583333333333333259, 0.6597222222222222099, 0.6611111111111110938, 0.6624999999999999778, 0.6638888888888888618, 0.6652777777777777457, 0.6666666666666666297, 0.6680555555555555136, 0.6694444444444443976, 0.6708333333333332815, 0.6722222222222222765, 0.6736111111111111605, 0.6750000000000000444, 0.6763888888888889284, 0.6777777777777778123, 0.6791666666666666963, 0.6805555555555555802, 0.6819444444444444642, 0.6833333333333333481, 0.6847222222222222321, 0.6861111111111111160, 0.6875000000000000000, 0.6888888888888888840, 0.6902777777777777679, 0.6916666666666666519, 0.6930555555555555358, 0.6944444444444444198, 0.6958333333333333037, 0.6972222222222221877, 0.6986111111111110716, 0.6999999999999999556, 0.7013888888888888395, 0.7027777777777777235, 0.7041666666666667185, 0.7055555555555556024, 0.7069444444444444864, 0.7083333333333333703, 0.7097222222222222543, 0.7111111111111111382, 0.7125000000000000222, 0.7138888888888889062, 0.7152777777777777901, 0.7166666666666666741, 0.7180555555555555580, 0.7194444444444444420, 0.7208333333333333259, 0.7222222222222222099, 0.7236111111111110938, 0.7249999999999999778, 0.7263888888888888618, 0.7277777777777777457, 0.7291666666666666297, 0.7305555555555555136, 0.7319444444444443976, 0.7333333333333332815, 0.7347222222222222765, 0.7361111111111111605, 0.7375000000000000444, 0.7388888888888889284, 0.7402777777777778123, 0.7416666666666666963, 0.7430555555555555802, 0.7444444444444444642, 0.7458333333333333481, 0.7472222222222222321, 0.7486111111111111160, 0.7500000000000000000, 0.7513888888888888840, 0.7527777777777777679, 0.7541666666666666519, 0.7555555555555555358, 0.7569444444444444198, 0.7583333333333333037, 0.7597222222222221877, 0.7611111111111110716, 0.7624999999999999556, 0.7638888888888888395, 0.7652777777777777235, 0.7666666666666667185, 0.7680555555555556024, 0.7694444444444444864, 0.7708333333333333703, 0.7722222222222222543, 0.7736111111111111382, 0.7750000000000000222, 0.7763888888888889062, 0.7777777777777777901, 0.7791666666666666741, 0.7805555555555555580, 0.7819444444444444420, 0.7833333333333333259, 0.7847222222222222099, 0.7861111111111110938, 0.7874999999999999778, 0.7888888888888888618, 0.7902777777777777457, 0.7916666666666666297, 0.7930555555555555136, 0.7944444444444443976, 0.7958333333333332815, 0.7972222222222222765, 0.7986111111111111605, 0.8000000000000000444, 0.8013888888888889284, 0.8027777777777778123, 0.8041666666666666963, 0.8055555555555555802, 0.8069444444444444642, 0.8083333333333333481, 0.8097222222222222321, 0.8111111111111111160, 0.8125000000000000000, 0.8138888888888888840, 0.8152777777777777679, 0.8166666666666666519, 0.8180555555555555358, 0.8194444444444444198, 0.8208333333333333037, 0.8222222222222221877, 0.8236111111111110716, 0.8249999999999999556, 0.8263888888888888395, 0.8277777777777777235, 0.8291666666666667185, 0.8305555555555556024, 0.8319444444444444864, 0.8333333333333333703, 0.8347222222222222543, 0.8361111111111111382, 0.8375000000000000222, 0.8388888888888889062, 0.8402777777777777901, 0.8416666666666666741, 0.8430555555555555580, 0.8444444444444444420, 0.8458333333333333259, 0.8472222222222222099, 0.8486111111111110938, 0.8499999999999999778, 0.8513888888888888618, 0.8527777777777777457, 0.8541666666666666297, 0.8555555555555555136, 0.8569444444444443976, 0.8583333333333332815, 0.8597222222222222765, 0.8611111111111111605, 0.8625000000000000444, 0.8638888888888889284, 0.8652777777777778123, 0.8666666666666666963, 0.8680555555555555802, 0.8694444444444444642, 0.8708333333333333481, 0.8722222222222222321, 0.8736111111111111160, 0.8750000000000000000, 0.8763888888888888840, 0.8777777777777777679, 0.8791666666666666519, 0.8805555555555555358, 0.8819444444444444198, 0.8833333333333333037, 0.8847222222222221877, 0.8861111111111110716, 0.8874999999999999556, 0.8888888888888888395, 0.8902777777777777235, 0.8916666666666667185, 0.8930555555555556024, 0.8944444444444444864, 0.8958333333333333703, 0.8972222222222222543, 0.8986111111111111382, 0.9000000000000000222, 0.9013888888888889062, 0.9027777777777777901, 0.9041666666666666741, 0.9055555555555555580, 0.9069444444444444420, 0.9083333333333333259, 0.9097222222222222099, 0.9111111111111110938, 0.9124999999999999778, 0.9138888888888888618, 0.9152777777777777457, 0.9166666666666666297, 0.9180555555555555136, 0.9194444444444443976, 0.9208333333333332815, 0.9222222222222222765, 0.9236111111111111605, 0.9250000000000000444, 0.9263888888888889284, 0.9277777777777778123, 0.9291666666666666963, 0.9305555555555555802, 0.9319444444444444642, 0.9333333333333333481, 0.9347222222222222321, 0.9361111111111111160, 0.9375000000000000000, 0.9388888888888888840, 0.9402777777777777679, 0.9416666666666666519, 0.9430555555555555358, 0.9444444444444444198, 0.9458333333333333037, 0.9472222222222221877, 0.9486111111111110716, 0.9499999999999999556, 0.9513888888888888395, 0.9527777777777777235, 0.9541666666666667185, 0.9555555555555556024, 0.9569444444444444864, 0.9583333333333333703, 0.9597222222222222543, 0.9611111111111111382, 0.9625000000000000222, 0.9638888888888889062, 0.9652777777777777901, 0.9666666666666666741, 0.9680555555555555580, 0.9694444444444444420, 0.9708333333333333259, 0.9722222222222222099, 0.9736111111111110938, 0.9749999999999999778, 0.9763888888888888618, 0.9777777777777777457, 0.9791666666666666297, 0.9805555555555555136, 0.9819444444444443976, 0.9833333333333332815, 0.9847222222222222765, 0.9861111111111111605, 0.9875000000000000444, 0.9888888888888889284, 0.9902777777777778123, 0.9916666666666666963, 0.9930555555555555802, 0.9944444444444444642, 0.9958333333333333481, 0.9972222222222222321, 0.9986111111111111160, 1.000000000000000000 ),
 .UNSPECIFIED. ) 
 GEOMETRIC_REPRESENTATION_ITEM ( )  RATIONAL_B_SPLINE_SURFACE ( (
 ( 1.000000000000000000, 0.8660254037844387076, 1.000000000000000000, 0.8660254037844387076, 1.000000000000000000, 0.8660254037844387076, 1.000000000000000000, 0.8660254037844387076, 1.000000000000000000, 0.8660254037844387076, 1.000000000000000000, 0.8660254037844387076, 1.000000000000000000, 0.8660254037844387076, 1.000000000000000000, 0.8660254037844387076, 1.000000000000000000, 0.8660254037844387076, 1.000000000000000000, 0.8660254037844387076, 1.000000000000000000, 0.8660254037844387076, 1.000000000000000000, 0.8660254037844387076, 1.000000000000000000, 0.8660254037844387076, 1.000000000000000000, 0.8660254037844387076, 1.000000000000000000, 0.8660254037844387076, 1.000000000000000000, 0.8660254037844387076, 1.000000000000000000, 0.8660254037844387076, 1.000000000000000000, 0.8660254037844387076, 1.000000000000000000, 0.8660254037844387076, 1.000000000000000000, 0.8660254037844387076, 1.000000000000000000, 0.8660254037844387076, 1.000000000000000000, 0.8660254037844387076, 1.000000000000000000, 0.8660254037844387076, 1.000000000000000000, 0.8660254037844387076, 1.000000000000000000, 0.8660254037844387076, 1.000000000000000000, 0.8660254037844387076, 1.000000000000000000, 0.8660254037844387076, 1.000000000000000000, 0.8660254037844387076, 1.000000000000000000, 0.8660254037844387076, 1.000000000000000000, 0.8660254037844387076, 1.000000000000000000, 0.8660254037844387076, 1.000000000000000000, 0.8660254037844387076, 1.000000000000000000, 0.8660254037844387076, 1.000000000000000000, 0.8660254037844387076, 1.000000000000000000, 0.8660254037844387076, 1.000000000000000000, 0.8660254037844387076, 1.000000000000000000, 0.8660254037844387076, 1.000000000000000000, 0.8660254037844387076, 1.000000000000000000, 0.8660254037844387076, 1.000000000000000000, 0.8660254037844387076, 1.000000000000000000, 0.8660254037844387076, 1.000000000000000000, 0.8660254037844387076, 1.000000000000000000, 0.8660254037844387076, 1.000000000000000000, 0.8660254037844387076, 1.000000000000000000, 0.8660254037844387076, 1.000000000000000000, 0.8660254037844387076, 1.000000000000000000, 0.8660254037844387076, 1.000000000000000000, 0.8660254037844387076, 1.000000000000000000, 0.8660254037844387076, 1.000000000000000000, 0.8660254037844387076, 1.000000000000000000, 0.8660254037844387076, 1.000000000000000000, 0.8660254037844387076, 1.000000000000000000, 0.8660254037844387076, 1.000000000000000000, 0.8660254037844387076, 1.000000000000000000, 0.8660254037844387076, 1.000000000000000000, 0.8660254037844387076, 1.000000000000000000, 0.8660254037844387076, 1.000000000000000000, 0.8660254037844387076, 1.000000000000000000, 0.8660254037844387076, 1.000000000000000000, 0.8660254037844387076, 1.000000000000000000, 0.8660254037844387076, 1.000000000000000000, 0.8660254037844387076, 1.000000000000000000, 0.8660254037844387076, 1.000000000000000000, 0.8660254037844387076, 1.000000000000000000, 0.8660254037844387076, 1.000000000000000000, 0.8660254037844387076, 1.000000000000000000, 0.8660254037844387076, 1.000000000000000000, 0.8660254037844387076, 1.000000000000000000, 0.8660254037844387076, 1.000000000000000000, 0.8660254037844387076, 1.000000000000000000, 0.8660254037844387076, 1.000000000000000000, 0.8660254037844387076, 1.000000000000000000, 0.8660254037844387076, 1.000000000000000000, 0.8660254037844387076, 1.000000000000000000, 0.8660254037844387076, 1.000000000000000000, 0.8660254037844387076, 1.000000000000000000, 0.8660254037844387076, 1.000000000000000000, 0.8660254037844387076, 1.000000000000000000, 0.8660254037844387076, 1.000000000000000000, 0.8660254037844387076, 1.000000000000000000, 0.8660254037844387076, 1.000000000000000000, 0.8660254037844387076, 1.000000000000000000, 0.8660254037844387076, 1.000000000000000000, 0.8660254037844387076, 1.000000000000000000, 0.8660254037844387076, 1.000000000000000000, 0.8660254037844387076, 1.000000000000000000, 0.8660254037844387076, 1.000000000000000000, 0.8660254037844387076, 1.000000000000000000, 0.8660254037844387076, 1.000000000000000000, 0.8660254037844387076, 1.000000000000000000, 0.8660254037844387076, 1.000000000000000000, 0.8660254037844387076, 1.000000000000000000, 0.8660254037844387076, 1.000000000000000000, 0.8660254037844387076, 1.000000000000000000, 0.8660254037844387076, 1.000000000000000000, 0.8660254037844387076, 1.000000000000000000, 0.8660254037844387076, 1.000000000000000000, 0.8660254037844387076, 1.000000000000000000, 0.8660254037844387076, 1.000000000000000000, 0.8660254037844387076, 1.000000000000000000, 0.8660254037844387076, 1.000000000000000000, 0.8660254037844387076, 1.000000000000000000, 0.8660254037844387076, 1.000000000000000000, 0.8660254037844387076, 1.000000000000000000, 0.8660254037844387076, 1.000000000000000000, 0.8660254037844387076, 1.000000000000000000, 0.8660254037844387076, 1.000000000000000000, 0.8660254037844387076, 1.000000000000000000, 0.8660254037844387076, 1.000000000000000000, 0.8660254037844387076, 1.000000000000000000, 0.8660254037844387076, 1.000000000000000000, 0.8660254037844387076, 1.000000000000000000, 0.8660254037844387076, 1.000000000000000000, 0.8660254037844387076, 1.000000000000000000, 0.8660254037844387076, 1.000000000000000000, 0.8660254037844387076, 1.000000000000000000, 0.8660254037844387076, 1.000000000000000000, 0.8660254037844387076, 1.000000000000000000, 0.8660254037844387076, 1.000000000000000000, 0.8660254037844387076, 1.000000000000000000, 0.8660254037844387076, 1.000000000000000000, 0.8660254037844387076, 1.000000000000000000, 0.8660254037844387076, 1.000000000000000000, 0.8660254037844387076, 1.000000000000000000, 0.8660254037844387076, 1.000000000000000000, 0.8660254037844387076, 1.000000000000000000, 0.8660254037844387076, 1.000000000000000000, 0.8660254037844387076, 1.000000000000000000, 0.8660254037844387076, 1.000000000000000000, 0.8660254037844387076, 1.000000000000000000, 0.8660254037844387076, 1.000000000000000000, 0.8660254037844387076, 1.000000000000000000, 0.8660254037844387076, 1.000000000000000000, 0.8660254037844387076, 1.000000000000000000, 0.8660254037844387076, 1.000000000000000000, 0.8660254037844387076, 1.000000000000000000, 0.8660254037844387076, 1.000000000000000000, 0.8660254037844387076, 1.000000000000000000, 0.8660254037844387076, 1.000000000000000000, 0.8660254037844387076, 1.000000000000000000, 0.8660254037844387076, 1.000000000000000000, 0.8660254037844387076, 1.000000000000000000, 0.8660254037844387076, 1.000000000000000000, 0.8660254037844387076, 1.000000000000000000, 0.8660254037844387076, 1.000000000000000000, 0.8660254037844387076, 1.000000000000000000, 0.8660254037844387076, 1.000000000000000000, 0.8660254037844387076, 1.000000000000000000, 0.8660254037844387076, 1.000000000000000000, 0.8660254037844387076, 1.000000000000000000, 0.8660254037844387076, 1.000000000000000000, 0.8660254037844387076, 1.000000000000000000, 0.8660254037844387076, 1.000000000000000000, 0.8660254037844387076, 1.000000000000000000, 0.8660254037844387076, 1.000000000000000000, 0.8660254037844387076, 1.000000000000000000, 0.8660254037844387076, 1.000000000000000000, 0.8660254037844387076, 1.000000000000000000, 0.8660254037844387076, 1.000000000000000000, 0.8660254037844387076, 1.000000000000000000, 0.8660254037844387076, 1.000000000000000000, 0.8660254037844387076, 1.000000000000000000, 0.8660254037844387076, 1.000000000000000000, 0.8660254037844387076, 1.000000000000000000, 0.8660254037844387076, 1.000000000000000000, 0.8660254037844387076, 1.000000000000000000, 0.8660254037844387076, 1.000000000000000000, 0.8660254037844387076, 1.000000000000000000, 0.8660254037844387076, 1.000000000000000000, 0.8660254037844387076, 1.000000000000000000, 0.8660254037844387076, 1.000000000000000000, 0.8660254037844387076, 1.000000000000000000, 0.8660254037844387076, 1.000000000000000000, 0.8660254037844387076, 1.000000000000000000, 0.8660254037844387076, 1.000000000000000000, 0.8660254037844387076, 1.000000000000000000, 0.8660254037844387076, 1.000000000000000000, 0.8660254037844387076, 1.000000000000000000, 0.8660254037844387076, 1.000000000000000000, 0.8660254037844387076, 1.000000000000000000, 0.8660254037844387076, 1.000000000000000000, 0.8660254037844387076, 1.000000000000000000, 0.8660254037844387076, 1.000000000000000000, 0.8660254037844387076, 1.000000000000000000, 0.8660254037844387076, 1.000000000000000000, 0.8660254037844387076, 1.000000000000000000, 0.8660254037844387076, 1.000000000000000000, 0.8660254037844387076, 1.000000000000000000, 0.8660254037844387076, 1.000000000000000000, 0.8660254037844387076, 1.000000000000000000, 0.8660254037844387076, 1.000000000000000000, 0.8660254037844387076, 1.000000000000000000, 0.8660254037844387076, 1.000000000000000000, 0.8660254037844387076, 1.000000000000000000, 0.8660254037844387076, 1.000000000000000000, 0.8660254037844387076, 1.000000000000000000, 0.8660254037844387076, 1.000000000000000000, 0.8660254037844387076, 1.000000000000000000, 0.8660254037844387076, 1.000000000000000000, 0.8660254037844387076, 1.000000000000000000, 0.8660254037844387076, 1.000000000000000000, 0.8660254037844387076, 1.000000000000000000, 0.8660254037844387076, 1.000000000000000000, 0.8660254037844387076, 1.000000000000000000, 0.8660254037844387076, 1.000000000000000000, 0.8660254037844387076, 1.000000000000000000, 0.8660254037844387076, 1.000000000000000000, 0.8660254037844387076, 1.000000000000000000, 0.8660254037844387076, 1.000000000000000000, 0.8660254037844387076, 1.000000000000000000, 0.8660254037844387076, 1.000000000000000000, 0.8660254037844387076, 1.000000000000000000, 0.8660254037844387076, 1.000000000000000000, 0.8660254037844387076, 1.000000000000000000, 0.8660254037844387076, 1.000000000000000000, 0.8660254037844387076, 1.000000000000000000, 0.8660254037844387076, 1.000000000000000000, 0.8660254037844387076, 1.000000000000000000, 0.8660254037844387076, 1.000000000000000000, 0.8660254037844387076, 1.000000000000000000, 0.8660254037844387076, 1.000000000000000000, 0.8660254037844387076, 1.000000000000000000, 0.8660254037844387076, 1.000000000000000000, 0.8660254037844387076, 1.000000000000000000, 0.8660254037844387076, 1.000000000000000000, 0.8660254037844387076, 1.000000000000000000, 0.8660254037844387076, 1.000000000000000000, 0.8660254037844387076, 1.000000000000000000, 0.8660254037844387076, 1.000000000000000000, 0.8660254037844387076, 1.000000000000000000, 0.8660254037844387076, 1.000000000000000000, 0.8660254037844387076, 1.000000000000000000, 0.8660254037844387076, 1.000000000000000000, 0.8660254037844387076, 1.000000000000000000, 0.8660254037844387076, 1.000000000000000000, 0.8660254037844387076, 1.000000000000000000, 0.8660254037844387076, 1.000000000000000000, 0.8660254037844387076, 1.000000000000000000, 0.8660254037844387076, 1.000000000000000000, 0.8660254037844387076, 1.000000000000000000, 0.8660254037844387076, 1.000000000000000000, 0.8660254037844387076, 1.000000000000000000, 0.8660254037844387076, 1.000000000000000000, 0.8660254037844387076, 1.000000000000000000, 0.8660254037844387076, 1.000000000000000000, 0.8660254037844387076, 1.000000000000000000, 0.8660254037844387076, 1.000000000000000000, 0.8660254037844387076, 1.000000000000000000, 0.8660254037844387076, 1.000000000000000000, 0.8660254037844387076, 1.000000000000000000, 0.8660254037844387076, 1.000000000000000000, 0.8660254037844387076, 1.000000000000000000, 0.8660254037844387076, 1.000000000000000000, 0.8660254037844387076, 1.000000000000000000, 0.8660254037844387076, 1.000000000000000000, 0.8660254037844387076, 1.000000000000000000, 0.8660254037844387076, 1.000000000000000000, 0.8660254037844387076, 1.000000000000000000, 0.8660254037844387076, 1.000000000000000000, 0.8660254037844387076, 1.000000000000000000, 0.8660254037844387076, 1.000000000000000000, 0.8660254037844387076, 1.000000000000000000, 0.8660254037844387076, 1.000000000000000000, 0.8660254037844387076, 1.000000000000000000, 0.8660254037844387076, 1.000000000000000000, 0.8660254037844387076, 1.000000000000000000, 0.8660254037844387076, 1.000000000000000000, 0.8660254037844387076, 1.000000000000000000, 0.8660254037844387076, 1.000000000000000000, 0.8660254037844387076, 1.000000000000000000, 0.8660254037844387076, 1.000000000000000000, 0.8660254037844387076, 1.000000000000000000, 0.8660254037844387076, 1.000000000000000000, 0.8660254037844387076, 1.000000000000000000, 0.8660254037844387076, 1.000000000000000000, 0.8660254037844387076, 1.000000000000000000, 0.8660254037844387076, 1.000000000000000000, 0.8660254037844387076, 1.000000000000000000, 0.8660254037844387076, 1.000000000000000000, 0.8660254037844387076, 1.000000000000000000, 0.8660254037844387076, 1.000000000000000000, 0.8660254037844387076, 1.000000000000000000, 0.8660254037844387076, 1.000000000000000000, 0.8660254037844387076, 1.000000000000000000, 0.8660254037844387076, 1.000000000000000000, 0.8660254037844387076, 1.000000000000000000, 0.8660254037844387076, 1.000000000000000000, 0.8660254037844387076, 1.000000000000000000, 0.8660254037844387076, 1.000000000000000000, 0.8660254037844387076, 1.000000000000000000, 0.8660254037844387076, 1.000000000000000000, 0.8660254037844387076, 1.000000000000000000, 0.8660254037844387076, 1.000000000000000000, 0.8660254037844387076, 1.000000000000000000, 0.8660254037844387076, 1.000000000000000000, 0.8660254037844387076, 1.000000000000000000, 0.8660254037844387076, 1.000000000000000000, 0.8660254037844387076, 1.000000000000000000, 0.8660254037844387076, 1.000000000000000000, 0.8660254037844387076, 1.000000000000000000, 0.8660254037844387076, 1.000000000000000000, 0.8660254037844387076, 1.000000000000000000, 0.8660254037844387076, 1.000000000000000000, 0.8660254037844387076, 1.000000000000000000, 0.8660254037844387076, 1.000000000000000000, 0.8660254037844387076, 1.000000000000000000, 0.8660254037844387076, 1.000000000000000000, 0.8660254037844387076, 1.000000000000000000, 0.8660254037844387076, 1.000000000000000000, 0.8660254037844387076, 1.000000000000000000, 0.8660254037844387076, 1.000000000000000000, 0.8660254037844387076, 1.000000000000000000, 0.8660254037844387076, 1.000000000000000000, 0.8660254037844387076, 1.000000000000000000, 0.8660254037844387076, 1.000000000000000000, 0.8660254037844387076, 1.000000000000000000, 0.8660254037844387076, 1.000000000000000000, 0.8660254037844387076, 1.000000000000000000, 0.8660254037844387076, 1.000000000000000000, 0.8660254037844387076, 1.000000000000000000, 0.8660254037844387076, 1.000000000000000000, 0.8660254037844387076, 1.000000000000000000, 0.8660254037844387076, 1.000000000000000000, 0.8660254037844387076, 1.000000000000000000, 0.8660254037844387076, 1.000000000000000000, 0.8660254037844387076, 1.000000000000000000, 0.8660254037844387076, 1.000000000000000000, 0.8660254037844387076, 1.000000000000000000, 0.8660254037844387076, 1.000000000000000000, 0.8660254037844387076, 1.000000000000000000, 0.8660254037844387076, 1.000000000000000000, 0.8660254037844387076, 1.000000000000000000, 0.8660254037844387076, 1.000000000000000000, 0.8660254037844387076, 1.000000000000000000, 0.8660254037844387076, 1.000000000000000000, 0.8660254037844387076, 1.000000000000000000, 0.8660254037844387076, 1.000000000000000000, 0.8660254037844387076, 1.000000000000000000, 0.8660254037844387076, 1.000000000000000000, 0.8660254037844387076, 1.000000000000000000, 0.8660254037844387076, 1.000000000000000000, 0.8660254037844387076, 1.000000000000000000, 0.8660254037844387076, 1.000000000000000000, 0.8660254037844387076, 1.000000000000000000, 0.8660254037844387076, 1.000000000000000000, 0.8660254037844387076, 1.000000000000000000, 0.8660254037844387076, 1.000000000000000000, 0.8660254037844387076, 1.000000000000000000, 0.8660254037844387076, 1.000000000000000000, 0.8660254037844387076, 1.000000000000000000, 0.8660254037844387076, 1.000000000000000000, 0.8660254037844387076, 1.000000000000000000, 0.8660254037844387076, 1.000000000000000000, 0.8660254037844387076, 1.000000000000000000, 0.8660254037844387076, 1.000000000000000000, 0.8660254037844387076, 1.000000000000000000, 0.8660254037844387076, 1.000000000000000000, 0.8660254037844387076, 1.000000000000000000, 0.8660254037844387076, 1.000000000000000000, 0.8660254037844387076, 1.000000000000000000, 0.8660254037844387076, 1.000000000000000000, 0.8660254037844387076, 1.000000000000000000, 0.8660254037844387076, 1.000000000000000000, 0.8660254037844387076, 1.000000000000000000, 0.8660254037844387076, 1.000000000000000000, 0.8660254037844387076, 1.000000000000000000, 0.8660254037844387076, 1.000000000000000000, 0.8660254037844387076, 1.000000000000000000, 0.8660254037844387076, 1.000000000000000000, 0.8660254037844387076, 1.000000000000000000, 0.8660254037844387076, 1.000000000000000000, 0.8660254037844387076, 1.000000000000000000, 0.8660254037844387076, 1.000000000000000000, 0.8660254037844387076, 1.000000000000000000, 0.8660254037844387076, 1.000000000000000000, 0.8660254037844387076, 1.000000000000000000, 0.8660254037844387076, 1.000000000000000000, 0.8660254037844387076, 1.000000000000000000, 0.8660254037844387076, 1.000000000000000000, 0.8660254037844387076, 1.000000000000000000, 0.8660254037844387076, 1.000000000000000000, 0.8660254037844387076, 1.000000000000000000, 0.8660254037844387076, 1.000000000000000000, 0.8660254037844387076, 1.000000000000000000, 0.8660254037844387076, 1.000000000000000000, 0.8660254037844387076, 1.000000000000000000, 0.8660254037844387076, 1.000000000000000000, 0.8660254037844387076, 1.000000000000000000, 0.8660254037844387076, 1.000000000000000000, 0.8660254037844387076, 1.000000000000000000, 0.8660254037844387076, 1.000000000000000000, 0.8660254037844387076, 1.000000000000000000, 0.8660254037844387076, 1.000000000000000000, 0.8660254037844387076, 1.000000000000000000, 0.8660254037844387076, 1.000000000000000000, 0.8660254037844387076, 1.000000000000000000, 0.8660254037844387076, 1.000000000000000000, 0.8660254037844387076, 1.000000000000000000, 0.8660254037844387076, 1.000000000000000000, 0.8660254037844387076, 1.000000000000000000, 0.8660254037844387076, 1.000000000000000000, 0.8660254037844387076, 1.000000000000000000, 0.8660254037844387076, 1.000000000000000000, 0.8660254037844387076, 1.000000000000000000, 0.8660254037844387076, 1.000000000000000000, 0.8660254037844387076, 1.000000000000000000, 0.8660254037844387076, 1.000000000000000000, 0.8660254037844387076, 1.000000000000000000, 0.8660254037844387076, 1.000000000000000000, 0.8660254037844387076, 1.000000000000000000, 0.8660254037844387076, 1.000000000000000000, 0.8660254037844387076, 1.000000000000000000, 0.8660254037844387076, 1.000000000000000000, 0.8660254037844387076, 1.000000000000000000, 0.8660254037844387076, 1.000000000000000000, 0.8660254037844387076, 1.000000000000000000, 0.8660254037844387076, 1.000000000000000000, 0.8660254037844387076, 1.000000000000000000, 0.8660254037844387076, 1.000000000000000000, 0.8660254037844387076, 1.000000000000000000, 0.8660254037844387076, 1.000000000000000000, 0.8660254037844387076, 1.000000000000000000, 0.8660254037844387076, 1.000000000000000000, 0.8660254037844387076, 1.000000000000000000, 0.8660254037844387076, 1.000000000000000000, 0.8660254037844387076, 1.000000000000000000, 0.8660254037844387076, 1.000000000000000000, 0.8660254037844387076, 1.000000000000000000, 0.8660254037844387076, 1.000000000000000000, 0.8660254037844387076, 1.000000000000000000, 0.8660254037844387076, 1.000000000000000000, 0.8660254037844387076, 1.000000000000000000, 0.8660254037844387076, 1.000000000000000000, 0.8660254037844387076, 1.000000000000000000, 0.8660254037844387076, 1.000000000000000000, 0.8660254037844387076, 1.000000000000000000, 0.8660254037844387076, 1.000000000000000000, 0.8660254037844387076, 1.000000000000000000, 0.8660254037844387076, 1.000000000000000000, 0.8660254037844387076, 1.000000000000000000, 0.8660254037844387076, 1.000000000000000000, 0.8660254037844387076, 1.000000000000000000, 0.8660254037844387076, 1.000000000000000000, 0.8660254037844387076, 1.000000000000000000, 0.8660254037844387076, 1.000000000000000000, 0.8660254037844387076, 1.000000000000000000, 0.8660254037844387076, 1.000000000000000000, 0.8660254037844387076, 1.000000000000000000, 0.8660254037844387076, 1.000000000000000000, 0.8660254037844387076, 1.000000000000000000, 0.8660254037844387076, 1.000000000000000000, 0.8660254037844387076, 1.000000000000000000, 0.8660254037844387076, 1.000000000000000000, 0.8660254037844387076, 1.000000000000000000, 0.8660254037844387076, 1.000000000000000000, 0.8660254037844387076, 1.000000000000000000, 0.8660254037844387076, 1.000000000000000000, 0.8660254037844387076, 1.000000000000000000, 0.8660254037844387076, 1.000000000000000000, 0.8660254037844387076, 1.000000000000000000, 0.8660254037844387076, 1.000000000000000000, 0.8660254037844387076, 1.000000000000000000, 0.8660254037844387076, 1.000000000000000000, 0.8660254037844387076, 1.000000000000000000, 0.8660254037844387076, 1.000000000000000000, 0.8660254037844387076, 1.000000000000000000, 0.8660254037844387076, 1.000000000000000000, 0.8660254037844387076, 1.000000000000000000, 0.8660254037844387076, 1.000000000000000000, 0.8660254037844387076, 1.000000000000000000, 0.8660254037844387076, 1.000000000000000000, 0.8660254037844387076, 1.000000000000000000, 0.8660254037844387076, 1.000000000000000000, 0.8660254037844387076, 1.000000000000000000, 0.8660254037844387076, 1.000000000000000000, 0.8660254037844387076, 1.000000000000000000, 0.8660254037844387076, 1.000000000000000000, 0.8660254037844387076, 1.000000000000000000, 0.8660254037844387076, 1.000000000000000000, 0.8660254037844387076, 1.000000000000000000, 0.8660254037844387076, 1.000000000000000000, 0.8660254037844387076, 1.000000000000000000, 0.8660254037844387076, 1.000000000000000000, 0.8660254037844387076, 1.000000000000000000, 0.8660254037844387076, 1.000000000000000000, 0.8660254037844387076, 1.000000000000000000, 0.8660254037844387076, 1.000000000000000000, 0.8660254037844387076, 1.000000000000000000, 0.8660254037844387076, 1.000000000000000000, 0.8660254037844387076, 1.000000000000000000, 0.8660254037844387076, 1.000000000000000000, 0.8660254037844387076, 1.000000000000000000, 0.8660254037844387076, 1.000000000000000000, 0.8660254037844387076, 1.000000000000000000, 0.8660254037844387076, 1.000000000000000000, 0.8660254037844387076, 1.000000000000000000, 0.8660254037844387076, 1.000000000000000000, 0.8660254037844387076, 1.000000000000000000, 0.8660254037844387076, 1.000000000000000000, 0.8660254037844387076, 1.000000000000000000, 0.8660254037844387076, 1.000000000000000000, 0.8660254037844387076, 1.000000000000000000, 0.8660254037844387076, 1.000000000000000000, 0.8660254037844387076, 1.000000000000000000, 0.8660254037844387076, 1.000000000000000000, 0.8660254037844387076, 1.000000000000000000, 0.8660254037844387076, 1.000000000000000000, 0.8660254037844387076, 1.000000000000000000, 0.8660254037844387076, 1.000000000000000000, 0.8660254037844387076, 1.000000000000000000, 0.8660254037844387076, 1.000000000000000000, 0.8660254037844387076, 1.000000000000000000, 0.8660254037844387076, 1.000000000000000000, 0.8660254037844387076, 1.000000000000000000, 0.8660254037844387076, 1.000000000000000000, 0.8660254037844387076, 1.000000000000000000, 0.8660254037844387076, 1.000000000000000000, 0.8660254037844387076, 1.000000000000000000, 0.8660254037844387076, 1.000000000000000000, 0.8660254037844387076, 1.000000000000000000, 0.8660254037844387076, 1.000000000000000000, 0.8660254037844387076, 1.000000000000000000, 0.8660254037844387076, 1.000000000000000000, 0.8660254037844387076, 1.000000000000000000, 0.8660254037844387076, 1.000000000000000000, 0.8660254037844387076, 1.000000000000000000, 0.8660254037844387076, 1.000000000000000000, 0.8660254037844387076, 1.000000000000000000, 0.8660254037844387076, 1.000000000000000000, 0.8660254037844387076, 1.000000000000000000, 0.8660254037844387076, 1.000000000000000000, 0.8660254037844387076, 1.000000000000000000, 0.8660254037844387076, 1.000000000000000000, 0.8660254037844387076, 1.000000000000000000, 0.8660254037844387076, 1.000000000000000000, 0.8660254037844387076, 1.000000000000000000, 0.8660254037844387076, 1.000000000000000000, 0.8660254037844387076, 1.000000000000000000, 0.8660254037844387076, 1.000000000000000000, 0.8660254037844387076, 1.000000000000000000, 0.8660254037844387076, 1.000000000000000000, 0.8660254037844387076, 1.000000000000000000, 0.8660254037844387076, 1.000000000000000000, 0.8660254037844387076, 1.000000000000000000, 0.8660254037844387076, 1.000000000000000000, 0.8660254037844387076, 1.000000000000000000, 0.8660254037844387076, 1.000000000000000000, 0.8660254037844387076, 1.000000000000000000, 0.8660254037844387076, 1.000000000000000000, 0.8660254037844387076, 1.000000000000000000, 0.8660254037844387076, 1.000000000000000000, 0.8660254037844387076, 1.000000000000000000, 0.8660254037844387076, 1.000000000000000000, 0.8660254037844387076, 1.000000000000000000, 0.8660254037844387076, 1.000000000000000000, 0.8660254037844387076, 1.000000000000000000, 0.8660254037844387076, 1.000000000000000000, 0.8660254037844387076, 1.000000000000000000, 0.8660254037844387076, 1.000000000000000000, 0.8660254037844387076, 1.000000000000000000, 0.8660254037844387076, 1.000000000000000000, 0.8660254037844387076, 1.000000000000000000, 0.8660254037844387076, 1.000000000000000000, 0.8660254037844387076, 1.000000000000000000, 0.8660254037844387076, 1.000000000000000000, 0.8660254037844387076, 1.000000000000000000, 0.8660254037844387076, 1.000000000000000000, 0.8660254037844387076, 1.000000000000000000, 0.8660254037844387076, 1.000000000000000000, 0.8660254037844387076, 1.000000000000000000, 0.8660254037844387076, 1.000000000000000000, 0.8660254037844387076, 1.000000000000000000, 0.8660254037844387076, 1.000000000000000000, 0.8660254037844387076, 1.000000000000000000, 0.8660254037844387076, 1.000000000000000000, 0.8660254037844387076, 1.000000000000000000, 0.8660254037844387076, 1.000000000000000000, 0.8660254037844387076, 1.000000000000000000, 0.8660254037844387076, 1.000000000000000000, 0.8660254037844387076, 1.000000000000000000, 0.8660254037844387076, 1.000000000000000000, 0.8660254037844387076, 1.000000000000000000, 0.8660254037844387076, 1.000000000000000000, 0.8660254037844387076, 1.000000000000000000, 0.8660254037844387076, 1.000000000000000000, 0.8660254037844387076, 1.000000000000000000, 0.8660254037844387076, 1.000000000000000000, 0.8660254037844387076, 1.000000000000000000, 0.8660254037844387076, 1.000000000000000000, 0.8660254037844387076, 1.000000000000000000, 0.8660254037844387076, 1.000000000000000000, 0.8660254037844387076, 1.000000000000000000, 0.8660254037844387076, 1.000000000000000000, 0.8660254037844387076, 1.000000000000000000, 0.8660254037844387076, 1.000000000000000000, 0.8660254037844387076, 1.000000000000000000, 0.8660254037844387076, 1.000000000000000000, 0.8660254037844387076, 1.000000000000000000, 0.8660254037844387076, 1.000000000000000000, 0.8660254037844387076, 1.000000000000000000, 0.8660254037844387076, 1.000000000000000000, 0.8660254037844387076, 1.000000000000000000, 0.8660254037844387076, 1.000000000000000000, 0.8660254037844387076, 1.000000000000000000, 0.8660254037844387076, 1.000000000000000000, 0.8660254037844387076, 1.000000000000000000, 0.8660254037844387076, 1.000000000000000000, 0.8660254037844387076, 1.000000000000000000, 0.8660254037844387076, 1.000000000000000000, 0.8660254037844387076, 1.000000000000000000, 0.8660254037844387076, 1.000000000000000000, 0.8660254037844387076, 1.000000000000000000, 0.8660254037844387076, 1.000000000000000000, 0.8660254037844387076, 1.000000000000000000, 0.8660254037844387076, 1.000000000000000000, 0.8660254037844387076, 1.000000000000000000, 0.8660254037844387076, 1.000000000000000000, 0.8660254037844387076, 1.000000000000000000, 0.8660254037844387076, 1.000000000000000000, 0.8660254037844387076, 1.000000000000000000, 0.8660254037844387076, 1.000000000000000000, 0.8660254037844387076, 1.000000000000000000, 0.8660254037844387076, 1.000000000000000000, 0.8660254037844387076, 1.000000000000000000, 0.8660254037844387076, 1.000000000000000000, 0.8660254037844387076, 1.000000000000000000, 0.8660254037844387076, 1.000000000000000000, 0.8660254037844387076, 1.000000000000000000, 0.8660254037844387076, 1.000000000000000000, 0.8660254037844387076, 1.000000000000000000, 0.8660254037844387076, 1.000000000000000000, 0.8660254037844387076, 1.000000000000000000, 0.8660254037844387076, 1.000000000000000000, 0.8660254037844387076, 1.000000000000000000, 0.8660254037844387076, 1.000000000000000000, 0.8660254037844387076, 1.000000000000000000, 0.8660254037844387076, 1.000000000000000000, 0.8660254037844387076, 1.000000000000000000, 0.8660254037844387076, 1.000000000000000000, 0.8660254037844387076, 1.000000000000000000, 0.8660254037844387076, 1.000000000000000000, 0.8660254037844387076, 1.000000000000000000, 0.8660254037844387076, 1.000000000000000000, 0.8660254037844387076, 1.000000000000000000, 0.8660254037844387076, 1.000000000000000000, 0.8660254037844387076, 1.000000000000000000, 0.8660254037844387076, 1.000000000000000000, 0.8660254037844387076, 1.000000000000000000, 0.8660254037844387076, 1.000000000000000000, 0.8660254037844387076, 1.000000000000000000, 0.8660254037844387076, 1.000000000000000000, 0.8660254037844387076, 1.000000000000000000, 0.8660254037844387076, 1.000000000000000000, 0.8660254037844387076, 1.000000000000000000, 0.8660254037844387076, 1.000000000000000000, 0.8660254037844387076, 1.000000000000000000, 0.8660254037844387076, 1.000000000000000000, 0.8660254037844387076, 1.000000000000000000, 0.8660254037844387076, 1.000000000000000000, 0.8660254037844387076, 1.000000000000000000, 0.8660254037844387076, 1.000000000000000000, 0.8660254037844387076, 1.000000000000000000, 0.8660254037844387076, 1.000000000000000000, 0.8660254037844387076, 1.000000000000000000, 0.8660254037844387076, 1.000000000000000000, 0.8660254037844387076, 1.000000000000000000, 0.8660254037844387076, 1.000000000000000000, 0.8660254037844387076, 1.000000000000000000, 0.8660254037844387076, 1.000000000000000000, 0.8660254037844387076, 1.000000000000000000, 0.8660254037844387076, 1.000000000000000000, 0.8660254037844387076, 1.000000000000000000, 0.8660254037844387076, 1.000000000000000000, 0.8660254037844387076, 1.000000000000000000, 0.8660254037844387076, 1.000000000000000000, 0.8660254037844387076, 1.000000000000000000, 0.8660254037844387076, 1.000000000000000000, 0.8660254037844387076, 1.000000000000000000, 0.8660254037844387076, 1.000000000000000000, 0.8660254037844387076, 1.000000000000000000, 0.8660254037844387076, 1.000000000000000000, 0.8660254037844387076, 1.000000000000000000, 0.8660254037844387076, 1.000000000000000000, 0.8660254037844387076, 1.000000000000000000, 0.8660254037844387076, 1.000000000000000000, 0.8660254037844387076, 1.000000000000000000, 0.8660254037844387076, 1.000000000000000000, 0.8660254037844387076, 1.000000000000000000, 0.8660254037844387076, 1.000000000000000000, 0.8660254037844387076, 1.000000000000000000, 0.8660254037844387076, 1.000000000000000000, 0.8660254037844387076, 1.000000000000000000, 0.8660254037844387076, 1.000000000000000000, 0.8660254037844387076, 1.000000000000000000, 0.8660254037844387076, 1.000000000000000000, 0.8660254037844387076, 1.000000000000000000, 0.8660254037844387076, 1.000000000000000000, 0.8660254037844387076, 1.000000000000000000, 0.8660254037844387076, 1.000000000000000000, 0.8660254037844387076, 1.000000000000000000, 0.8660254037844387076, 1.000000000000000000, 0.8660254037844387076, 1.000000000000000000, 0.8660254037844387076, 1.000000000000000000, 0.8660254037844387076, 1.000000000000000000, 0.8660254037844387076, 1.000000000000000000, 0.8660254037844387076, 1.000000000000000000, 0.8660254037844387076, 1.000000000000000000, 0.8660254037844387076, 1.000000000000000000, 0.8660254037844387076, 1.000000000000000000, 0.8660254037844387076, 1.000000000000000000, 0.8660254037844387076, 1.000000000000000000, 0.8660254037844387076, 1.000000000000000000, 0.8660254037844387076, 1.000000000000000000, 0.8660254037844387076, 1.000000000000000000, 0.8660254037844387076, 1.000000000000000000, 0.8660254037844387076, 1.000000000000000000, 0.8660254037844387076, 1.000000000000000000, 0.8660254037844387076, 1.000000000000000000, 0.8660254037844387076, 1.000000000000000000, 0.8660254037844387076, 1.000000000000000000),
 ( 1.000000000000000000, 0.8660254037844387076, 1.000000000000000000, 0.8660254037844387076, 1.000000000000000000, 0.8660254037844387076, 1.000000000000000000, 0.8660254037844387076, 1.000000000000000000, 0.8660254037844387076, 1.000000000000000000, 0.8660254037844387076, 1.000000000000000000, 0.8660254037844387076, 1.000000000000000000, 0.8660254037844387076, 1.000000000000000000, 0.8660254037844387076, 1.000000000000000000, 0.8660254037844387076, 1.000000000000000000, 0.8660254037844387076, 1.000000000000000000, 0.8660254037844387076, 1.000000000000000000, 0.8660254037844387076, 1.000000000000000000, 0.8660254037844387076, 1.000000000000000000, 0.8660254037844387076, 1.000000000000000000, 0.8660254037844387076, 1.000000000000000000, 0.8660254037844387076, 1.000000000000000000, 0.8660254037844387076, 1.000000000000000000, 0.8660254037844387076, 1.000000000000000000, 0.8660254037844387076, 1.000000000000000000, 0.8660254037844387076, 1.000000000000000000, 0.8660254037844387076, 1.000000000000000000, 0.8660254037844387076, 1.000000000000000000, 0.8660254037844387076, 1.000000000000000000, 0.8660254037844387076, 1.000000000000000000, 0.8660254037844387076, 1.000000000000000000, 0.8660254037844387076, 1.000000000000000000, 0.8660254037844387076, 1.000000000000000000, 0.8660254037844387076, 1.000000000000000000, 0.8660254037844387076, 1.000000000000000000, 0.8660254037844387076, 1.000000000000000000, 0.8660254037844387076, 1.000000000000000000, 0.8660254037844387076, 1.000000000000000000, 0.8660254037844387076, 1.000000000000000000, 0.8660254037844387076, 1.000000000000000000, 0.8660254037844387076, 1.000000000000000000, 0.8660254037844387076, 1.000000000000000000, 0.8660254037844387076, 1.000000000000000000, 0.8660254037844387076, 1.000000000000000000, 0.8660254037844387076, 1.000000000000000000, 0.8660254037844387076, 1.000000000000000000, 0.8660254037844387076, 1.000000000000000000, 0.8660254037844387076, 1.000000000000000000, 0.8660254037844387076, 1.000000000000000000, 0.8660254037844387076, 1.000000000000000000, 0.8660254037844387076, 1.000000000000000000, 0.8660254037844387076, 1.000000000000000000, 0.8660254037844387076, 1.000000000000000000, 0.8660254037844387076, 1.000000000000000000, 0.8660254037844387076, 1.000000000000000000, 0.8660254037844387076, 1.000000000000000000, 0.8660254037844387076, 1.000000000000000000, 0.8660254037844387076, 1.000000000000000000, 0.8660254037844387076, 1.000000000000000000, 0.8660254037844387076, 1.000000000000000000, 0.8660254037844387076, 1.000000000000000000, 0.8660254037844387076, 1.000000000000000000, 0.8660254037844387076, 1.000000000000000000, 0.8660254037844387076, 1.000000000000000000, 0.8660254037844387076, 1.000000000000000000, 0.8660254037844387076, 1.000000000000000000, 0.8660254037844387076, 1.000000000000000000, 0.8660254037844387076, 1.000000000000000000, 0.8660254037844387076, 1.000000000000000000, 0.8660254037844387076, 1.000000000000000000, 0.8660254037844387076, 1.000000000000000000, 0.8660254037844387076, 1.000000000000000000, 0.8660254037844387076, 1.000000000000000000, 0.8660254037844387076, 1.000000000000000000, 0.8660254037844387076, 1.000000000000000000, 0.8660254037844387076, 1.000000000000000000, 0.8660254037844387076, 1.000000000000000000, 0.8660254037844387076, 1.000000000000000000, 0.8660254037844387076, 1.000000000000000000, 0.8660254037844387076, 1.000000000000000000, 0.8660254037844387076, 1.000000000000000000, 0.8660254037844387076, 1.000000000000000000, 0.8660254037844387076, 1.000000000000000000, 0.8660254037844387076, 1.000000000000000000, 0.8660254037844387076, 1.000000000000000000, 0.8660254037844387076, 1.000000000000000000, 0.8660254037844387076, 1.000000000000000000, 0.8660254037844387076, 1.000000000000000000, 0.8660254037844387076, 1.000000000000000000, 0.8660254037844387076, 1.000000000000000000, 0.8660254037844387076, 1.000000000000000000, 0.8660254037844387076, 1.000000000000000000, 0.8660254037844387076, 1.000000000000000000, 0.8660254037844387076, 1.000000000000000000, 0.8660254037844387076, 1.000000000000000000, 0.8660254037844387076, 1.000000000000000000, 0.8660254037844387076, 1.000000000000000000, 0.8660254037844387076, 1.000000000000000000, 0.8660254037844387076, 1.000000000000000000, 0.8660254037844387076, 1.000000000000000000, 0.8660254037844387076, 1.000000000000000000, 0.8660254037844387076, 1.000000000000000000, 0.8660254037844387076, 1.000000000000000000, 0.8660254037844387076, 1.000000000000000000, 0.8660254037844387076, 1.000000000000000000, 0.8660254037844387076, 1.000000000000000000, 0.8660254037844387076, 1.000000000000000000, 0.8660254037844387076, 1.000000000000000000, 0.8660254037844387076, 1.000000000000000000, 0.8660254037844387076, 1.000000000000000000, 0.8660254037844387076, 1.000000000000000000, 0.8660254037844387076, 1.000000000000000000, 0.8660254037844387076, 1.000000000000000000, 0.8660254037844387076, 1.000000000000000000, 0.8660254037844387076, 1.000000000000000000, 0.8660254037844387076, 1.000000000000000000, 0.8660254037844387076, 1.000000000000000000, 0.8660254037844387076, 1.000000000000000000, 0.8660254037844387076, 1.000000000000000000, 0.8660254037844387076, 1.000000000000000000, 0.8660254037844387076, 1.000000000000000000, 0.8660254037844387076, 1.000000000000000000, 0.8660254037844387076, 1.000000000000000000, 0.8660254037844387076, 1.000000000000000000, 0.8660254037844387076, 1.000000000000000000, 0.8660254037844387076, 1.000000000000000000, 0.8660254037844387076, 1.000000000000000000, 0.8660254037844387076, 1.000000000000000000, 0.8660254037844387076, 1.000000000000000000, 0.8660254037844387076, 1.000000000000000000, 0.8660254037844387076, 1.000000000000000000, 0.8660254037844387076, 1.000000000000000000, 0.8660254037844387076, 1.000000000000000000, 0.8660254037844387076, 1.000000000000000000, 0.8660254037844387076, 1.000000000000000000, 0.8660254037844387076, 1.000000000000000000, 0.8660254037844387076, 1.000000000000000000, 0.8660254037844387076, 1.000000000000000000, 0.8660254037844387076, 1.000000000000000000, 0.8660254037844387076, 1.000000000000000000, 0.8660254037844387076, 1.000000000000000000, 0.8660254037844387076, 1.000000000000000000, 0.8660254037844387076, 1.000000000000000000, 0.8660254037844387076, 1.000000000000000000, 0.8660254037844387076, 1.000000000000000000, 0.8660254037844387076, 1.000000000000000000, 0.8660254037844387076, 1.000000000000000000, 0.8660254037844387076, 1.000000000000000000, 0.8660254037844387076, 1.000000000000000000, 0.8660254037844387076, 1.000000000000000000, 0.8660254037844387076, 1.000000000000000000, 0.8660254037844387076, 1.000000000000000000, 0.8660254037844387076, 1.000000000000000000, 0.8660254037844387076, 1.000000000000000000, 0.8660254037844387076, 1.000000000000000000, 0.8660254037844387076, 1.000000000000000000, 0.8660254037844387076, 1.000000000000000000, 0.8660254037844387076, 1.000000000000000000, 0.8660254037844387076, 1.000000000000000000, 0.8660254037844387076, 1.000000000000000000, 0.8660254037844387076, 1.000000000000000000, 0.8660254037844387076, 1.000000000000000000, 0.8660254037844387076, 1.000000000000000000, 0.8660254037844387076, 1.000000000000000000, 0.8660254037844387076, 1.000000000000000000, 0.8660254037844387076, 1.000000000000000000, 0.8660254037844387076, 1.000000000000000000, 0.8660254037844387076, 1.000000000000000000, 0.8660254037844387076, 1.000000000000000000, 0.8660254037844387076, 1.000000000000000000, 0.8660254037844387076, 1.000000000000000000, 0.8660254037844387076, 1.000000000000000000, 0.8660254037844387076, 1.000000000000000000, 0.8660254037844387076, 1.000000000000000000, 0.8660254037844387076, 1.000000000000000000, 0.8660254037844387076, 1.000000000000000000, 0.8660254037844387076, 1.000000000000000000, 0.8660254037844387076, 1.000000000000000000, 0.8660254037844387076, 1.000000000000000000, 0.8660254037844387076, 1.000000000000000000, 0.8660254037844387076, 1.000000000000000000, 0.8660254037844387076, 1.000000000000000000, 0.8660254037844387076, 1.000000000000000000, 0.8660254037844387076, 1.000000000000000000, 0.8660254037844387076, 1.000000000000000000, 0.8660254037844387076, 1.000000000000000000, 0.8660254037844387076, 1.000000000000000000, 0.8660254037844387076, 1.000000000000000000, 0.8660254037844387076, 1.000000000000000000, 0.8660254037844387076, 1.000000000000000000, 0.8660254037844387076, 1.000000000000000000, 0.8660254037844387076, 1.000000000000000000, 0.8660254037844387076, 1.000000000000000000, 0.8660254037844387076, 1.000000000000000000, 0.8660254037844387076, 1.000000000000000000, 0.8660254037844387076, 1.000000000000000000, 0.8660254037844387076, 1.000000000000000000, 0.8660254037844387076, 1.000000000000000000, 0.8660254037844387076, 1.000000000000000000, 0.8660254037844387076, 1.000000000000000000, 0.8660254037844387076, 1.000000000000000000, 0.8660254037844387076, 1.000000000000000000, 0.8660254037844387076, 1.000000000000000000, 0.8660254037844387076, 1.000000000000000000, 0.8660254037844387076, 1.000000000000000000, 0.8660254037844387076, 1.000000000000000000, 0.8660254037844387076, 1.000000000000000000, 0.8660254037844387076, 1.000000000000000000, 0.8660254037844387076, 1.000000000000000000, 0.8660254037844387076, 1.000000000000000000, 0.8660254037844387076, 1.000000000000000000, 0.8660254037844387076, 1.000000000000000000, 0.8660254037844387076, 1.000000000000000000, 0.8660254037844387076, 1.000000000000000000, 0.8660254037844387076, 1.000000000000000000, 0.8660254037844387076, 1.000000000000000000, 0.8660254037844387076, 1.000000000000000000, 0.8660254037844387076, 1.000000000000000000, 0.8660254037844387076, 1.000000000000000000, 0.8660254037844387076, 1.000000000000000000, 0.8660254037844387076, 1.000000000000000000, 0.8660254037844387076, 1.000000000000000000, 0.8660254037844387076, 1.000000000000000000, 0.8660254037844387076, 1.000000000000000000, 0.8660254037844387076, 1.000000000000000000, 0.8660254037844387076, 1.000000000000000000, 0.8660254037844387076, 1.000000000000000000, 0.8660254037844387076, 1.000000000000000000, 0.8660254037844387076, 1.000000000000000000, 0.8660254037844387076, 1.000000000000000000, 0.8660254037844387076, 1.000000000000000000, 0.8660254037844387076, 1.000000000000000000, 0.8660254037844387076, 1.000000000000000000, 0.8660254037844387076, 1.000000000000000000, 0.8660254037844387076, 1.000000000000000000, 0.8660254037844387076, 1.000000000000000000, 0.8660254037844387076, 1.000000000000000000, 0.8660254037844387076, 1.000000000000000000, 0.8660254037844387076, 1.000000000000000000, 0.8660254037844387076, 1.000000000000000000, 0.8660254037844387076, 1.000000000000000000, 0.8660254037844387076, 1.000000000000000000, 0.8660254037844387076, 1.000000000000000000, 0.8660254037844387076, 1.000000000000000000, 0.8660254037844387076, 1.000000000000000000, 0.8660254037844387076, 1.000000000000000000, 0.8660254037844387076, 1.000000000000000000, 0.8660254037844387076, 1.000000000000000000, 0.8660254037844387076, 1.000000000000000000, 0.8660254037844387076, 1.000000000000000000, 0.8660254037844387076, 1.000000000000000000, 0.8660254037844387076, 1.000000000000000000, 0.8660254037844387076, 1.000000000000000000, 0.8660254037844387076, 1.000000000000000000, 0.8660254037844387076, 1.000000000000000000, 0.8660254037844387076, 1.000000000000000000, 0.8660254037844387076, 1.000000000000000000, 0.8660254037844387076, 1.000000000000000000, 0.8660254037844387076, 1.000000000000000000, 0.8660254037844387076, 1.000000000000000000, 0.8660254037844387076, 1.000000000000000000, 0.8660254037844387076, 1.000000000000000000, 0.8660254037844387076, 1.000000000000000000, 0.8660254037844387076, 1.000000000000000000, 0.8660254037844387076, 1.000000000000000000, 0.8660254037844387076, 1.000000000000000000, 0.8660254037844387076, 1.000000000000000000, 0.8660254037844387076, 1.000000000000000000, 0.8660254037844387076, 1.000000000000000000, 0.8660254037844387076, 1.000000000000000000, 0.8660254037844387076, 1.000000000000000000, 0.8660254037844387076, 1.000000000000000000, 0.8660254037844387076, 1.000000000000000000, 0.8660254037844387076, 1.000000000000000000, 0.8660254037844387076, 1.000000000000000000, 0.8660254037844387076, 1.000000000000000000, 0.8660254037844387076, 1.000000000000000000, 0.8660254037844387076, 1.000000000000000000, 0.8660254037844387076, 1.000000000000000000, 0.8660254037844387076, 1.000000000000000000, 0.8660254037844387076, 1.000000000000000000, 0.8660254037844387076, 1.000000000000000000, 0.8660254037844387076, 1.000000000000000000, 0.8660254037844387076, 1.000000000000000000, 0.8660254037844387076, 1.000000000000000000, 0.8660254037844387076, 1.000000000000000000, 0.8660254037844387076, 1.000000000000000000, 0.8660254037844387076, 1.000000000000000000, 0.8660254037844387076, 1.000000000000000000, 0.8660254037844387076, 1.000000000000000000, 0.8660254037844387076, 1.000000000000000000, 0.8660254037844387076, 1.000000000000000000, 0.8660254037844387076, 1.000000000000000000, 0.8660254037844387076, 1.000000000000000000, 0.8660254037844387076, 1.000000000000000000, 0.8660254037844387076, 1.000000000000000000, 0.8660254037844387076, 1.000000000000000000, 0.8660254037844387076, 1.000000000000000000, 0.8660254037844387076, 1.000000000000000000, 0.8660254037844387076, 1.000000000000000000, 0.8660254037844387076, 1.000000000000000000, 0.8660254037844387076, 1.000000000000000000, 0.8660254037844387076, 1.000000000000000000, 0.8660254037844387076, 1.000000000000000000, 0.8660254037844387076, 1.000000000000000000, 0.8660254037844387076, 1.000000000000000000, 0.8660254037844387076, 1.000000000000000000, 0.8660254037844387076, 1.000000000000000000, 0.8660254037844387076, 1.000000000000000000, 0.8660254037844387076, 1.000000000000000000, 0.8660254037844387076, 1.000000000000000000, 0.8660254037844387076, 1.000000000000000000, 0.8660254037844387076, 1.000000000000000000, 0.8660254037844387076, 1.000000000000000000, 0.8660254037844387076, 1.000000000000000000, 0.8660254037844387076, 1.000000000000000000, 0.8660254037844387076, 1.000000000000000000, 0.8660254037844387076, 1.000000000000000000, 0.8660254037844387076, 1.000000000000000000, 0.8660254037844387076, 1.000000000000000000, 0.8660254037844387076, 1.000000000000000000, 0.8660254037844387076, 1.000000000000000000, 0.8660254037844387076, 1.000000000000000000, 0.8660254037844387076, 1.000000000000000000, 0.8660254037844387076, 1.000000000000000000, 0.8660254037844387076, 1.000000000000000000, 0.8660254037844387076, 1.000000000000000000, 0.8660254037844387076, 1.000000000000000000, 0.8660254037844387076, 1.000000000000000000, 0.8660254037844387076, 1.000000000000000000, 0.8660254037844387076, 1.000000000000000000, 0.8660254037844387076, 1.000000000000000000, 0.8660254037844387076, 1.000000000000000000, 0.8660254037844387076, 1.000000000000000000, 0.8660254037844387076, 1.000000000000000000, 0.8660254037844387076, 1.000000000000000000, 0.8660254037844387076, 1.000000000000000000, 0.8660254037844387076, 1.000000000000000000, 0.8660254037844387076, 1.000000000000000000, 0.8660254037844387076, 1.000000000000000000, 0.8660254037844387076, 1.000000000000000000, 0.8660254037844387076, 1.000000000000000000, 0.8660254037844387076, 1.000000000000000000, 0.8660254037844387076, 1.000000000000000000, 0.8660254037844387076, 1.000000000000000000, 0.8660254037844387076, 1.000000000000000000, 0.8660254037844387076, 1.000000000000000000, 0.8660254037844387076, 1.000000000000000000, 0.8660254037844387076, 1.000000000000000000, 0.8660254037844387076, 1.000000000000000000, 0.8660254037844387076, 1.000000000000000000, 0.8660254037844387076, 1.000000000000000000, 0.8660254037844387076, 1.000000000000000000, 0.8660254037844387076, 1.000000000000000000, 0.8660254037844387076, 1.000000000000000000, 0.8660254037844387076, 1.000000000000000000, 0.8660254037844387076, 1.000000000000000000, 0.8660254037844387076, 1.000000000000000000, 0.8660254037844387076, 1.000000000000000000, 0.8660254037844387076, 1.000000000000000000, 0.8660254037844387076, 1.000000000000000000, 0.8660254037844387076, 1.000000000000000000, 0.8660254037844387076, 1.000000000000000000, 0.8660254037844387076, 1.000000000000000000, 0.8660254037844387076, 1.000000000000000000, 0.8660254037844387076, 1.000000000000000000, 0.8660254037844387076, 1.000000000000000000, 0.8660254037844387076, 1.000000000000000000, 0.8660254037844387076, 1.000000000000000000, 0.8660254037844387076, 1.000000000000000000, 0.8660254037844387076, 1.000000000000000000, 0.8660254037844387076, 1.000000000000000000, 0.8660254037844387076, 1.000000000000000000, 0.8660254037844387076, 1.000000000000000000, 0.8660254037844387076, 1.000000000000000000, 0.8660254037844387076, 1.000000000000000000, 0.8660254037844387076, 1.000000000000000000, 0.8660254037844387076, 1.000000000000000000, 0.8660254037844387076, 1.000000000000000000, 0.8660254037844387076, 1.000000000000000000, 0.8660254037844387076, 1.000000000000000000, 0.8660254037844387076, 1.000000000000000000, 0.8660254037844387076, 1.000000000000000000, 0.8660254037844387076, 1.000000000000000000, 0.8660254037844387076, 1.000000000000000000, 0.8660254037844387076, 1.000000000000000000, 0.8660254037844387076, 1.000000000000000000, 0.8660254037844387076, 1.000000000000000000, 0.8660254037844387076, 1.000000000000000000, 0.8660254037844387076, 1.000000000000000000, 0.8660254037844387076, 1.000000000000000000, 0.8660254037844387076, 1.000000000000000000, 0.8660254037844387076, 1.000000000000000000, 0.8660254037844387076, 1.000000000000000000, 0.8660254037844387076, 1.000000000000000000, 0.8660254037844387076, 1.000000000000000000, 0.8660254037844387076, 1.000000000000000000, 0.8660254037844387076, 1.000000000000000000, 0.8660254037844387076, 1.000000000000000000, 0.8660254037844387076, 1.000000000000000000, 0.8660254037844387076, 1.000000000000000000, 0.8660254037844387076, 1.000000000000000000, 0.8660254037844387076, 1.000000000000000000, 0.8660254037844387076, 1.000000000000000000, 0.8660254037844387076, 1.000000000000000000, 0.8660254037844387076, 1.000000000000000000, 0.8660254037844387076, 1.000000000000000000, 0.8660254037844387076, 1.000000000000000000, 0.8660254037844387076, 1.000000000000000000, 0.8660254037844387076, 1.000000000000000000, 0.8660254037844387076, 1.000000000000000000, 0.8660254037844387076, 1.000000000000000000, 0.8660254037844387076, 1.000000000000000000, 0.8660254037844387076, 1.000000000000000000, 0.8660254037844387076, 1.000000000000000000, 0.8660254037844387076, 1.000000000000000000, 0.8660254037844387076, 1.000000000000000000, 0.8660254037844387076, 1.000000000000000000, 0.8660254037844387076, 1.000000000000000000, 0.8660254037844387076, 1.000000000000000000, 0.8660254037844387076, 1.000000000000000000, 0.8660254037844387076, 1.000000000000000000, 0.8660254037844387076, 1.000000000000000000, 0.8660254037844387076, 1.000000000000000000, 0.8660254037844387076, 1.000000000000000000, 0.8660254037844387076, 1.000000000000000000, 0.8660254037844387076, 1.000000000000000000, 0.8660254037844387076, 1.000000000000000000, 0.8660254037844387076, 1.000000000000000000, 0.8660254037844387076, 1.000000000000000000, 0.8660254037844387076, 1.000000000000000000, 0.8660254037844387076, 1.000000000000000000, 0.8660254037844387076, 1.000000000000000000, 0.8660254037844387076, 1.000000000000000000, 0.8660254037844387076, 1.000000000000000000, 0.8660254037844387076, 1.000000000000000000, 0.8660254037844387076, 1.000000000000000000, 0.8660254037844387076, 1.000000000000000000, 0.8660254037844387076, 1.000000000000000000, 0.8660254037844387076, 1.000000000000000000, 0.8660254037844387076, 1.000000000000000000, 0.8660254037844387076, 1.000000000000000000, 0.8660254037844387076, 1.000000000000000000, 0.8660254037844387076, 1.000000000000000000, 0.8660254037844387076, 1.000000000000000000, 0.8660254037844387076, 1.000000000000000000, 0.8660254037844387076, 1.000000000000000000, 0.8660254037844387076, 1.000000000000000000, 0.8660254037844387076, 1.000000000000000000, 0.8660254037844387076, 1.000000000000000000, 0.8660254037844387076, 1.000000000000000000, 0.8660254037844387076, 1.000000000000000000, 0.8660254037844387076, 1.000000000000000000, 0.8660254037844387076, 1.000000000000000000, 0.8660254037844387076, 1.000000000000000000, 0.8660254037844387076, 1.000000000000000000, 0.8660254037844387076, 1.000000000000000000, 0.8660254037844387076, 1.000000000000000000, 0.8660254037844387076, 1.000000000000000000, 0.8660254037844387076, 1.000000000000000000, 0.8660254037844387076, 1.000000000000000000, 0.8660254037844387076, 1.000000000000000000, 0.8660254037844387076, 1.000000000000000000, 0.8660254037844387076, 1.000000000000000000, 0.8660254037844387076, 1.000000000000000000, 0.8660254037844387076, 1.000000000000000000, 0.8660254037844387076, 1.000000000000000000, 0.8660254037844387076, 1.000000000000000000, 0.8660254037844387076, 1.000000000000000000, 0.8660254037844387076, 1.000000000000000000, 0.8660254037844387076, 1.000000000000000000, 0.8660254037844387076, 1.000000000000000000, 0.8660254037844387076, 1.000000000000000000, 0.8660254037844387076, 1.000000000000000000, 0.8660254037844387076, 1.000000000000000000, 0.8660254037844387076, 1.000000000000000000, 0.8660254037844387076, 1.000000000000000000, 0.8660254037844387076, 1.000000000000000000, 0.8660254037844387076, 1.000000000000000000, 0.8660254037844387076, 1.000000000000000000, 0.8660254037844387076, 1.000000000000000000, 0.8660254037844387076, 1.000000000000000000, 0.8660254037844387076, 1.000000000000000000, 0.8660254037844387076, 1.000000000000000000, 0.8660254037844387076, 1.000000000000000000, 0.8660254037844387076, 1.000000000000000000, 0.8660254037844387076, 1.000000000000000000, 0.8660254037844387076, 1.000000000000000000, 0.8660254037844387076, 1.000000000000000000, 0.8660254037844387076, 1.000000000000000000, 0.8660254037844387076, 1.000000000000000000, 0.8660254037844387076, 1.000000000000000000, 0.8660254037844387076, 1.000000000000000000, 0.8660254037844387076, 1.000000000000000000, 0.8660254037844387076, 1.000000000000000000, 0.8660254037844387076, 1.000000000000000000, 0.8660254037844387076, 1.000000000000000000, 0.8660254037844387076, 1.000000000000000000, 0.8660254037844387076, 1.000000000000000000, 0.8660254037844387076, 1.000000000000000000, 0.8660254037844387076, 1.000000000000000000, 0.8660254037844387076, 1.000000000000000000, 0.8660254037844387076, 1.000000000000000000, 0.8660254037844387076, 1.000000000000000000, 0.8660254037844387076, 1.000000000000000000, 0.8660254037844387076, 1.000000000000000000, 0.8660254037844387076, 1.000000000000000000, 0.8660254037844387076, 1.000000000000000000, 0.8660254037844387076, 1.000000000000000000, 0.8660254037844387076, 1.000000000000000000, 0.8660254037844387076, 1.000000000000000000, 0.8660254037844387076, 1.000000000000000000, 0.8660254037844387076, 1.000000000000000000, 0.8660254037844387076, 1.000000000000000000, 0.8660254037844387076, 1.000000000000000000, 0.8660254037844387076, 1.000000000000000000, 0.8660254037844387076, 1.000000000000000000, 0.8660254037844387076, 1.000000000000000000, 0.8660254037844387076, 1.000000000000000000, 0.8660254037844387076, 1.000000000000000000, 0.8660254037844387076, 1.000000000000000000, 0.8660254037844387076, 1.000000000000000000, 0.8660254037844387076, 1.000000000000000000, 0.8660254037844387076, 1.000000000000000000, 0.8660254037844387076, 1.000000000000000000, 0.8660254037844387076, 1.000000000000000000, 0.8660254037844387076, 1.000000000000000000, 0.8660254037844387076, 1.000000000000000000, 0.8660254037844387076, 1.000000000000000000, 0.8660254037844387076, 1.000000000000000000, 0.8660254037844387076, 1.000000000000000000, 0.8660254037844387076, 1.000000000000000000, 0.8660254037844387076, 1.000000000000000000, 0.8660254037844387076, 1.000000000000000000, 0.8660254037844387076, 1.000000000000000000, 0.8660254037844387076, 1.000000000000000000, 0.8660254037844387076, 1.000000000000000000, 0.8660254037844387076, 1.000000000000000000, 0.8660254037844387076, 1.000000000000000000, 0.8660254037844387076, 1.000000000000000000, 0.8660254037844387076, 1.000000000000000000, 0.8660254037844387076, 1.000000000000000000, 0.8660254037844387076, 1.000000000000000000, 0.8660254037844387076, 1.000000000000000000, 0.8660254037844387076, 1.000000000000000000, 0.8660254037844387076, 1.000000000000000000, 0.8660254037844387076, 1.000000000000000000, 0.8660254037844387076, 1.000000000000000000, 0.8660254037844387076, 1.000000000000000000, 0.8660254037844387076, 1.000000000000000000, 0.8660254037844387076, 1.000000000000000000, 0.8660254037844387076, 1.000000000000000000, 0.8660254037844387076, 1.000000000000000000, 0.8660254037844387076, 1.000000000000000000, 0.8660254037844387076, 1.000000000000000000, 0.8660254037844387076, 1.000000000000000000, 0.8660254037844387076, 1.000000000000000000, 0.8660254037844387076, 1.000000000000000000, 0.8660254037844387076, 1.000000000000000000, 0.8660254037844387076, 1.000000000000000000, 0.8660254037844387076, 1.000000000000000000, 0.8660254037844387076, 1.000000000000000000, 0.8660254037844387076, 1.000000000000000000, 0.8660254037844387076, 1.000000000000000000, 0.8660254037844387076, 1.000000000000000000, 0.8660254037844387076, 1.000000000000000000, 0.8660254037844387076, 1.000000000000000000, 0.8660254037844387076, 1.000000000000000000, 0.8660254037844387076, 1.000000000000000000, 0.8660254037844387076, 1.000000000000000000, 0.8660254037844387076, 1.000000000000000000, 0.8660254037844387076, 1.000000000000000000, 0.8660254037844387076, 1.000000000000000000, 0.8660254037844387076, 1.000000000000000000, 0.8660254037844387076, 1.000000000000000000, 0.8660254037844387076, 1.000000000000000000, 0.8660254037844387076, 1.000000000000000000, 0.8660254037844387076, 1.000000000000000000, 0.8660254037844387076, 1.000000000000000000, 0.8660254037844387076, 1.000000000000000000, 0.8660254037844387076, 1.000000000000000000, 0.8660254037844387076, 1.000000000000000000, 0.8660254037844387076, 1.000000000000000000, 0.8660254037844387076, 1.000000000000000000, 0.8660254037844387076, 1.000000000000000000, 0.8660254037844387076, 1.000000000000000000, 0.8660254037844387076, 1.000000000000000000, 0.8660254037844387076, 1.000000000000000000, 0.8660254037844387076, 1.000000000000000000, 0.8660254037844387076, 1.000000000000000000, 0.8660254037844387076, 1.000000000000000000, 0.8660254037844387076, 1.000000000000000000, 0.8660254037844387076, 1.000000000000000000, 0.8660254037844387076, 1.000000000000000000, 0.8660254037844387076, 1.000000000000000000, 0.8660254037844387076, 1.000000000000000000, 0.8660254037844387076, 1.000000000000000000, 0.8660254037844387076, 1.000000000000000000, 0.8660254037844387076, 1.000000000000000000, 0.8660254037844387076, 1.000000000000000000, 0.8660254037844387076, 1.000000000000000000, 0.8660254037844387076, 1.000000000000000000, 0.8660254037844387076, 1.000000000000000000, 0.8660254037844387076, 1.000000000000000000, 0.8660254037844387076, 1.000000000000000000, 0.8660254037844387076, 1.000000000000000000, 0.8660254037844387076, 1.000000000000000000, 0.8660254037844387076, 1.000000000000000000, 0.8660254037844387076, 1.000000000000000000, 0.8660254037844387076, 1.000000000000000000, 0.8660254037844387076, 1.000000000000000000, 0.8660254037844387076, 1.000000000000000000, 0.8660254037844387076, 1.000000000000000000, 0.8660254037844387076, 1.000000000000000000, 0.8660254037844387076, 1.000000000000000000, 0.8660254037844387076, 1.000000000000000000, 0.8660254037844387076, 1.000000000000000000, 0.8660254037844387076, 1.000000000000000000, 0.8660254037844387076, 1.000000000000000000, 0.8660254037844387076, 1.000000000000000000, 0.8660254037844387076, 1.000000000000000000, 0.8660254037844387076, 1.000000000000000000, 0.8660254037844387076, 1.000000000000000000, 0.8660254037844387076, 1.000000000000000000, 0.8660254037844387076, 1.000000000000000000, 0.8660254037844387076, 1.000000000000000000, 0.8660254037844387076, 1.000000000000000000, 0.8660254037844387076, 1.000000000000000000, 0.8660254037844387076, 1.000000000000000000, 0.8660254037844387076, 1.000000000000000000, 0.8660254037844387076, 1.000000000000000000, 0.8660254037844387076, 1.000000000000000000, 0.8660254037844387076, 1.000000000000000000, 0.8660254037844387076, 1.000000000000000000, 0.8660254037844387076, 1.000000000000000000, 0.8660254037844387076, 1.000000000000000000, 0.8660254037844387076, 1.000000000000000000, 0.8660254037844387076, 1.000000000000000000, 0.8660254037844387076, 1.000000000000000000, 0.8660254037844387076, 1.000000000000000000, 0.8660254037844387076, 1.000000000000000000, 0.8660254037844387076, 1.000000000000000000, 0.8660254037844387076, 1.000000000000000000, 0.8660254037844387076, 1.000000000000000000, 0.8660254037844387076, 1.000000000000000000, 0.8660254037844387076, 1.000000000000000000, 0.8660254037844387076, 1.000000000000000000, 0.8660254037844387076, 1.000000000000000000, 0.8660254037844387076, 1.000000000000000000, 0.8660254037844387076, 1.000000000000000000, 0.8660254037844387076, 1.000000000000000000, 0.8660254037844387076, 1.000000000000000000, 0.8660254037844387076, 1.000000000000000000, 0.8660254037844387076, 1.000000000000000000, 0.8660254037844387076, 1.000000000000000000, 0.8660254037844387076, 1.000000000000000000, 0.8660254037844387076, 1.000000000000000000, 0.8660254037844387076, 1.000000000000000000, 0.8660254037844387076, 1.000000000000000000, 0.8660254037844387076, 1.000000000000000000, 0.8660254037844387076, 1.000000000000000000, 0.8660254037844387076, 1.000000000000000000, 0.8660254037844387076, 1.000000000000000000, 0.8660254037844387076, 1.000000000000000000, 0.8660254037844387076, 1.000000000000000000, 0.8660254037844387076, 1.000000000000000000, 0.8660254037844387076, 1.000000000000000000, 0.8660254037844387076, 1.000000000000000000, 0.8660254037844387076, 1.000000000000000000, 0.8660254037844387076, 1.000000000000000000, 0.8660254037844387076, 1.000000000000000000, 0.8660254037844387076, 1.000000000000000000, 0.8660254037844387076, 1.000000000000000000, 0.8660254037844387076, 1.000000000000000000, 0.8660254037844387076, 1.000000000000000000, 0.8660254037844387076, 1.000000000000000000, 0.8660254037844387076, 1.000000000000000000, 0.8660254037844387076, 1.000000000000000000, 0.8660254037844387076, 1.000000000000000000, 0.8660254037844387076, 1.000000000000000000, 0.8660254037844387076, 1.000000000000000000, 0.8660254037844387076, 1.000000000000000000, 0.8660254037844387076, 1.000000000000000000, 0.8660254037844387076, 1.000000000000000000, 0.8660254037844387076, 1.000000000000000000, 0.8660254037844387076, 1.000000000000000000, 0.8660254037844387076, 1.000000000000000000, 0.8660254037844387076, 1.000000000000000000, 0.8660254037844387076, 1.000000000000000000, 0.8660254037844387076, 1.000000000000000000, 0.8660254037844387076, 1.000000000000000000, 0.8660254037844387076, 1.000000000000000000, 0.8660254037844387076, 1.000000000000000000, 0.8660254037844387076, 1.000000000000000000, 0.8660254037844387076, 1.000000000000000000, 0.8660254037844387076, 1.000000000000000000, 0.8660254037844387076, 1.000000000000000000, 0.8660254037844387076, 1.000000000000000000, 0.8660254037844387076, 1.000000000000000000, 0.8660254037844387076, 1.000000000000000000, 0.8660254037844387076, 1.000000000000000000, 0.8660254037844387076, 1.000000000000000000, 0.8660254037844387076, 1.000000000000000000, 0.8660254037844387076, 1.000000000000000000, 0.8660254037844387076, 1.000000000000000000, 0.8660254037844387076, 1.000000000000000000, 0.8660254037844387076, 1.000000000000000000, 0.8660254037844387076, 1.000000000000000000, 0.8660254037844387076, 1.000000000000000000, 0.8660254037844387076, 1.000000000000000000, 0.8660254037844387076, 1.000000000000000000, 0.8660254037844387076, 1.000000000000000000, 0.8660254037844387076, 1.000000000000000000, 0.8660254037844387076, 1.000000000000000000, 0.8660254037844387076, 1.000000000000000000, 0.8660254037844387076, 1.000000000000000000, 0.8660254037844387076, 1.000000000000000000, 0.8660254037844387076, 1.000000000000000000, 0.8660254037844387076, 1.000000000000000000, 0.8660254037844387076, 1.000000000000000000, 0.8660254037844387076, 1.000000000000000000, 0.8660254037844387076, 1.000000000000000000, 0.8660254037844387076, 1.000000000000000000, 0.8660254037844387076, 1.000000000000000000, 0.8660254037844387076, 1.000000000000000000) ) ) 
 REPRESENTATION_ITEM ( '' )  SURFACE ( )  );
#21670=CARTESIAN_POINT ( 'NONE',  ( -7.022189441860112050E-16, 13.67729811471671653, -50.60160580289946353 ) ) ;
#21671=CARTESIAN_POINT ( 'NONE',  ( 1.655278471874998436, 14.63297358603754894, -109.5182724695661420 ) ) ;
#21672=ORIENTED_EDGE ( 'NONE', *, *, #38659, .F. ) ;
#21673=EDGE_CURVE ( 'NONE', #11460, #29607, #1883, .T. ) ;
#21675=VECTOR ( 'NONE', #19900, 1000.000000000000000 ) ;
#21677=CARTESIAN_POINT ( 'NONE',  ( 1.655278471874998436, 14.63297358603753828, -36.43077246956613635 ) ) ;
#21678=CARTESIAN_POINT ( 'NONE',  ( -3.310556943750002645, 15.58864905735836892, -63.76827246956614204 ) ) ;
#21679=CARTESIAN_POINT ( 'NONE',  ( 1.750000000000001110, 20.53108891324555785, -110.2943141357548456 ) ) ;
#21681=CARTESIAN_POINT ( 'NONE',  ( 2.340729813953370519E-16, 21.32270188528331190, -92.01410580289947916 ) ) ;
#21682=CARTESIAN_POINT ( 'NONE',  ( -1.394453263437886604E-15, 14.00000000000001421, -67.71098080242148853 ) ) ;
#21685=CARTESIAN_POINT ( 'NONE',  ( 3.500000000000001332, 17.50000000000001421, -63.46098080242150274 ) ) ;
#21687=CARTESIAN_POINT ( 'NONE',  ( 1.655278471875001101, 20.36702641396248481, -29.09743913623280420 ) ) ;
#21688=CARTESIAN_POINT ( 'NONE',  ( 3.500000000000001332, 17.50000000000001421, -56.15473080337743284 ) ) ;
#21690=CARTESIAN_POINT ( 'NONE',  ( -1.655278471875002211, 14.63297358603754894, -108.6849391362327992 ) ) ;
#21691=CARTESIAN_POINT ( 'NONE',  ( -7.022189441860112050E-16, 13.67729811471671653, -37.60160580289946353 ) ) ;
#21697=CARTESIAN_POINT ( 'NONE',  ( -3.310556943750001313, 17.50000000000001776, -87.76410580289947916 ) ) ;
#21699=EDGE_CURVE ( 'NONE', #25189, #25556, #40039, .T. ) ;
#21702=ORIENTED_EDGE ( 'NONE', *, *, #20859, .T. ) ;
#21704=CARTESIAN_POINT ( 'NONE',  ( 3.500000000000000000, 15.47927405783633503, -133.2380641367107614 ) ) ;
#21707=EDGE_CURVE ( 'NONE', #16409, #27367, #6231, .T. ) ;
#21709=CARTESIAN_POINT ( 'NONE',  ( 3.310556943749999981, 15.58864905735837070, -95.34743913623282197 ) ) ;
#21712=ORIENTED_EDGE ( 'NONE', *, *, #41780, .T. ) ;
#21716=ADVANCED_FACE ( 'NONE', ( #7931 ), #20897, .T. ) ;
#21722=CARTESIAN_POINT ( 'NONE',  ( -1.394453263437886604E-15, 14.00000000000001421, -56.71098080242150985 ) ) ;
#21724=CARTESIAN_POINT ( 'NONE',  ( -3.310556943750000425, 19.41135094264167549, -134.8474391362328220 ) ) ;
#21725=CARTESIAN_POINT ( 'NONE',  ( 0.9378221735089281585, 14.00000000000002309, -133.6663226036829712 ) ) ;
#21726=ORIENTED_EDGE ( 'NONE', *, *, #2258, .T. ) ;
#21727=CARTESIAN_POINT ( 'NONE',  ( 3.500000000000001332, 17.50000000000001776, -101.4609808024215170 ) ) ;
#21728=CARTESIAN_POINT ( 'NONE',  ( 1.655278471875001101, 20.36702641396249547, -126.1849391362327992 ) ) ;
#21729=CARTESIAN_POINT ( 'NONE',  ( 3.310556943749999981, 15.58864905735836537, -55.43493913623281344 ) ) ;
#21732=CARTESIAN_POINT ( 'NONE',  ( -3.500000000000001332, 17.50000000000002487, -133.6547308033774186 ) ) ;
#21735=CARTESIAN_POINT ( 'NONE',  ( -7.022189441860112050E-16, 13.67729811471672186, -79.60160580289945642 ) ) ;
#21736=CARTESIAN_POINT ( 'NONE',  ( 1.749999999999998224, 14.46891108675448656, -129.6276474690881741 ) ) ;
#21737=CARTESIAN_POINT ( 'NONE',  ( -3.310556943750002645, 15.58864905735837780, -112.6807724695661364 ) ) ;
#21740=CARTESIAN_POINT ( 'NONE',  ( 1.749999999999998224, 14.46891108675447946, -80.62764746908818836 ) ) ;
#21741=CARTESIAN_POINT ( 'NONE',  ( -1.750000000000002220, 14.46891108675447946, -61.79431413575483845 ) ) ;
#21742=CARTESIAN_POINT ( 'NONE',  ( -1.655278471875002211, 14.63297358603754184, -41.59743913623280065 ) ) ;
#21744=CARTESIAN_POINT ( 'NONE',  ( 2.340729813953370519E-16, 21.32270188528331190, -99.10160580289947063 ) ) ;
#21745=CARTESIAN_POINT ( 'NONE',  ( 4.648177544792955347E-16, 21.00000000000002487, -130.2109808024214885 ) ) ;
#21749=CARTESIAN_POINT ( 'NONE',  ( 1.655278471874998436, 14.63297358603755072, -124.5182724695661278 ) ) ;
#21750=CARTESIAN_POINT ( 'NONE',  ( -1.750000000000002220, 14.46891108675447768, -48.79431413575484555 ) ) ;
#21755=CYLINDRICAL_SURFACE ( 'NONE', #24715, 3.499999999999999556 ) ;
#21758=CARTESIAN_POINT ( 'NONE',  ( 3.310556943749999981, 15.58864905735836714, -77.43493913623279923 ) ) ;
#21759=FACE_OUTER_BOUND ( 'NONE', #38294, .T. ) ;
#21760=CARTESIAN_POINT ( 'NONE',  ( -1.749999999999999778, 20.53108891324555785, -102.8213974700440900 ) ) ;
#21761=CARTESIAN_POINT ( 'NONE',  ( 1.750000000000001110, 20.53108891324555429, -98.98806413671076143 ) ) ;
#21765=CARTESIAN_POINT ( 'NONE',  ( -3.310556943750000425, 19.41135094264166128, -32.84743913623280775 ) ) ;
#21766=EDGE_CURVE ( 'NONE', #12468, #32893, #10595, .T. ) ;
#21768=ADVANCED_FACE ( 'NONE', ( #5776 ), #11320, .T. ) ;
#21770=EDGE_LOOP ( 'NONE', ( #27993, #29385, #9114, #17444 ) ) ;
#21772=CARTESIAN_POINT ( 'NONE',  ( -3.310556943750001313, 17.50000000000001421, -49.76410580289947205 ) ) ;
#21773=ORIENTED_EDGE ( 'NONE', *, *, #41198, .F. ) ;
#21779=CARTESIAN_POINT ( 'NONE',  ( -1.749999999999999778, 20.53108891324555785, -119.8213974700440900 ) ) ;
#21780=CARTESIAN_POINT ( 'NONE',  ( 1.749999999999998224, 14.46891108675447590, -43.62764746908817415 ) ) ;
#21781=CARTESIAN_POINT ( 'NONE',  ( 1.750000000000001110, 20.53108891324554719, -41.29431413575483845 ) ) ;
#21782=CARTESIAN_POINT ( 'NONE',  ( 1.750000000000001110, 20.53108891324555429, -86.29431413575483134 ) ) ;
#21783=CARTESIAN_POINT ( 'NONE',  ( -3.500000000000000000, 19.52072594216370760, -64.73806413671076143 ) ) ;
#21784=DIRECTION ( 'NONE',  ( -0.000000000000000000, 1.259100132267607459E-16, -1.000000000000000000 ) ) ;
#21786=CARTESIAN_POINT ( 'NONE',  ( -3.310556943750000425, 19.41135094264165772, -24.93493913623280278 ) ) ;
#21787=CARTESIAN_POINT ( 'NONE',  ( 4.286263797015737581E-16, 14.00000000000002487, -149.5231586289125687 ) ) ;
#21788=CARTESIAN_POINT ( 'NONE',  ( 3.310556943749999981, 15.58864905735837425, -130.3474391362328220 ) ) ;
#21792=DIRECTION ( 'NONE',  ( 0.000000000000000000, 1.000000000000000000, 0.000000000000000000 ) ) ;
#21794=EDGE_CURVE ( 'NONE', #19108, #25556, #36668, .T. ) ;
#21795=CARTESIAN_POINT ( 'NONE',  ( 2.340729813953370519E-16, 21.32270188528331900, -115.1016058028994706 ) ) ;
#21796=CARTESIAN_POINT ( 'NONE',  ( 3.500000000000001332, 17.50000000000002487, -134.1547308033774186 ) ) ;
#21797=CARTESIAN_POINT ( 'NONE',  ( -3.500000000000002220, 15.47927405783632082, -39.57139747004409713 ) ) ;
#21798=CARTESIAN_POINT ( 'NONE',  ( -3.500000000000002220, 15.47927405783632437, -49.57139747004410424 ) ) ;
#21799=DIRECTION ( 'NONE',  ( -0.000000000000000000, 1.259100132267607459E-16, -1.000000000000000000 ) ) ;
#21801=CARTESIAN_POINT ( 'NONE',  ( 1.655278471875001101, 20.36702641396249902, -141.1849391362327708 ) ) ;
#21803=CARTESIAN_POINT ( 'NONE',  ( -3.310556943750001313, 17.50000000000001421, -50.85160580289946353 ) ) ;
#21806=CARTESIAN_POINT ( 'NONE',  ( 3.310556943750001313, 17.50000000000001421, -72.35160580289947063 ) ) ;
#21808=CARTESIAN_POINT ( 'NONE',  ( -3.310556943750002201, 15.58864905735837425, -97.68077246956613635 ) ) ;
#21809=CARTESIAN_POINT ( 'NONE',  ( -3.310556943750002645, 15.58864905735837070, -72.68077246956613635 ) ) ;
#21810=VERTEX_POINT ( 'NONE', #37481 ) ;
#21813=CARTESIAN_POINT ( 'NONE',  ( 3.310556943749999981, 15.58864905735836892, -90.43493913623281344 ) ) ;
#21816=EDGE_CURVE ( 'NONE', #5958, #5926, #4536, .T. ) ;
#21817=CARTESIAN_POINT ( 'NONE',  ( 0.9378221735089455890, 14.00000000000003197, -117.6663226036829712 ) ) ;
#21818=CARTESIAN_POINT ( 'NONE',  ( -3.310556943750001313, 17.50000000000001421, -53.76410580289947916 ) ) ;
#21819=CARTESIAN_POINT ( 'NONE',  ( 0.000000000000000000, 17.50000000000002487, -149.5231586289125687 ) ) ;
#21820=CARTESIAN_POINT ( 'NONE',  ( -3.310556943750000425, 19.41135094264166838, -109.8474391362328078 ) ) ;
#21822=ORIENTED_EDGE ( 'NONE', *, *, #26639, .F. ) ;
#21824=ORIENTED_EDGE ( 'NONE', *, *, #25616, .T. ) ;
#21826=CARTESIAN_POINT ( 'NONE',  ( 3.310556943750001313, 19.41135094264166128, -62.18077246956614346 ) ) ;
#21827=ORIENTED_EDGE ( 'NONE', *, *, #1325, .T. ) ;
#21830=DIRECTION ( 'NONE',  ( 0.000000000000000000, 1.000000000000000000, 0.000000000000000000 ) ) ;
#21833=ORIENTED_EDGE ( 'NONE', *, *, #25856, .F. ) ;
#21834=CYLINDRICAL_SURFACE ( 'NONE', #5860, 3.499999999999999556 ) ;
#21835=CARTESIAN_POINT ( 'NONE',  ( 1.655278471874998436, 14.63297358603755072, -130.4307724695661364 ) ) ;
#21838=CARTESIAN_POINT ( 'NONE',  ( 3.310556943750001313, 19.41135094264165772, -40.26827246956612782 ) ) ;
#21839=EDGE_CURVE ( 'NONE', #22548, #13986, #8885, .T. ) ;
#21840=CARTESIAN_POINT ( 'NONE',  ( 3.310556943750001313, 19.41135094264165772, -25.26827246956613138 ) ) ;
#21841=CARTESIAN_POINT ( 'NONE',  ( 3.310556943749999981, 15.58864905735837070, -95.43493913623279923 ) ) ;
#21842=CARTESIAN_POINT ( 'NONE',  ( -3.500000000000002220, 15.47927405783632082, -23.57139747004409713 ) ) ;
#21845=CARTESIAN_POINT ( 'NONE',  ( -1.655278471874999990, 20.36702641396249902, -141.0182724695661420 ) ) ;
#21847=CARTESIAN_POINT ( 'NONE',  ( -3.500000000000001332, 17.50000000000002132, -122.9609808024215027 ) ) ;
#21848=CARTESIAN_POINT ( 'NONE',  ( -3.500000000000002220, 15.47927405783632615, -80.57139747004410424 ) ) ;
#21849=CARTESIAN_POINT ( 'NONE',  ( -3.310556943750002201, 15.58864905735836892, -65.76827246956612782 ) ) ;
#21851=CARTESIAN_POINT ( 'NONE',  ( -1.394453263437886604E-15, 14.00000000000002132, -126.7109808024214885 ) ) ;
#21852=CARTESIAN_POINT ( 'NONE',  ( 0.000000000000000000, 17.50000000000002487, -149.5231586289125687 ) ) ;
#21853=CYLINDRICAL_SURFACE ( 'NONE', #8525, 3.499999999999999556 ) ;
#21854=ORIENTED_EDGE ( 'NONE', *, *, #34536, .T. ) ;
#21855=CARTESIAN_POINT ( 'NONE',  ( 3.310556943750001313, 17.50000000000002132, -120.2641058028994792 ) ) ;
#21857=CARTESIAN_POINT ( 'NONE',  ( 3.500000000000001332, 17.50000000000001421, -62.15473080337742573 ) ) ;
#21859=CARTESIAN_POINT ( 'NONE',  ( 3.500000000000001776, 19.52072594216371826, -106.0713974700441184 ) ) ;
#21862=DIRECTION ( 'NONE',  ( -0.000000000000000000, 1.259100132267607459E-16, -1.000000000000000000 ) ) ;
#21863=ADVANCED_FACE ( 'NONE', ( #18753 ), #11939, .T. ) ;
#21864=CARTESIAN_POINT ( 'NONE',  ( -0.9378221735089310451, 14.00000000000001066, -32.44938900211595012 ) ) ;
#21866=CARTESIAN_POINT ( 'NONE',  ( 3.310556943750001313, 19.41135094264166483, -71.18077246956613635 ) ) ;
#21867=DIRECTION ( 'NONE',  ( -0.000000000000000000, 1.259100132267607459E-16, -1.000000000000000000 ) ) ;
#21868=CARTESIAN_POINT ( 'NONE',  ( -4.299564228933483745E-15, 21.00000000000002842, -139.9047308033774186 ) ) ;
#21870=CARTESIAN_POINT ( 'NONE',  ( 4.648177544792955347E-16, 21.00000000000001776, -79.21098080242148853 ) ) ;
#21871=ORIENTED_EDGE ( 'NONE', *, *, #41246, .T. ) ;
#21873=CARTESIAN_POINT ( 'NONE',  ( -1.655278471875002211, 14.63297358603754539, -77.59743913623280775 ) ) ;
#21874=ORIENTED_EDGE ( 'NONE', *, *, #36802, .T. ) ;
#21875=ORIENTED_EDGE ( 'NONE', *, *, #8430, .F. ) ;
#21879=CARTESIAN_POINT ( 'NONE',  ( 1.749999999999998224, 14.46891108675448656, -129.3213974700441042 ) ) ;
#21880=CARTESIAN_POINT ( 'NONE',  ( 0.000000000000000000, 21.00000000000002487, -149.5231586289125687 ) ) ;
#21881=CARTESIAN_POINT ( 'NONE',  ( -3.310556943750002645, 15.58864905735836714, -46.76827246956613493 ) ) ;
#21882=CARTESIAN_POINT ( 'NONE',  ( 3.310556943750001313, 19.41135094264166838, -107.2682724695661420 ) ) ;
#21884=CARTESIAN_POINT ( 'NONE',  ( 1.655278471875001101, 20.36702641396248481, -36.09743913623281486 ) ) ;
#21885=CARTESIAN_POINT ( 'NONE',  ( -3.310556943750002645, 15.58864905735836892, -60.76827246956613493 ) ) ;
#21886=CARTESIAN_POINT ( 'NONE',  ( -3.500000000000002220, 15.47927405783632970, -106.8776474690881884 ) ) ;
#21888=CARTESIAN_POINT ( 'NONE',  ( -1.655278471874999990, 20.36702641396249192, -92.93077246956613635 ) ) ;
#21889=CARTESIAN_POINT ( 'NONE',  ( -3.500000000000002220, 15.47927405783632970, -96.57139747004409003 ) ) ;
#21890=DIRECTION ( 'NONE',  ( -0.000000000000000000, 1.259100132267607459E-16, -1.000000000000000000 ) ) ;
#21893=CARTESIAN_POINT ( 'NONE',  ( 3.500000000000000000, 15.47927405783632260, -61.54431413575484555 ) ) ;
#21894=CARTESIAN_POINT ( 'NONE',  ( -0.9378221735089291577, 21.00000000000001421, -72.16632260368299967 ) ) ;
#21895=CARTESIAN_POINT ( 'NONE',  ( -3.310556943750002645, 15.58864905735836182, -24.68077246956613990 ) ) ;
#21896=CARTESIAN_POINT ( 'NONE',  ( -3.500000000000000888, 19.52072594216370760, -50.73806413671076143 ) ) ;
#21898=CARTESIAN_POINT ( 'NONE',  ( -3.310556943750000425, 19.41135094264166838, -107.9349391362327992 ) ) ;
#21899=CARTESIAN_POINT ( 'NONE',  ( -3.310556943750000425, 19.41135094264166128, -30.93493913623279923 ) ) ;
#21906=CARTESIAN_POINT ( 'NONE',  ( -3.310556943750000425, 19.41135094264166838, -89.84743913623280775 ) ) ;
#21908=CARTESIAN_POINT ( 'NONE',  ( 4.648177544792955347E-16, 21.00000000000001066, -24.21098080242150985 ) ) ;
#21911=CARTESIAN_POINT ( 'NONE',  ( 3.500000000000001332, 19.52072594216370760, -74.37764746908817415 ) ) ;
#21915=CARTESIAN_POINT ( 'NONE',  ( -3.310556943750002645, 15.58864905735837425, -97.68077246956613635 ) ) ;
#21917=ORIENTED_EDGE ( 'NONE', *, *, #3480, .F. ) ;
#21918=CARTESIAN_POINT ( 'NONE',  ( 0.000000000000000000, 17.50000000000002487, -149.5231586289125687 ) ) ;
#21919=ORIENTED_EDGE ( 'NONE', *, *, #14798, .T. ) ;
#21920=( BOUNDED_CURVE ( )  B_SPLINE_CURVE ( 2, ( #27950, #40925, #11780, #22199, #17965, #24776, #41145, #37740, #11569 ),
 .UNSPECIFIED., .F., .F. ) 
 B_SPLINE_CURVE_WITH_KNOTS ( ( 3, 2, 2, 2, 3 ),
 ( 0.2479166666666666741, 0.2486111111111111160, 0.2500000000000000000, 0.2513888888888888840, 0.2520833333333333259 ),
 .UNSPECIFIED. ) 
 CURVE ( )  GEOMETRIC_REPRESENTATION_ITEM ( )  RATIONAL_B_SPLINE_CURVE ( ( 0.9330127018922194093, 0.9330127018922194093, 1.000000000000000000, 0.8660254037844387076, 1.000000000000000000, 0.8660254037844387076, 1.000000000000000000, 0.9330127018922194093, 0.9330127018922194093 ) ) 
 REPRESENTATION_ITEM ( '' )  );
#21922=( BOUNDED_CURVE ( )  B_SPLINE_CURVE ( 2, ( #21745, #28126, #1565, #15162, #20915, #24325, #31113, #34719, #5587 ),
 .UNSPECIFIED., .F., .T. ) 
 B_SPLINE_CURVE_WITH_KNOTS ( ( 3, 2, 2, 2, 3 ),
 ( 0.1104166666666666630, 0.1111111111111111049, 0.1125000000000000028, 0.1138888888888888867, 0.1145833333333333426 ),
 .UNSPECIFIED. ) 
 CURVE ( )  GEOMETRIC_REPRESENTATION_ITEM ( )  RATIONAL_B_SPLINE_CURVE ( ( 0.9330127018922194093, 0.9330127018922194093, 1.000000000000000000, 0.8660254037844387076, 1.000000000000000000, 0.8660254037844387076, 1.000000000000000000, 0.9330127018922187432, 0.9330127018922194093 ) ) 
 REPRESENTATION_ITEM ( '' )  );
#21927=ORIENTED_EDGE ( 'NONE', *, *, #20988, .T. ) ;
#21930=CARTESIAN_POINT ( 'NONE',  ( 3.310556943750001313, 19.41135094264167549, -136.1807724695661364 ) ) ;
#21931=CARTESIAN_POINT ( 'NONE',  ( 4.648177544792955347E-16, 21.00000000000001066, -37.90473080337743284 ) ) ;
#21932=ORIENTED_EDGE ( 'NONE', *, *, #10494, .T. ) ;
#21935=CARTESIAN_POINT ( 'NONE',  ( -3.310556943750000425, 19.41135094264166838, -125.9349391362327992 ) ) ;
#21936=CARTESIAN_POINT ( 'NONE',  ( 1.655278471875001101, 20.36702641396248836, -50.18493913623279923 ) ) ;
#21938=VECTOR ( 'NONE', #31092, 1000.000000000000000 ) ;
#21940=CARTESIAN_POINT ( 'NONE',  ( 3.500000000000001776, 19.52072594216372181, -134.0713974700440758 ) ) ;
#21942=CARTESIAN_POINT ( 'NONE',  ( 2.340729813953370519E-16, 21.32270188528331190, -77.10160580289947063 ) ) ;
#21943=CARTESIAN_POINT ( 'NONE',  ( -1.749999999999999778, 20.53108891324555785, -125.1276474690881599 ) ) ;
#21944=CARTESIAN_POINT ( 'NONE',  ( -3.310556943750000425, 19.41135094264166838, -108.8474391362328220 ) ) ;
#21945=EDGE_CURVE ( 'NONE', #5191, #15247, #13233, .T. ) ;
#21946=CARTESIAN_POINT ( 'NONE',  ( 4.286263797015737581E-16, 14.00000000000002487, -149.5231586289125687 ) ) ;
#21949=CARTESIAN_POINT ( 'NONE',  ( 1.749999999999998224, 14.46891108675448123, -82.62764746908818836 ) ) ;
#21950=CARTESIAN_POINT ( 'NONE',  ( 3.500000000000001332, 17.50000000000002132, -103.1547308033774186 ) ) ;
#21951=CARTESIAN_POINT ( 'NONE',  ( -1.655278471874999990, 20.36702641396248481, -44.93077246956614346 ) ) ;
#21953=CARTESIAN_POINT ( 'NONE',  ( -1.655278471874999990, 20.36702641396249547, -104.0182724695661278 ) ) ;
#21954=CARTESIAN_POINT ( 'NONE',  ( -1.750000000000002220, 14.46891108675448656, -113.7943141357548456 ) ) ;
#21956=VERTEX_POINT ( 'NONE', #9172 ) ;
#21957=CARTESIAN_POINT ( 'NONE',  ( -1.655278471874999990, 20.36702641396249547, -121.0182724695661278 ) ) ;
#21962=CARTESIAN_POINT ( 'NONE',  ( 3.500000000000001332, 17.50000000000001421, -60.46098080242151696 ) ) ;
#21963=CARTESIAN_POINT ( 'NONE',  ( -1.749999999999999778, 20.53108891324555074, -63.12764746908818125 ) ) ;
#21966=CARTESIAN_POINT ( 'NONE',  ( 1.655278471874998436, 14.63297358603754361, -74.51827246956612782 ) ) ;
#21970=CARTESIAN_POINT ( 'NONE',  ( 4.648177544792955347E-16, 21.00000000000001421, -69.90473080337741862 ) ) ;
#21973=AXIS2_PLACEMENT_3D ( 'NONE', #10760, #13746, #13324 ) ;
#21975=CARTESIAN_POINT ( 'NONE',  ( 3.310556943750001313, 17.50000000000001066, -36.26410580289947205 ) ) ;
#21976=VECTOR ( 'NONE', #25275, 1000.000000000000000 ) ;
#21977=EDGE_CURVE ( 'NONE', #2623, #3992, #17594, .T. ) ;
#21984=CARTESIAN_POINT ( 'NONE',  ( 2.340729813953370519E-16, 21.32270188528330834, -47.01410580289947205 ) ) ;
#21986=ORIENTED_EDGE ( 'NONE', *, *, #14337, .T. ) ;
#21988=CARTESIAN_POINT ( 'NONE',  ( -1.749999999999999778, 20.53108891324554719, -25.12764746908817415 ) ) ;
#21991=FACE_OUTER_BOUND ( 'NONE', #6910, .T. ) ;
#21992=CARTESIAN_POINT ( 'NONE',  ( 2.474675557024783212E-16, 21.54145188432739033, -35.21098080242150985 ) ) ;
#21994=CARTESIAN_POINT ( 'NONE',  ( 0.9378221735089300459, 21.00000000000001776, -82.25563900116002003 ) ) ;
#21995=VECTOR ( 'NONE', #13649, 1000.000000000000000 ) ;
#21996=CARTESIAN_POINT ( 'NONE',  ( -1.394453263437886604E-15, 14.00000000000001776, -96.71098080242150274 ) ) ;
#21998=CARTESIAN_POINT ( 'NONE',  ( -3.500000000000000888, 19.52072594216372181, -142.0443141357548313 ) ) ;
#22000=CARTESIAN_POINT ( 'NONE',  ( -7.022189441860112050E-16, 13.67729811471672718, -123.5141058028994649 ) ) ;
#22003=ADVANCED_FACE ( 'NONE', ( #29942 ), #35119, .T. ) ;
#22004=( BOUNDED_CURVE ( )  B_SPLINE_CURVE ( 2, ( #35202, #28612, #41816, #38608, #9473, #28401, #6281, #41387, #13079 ),
 .UNSPECIFIED., .F., .F. ) 
 B_SPLINE_CURVE_WITH_KNOTS ( ( 3, 2, 2, 2, 3 ),
 ( 0.6104166666666667185, 0.6111111111111111605, 0.6125000000000000444, 0.6138888888888889284, 0.6145833333333333703 ),
 .UNSPECIFIED. ) 
 CURVE ( )  GEOMETRIC_REPRESENTATION_ITEM ( )  RATIONAL_B_SPLINE_CURVE ( ( 0.9330127018922194093, 0.9330127018922194093, 1.000000000000000000, 0.8660254037844387076, 1.000000000000000000, 0.8660254037844387076, 1.000000000000000000, 0.9330127018922194093, 0.9330127018922194093 ) ) 
 REPRESENTATION_ITEM ( '' )  );
#22006=CARTESIAN_POINT ( 'NONE',  ( 4.648177544792955347E-16, 21.00000000000001066, -23.90473080337742928 ) ) ;
#22007=EDGE_CURVE ( 'NONE', #19887, #12825, #3786, .T. ) ;
#22008=CARTESIAN_POINT ( 'NONE',  ( 3.310556943750001313, 17.50000000000002132, -117.3516058028994706 ) ) ;
#22010=CARTESIAN_POINT ( 'NONE',  ( -1.750000000000002220, 14.46891108675447590, -35.48806413671076854 ) ) ;
#22011=CARTESIAN_POINT ( 'NONE',  ( 1.749999999999998224, 14.46891108675448123, -92.32139747004409003 ) ) ;
#22013=CARTESIAN_POINT ( 'NONE',  ( 2.340729813953370519E-16, 21.32270188528332255, -137.1016058028994564 ) ) ;
#22016=CARTESIAN_POINT ( 'NONE',  ( 1.655278471875001101, 20.36702641396248481, -46.18493913623279923 ) ) ;
#22018=CARTESIAN_POINT ( 'NONE',  ( -1.749999999999999778, 20.53108891324555785, -114.8213974700440900 ) ) ;
#22019=CARTESIAN_POINT ( 'NONE',  ( -1.655278471875002211, 14.63297358603754539, -67.68493913623279923 ) ) ;
#22021=CARTESIAN_POINT ( 'NONE',  ( -3.310556943750000425, 19.41135094264166128, -67.84743913623280775 ) ) ;
#22022=ORIENTED_EDGE ( 'NONE', *, *, #1843, .T. ) ;
#22023=CARTESIAN_POINT ( 'NONE',  ( 1.655278471875001101, 20.36702641396249192, -90.18493913623279923 ) ) ;
#22025=CARTESIAN_POINT ( 'NONE',  ( -3.500000000000001332, 17.50000000000002132, -107.9609808024215027 ) ) ;
#22026=DIRECTION ( 'NONE',  ( -0.000000000000000000, 1.259100132267607459E-16, -1.000000000000000000 ) ) ;
#22027=CARTESIAN_POINT ( 'NONE',  ( 3.500000000000001332, 17.50000000000002487, -131.4609808024214885 ) ) ;
#22028=CARTESIAN_POINT ( 'NONE',  ( 1.655278471875001101, 20.36702641396248836, -49.09743913623280775 ) ) ;
#22029=CARTESIAN_POINT ( 'NONE',  ( -3.500000000000000000, 19.52072594216371826, -137.7380641367107614 ) ) ;
#22030=CARTESIAN_POINT ( 'NONE',  ( -3.310556943750002645, 15.58864905735837780, -112.6807724695661364 ) ) ;
#22032=VERTEX_POINT ( 'NONE', #20379 ) ;
#22035=ORIENTED_EDGE ( 'NONE', *, *, #17284, .T. ) ;
#22037=CARTESIAN_POINT ( 'NONE',  ( 3.310556943750001313, 17.50000000000001421, -63.26410580289947205 ) ) ;
#22038=ORIENTED_EDGE ( 'NONE', *, *, #41073, .F. ) ;
#22039=ORIENTED_EDGE ( 'NONE', *, *, #22574, .F. ) ;
#22044=AXIS2_PLACEMENT_3D ( 'NONE', #38155, #14576, #8808 ) ;
#22048=CARTESIAN_POINT ( 'NONE',  ( 3.310556943749999981, 15.58864905735837425, -128.3474391362328220 ) ) ;
#22050=CARTESIAN_POINT ( 'NONE',  ( -7.022189441860112050E-16, 13.67729811471671653, -40.60160580289947063 ) ) ;
#22051=CARTESIAN_POINT ( 'NONE',  ( -1.655278471875002211, 14.63297358603754006, -26.68493913623279212 ) ) ;
#22052=EDGE_CURVE ( 'NONE', #19472, #28716, #36326, .T. ) ;
#22053=CARTESIAN_POINT ( 'NONE',  ( -3.310556943750000425, 19.41135094264166483, -93.93493913623279923 ) ) ;
#22054=CARTESIAN_POINT ( 'NONE',  ( -1.655278471875002211, 14.63297358603755427, -142.5974391362327935 ) ) ;
#22056=( BOUNDED_CURVE ( )  B_SPLINE_CURVE ( 2, ( #41109, #24740, #28331, #8979, #21950, #24951, #31524, #41317, #12165 ),
 .UNSPECIFIED., .F., .T. ) 
 B_SPLINE_CURVE_WITH_KNOTS ( ( 3, 2, 2, 2, 3 ),
 ( 0.3312499999999999889, 0.3319444444444444309, 0.3333333333333333148, 0.3347222222222221988, 0.3354166666666666963 ),
 .UNSPECIFIED. ) 
 CURVE ( )  GEOMETRIC_REPRESENTATION_ITEM ( )  RATIONAL_B_SPLINE_CURVE ( ( 0.9330127018922194093, 0.9330127018922194093, 1.000000000000000000, 0.8660254037844387076, 1.000000000000000000, 0.8660254037844387076, 1.000000000000000000, 0.9330127018922167448, 0.9330127018922194093 ) ) 
 REPRESENTATION_ITEM ( '' )  );
#22058=EDGE_CURVE ( 'NONE', #16447, #12311, #6192, .T. ) ;
#22059=CARTESIAN_POINT ( 'NONE',  ( 3.310556943750001313, 19.41135094264167549, -133.2682724695661136 ) ) ;
#22061=CARTESIAN_POINT ( 'NONE',  ( -1.394453263437886604E-15, 14.00000000000001776, -83.71098080242150274 ) ) ;
#22064=CARTESIAN_POINT ( 'NONE',  ( -1.749999999999999778, 20.53108891324555785, -122.8213974700441042 ) ) ;
#22065=CARTESIAN_POINT ( 'NONE',  ( -7.424026671074350129E-16, 13.45854811567263631, -81.40473080337743284 ) ) ;
#22066=CARTESIAN_POINT ( 'NONE',  ( -1.655278471874999990, 20.36702641396248836, -65.01827246956614204 ) ) ;
#22069=CARTESIAN_POINT ( 'NONE',  ( -3.500000000000000000, 19.52072594216370760, -58.73806413671076143 ) ) ;
#22070=CARTESIAN_POINT ( 'NONE',  ( -3.310556943750002645, 15.58864905735837247, -83.76827246956612782 ) ) ;
#22072=CARTESIAN_POINT ( 'NONE',  ( 1.655278471874998436, 14.63297358603754894, -115.4307724695661364 ) ) ;
#22076=EDGE_LOOP ( 'NONE', ( #8954, #12085, #17061, #7061 ) ) ;
#22077=CARTESIAN_POINT ( 'NONE',  ( -1.749999999999999778, 20.53108891324555785, -105.8213974700441042 ) ) ;
#22078=CARTESIAN_POINT ( 'NONE',  ( -1.750000000000002220, 14.46891108675447590, -28.48806413671076143 ) ) ;
#22081=CARTESIAN_POINT ( 'NONE',  ( 7.367361408496833051E-14, 14.00000000000001776, -108.4047308033774186 ) ) ;
#22084=CARTESIAN_POINT ( 'NONE',  ( -1.655278471874999990, 20.36702641396248836, -63.93077246956614346 ) ) ;
#22087=CARTESIAN_POINT ( 'NONE',  ( -3.500000000000001332, 17.50000000000002132, -125.6547308033774470 ) ) ;
#22088=ORIENTED_EDGE ( 'NONE', *, *, #36346, .F. ) ;
#22089=CARTESIAN_POINT ( 'NONE',  ( 1.655278471874998436, 14.63297358603753651, -25.43077246956613990 ) ) ;
#22090=CARTESIAN_POINT ( 'NONE',  ( -3.310556943750001313, 17.50000000000001776, -80.76410580289946495 ) ) ;
#22092=ORIENTED_EDGE ( 'NONE', *, *, #5303, .F. ) ;
#22093=CARTESIAN_POINT ( 'NONE',  ( 0.000000000000000000, 17.50000000000002487, -149.5231586289125687 ) ) ;
#22100=CARTESIAN_POINT ( 'NONE',  ( 1.655278471874998436, 14.63297358603754006, -42.51827246956613493 ) ) ;
#22102=CARTESIAN_POINT ( 'NONE',  ( -1.655278471874999990, 20.36702641396249547, -107.0182724695661278 ) ) ;
#22103=VERTEX_POINT ( 'NONE', #18957 ) ;
#22104=CARTESIAN_POINT ( 'NONE',  ( -3.310556943750000425, 19.41135094264165772, -27.84743913623280065 ) ) ;
#22105=CARTESIAN_POINT ( 'NONE',  ( 3.310556943750001313, 19.41135094264166128, -59.26827246956613493 ) ) ;
#22106=CARTESIAN_POINT ( 'NONE',  ( 2.474675557024783212E-16, 21.54145188432740099, -105.2109808024215027 ) ) ;
#22108=CARTESIAN_POINT ( 'NONE',  ( 3.500000000000001332, 17.50000000000001776, -96.15473080337743284 ) ) ;
#22111=CARTESIAN_POINT ( 'NONE',  ( 2.474675557024783212E-16, 21.54145188432739388, -58.21098080242151696 ) ) ;
#22112=CARTESIAN_POINT ( 'NONE',  ( -3.500000000000002220, 15.47927405783632437, -46.87764746908817415 ) ) ;
#22113=CARTESIAN_POINT ( 'NONE',  ( -1.655278471874999990, 20.36702641396248481, -27.93077246956614346 ) ) ;
#22114=CARTESIAN_POINT ( 'NONE',  ( -3.500000000000001332, 17.50000000000001421, -49.65473080337742573 ) ) ;
#22115=CARTESIAN_POINT ( 'NONE',  ( -3.500000000000001332, 17.50000000000001066, -45.96098080242150274 ) ) ;
#22116=CARTESIAN_POINT ( 'NONE',  ( -1.655278471875002211, 14.63297358603754894, -103.6849391362328134 ) ) ;
#22117=CARTESIAN_POINT ( 'NONE',  ( 1.655278471874998436, 14.63297358603753828, -32.51827246956613493 ) ) ;
#22124=CARTESIAN_POINT ( 'NONE',  ( -7.022189441860112050E-16, 13.67729811471672363, -88.51410580289947916 ) ) ;
#22127=CARTESIAN_POINT ( 'NONE',  ( -3.500000000000001332, 17.50000000000001776, -101.9609808024215170 ) ) ;
#22130=ORIENTED_EDGE ( 'NONE', *, *, #17519, .T. ) ;
#22133=CARTESIAN_POINT ( 'NONE',  ( -1.655278471875002211, 14.63297358603754716, -93.59743913623280775 ) ) ;
#22135=EDGE_LOOP ( 'NONE', ( #9366, #4142, #39765, #20577 ) ) ;
#22136=DIRECTION ( 'NONE',  ( -0.000000000000000000, 1.259100132267607459E-16, -1.000000000000000000 ) ) ;
#22140=DIRECTION ( 'NONE',  ( -0.000000000000000000, 1.259100132267607459E-16, -1.000000000000000000 ) ) ;
#22145=CARTESIAN_POINT ( 'NONE',  ( -1.394453263437886604E-15, 14.00000000000001421, -79.71098080242148853 ) ) ;
#22146=CARTESIAN_POINT ( 'NONE',  ( 1.655278471875001101, 20.36702641396249902, -130.0974391362328220 ) ) ;
#22148=ORIENTED_EDGE ( 'NONE', *, *, #39361, .F. ) ;
#22149=CARTESIAN_POINT ( 'NONE',  ( -3.500000000000001332, 17.50000000000001066, -31.65473080337742573 ) ) ;
#22150=EDGE_CURVE ( 'NONE', #28708, #34399, #31806, .T. ) ;
#22151=CARTESIAN_POINT ( 'NONE',  ( 3.310556943750001313, 17.50000000000002132, -127.3516058028994422 ) ) ;
#22152=CARTESIAN_POINT ( 'NONE',  ( 3.310556943750001313, 17.50000000000001421, -52.35160580289946353 ) ) ;
#22153=ORIENTED_EDGE ( 'NONE', *, *, #4892, .F. ) ;
#22154=CARTESIAN_POINT ( 'NONE',  ( 1.749999999999998224, 14.46891108675448656, -129.3213974700441042 ) ) ;
#22156=VECTOR ( 'NONE', #36267, 1000.000000000000000 ) ;
#22159=CARTESIAN_POINT ( 'NONE',  ( -3.310556943750002645, 15.58864905735837070, -78.76827246956614204 ) ) ;
#22160=CARTESIAN_POINT ( 'NONE',  ( 1.750000000000001110, 20.53108891324555785, -123.2943141357548456 ) ) ;
#22161=CARTESIAN_POINT ( 'NONE',  ( 3.310556943750001313, 17.50000000000002132, -107.2641058028994649 ) ) ;
#22162=CARTESIAN_POINT ( 'NONE',  ( 3.310556943750001313, 17.50000000000001066, -23.35160580289946708 ) ) ;
#22165=CARTESIAN_POINT ( 'NONE',  ( -3.500000000000002220, 15.47927405783632615, -73.87764746908817415 ) ) ;
#22167=CARTESIAN_POINT ( 'NONE',  ( -1.655278471874999990, 20.36702641396248481, -41.93077246956614346 ) ) ;
#22168=CARTESIAN_POINT ( 'NONE',  ( -3.310556943750000425, 19.41135094264166838, -102.9349391362327992 ) ) ;
#22170=CARTESIAN_POINT ( 'NONE',  ( 3.500000000000001776, 19.52072594216370760, -62.07139747004410424 ) ) ;
#22172=CARTESIAN_POINT ( 'NONE',  ( 2.340729813953370519E-16, 21.32270188528331900, -123.1016058028994564 ) ) ;
#22177=CARTESIAN_POINT ( 'NONE',  ( -1.749999999999999778, 20.53108891324555074, -71.82139747004409003 ) ) ;
#22178=CARTESIAN_POINT ( 'NONE',  ( -1.750000000000002220, 14.46891108675447768, -52.48806413671076854 ) ) ;
#22180=ORIENTED_EDGE ( 'NONE', *, *, #5585, .T. ) ;
#22181=( BOUNDED_CURVE ( )  B_SPLINE_CURVE ( 2, ( #15859, #3487, #6055, #12656, #6482, #16477, #38596, #2868, #13279 ),
 .UNSPECIFIED., .F., .T. ) 
 B_SPLINE_CURVE_WITH_KNOTS ( ( 3, 2, 2, 2, 3 ),
 ( 0.03958333333333333842, 0.04027777777777778040, 0.04166666666666666435, 0.04305555555555555525, 0.04375000000000000416 ),
 .UNSPECIFIED. ) 
 CURVE ( )  GEOMETRIC_REPRESENTATION_ITEM ( )  RATIONAL_B_SPLINE_CURVE ( ( 0.9330127018922192983, 0.9330127018922196314, 1.000000000000000000, 0.8660254037844387076, 1.000000000000000000, 0.8660254037844387076, 1.000000000000000000, 0.9330127018922189652, 0.9330127018922192983 ) ) 
 REPRESENTATION_ITEM ( '' )  );
#22182=CARTESIAN_POINT ( 'NONE',  ( -3.310556943750000425, 19.41135094264166838, -75.93493913623279923 ) ) ;
#22183=CARTESIAN_POINT ( 'NONE',  ( 3.500000000000001332, 19.52072594216370405, -40.37764746908817415 ) ) ;
#22185=CARTESIAN_POINT ( 'NONE',  ( -3.500000000000001332, 17.50000000000002487, -139.6547308033774186 ) ) ;
#22188=CARTESIAN_POINT ( 'NONE',  ( -3.310556943750002201, 15.58864905735836537, -35.68077246956613635 ) ) ;
#22189=CARTESIAN_POINT ( 'NONE',  ( 0.9378221735089300459, 21.00000000000001421, -71.94938900211595012 ) ) ;
#22191=ORIENTED_EDGE ( 'NONE', *, *, #29335, .F. ) ;
#22197=DIRECTION ( 'NONE',  ( 0.000000000000000000, 1.000000000000000000, 0.000000000000000000 ) ) ;
#22199=CARTESIAN_POINT ( 'NONE',  ( 3.500000000000000000, 15.47927405783633326, -113.2380641367107614 ) ) ;
#22200=CARTESIAN_POINT ( 'NONE',  ( -3.500000000000002220, 15.47927405783633503, -120.5713974700440900 ) ) ;
#22201=CARTESIAN_POINT ( 'NONE',  ( -1.750000000000002220, 14.46891108675447590, -32.79431413575484555 ) ) ;
#22202=CARTESIAN_POINT ( 'NONE',  ( -1.750000000000002220, 14.46891108675447946, -65.79431413575484555 ) ) ;
#22203=CARTESIAN_POINT ( 'NONE',  ( -3.500000000000001332, 17.50000000000001421, -64.65473080337743284 ) ) ;
#22204=CARTESIAN_POINT ( 'NONE',  ( 0.9378221735089290467, 21.00000000000002842, -142.2556390011600342 ) ) ;
#22206=CARTESIAN_POINT ( 'NONE',  ( -1.749999999999999778, 20.53108891324556140, -138.1276474690881741 ) ) ;
#22207=CARTESIAN_POINT ( 'NONE',  ( 4.648177544792955347E-16, 21.00000000000001421, -73.21098080242151696 ) ) ;
#22208=CARTESIAN_POINT ( 'NONE',  ( 3.310556943750001313, 17.50000000000002132, -124.2641058028994649 ) ) ;
#22212=CARTESIAN_POINT ( 'NONE',  ( 0.000000000000000000, 21.00000000000002487, -149.5231586289125687 ) ) ;
#22213=CARTESIAN_POINT ( 'NONE',  ( -1.750000000000002220, 14.46891108675448301, -93.79431413575484555 ) ) ;
#22214=CARTESIAN_POINT ( 'NONE',  ( 3.310556943750001313, 19.41135094264166838, -115.2682724695661278 ) ) ;
#22215=EDGE_CURVE ( 'NONE', #40707, #3516, #39384, .T. ) ;
#22217=CARTESIAN_POINT ( 'NONE',  ( -1.750000000000002220, 14.46891108675447590, -30.48806413671076143 ) ) ;
#22218=CARTESIAN_POINT ( 'NONE',  ( -0.9378221735088960731, 14.00000000000000000, -108.7556390011600200 ) ) ;
#22220=CARTESIAN_POINT ( 'NONE',  ( -3.310556943750001313, 17.50000000000002487, -138.8516058028994564 ) ) ;
#22222=CARTESIAN_POINT ( 'NONE',  ( -3.500000000000002220, 15.47927405783632082, -29.57139747004410069 ) ) ;
#22223=CARTESIAN_POINT ( 'NONE',  ( -1.655278471875002211, 14.63297358603754184, -48.68493913623279923 ) ) ;
#22225=CARTESIAN_POINT ( 'NONE',  ( 2.340729813953370519E-16, 21.32270188528330834, -69.10160580289947063 ) ) ;
#22227=CARTESIAN_POINT ( 'NONE',  ( -1.655278471875002211, 14.63297358603754539, -68.59743913623280775 ) ) ;
#22229=CARTESIAN_POINT ( 'NONE',  ( -1.655278471874999990, 20.36702641396249192, -92.01827246956611361 ) ) ;
#22232=CARTESIAN_POINT ( 'NONE',  ( -0.9378221735089291577, 21.00000000000002132, -106.1663226036829855 ) ) ;
#22233=CARTESIAN_POINT ( 'NONE',  ( -1.394453263437886604E-15, 14.00000000000001066, -41.71098080242150274 ) ) ;
#22234=CARTESIAN_POINT ( 'NONE',  ( 2.340729813953370519E-16, 21.32270188528331190, -49.01410580289947205 ) ) ;
#22236=CARTESIAN_POINT ( 'NONE',  ( -7.022189441860112050E-16, 13.67729811471672541, -105.5141058028994649 ) ) ;
#22242=CARTESIAN_POINT ( 'NONE',  ( 3.310556943749999981, 15.58864905735836537, -56.34743913623280065 ) ) ;
#22243=ORIENTED_EDGE ( 'NONE', *, *, #18387, .F. ) ;
#22244=VERTEX_POINT ( 'NONE', #1447 ) ;
#22249=DIRECTION ( 'NONE',  ( -0.000000000000000000, 1.259100132267607459E-16, -1.000000000000000000 ) ) ;
#22251=( BOUNDED_CURVE ( )  B_SPLINE_CURVE ( 2, ( #12669, #35630, #38187, #9051, #22027, #35001, #5864, #29223, #35417 ),
 .UNSPECIFIED., .F., .F. ) 
 B_SPLINE_CURVE_WITH_KNOTS ( ( 3, 2, 2, 2, 3 ),
 ( 0.09791666666666666574, 0.09861111111111110772, 0.1000000000000000056, 0.1013888888888888895, 0.1020833333333333315 ),
 .UNSPECIFIED. ) 
 CURVE ( )  GEOMETRIC_REPRESENTATION_ITEM ( )  RATIONAL_B_SPLINE_CURVE ( ( 0.9330127018922194093, 0.9330127018922194093, 1.000000000000000000, 0.8660254037844387076, 1.000000000000000000, 0.8660254037844387076, 1.000000000000000000, 0.9330127018922194093, 0.9330127018922194093 ) ) 
 REPRESENTATION_ITEM ( '' )  );
#22252=DIRECTION ( 'NONE',  ( -0.000000000000000000, 1.259100132267607459E-16, -1.000000000000000000 ) ) ;
#22253=CARTESIAN_POINT ( 'NONE',  ( -3.310556943750000425, 19.41135094264166838, -124.8474391362328078 ) ) ;
#22256=CARTESIAN_POINT ( 'NONE',  ( -3.310556943750002645, 15.58864905735836537, -36.76827246956612782 ) ) ;
#22257=CARTESIAN_POINT ( 'NONE',  ( 2.340729813953370519E-16, 21.32270188528330479, -26.10160580289947063 ) ) ;
#22258=CARTESIAN_POINT ( 'NONE',  ( -3.310556943750002645, 15.58864905735837247, -88.76827246956612782 ) ) ;
#22259=CARTESIAN_POINT ( 'NONE',  ( -1.655278471875002211, 14.63297358603755427, -137.5974391362328220 ) ) ;
#22262=CARTESIAN_POINT ( 'NONE',  ( -1.655278471875002211, 14.63297358603755249, -132.6849391362327992 ) ) ;
#22263=CARTESIAN_POINT ( 'NONE',  ( 0.9378221735089300459, 21.00000000000001421, -56.25563900116002714 ) ) ;
#22265=FACE_OUTER_BOUND ( 'NONE', #4963, .T. ) ;
#22267=CARTESIAN_POINT ( 'NONE',  ( 3.500000000000001776, 19.52072594216371115, -82.07139747004410424 ) ) ;
#22268=CARTESIAN_POINT ( 'NONE',  ( 3.310556943749999981, 15.58864905735836537, -66.43493913623279923 ) ) ;
#22270=DIRECTION ( 'NONE',  ( -0.000000000000000000, 1.259100132267607459E-16, -1.000000000000000000 ) ) ;
#22271=LINE ( 'NONE', #31840, #36972 ) ;
#22272=CARTESIAN_POINT ( 'NONE',  ( -3.310556943750002645, 15.58864905735837247, -87.76827246956614204 ) ) ;
#22273=CARTESIAN_POINT ( 'NONE',  ( -0.9378221735089291577, 21.00000000000002132, -116.8600726046389155 ) ) ;
#22274=CARTESIAN_POINT ( 'NONE',  ( 3.310556943750001313, 19.41135094264166838, -116.1807724695661364 ) ) ;
#22275=CARTESIAN_POINT ( 'NONE',  ( 1.750000000000001110, 20.53108891324554719, -34.29431413575484555 ) ) ;
#22278=ORIENTED_EDGE ( 'NONE', *, *, #34250, .F. ) ;
#22279=CARTESIAN_POINT ( 'NONE',  ( -1.750000000000002220, 14.46891108675448478, -107.4880641367107614 ) ) ;
#22281=EDGE_CURVE ( 'NONE', #29219, #6503, #1638, .T. ) ;
#22283=CARTESIAN_POINT ( 'NONE',  ( 4.648177544792955347E-16, 21.00000000000001776, -75.90473080337740441 ) ) ;
#22284=CARTESIAN_POINT ( 'NONE',  ( 0.000000000000000000, 17.50000000000002487, -149.5231586289125687 ) ) ;
#22287=CARTESIAN_POINT ( 'NONE',  ( 2.340729813953370519E-16, 21.32270188528331190, -66.01410580289947916 ) ) ;
#22288=CARTESIAN_POINT ( 'NONE',  ( 4.648177544792955347E-16, 21.00000000000002487, -135.9047308033774186 ) ) ;
#22289=CARTESIAN_POINT ( 'NONE',  ( -3.310556943750001313, 17.50000000000002132, -119.7641058028994792 ) ) ;
#22292=ORIENTED_EDGE ( 'NONE', *, *, #36386, .F. ) ;
#22293=CARTESIAN_POINT ( 'NONE',  ( -1.394453263437886604E-15, 14.00000000000001776, -99.71098080242150274 ) ) ;
#22295=CARTESIAN_POINT ( 'NONE',  ( 1.655278471875001101, 20.36702641396249192, -77.09743913623280775 ) ) ;
#22297=ORIENTED_EDGE ( 'NONE', *, *, #31887, .F. ) ;
#22298=CARTESIAN_POINT ( 'NONE',  ( -3.500000000000001332, 17.50000000000001421, -53.65473080337743284 ) ) ;
#22300=CARTESIAN_POINT ( 'NONE',  ( -1.655278471874999990, 20.36702641396249902, -141.9307724695661364 ) ) ;
#22303=CARTESIAN_POINT ( 'NONE',  ( -3.310556943750002645, 15.58864905735836714, -43.76827246956612782 ) ) ;
#22304=CARTESIAN_POINT ( 'NONE',  ( 2.340729813953370519E-16, 21.32270188528331900, -105.1016058028994564 ) ) ;
#22307=CARTESIAN_POINT ( 'NONE',  ( 1.655278471874998436, 14.63297358603753828, -28.43077246956614346 ) ) ;
#22308=CARTESIAN_POINT ( 'NONE',  ( -1.655278471874999990, 20.36702641396248836, -63.01827246956613493 ) ) ;
#22309=CARTESIAN_POINT ( 'NONE',  ( -3.500000000000000888, 19.52072594216371826, -109.0443141357548313 ) ) ;
#22311=CARTESIAN_POINT ( 'NONE',  ( -2.324088772396477673E-16, 14.00000000000002309, -142.4047308033774186 ) ) ;
#22312=CARTESIAN_POINT ( 'NONE',  ( 1.749999999999998224, 14.46891108675448301, -98.32139747004409003 ) ) ;
#22316=CARTESIAN_POINT ( 'NONE',  ( -1.750000000000002220, 14.46891108675447946, -57.79431413575483845 ) ) ;
#22318=CARTESIAN_POINT ( 'NONE',  ( 3.310556943749999981, 15.58864905735836182, -27.34743913623280420 ) ) ;
#22319=CARTESIAN_POINT ( 'NONE',  ( -3.500000000000002220, 15.47927405783632260, -50.57139747004409003 ) ) ;
#22321=EDGE_CURVE ( 'NONE', #15451, #21056, #7346, .T. ) ;
#22322=CARTESIAN_POINT ( 'NONE',  ( -1.655278471875002211, 14.63297358603754006, -33.68493913623279923 ) ) ;
#22325=CARTESIAN_POINT ( 'NONE',  ( -3.500000000000000000, 19.52072594216371826, -142.0443141357548313 ) ) ;
#22327=LINE ( 'NONE', #38918, #29425 ) ;
#22329=CARTESIAN_POINT ( 'NONE',  ( -1.655278471874999990, 20.36702641396249192, -79.93077246956615056 ) ) ;
#22337=CARTESIAN_POINT ( 'NONE',  ( 2.340729813953370519E-16, 21.32270188528331190, -96.01410580289946495 ) ) ;
#22339=ORIENTED_EDGE ( 'NONE', *, *, #27776, .F. ) ;
#22340=CARTESIAN_POINT ( 'NONE',  ( 3.500000000000001332, 19.52072594216371826, -121.0713974700441184 ) ) ;
#22341=ORIENTED_EDGE ( 'NONE', *, *, #37130, .F. ) ;
#22343=CARTESIAN_POINT ( 'NONE',  ( -1.749999999999999778, 20.53108891324555429, -84.82139747004409003 ) ) ;
#22346=ORIENTED_EDGE ( 'NONE', *, *, #39638, .T. ) ;
#22347=DIRECTION ( 'NONE',  ( -0.000000000000000000, 1.259100132267607459E-16, -1.000000000000000000 ) ) ;
#22349=CARTESIAN_POINT ( 'NONE',  ( 3.310556943749999981, 15.58864905735837425, -132.3474391362328220 ) ) ;
#22351=ORIENTED_EDGE ( 'NONE', *, *, #38867, .F. ) ;
#22352=CARTESIAN_POINT ( 'NONE',  ( -0.9378221735089288247, 14.00000000000002309, -140.7556390011600342 ) ) ;
#22353=CARTESIAN_POINT ( 'NONE',  ( 3.310556943750001313, 17.50000000000002132, -125.3516058028994706 ) ) ;
#22354=CARTESIAN_POINT ( 'NONE',  ( 3.310556943749999981, 15.58864905735836182, -50.43493913623279923 ) ) ;
#22356=CARTESIAN_POINT ( 'NONE',  ( 3.500000000000001332, 17.50000000000002487, -133.1547308033774186 ) ) ;
#22358=CARTESIAN_POINT ( 'NONE',  ( 2.340729813953370519E-16, 21.32270188528331190, -79.10160580289945642 ) ) ;
#22359=CARTESIAN_POINT ( 'NONE',  ( 3.500000000000000000, 15.47927405783633503, -123.5443141357548456 ) ) ;
#22360=CARTESIAN_POINT ( 'NONE',  ( -3.310556943750002645, 15.58864905735837425, -106.6807724695661506 ) ) ;
#22361=( BOUNDED_CURVE ( )  B_SPLINE_CURVE ( 2, ( #8211, #24387, #36729, #21184, #34159, #30976, #1832, #14811, #11603 ),
 .UNSPECIFIED., .F., .T. ) 
 B_SPLINE_CURVE_WITH_KNOTS ( ( 3, 2, 2, 2, 3 ),
 ( 0.9187499999999999556, 0.9194444444444443976, 0.9208333333333332815, 0.9222222222222222765, 0.9229166666666667185 ),
 .UNSPECIFIED. ) 
 CURVE ( )  GEOMETRIC_REPRESENTATION_ITEM ( )  RATIONAL_B_SPLINE_CURVE ( ( 0.9330127018922194093, 0.9330127018922194093, 1.000000000000000000, 0.8660254037844387076, 1.000000000000000000, 0.8660254037844387076, 1.000000000000000000, 0.9330127018922194093, 0.9330127018922194093 ) ) 
 REPRESENTATION_ITEM ( '' )  );
#22362=CARTESIAN_POINT ( 'NONE',  ( 3.500000000000001332, 17.50000000000001776, -93.15473080337743284 ) ) ;
#22365=CARTESIAN_POINT ( 'NONE',  ( -1.749999999999999778, 20.53108891324555074, -73.12764746908817415 ) ) ;
#22368=CARTESIAN_POINT ( 'NONE',  ( 1.655278471874998436, 14.63297358603754006, -45.43077246956614346 ) ) ;
#22369=CARTESIAN_POINT ( 'NONE',  ( -3.310556943750001313, 17.50000000000002132, -103.8516058028994564 ) ) ;
#22370=CARTESIAN_POINT ( 'NONE',  ( -1.394453263437886604E-15, 14.00000000000001421, -73.71098080242150274 ) ) ;
#22371=CARTESIAN_POINT ( 'NONE',  ( 3.500000000000000000, 15.47927405783632260, -64.23806413671076143 ) ) ;
#22373=ORIENTED_EDGE ( 'NONE', *, *, #13497, .T. ) ;
#22374=CARTESIAN_POINT ( 'NONE',  ( -3.310556943750000425, 19.41135094264166838, -117.9349391362327850 ) ) ;
#22375=CARTESIAN_POINT ( 'NONE',  ( 7.785697387528201340E-15, 14.00000000000002487, -136.4047308033774186 ) ) ;
#22382=VERTEX_POINT ( 'NONE', #31618 ) ;
#22383=CARTESIAN_POINT ( 'NONE',  ( 4.648177544792955347E-16, 21.00000000000001066, -29.21098080242150630 ) ) ;
#22385=CARTESIAN_POINT ( 'NONE',  ( 3.500000000000001332, 19.52072594216370760, -48.07139747004410424 ) ) ;
#22386=DIRECTION ( 'NONE',  ( -0.000000000000000000, 1.259100132267607459E-16, -1.000000000000000000 ) ) ;
#22391=CARTESIAN_POINT ( 'NONE',  ( -1.655278471874999990, 20.36702641396248481, -34.93077246956615056 ) ) ;
#22396=CARTESIAN_POINT ( 'NONE',  ( -1.750000000000002220, 14.46891108675448478, -99.79431413575484555 ) ) ;
#22403=CARTESIAN_POINT ( 'NONE',  ( -3.500000000000001332, 17.50000000000002132, -118.6547308033774328 ) ) ;
#22405=CARTESIAN_POINT ( 'NONE',  ( -3.500000000000001332, 17.50000000000001066, -32.96098080242150274 ) ) ;
#22406=CARTESIAN_POINT ( 'NONE',  ( 0.9378221735089281585, 14.00000000000000888, -35.66632260368298546 ) ) ;
#22411=CARTESIAN_POINT ( 'NONE',  ( -3.500000000000001332, 17.50000000000002487, -137.9609808024214885 ) ) ;
#22413=CARTESIAN_POINT ( 'NONE',  ( 1.655278471874998436, 14.63297358603755072, -125.4307724695661364 ) ) ;
#22417=CARTESIAN_POINT ( 'NONE',  ( -3.500000000000001332, 17.50000000000001776, -90.96098080242151696 ) ) ;
#22418=( BOUNDED_CURVE ( )  B_SPLINE_CURVE ( 2, ( #12073, #35257, #5707, #12721, #2510, #38029, #8893, #38873, #6333 ),
 .UNSPECIFIED., .F., .T. ) 
 B_SPLINE_CURVE_WITH_KNOTS ( ( 3, 2, 2, 2, 3 ),
 ( 0.6979166666666666297, 0.6986111111111110716, 0.6999999999999999556, 0.7013888888888888395, 0.7020833333333332815 ),
 .UNSPECIFIED. ) 
 CURVE ( )  GEOMETRIC_REPRESENTATION_ITEM ( )  RATIONAL_B_SPLINE_CURVE ( ( 0.9330127018922194093, 0.9330127018922194093, 1.000000000000000000, 0.8660254037844387076, 1.000000000000000000, 0.8660254037844387076, 1.000000000000000000, 0.9330127018922194093, 0.9330127018922194093 ) ) 
 REPRESENTATION_ITEM ( '' )  );
#22419=CARTESIAN_POINT ( 'NONE',  ( 0.9378221735089300459, 21.00000000000001066, -32.94938900211595012 ) ) ;
#22420=CARTESIAN_POINT ( 'NONE',  ( 1.655278471875001101, 20.36702641396248836, -60.09743913623280775 ) ) ;
#22421=CARTESIAN_POINT ( 'NONE',  ( -7.022189441860112050E-16, 13.67729811471672718, -118.6016058028994706 ) ) ;
#22422=CARTESIAN_POINT ( 'NONE',  ( -1.749999999999999778, 20.53108891324555785, -122.1276474690881741 ) ) ;
#22423=CARTESIAN_POINT ( 'NONE',  ( 1.750000000000001110, 20.53108891324554719, -31.98806413671076498 ) ) ;
#22426=CARTESIAN_POINT ( 'NONE',  ( 3.310556943749999981, 15.58864905735837425, -136.4349391362327992 ) ) ;
#22429=CARTESIAN_POINT ( 'NONE',  ( 2.340729813953370519E-16, 21.32270188528330834, -45.10160580289947063 ) ) ;
#22430=CARTESIAN_POINT ( 'NONE',  ( 0.000000000000000000, 21.00000000000002487, -149.5231586289125687 ) ) ;
#22431=CARTESIAN_POINT ( 'NONE',  ( -3.310556943750002645, 15.58864905735837070, -67.76827246956612782 ) ) ;
#22433=CARTESIAN_POINT ( 'NONE',  ( -3.310556943750000425, 19.41135094264166128, -62.84743913623280775 ) ) ;
#22434=ORIENTED_EDGE ( 'NONE', *, *, #20192, .T. ) ;
#22435=CARTESIAN_POINT ( 'NONE',  ( -3.310556943750001313, 17.50000000000001776, -92.85160580289947063 ) ) ;
#22437=CARTESIAN_POINT ( 'NONE',  ( -1.750000000000002220, 14.46891108675448478, -107.7943141357548456 ) ) ;
#22438=CARTESIAN_POINT ( 'NONE',  ( -0.9378221735089310451, 14.00000000000002132, -105.7556390011600342 ) ) ;
#22439=DIRECTION ( 'NONE',  ( 0.000000000000000000, 1.000000000000000000, 0.000000000000000000 ) ) ;
#22440=CARTESIAN_POINT ( 'NONE',  ( -1.655278471875002211, 14.63297358603754184, -48.59743913623280775 ) ) ;
#22442=CARTESIAN_POINT ( 'NONE',  ( 2.340729813953370519E-16, 21.32270188528331900, -108.0141058028994649 ) ) ;
#22444=ORIENTED_EDGE ( 'NONE', *, *, #40725, .F. ) ;
#22448=CARTESIAN_POINT ( 'NONE',  ( -3.310556943750002645, 15.58864905735836892, -57.68077246956614346 ) ) ;
#22451=EDGE_CURVE ( 'NONE', #5598, #7495, #36419, .T. ) ;
#22458=CARTESIAN_POINT ( 'NONE',  ( -3.310556943750001313, 17.50000000000002132, -126.7641058028994792 ) ) ;
#22459=AXIS2_PLACEMENT_3D ( 'NONE', #15118, #15335, #5538 ) ;
#22461=CARTESIAN_POINT ( 'NONE',  ( 3.310556943749999981, 15.58864905735836182, -34.43493913623279923 ) ) ;
#22462=CARTESIAN_POINT ( 'NONE',  ( -1.655278471874999990, 20.36702641396248481, -26.01827246956613138 ) ) ;
#22463=CARTESIAN_POINT ( 'NONE',  ( -1.655278471875002211, 14.63297358603754716, -88.68493913623279923 ) ) ;
#22464=CARTESIAN_POINT ( 'NONE',  ( -3.310556943750000425, 19.41135094264167549, -136.8474391362328220 ) ) ;
#22466=CARTESIAN_POINT ( 'NONE',  ( 0.9378221735089300459, 21.00000000000001421, -48.94938900211595012 ) ) ;
#22468=CARTESIAN_POINT ( 'NONE',  ( 1.655278471874998436, 14.63297358603755072, -135.5182724695661420 ) ) ;
#22471=CARTESIAN_POINT ( 'NONE',  ( -3.500000000000002220, 15.47927405783632793, -75.87764746908817415 ) ) ;
#22472=CARTESIAN_POINT ( 'NONE',  ( 4.648177544792955347E-16, 21.00000000000001421, -55.21098080242150274 ) ) ;
#22473=CARTESIAN_POINT ( 'NONE',  ( -7.424026671074350129E-16, 13.45854811567263454, -80.40473080337741862 ) ) ;
#22475=CARTESIAN_POINT ( 'NONE',  ( -1.655278471875002211, 14.63297358603754361, -65.68493913623279923 ) ) ;
#22479=CARTESIAN_POINT ( 'NONE',  ( 1.655278471874998436, 14.63297358603754539, -83.51827246956614204 ) ) ;
#22481=CARTESIAN_POINT ( 'NONE',  ( -3.310556943750002201, 15.58864905735837780, -116.6807724695661364 ) ) ;
#22482=CARTESIAN_POINT ( 'NONE',  ( 1.655278471875001101, 20.36702641396249192, -82.09743913623279354 ) ) ;
#22483=CARTESIAN_POINT ( 'NONE',  ( 0.000000000000000000, 17.50000000000002487, -149.5231586289125687 ) ) ;
#22484=ORIENTED_EDGE ( 'NONE', *, *, #37416, .T. ) ;
#22485=EDGE_CURVE ( 'NONE', #2263, #16185, #5478, .T. ) ;
#22486=CARTESIAN_POINT ( 'NONE',  ( 3.500000000000000000, 15.47927405783632793, -108.2380641367107614 ) ) ;
#22493=CARTESIAN_POINT ( 'NONE',  ( -3.310556943750002201, 15.58864905735836892, -66.68077246956613635 ) ) ;
#22495=CARTESIAN_POINT ( 'NONE',  ( 1.655278471874998436, 14.63297358603754894, -122.4307724695661364 ) ) ;
#22499=EDGE_LOOP ( 'NONE', ( #35530, #11666, #28671, #27056 ) ) ;
#22500=CARTESIAN_POINT ( 'NONE',  ( -3.500000000000000000, 19.52072594216370405, -43.04431413575483134 ) ) ;
#22501=CARTESIAN_POINT ( 'NONE',  ( -3.500000000000000000, 19.52072594216370405, -32.04431413575484555 ) ) ;
#22502=CARTESIAN_POINT ( 'NONE',  ( 3.310556943750001313, 17.50000000000001421, -74.26410580289947916 ) ) ;
#22503=ORIENTED_EDGE ( 'NONE', *, *, #33970, .F. ) ;
#22504=ORIENTED_EDGE ( 'NONE', *, *, #14424, .F. ) ;
#22505=VECTOR ( 'NONE', #31573, 1000.000000000000000 ) ;
#22507=EDGE_CURVE ( 'NONE', #37791, #12093, #12897, .T. ) ;
#22508=CARTESIAN_POINT ( 'NONE',  ( -3.310556943750001313, 17.50000000000002487, -139.7641058028994792 ) ) ;
#22511=CARTESIAN_POINT ( 'NONE',  ( 1.655278471875001101, 20.36702641396248481, -42.18493913623279212 ) ) ;
#22512=CARTESIAN_POINT ( 'NONE',  ( 1.655278471875001101, 20.36702641396249547, -104.1849391362328134 ) ) ;
#22513=CARTESIAN_POINT ( 'NONE',  ( 3.310556943749999981, 15.58864905735836182, -27.34743913623280420 ) ) ;
#22515=CARTESIAN_POINT ( 'NONE',  ( 3.500000000000001776, 19.52072594216371826, -109.3776474690881741 ) ) ;
#22518=CARTESIAN_POINT ( 'NONE',  ( -1.750000000000002220, 14.46891108675448301, -94.48806413671076143 ) ) ;
#22519=EDGE_CURVE ( 'NONE', #3992, #41237, #39043, .T. ) ;
#22520=CARTESIAN_POINT ( 'NONE',  ( 4.648177544792955347E-16, 21.00000000000002132, -116.9047308033774328 ) ) ;
#22523=CARTESIAN_POINT ( 'NONE',  ( -1.750000000000002220, 14.46891108675447946, -59.79431413575483845 ) ) ;
#22525=CARTESIAN_POINT ( 'NONE',  ( 3.310556943750001313, 19.41135094264165772, -24.18077246956613990 ) ) ;
#22527=EDGE_CURVE ( 'NONE', #14300, #2506, #16306, .T. ) ;
#22528=CARTESIAN_POINT ( 'NONE',  ( -1.750000000000002220, 14.46891108675447768, -50.48806413671076854 ) ) ;
#22530=CARTESIAN_POINT ( 'NONE',  ( -3.310556943750001313, 17.50000000000001066, -30.85160580289945997 ) ) ;
#22533=CARTESIAN_POINT ( 'NONE',  ( 0.9378221735089300459, 21.00000000000001421, -49.94938900211594301 ) ) ;
#22535=FACE_OUTER_BOUND ( 'NONE', #36737, .T. ) ;
#22537=CARTESIAN_POINT ( 'NONE',  ( 3.310556943750001313, 19.41135094264166838, -81.18077246956615056 ) ) ;
#22542=( BOUNDED_CURVE ( )  B_SPLINE_CURVE ( 2, ( #34160, #24191, #36730, #33543, #27580, #40547, #11403, #14184, #36949 ),
 .UNSPECIFIED., .F., .F. ) 
 B_SPLINE_CURVE_WITH_KNOTS ( ( 3, 2, 2, 2, 3 ),
 ( 0.7604166666666666297, 0.7611111111111110716, 0.7624999999999999556, 0.7638888888888888395, 0.7645833333333332815 ),
 .UNSPECIFIED. ) 
 CURVE ( )  GEOMETRIC_REPRESENTATION_ITEM ( )  RATIONAL_B_SPLINE_CURVE ( ( 0.9330127018922194093, 0.9330127018922194093, 1.000000000000000000, 0.8660254037844387076, 1.000000000000000000, 0.8660254037844387076, 1.000000000000000000, 0.9330127018922194093, 0.9330127018922194093 ) ) 
 REPRESENTATION_ITEM ( '' )  );
#22546=CARTESIAN_POINT ( 'NONE',  ( 1.655278471875001101, 20.36702641396249192, -88.09743913623280775 ) ) ;
#22548=VERTEX_POINT ( 'NONE', #29676 ) ;
#22549=FACE_OUTER_BOUND ( 'NONE', #20302, .T. ) ;
#22550=ORIENTED_EDGE ( 'NONE', *, *, #30462, .F. ) ;
#22551=( BOUNDED_CURVE ( )  B_SPLINE_CURVE ( 2, ( #36996, #34206, #18046, #31021, #1874, #8055, #7858, #20829, #26997 ),
 .UNSPECIFIED., .F., .T. ) 
 B_SPLINE_CURVE_WITH_KNOTS ( ( 3, 2, 2, 2, 3 ),
 ( 0.3979166666666666963, 0.3986111111111111382, 0.4000000000000000222, 0.4013888888888889062, 0.4020833333333333481 ),
 .UNSPECIFIED. ) 
 CURVE ( )  GEOMETRIC_REPRESENTATION_ITEM ( )  RATIONAL_B_SPLINE_CURVE ( ( 0.9330127018922194093, 0.9330127018922220739, 1.000000000000000000, 0.8660254037844387076, 1.000000000000000000, 0.8660254037844387076, 1.000000000000000000, 0.9330127018922194093, 0.9330127018922194093 ) ) 
 REPRESENTATION_ITEM ( '' )  );
#22554=FACE_OUTER_BOUND ( 'NONE', #9623, .T. ) ;
#22557=CARTESIAN_POINT ( 'NONE',  ( -3.500000000000000000, 19.52072594216371115, -88.73806413671076143 ) ) ;
#22559=CARTESIAN_POINT ( 'NONE',  ( 1.743066579297357930E-14, 14.00000000000002132, -129.7109808024214885 ) ) ;
#22560=EDGE_CURVE ( 'NONE', #18376, #35046, #2743, .T. ) ;
#22561=CARTESIAN_POINT ( 'NONE',  ( -3.310556943750002645, 15.58864905735837780, -129.6807724695661364 ) ) ;
#22564=CARTESIAN_POINT ( 'NONE',  ( -3.500000000000001332, 17.50000000000002487, -140.9609808024215170 ) ) ;
#22565=CARTESIAN_POINT ( 'NONE',  ( 2.340729813953370519E-16, 21.32270188528331900, -122.1016058028994564 ) ) ;
#22566=CARTESIAN_POINT ( 'NONE',  ( 3.310556943750001313, 17.50000000000001421, -51.35160580289946353 ) ) ;
#22567=ORIENTED_EDGE ( 'NONE', *, *, #38564, .T. ) ;
#22568=CARTESIAN_POINT ( 'NONE',  ( 2.474675557024783212E-16, 21.54145188432740810, -131.9047308033774186 ) ) ;
#22571=CARTESIAN_POINT ( 'NONE',  ( -1.655278471874999990, 20.36702641396248836, -74.01827246956612782 ) ) ;
#22572=CARTESIAN_POINT ( 'NONE',  ( -3.500000000000000888, 19.52072594216371826, -124.0443141357548456 ) ) ;
#22573=CARTESIAN_POINT ( 'NONE',  ( 3.310556943750001313, 17.50000000000002132, -106.2641058028994649 ) ) ;
#22574=EDGE_CURVE ( 'NONE', #41382, #26918, #14435, .T. ) ;
#22577=CARTESIAN_POINT ( 'NONE',  ( -1.394453263437886604E-15, 14.00000000000001421, -72.40473080337743284 ) ) ;
#22580=CARTESIAN_POINT ( 'NONE',  ( 1.750000000000001110, 20.53108891324555429, -77.29431413575484555 ) ) ;
#22581=CARTESIAN_POINT ( 'NONE',  ( -1.394453263437886604E-15, 14.00000000000001066, -50.71098080242150274 ) ) ;
#22582=CARTESIAN_POINT ( 'NONE',  ( 1.655278471875001101, 20.36702641396248481, -43.09743913623280065 ) ) ;
#22583=CARTESIAN_POINT ( 'NONE',  ( -7.022189441860112050E-16, 13.67729811471672541, -103.6016058028994564 ) ) ;
#22584=CARTESIAN_POINT ( 'NONE',  ( 4.648177544792955347E-16, 21.00000000000002132, -114.2109808024214885 ) ) ;
#22585=CARTESIAN_POINT ( 'NONE',  ( 1.750000000000001110, 20.53108891324555074, -64.98806413671076143 ) ) ;
#22587=ORIENTED_EDGE ( 'NONE', *, *, #5303, .T. ) ;
#22588=CARTESIAN_POINT ( 'NONE',  ( 3.310556943750001313, 17.50000000000002132, -120.3516058028994706 ) ) ;
#22592=CARTESIAN_POINT ( 'NONE',  ( 4.286263797015737581E-16, 14.00000000000002487, -149.5231586289125687 ) ) ;
#22593=CARTESIAN_POINT ( 'NONE',  ( 3.310556943749999981, 15.58864905735837070, -100.3474391362328078 ) ) ;
#22594=CARTESIAN_POINT ( 'NONE',  ( -0.9378221735089310451, 14.00000000000001066, -52.44938900211594301 ) ) ;
#22596=EDGE_LOOP ( 'NONE', ( #35014, #2928, #30358, #20683 ) ) ;
#22599=CARTESIAN_POINT ( 'NONE',  ( -1.749999999999999778, 20.53108891324555785, -112.8213974700440900 ) ) ;
#22603=CARTESIAN_POINT ( 'NONE',  ( 1.655278471875001101, 20.36702641396248481, -35.09743913623280775 ) ) ;
#22611=VERTEX_POINT ( 'NONE', #19484 ) ;
#22612=CARTESIAN_POINT ( 'NONE',  ( 0.000000000000000000, 21.00000000000002487, -149.5231586289125687 ) ) ;
#22613=LINE ( 'NONE', #3053, #18031 ) ;
#22615=CARTESIAN_POINT ( 'NONE',  ( -3.500000000000001332, 17.50000000000002132, -116.6547308033774328 ) ) ;
#22616=CARTESIAN_POINT ( 'NONE',  ( -0.9378221735089310451, 14.00000000000001066, -33.75563900116002714 ) ) ;
#22617=CARTESIAN_POINT ( 'NONE',  ( -3.310556943750000425, 19.41135094264167549, -135.9349391362327992 ) ) ;
#22618=CARTESIAN_POINT ( 'NONE',  ( 2.474675557024783212E-16, 21.54145188432739033, -34.21098080242150274 ) ) ;
#22619=( BOUNDED_CURVE ( )  B_SPLINE_CURVE ( 2, ( #7709, #1328, #27066, #14722, #27485, #37470, #21095, #30879, #33662 ),
 .UNSPECIFIED., .F., .F. ) 
 B_SPLINE_CURVE_WITH_KNOTS ( ( 3, 2, 2, 2, 3 ),
 ( 0.5062499999999999778, 0.5069444444444444198, 0.5083333333333333037, 0.5097222222222221877, 0.5104166666666666297 ),
 .UNSPECIFIED. ) 
 CURVE ( )  GEOMETRIC_REPRESENTATION_ITEM ( )  RATIONAL_B_SPLINE_CURVE ( ( 0.9330127018922194093, 0.9330127018922194093, 1.000000000000000000, 0.8660254037844387076, 1.000000000000000000, 0.8660254037844387076, 1.000000000000000000, 0.9330127018922194093, 0.9330127018922194093 ) ) 
 REPRESENTATION_ITEM ( '' )  );
#22622=CARTESIAN_POINT ( 'NONE',  ( 0.9378221735089281585, 14.00000000000000888, -32.66632260368299256 ) ) ;
#22623=CARTESIAN_POINT ( 'NONE',  ( 0.9378221735089281585, 14.00000000000002132, -106.3600726046389013 ) ) ;
#22625=CARTESIAN_POINT ( 'NONE',  ( 1.749999999999998224, 14.46891108675448834, -140.6276474690881741 ) ) ;
#22628=CARTESIAN_POINT ( 'NONE',  ( 3.310556943750001313, 17.50000000000002132, -125.2641058028994792 ) ) ;
#22632=CARTESIAN_POINT ( 'NONE',  ( 0.9378221735089300459, 21.00000000000001066, -28.94938900211595367 ) ) ;
#22633=CARTESIAN_POINT ( 'NONE',  ( -7.424026671074350129E-16, 13.45854811567263631, -91.71098080242153117 ) ) ;
#22635=CARTESIAN_POINT ( 'NONE',  ( 3.310556943750001313, 19.41135094264166128, -60.18077246956613635 ) ) ;
#22636=CARTESIAN_POINT ( 'NONE',  ( -3.310556943750001313, 17.50000000000002132, -119.8516058028994706 ) ) ;
#22637=FACE_OUTER_BOUND ( 'NONE', #32958, .T. ) ;
#22638=CARTESIAN_POINT ( 'NONE',  ( 3.500000000000001332, 17.50000000000001066, -31.15473080337742573 ) ) ;
#22639=CARTESIAN_POINT ( 'NONE',  ( -1.750000000000002220, 14.46891108675448478, -108.7943141357548456 ) ) ;
#22641=CARTESIAN_POINT ( 'NONE',  ( -3.310556943750002201, 15.58864905735837780, -135.7682724695661420 ) ) ;
#22643=CARTESIAN_POINT ( 'NONE',  ( 4.648177544792955347E-16, 21.00000000000001776, -79.90473080337741862 ) ) ;
#22644=CARTESIAN_POINT ( 'NONE',  ( 1.655278471875001101, 20.36702641396248481, -44.18493913623279212 ) ) ;
#22647=CARTESIAN_POINT ( 'NONE',  ( -3.310556943750002645, 15.58864905735836892, -66.76827246956612782 ) ) ;
#22649=CARTESIAN_POINT ( 'NONE',  ( 2.340729813953370519E-16, 21.32270188528330834, -67.01410580289947916 ) ) ;
#22650=ORIENTED_EDGE ( 'NONE', *, *, #41167, .F. ) ;
#22651=CARTESIAN_POINT ( 'NONE',  ( 3.310556943750001313, 17.50000000000001776, -85.35160580289947063 ) ) ;
#22653=DIRECTION ( 'NONE',  ( -0.000000000000000000, 1.259100132267607459E-16, -1.000000000000000000 ) ) ;
#22655=DIRECTION ( 'NONE',  ( -0.000000000000000000, 1.259100132267607459E-16, -1.000000000000000000 ) ) ;
#22656=CARTESIAN_POINT ( 'NONE',  ( -3.310556943750001313, 17.50000000000001421, -51.76410580289947205 ) ) ;
#22658=CARTESIAN_POINT ( 'NONE',  ( -7.022189441860112050E-16, 13.67729811471672541, -103.5141058028994649 ) ) ;
#22659=CARTESIAN_POINT ( 'NONE',  ( 3.500000000000001332, 17.50000000000001776, -96.15473080337743284 ) ) ;
#22660=ORIENTED_EDGE ( 'NONE', *, *, #25079, .F. ) ;
#22663=ORIENTED_EDGE ( 'NONE', *, *, #24893, .T. ) ;
#22665=CARTESIAN_POINT ( 'NONE',  ( -3.310556943750000425, 19.41135094264166128, -59.84743913623280775 ) ) ;
#22667=VERTEX_POINT ( 'NONE', #35850 ) ;
#22671=CARTESIAN_POINT ( 'NONE',  ( -1.750000000000002220, 14.46891108675449011, -140.4880641367107614 ) ) ;
#22673=CYLINDRICAL_SURFACE ( 'NONE', #14700, 3.499999999999999556 ) ;
#22674=CARTESIAN_POINT ( 'NONE',  ( -3.310556943750001313, 17.50000000000002132, -124.7641058028994649 ) ) ;
#22675=EDGE_CURVE ( 'NONE', #7014, #10678, #29080, .T. ) ;
#22676=( BOUNDED_CURVE ( )  B_SPLINE_CURVE ( 2, ( #16595, #19558, #9999, #32952, #36359, #3819, #415, #16799, #29550 ),
 .UNSPECIFIED., .F., .F. ) 
 B_SPLINE_CURVE_WITH_KNOTS ( ( 3, 2, 2, 2, 3 ),
 ( 0.01041666666666666782, 0.01111111111111111154, 0.01250000000000000069, 0.01388888888888888812, 0.01458333333333333356 ),
 .UNSPECIFIED. ) 
 CURVE ( )  GEOMETRIC_REPRESENTATION_ITEM ( )  RATIONAL_B_SPLINE_CURVE ( ( 0.9330127018922192983, 0.9330127018922194093, 1.000000000000000000, 0.8660254037844387076, 1.000000000000000000, 0.8660254037844387076, 1.000000000000000000, 0.9330127018922191873, 0.9330127018922192983 ) ) 
 REPRESENTATION_ITEM ( '' )  );
#22677=AXIS2_PLACEMENT_3D ( 'NONE', #27623, #11653, #18051 ) ;
#22679=CARTESIAN_POINT ( 'NONE',  ( -1.655278471875002211, 14.63297358603754006, -34.68493913623279923 ) ) ;
#22680=CARTESIAN_POINT ( 'NONE',  ( -3.310556943750002645, 15.58864905735836537, -28.76827246956613848 ) ) ;
#22681=CARTESIAN_POINT ( 'NONE',  ( 1.655278471874998436, 14.63297358603754539, -90.51827246956612782 ) ) ;
#22682=CARTESIAN_POINT ( 'NONE',  ( 1.655278471875001101, 20.36702641396249902, -139.0974391362327935 ) ) ;
#22685=CARTESIAN_POINT ( 'NONE',  ( -3.500000000000002220, 15.47927405783633326, -100.5713974700440900 ) ) ;
#22686=CARTESIAN_POINT ( 'NONE',  ( -1.655278471874999990, 20.36702641396249902, -133.0182724695661420 ) ) ;
#22687=DIRECTION ( 'NONE',  ( 0.000000000000000000, 1.000000000000000000, 0.000000000000000000 ) ) ;
#22688=CARTESIAN_POINT ( 'NONE',  ( -1.655278471874999990, 20.36702641396249192, -93.93077246956613635 ) ) ;
#22691=CARTESIAN_POINT ( 'NONE',  ( 0.9378221735089300459, 21.00000000000002132, -126.2556390011600485 ) ) ;
#22692=CARTESIAN_POINT ( 'NONE',  ( 2.474675557024783212E-16, 21.54145188432739744, -77.90473080337743284 ) ) ;
#22693=CARTESIAN_POINT ( 'NONE',  ( -3.310556943750000425, 19.41135094264166483, -60.93493913623279923 ) ) ;
#22697=CARTESIAN_POINT ( 'NONE',  ( 1.655278471874998436, 14.63297358603754539, -84.51827246956612782 ) ) ;
#22698=CARTESIAN_POINT ( 'NONE',  ( -1.655278471874999990, 20.36702641396249902, -143.0182724695661420 ) ) ;
#22699=CARTESIAN_POINT ( 'NONE',  ( 3.310556943750001313, 19.41135094264166838, -113.1807724695661221 ) ) ;
#22700=CARTESIAN_POINT ( 'NONE',  ( -3.310556943750002645, 15.58864905735837247, -81.68077246956616477 ) ) ;
#22703=CARTESIAN_POINT ( 'NONE',  ( 1.750000000000001110, 20.53108891324555785, -107.9880641367107614 ) ) ;
#22707=CARTESIAN_POINT ( 'NONE',  ( 3.500000000000000000, 15.47927405783632970, -105.2380641367107614 ) ) ;
#22708=CARTESIAN_POINT ( 'NONE',  ( 4.286263797015737581E-16, 14.00000000000002487, -149.5231586289125687 ) ) ;
#22711=CARTESIAN_POINT ( 'NONE',  ( -1.655278471874999990, 20.36702641396248836, -67.93077246956613635 ) ) ;
#22713=CARTESIAN_POINT ( 'NONE',  ( 3.310556943750001313, 19.41135094264166838, -120.1807724695661506 ) ) ;
#22714=CARTESIAN_POINT ( 'NONE',  ( 3.500000000000001332, 19.52072594216370760, -71.07139747004409003 ) ) ;
#22718=CARTESIAN_POINT ( 'NONE',  ( -1.394453263437886604E-15, 14.00000000000001776, -103.7109808024215027 ) ) ;
#22719=CARTESIAN_POINT ( 'NONE',  ( 3.500000000000000000, 15.47927405783632615, -79.23806413671076143 ) ) ;
#22720=CARTESIAN_POINT ( 'NONE',  ( 2.340729813953370519E-16, 21.32270188528330834, -73.01410580289947916 ) ) ;
#22722=ORIENTED_EDGE ( 'NONE', *, *, #28681, .F. ) ;
#22724=EDGE_CURVE ( 'NONE', #34588, #28207, #5729, .T. ) ;
#22725=CARTESIAN_POINT ( 'NONE',  ( 3.310556943750001313, 17.50000000000002487, -141.2641058028994792 ) ) ;
#22728=CARTESIAN_POINT ( 'NONE',  ( -1.394453263437886604E-15, 14.00000000000002132, -113.4047308033774186 ) ) ;
#22729=CARTESIAN_POINT ( 'NONE',  ( -3.310556943750000425, 19.41135094264165772, -43.93493913623279212 ) ) ;
#22730=CARTESIAN_POINT ( 'NONE',  ( 3.310556943750001313, 17.50000000000002132, -106.3516058028994564 ) ) ;
#22732=CARTESIAN_POINT ( 'NONE',  ( 3.310556943750001313, 19.41135094264165772, -31.18077246956614701 ) ) ;
#22733=VECTOR ( 'NONE', #34751, 1000.000000000000000 ) ;
#22735=CARTESIAN_POINT ( 'NONE',  ( -1.749999999999999778, 20.53108891324555785, -109.1276474690881741 ) ) ;
#22737=CARTESIAN_POINT ( 'NONE',  ( -1.750000000000002220, 14.46891108675448656, -118.7943141357548313 ) ) ;
#22738=CARTESIAN_POINT ( 'NONE',  ( 1.750000000000001110, 20.53108891324555429, -93.98806413671076143 ) ) ;
#22742=CARTESIAN_POINT ( 'NONE',  ( 1.750000000000001110, 20.53108891324555074, -61.29431413575483845 ) ) ;
#22743=CARTESIAN_POINT ( 'NONE',  ( -3.500000000000000000, 19.52072594216370760, -47.04431413575483134 ) ) ;
#22746=CARTESIAN_POINT ( 'NONE',  ( -3.500000000000000888, 19.52072594216370760, -49.73806413671076854 ) ) ;
#22747=CARTESIAN_POINT ( 'NONE',  ( 4.648177544792955347E-16, 21.00000000000001776, -75.21098080242151696 ) ) ;
#22748=CARTESIAN_POINT ( 'NONE',  ( 2.340729813953370519E-16, 21.32270188528330834, -32.10160580289946353 ) ) ;
#22755=CARTESIAN_POINT ( 'NONE',  ( -3.310556943750002201, 15.58864905735837247, -84.68077246956613635 ) ) ;
#22759=CARTESIAN_POINT ( 'NONE',  ( 4.286263797015737581E-16, 14.00000000000002487, -149.5231586289125687 ) ) ;
#22761=ORIENTED_EDGE ( 'NONE', *, *, #6640, .F. ) ;
#22763=CARTESIAN_POINT ( 'NONE',  ( 3.310556943749999981, 15.58864905735836892, -90.34743913623280775 ) ) ;
#22764=ORIENTED_EDGE ( 'NONE', *, *, #16552, .T. ) ;
#22765=EDGE_LOOP ( 'NONE', ( #28048, #40351, #9799, #22339 ) ) ;
#22768=CARTESIAN_POINT ( 'NONE',  ( 1.749999999999998224, 14.46891108675447768, -66.62764746908817415 ) ) ;
#22770=ADVANCED_FACE ( 'NONE', ( #4369 ), #4990, .T. ) ;
#22773=CARTESIAN_POINT ( 'NONE',  ( -1.394453263437886604E-15, 14.00000000000002132, -109.4047308033774186 ) ) ;
#22775=EDGE_CURVE ( 'NONE', #32548, #16409, #11678, .T. ) ;
#22776=CARTESIAN_POINT ( 'NONE',  ( 3.310556943750001313, 19.41135094264166838, -129.1807724695661364 ) ) ;
#22777=ORIENTED_EDGE ( 'NONE', *, *, #4765, .T. ) ;
#22778=ORIENTED_EDGE ( 'NONE', *, *, #29935, .T. ) ;
#22779=DIRECTION ( 'NONE',  ( 0.000000000000000000, 1.000000000000000000, 0.000000000000000000 ) ) ;
#22780=CARTESIAN_POINT ( 'NONE',  ( -3.310556943750001313, 17.50000000000002132, -119.8516058028994706 ) ) ;
#22781=CARTESIAN_POINT ( 'NONE',  ( 2.340729813953370519E-16, 21.32270188528330834, -48.10160580289946353 ) ) ;
#22782=ORIENTED_EDGE ( 'NONE', *, *, #41899, .T. ) ;
#22783=CARTESIAN_POINT ( 'NONE',  ( -1.749999999999999778, 20.53108891324556140, -131.8213974700441042 ) ) ;
#22784=CARTESIAN_POINT ( 'NONE',  ( -1.655278471875002211, 14.63297358603754539, -69.68493913623279923 ) ) ;
#22785=CARTESIAN_POINT ( 'NONE',  ( 2.474675557024783212E-16, 21.54145188432740099, -124.2109808024215027 ) ) ;
#22786=CARTESIAN_POINT ( 'NONE',  ( -3.310556943750001313, 17.50000000000002132, -104.7641058028994649 ) ) ;
#22787=LINE ( 'NONE', #28737, #20022 ) ;
#22788=CARTESIAN_POINT ( 'NONE',  ( -1.394453263437886604E-15, 14.00000000000001776, -105.7109808024215027 ) ) ;
#22790=CARTESIAN_POINT ( 'NONE',  ( 1.750000000000001110, 20.53108891324555429, -76.29431413575484555 ) ) ;
#22791=CARTESIAN_POINT ( 'NONE',  ( 4.648177544792955347E-16, 21.00000000000002487, -133.2109808024214885 ) ) ;
#22792=CARTESIAN_POINT ( 'NONE',  ( -1.655278471875002211, 14.63297358603754006, -38.59743913623281486 ) ) ;
#22793=CARTESIAN_POINT ( 'NONE',  ( 3.310556943750001313, 19.41135094264166483, -97.26827246956612782 ) ) ;
#22794=( BOUNDED_CURVE ( )  B_SPLINE_CURVE ( 2, ( #32141, #3415, #2795, #35121, #41723, #25977, #32549, #15779, #5985 ),
 .UNSPECIFIED., .F., .F. ) 
 B_SPLINE_CURVE_WITH_KNOTS ( ( 3, 2, 2, 2, 3 ),
 ( 0.9562500000000000444, 0.9569444444444444864, 0.9583333333333333703, 0.9597222222222222543, 0.9604166666666666963 ),
 .UNSPECIFIED. ) 
 CURVE ( )  GEOMETRIC_REPRESENTATION_ITEM ( )  RATIONAL_B_SPLINE_CURVE ( ( 0.9330127018922194093, 0.9330127018922194093, 1.000000000000000000, 0.8660254037844387076, 1.000000000000000000, 0.8660254037844387076, 1.000000000000000000, 0.9330127018922194093, 0.9330127018922194093 ) ) 
 REPRESENTATION_ITEM ( '' )  );
#22795=CARTESIAN_POINT ( 'NONE',  ( 1.750000000000001110, 20.53108891324555074, -65.98806413671076143 ) ) ;
#22798=CARTESIAN_POINT ( 'NONE',  ( -3.310556943750002201, 15.58864905735837780, -118.7682724695661278 ) ) ;
#22799=CARTESIAN_POINT ( 'NONE',  ( -0.9378221735089335986, 21.00000000000002842, -136.8600726046389298 ) ) ;
#22804=CARTESIAN_POINT ( 'NONE',  ( 3.310556943750001313, 19.41135094264166838, -100.1807724695661079 ) ) ;
#22806=VERTEX_POINT ( 'NONE', #10962 ) ;
#22808=ADVANCED_FACE ( 'NONE', ( #39673 ), #23949, .T. ) ;
#22809=CARTESIAN_POINT ( 'NONE',  ( -1.750000000000002220, 14.46891108675448834, -126.7943141357548456 ) ) ;
#22810=CARTESIAN_POINT ( 'NONE',  ( -1.394453263437886604E-15, 14.00000000000001776, -105.4047308033774186 ) ) ;
#22811=CARTESIAN_POINT ( 'NONE',  ( -0.9378221735089377065, 21.00000000000001421, -135.1663226036829712 ) ) ;
#22812=EDGE_CURVE ( 'NONE', #18739, #10325, #8457, .T. ) ;
#22816=CARTESIAN_POINT ( 'NONE',  ( -3.310556943750002201, 15.58864905735836537, -31.68077246956614701 ) ) ;
#22817=CARTESIAN_POINT ( 'NONE',  ( -0.9378221735089465882, 21.00000000000001066, -123.8600726046389013 ) ) ;
#22821=EDGE_LOOP ( 'NONE', ( #10479, #23675, #41612, #13190 ) ) ;
#22827=CARTESIAN_POINT ( 'NONE',  ( -1.749999999999999778, 20.53108891324555785, -117.8213974700440900 ) ) ;
#22829=CARTESIAN_POINT ( 'NONE',  ( 1.655278471875001101, 20.36702641396249902, -133.1849391362327992 ) ) ;
#22830=CARTESIAN_POINT ( 'NONE',  ( 2.474675557024783212E-16, 21.54145188432739033, -32.21098080242150274 ) ) ;
#22831=CARTESIAN_POINT ( 'NONE',  ( 4.648177544792955347E-16, 21.00000000000001421, -66.21098080242148853 ) ) ;
#22832=LINE ( 'NONE', #32602, #8147 ) ;
#22833=CARTESIAN_POINT ( 'NONE',  ( -1.394453263437886604E-15, 14.00000000000001066, -37.40473080337743284 ) ) ;
#22835=CARTESIAN_POINT ( 'NONE',  ( 3.500000000000001332, 17.50000000000002487, -141.4609808024215170 ) ) ;
#22836=CARTESIAN_POINT ( 'NONE',  ( -3.310556943750002645, 15.58864905735837780, -123.6807724695661364 ) ) ;
#22839=CARTESIAN_POINT ( 'NONE',  ( 4.648177544792955347E-16, 21.00000000000001066, -28.90473080337742928 ) ) ;
#22840=CARTESIAN_POINT ( 'NONE',  ( 2.474675557024783212E-16, 21.54145188432739744, -91.21098080242151696 ) ) ;
#22841=CARTESIAN_POINT ( 'NONE',  ( 4.648177544792955347E-16, 21.00000000000001066, -37.21098080242150985 ) ) ;
#22842=CARTESIAN_POINT ( 'NONE',  ( 3.310556943750001313, 17.50000000000001421, -56.26410580289947916 ) ) ;
#22843=CARTESIAN_POINT ( 'NONE',  ( 3.310556943749999981, 15.58864905735837247, -114.4349391362327850 ) ) ;
#22845=CARTESIAN_POINT ( 'NONE',  ( 3.500000000000001776, 19.52072594216370405, -35.07139747004410424 ) ) ;
#22848=CARTESIAN_POINT ( 'NONE',  ( -3.310556943750000425, 19.41135094264167549, -133.9349391362327992 ) ) ;
#22851=DIRECTION ( 'NONE',  ( 0.000000000000000000, 1.000000000000000000, 0.000000000000000000 ) ) ;
#22852=CARTESIAN_POINT ( 'NONE',  ( -3.310556943750002645, 15.58864905735837070, -68.76827246956612782 ) ) ;
#22854=CARTESIAN_POINT ( 'NONE',  ( -3.310556943750002645, 15.58864905735836892, -66.68077246956613635 ) ) ;
#22856=CARTESIAN_POINT ( 'NONE',  ( 1.655278471875001101, 20.36702641396249192, -84.18493913623278502 ) ) ;
#22858=EDGE_CURVE ( 'NONE', #14873, #29443, #24500, .T. ) ;
#22862=CARTESIAN_POINT ( 'NONE',  ( -3.310556943750000425, 19.41135094264166483, -50.84743913623280775 ) ) ;
#22864=CARTESIAN_POINT ( 'NONE',  ( -1.655278471874999990, 20.36702641396249547, -105.9307724695661364 ) ) ;
#22865=CARTESIAN_POINT ( 'NONE',  ( 1.750000000000001110, 20.53108891324555074, -52.98806413671076854 ) ) ;
#22872=EDGE_CURVE ( 'NONE', #2767, #7389, #23377, .T. ) ;
#22873=CARTESIAN_POINT ( 'NONE',  ( -7.022189441860112050E-16, 13.67729811471671830, -60.51410580289947205 ) ) ;
#22874=( BOUNDED_CURVE ( )  B_SPLINE_CURVE ( 2, ( #17700, #31084, #14512, #14092, #37066, #1937, #27885, #23882, #4924 ),
 .UNSPECIFIED., .F., .F. ) 
 B_SPLINE_CURVE_WITH_KNOTS ( ( 3, 2, 2, 2, 3 ),
 ( 0.2062499999999999889, 0.2069444444444444309, 0.2083333333333333426, 0.2097222222222222265, 0.2104166666666666685 ),
 .UNSPECIFIED. ) 
 CURVE ( )  GEOMETRIC_REPRESENTATION_ITEM ( )  RATIONAL_B_SPLINE_CURVE ( ( 0.9330127018922194093, 0.9330127018922194093, 1.000000000000000000, 0.8660254037844387076, 1.000000000000000000, 0.8660254037844387076, 1.000000000000000000, 0.9330127018922194093, 0.9330127018922194093 ) ) 
 REPRESENTATION_ITEM ( '' )  );
#22875=EDGE_LOOP ( 'NONE', ( #9909, #10634, #19319, #29021 ) ) ;
#22877=CARTESIAN_POINT ( 'NONE',  ( 0.000000000000000000, 17.50000000000002487, -149.5231586289125687 ) ) ;
#22878=CARTESIAN_POINT ( 'NONE',  ( 1.749999999999998224, 14.46891108675447768, -55.62764746908817415 ) ) ;
#22880=LINE ( 'NONE', #35648, #18378 ) ;
#22881=ORIENTED_EDGE ( 'NONE', *, *, #33934, .F. ) ;
#22883=CARTESIAN_POINT ( 'NONE',  ( -1.655278471874999990, 20.36702641396249547, -122.9307724695661506 ) ) ;
#22886=CARTESIAN_POINT ( 'NONE',  ( -3.310556943750001313, 17.50000000000001066, -34.85160580289946353 ) ) ;
#22888=CARTESIAN_POINT ( 'NONE',  ( -3.310556943750001313, 17.50000000000001776, -89.85160580289947063 ) ) ;
#22889=CARTESIAN_POINT ( 'NONE',  ( 3.310556943750001313, 17.50000000000002487, -141.2641058028994792 ) ) ;
#22894=CARTESIAN_POINT ( 'NONE',  ( -3.310556943750002645, 15.58864905735837780, -131.7682724695661136 ) ) ;
#22896=CARTESIAN_POINT ( 'NONE',  ( 3.310556943749999981, 15.58864905735836892, -90.34743913623280775 ) ) ;
#22899=CARTESIAN_POINT ( 'NONE',  ( 0.9378221735089300459, 21.00000000000002487, -131.9493890021159359 ) ) ;
#22900=EDGE_CURVE ( 'NONE', #17229, #21111, #15623, .T. ) ;
#22901=CARTESIAN_POINT ( 'NONE',  ( -7.424026671074350129E-16, 13.45854811567263454, -73.40473080337743284 ) ) ;
#22902=CARTESIAN_POINT ( 'NONE',  ( 3.310556943750001313, 17.50000000000001421, -58.35160580289947063 ) ) ;
#22904=LINE ( 'NONE', #3337, #14973 ) ;
#22906=CARTESIAN_POINT ( 'NONE',  ( -1.655278471875002211, 14.63297358603754716, -84.68493913623278502 ) ) ;
#22907=FACE_OUTER_BOUND ( 'NONE', #11997, .T. ) ;
#22908=EDGE_CURVE ( 'NONE', #31863, #3869, #27719, .T. ) ;
#22910=CARTESIAN_POINT ( 'NONE',  ( 1.655278471874998436, 14.63297358603754716, -108.4307724695661506 ) ) ;
#22911=CARTESIAN_POINT ( 'NONE',  ( 1.655278471875001101, 20.36702641396249192, -80.09743913623280775 ) ) ;
#22913=ORIENTED_EDGE ( 'NONE', *, *, #40594, .T. ) ;
#22914=CARTESIAN_POINT ( 'NONE',  ( -3.310556943750002201, 15.58864905735837425, -102.7682724695661278 ) ) ;
#22915=CARTESIAN_POINT ( 'NONE',  ( -7.424026671074350129E-16, 13.45854811567263809, -101.4047308033774186 ) ) ;
#22918=CARTESIAN_POINT ( 'NONE',  ( 3.500000000000001332, 19.52072594216370405, -44.07139747004409003 ) ) ;
#22919=CARTESIAN_POINT ( 'NONE',  ( 0.9378221735089281585, 14.00000000000001243, -54.36007260463890844 ) ) ;
#22921=CARTESIAN_POINT ( 'NONE',  ( 1.655278471875001101, 20.36702641396248836, -66.09743913623280775 ) ) ;
#22923=CARTESIAN_POINT ( 'NONE',  ( -1.655278471874999990, 20.36702641396249547, -120.9307724695661364 ) ) ;
#22924=DIRECTION ( 'NONE',  ( -0.000000000000000000, 1.259100132267607459E-16, -1.000000000000000000 ) ) ;
#22928=ADVANCED_FACE ( 'NONE', ( #6037 ), #38158, .T. ) ;
#22929=CARTESIAN_POINT ( 'NONE',  ( -1.655278471874999990, 20.36702641396249192, -75.93077246956613635 ) ) ;
#22930=ORIENTED_EDGE ( 'NONE', *, *, #22900, .T. ) ;
#22931=ORIENTED_EDGE ( 'NONE', *, *, #30793, .T. ) ;
#22934=CARTESIAN_POINT ( 'NONE',  ( -3.310556943750002201, 15.58864905735837958, -142.6807724695661364 ) ) ;
#22936=CARTESIAN_POINT ( 'NONE',  ( 1.749999999999998224, 14.46891108675447590, -41.32139747004409713 ) ) ;
#22937=CARTESIAN_POINT ( 'NONE',  ( 1.655278471875001101, 20.36702641396248481, -45.18493913623279923 ) ) ;
#22938=CARTESIAN_POINT ( 'NONE',  ( 3.310556943750001313, 17.50000000000001776, -101.3516058028994706 ) ) ;
#22939=CARTESIAN_POINT ( 'NONE',  ( -7.022189441860112050E-16, 13.67729811471671475, -30.51410580289946495 ) ) ;
#22940=CARTESIAN_POINT ( 'NONE',  ( -1.394453263437886604E-15, 14.00000000000001421, -69.40473080337741862 ) ) ;
#22941=CARTESIAN_POINT ( 'NONE',  ( 3.500000000000001776, 19.52072594216371826, -102.3776474690881884 ) ) ;
#22943=CARTESIAN_POINT ( 'NONE',  ( -3.500000000000002220, 15.47927405783633503, -118.8776474690881599 ) ) ;
#22944=CARTESIAN_POINT ( 'NONE',  ( -3.500000000000000888, 19.52072594216371115, -92.73806413671077564 ) ) ;
#22948=CARTESIAN_POINT ( 'NONE',  ( -3.500000000000001332, 17.50000000000001421, -51.96098080242150985 ) ) ;
#22950=FACE_OUTER_BOUND ( 'NONE', #22135, .T. ) ;
#22951=CARTESIAN_POINT ( 'NONE',  ( -1.750000000000002220, 14.46891108675447768, -42.48806413671076143 ) ) ;
#22952=CARTESIAN_POINT ( 'NONE',  ( 1.750000000000001110, 20.53108891324555785, -106.2943141357548456 ) ) ;
#22953=CARTESIAN_POINT ( 'NONE',  ( 2.340729813953370519E-16, 21.32270188528330834, -26.10160580289947063 ) ) ;
#22958=CARTESIAN_POINT ( 'NONE',  ( 1.749999999999998224, 14.46891108675448301, -102.3213974700440900 ) ) ;
#22959=ADVANCED_FACE ( 'NONE', ( #11785 ), #12422, .F. ) ;
#22961=CARTESIAN_POINT ( 'NONE',  ( -3.310556943750002201, 15.58864905735837247, -82.68077246956615056 ) ) ;
#22962=CARTESIAN_POINT ( 'NONE',  ( 3.500000000000001332, 19.52072594216370760, -52.37764746908817415 ) ) ;
#22963=VERTEX_POINT ( 'NONE', #24568 ) ;
#22964=CARTESIAN_POINT ( 'NONE',  ( 1.750000000000001110, 20.53108891324554719, -33.98806413671076854 ) ) ;
#22966=VERTEX_POINT ( 'NONE', #18386 ) ;
#22968=CARTESIAN_POINT ( 'NONE',  ( 3.310556943750001313, 17.50000000000001776, -88.26410580289947916 ) ) ;
#22969=ORIENTED_EDGE ( 'NONE', *, *, #19415, .T. ) ;
#22970=ORIENTED_EDGE ( 'NONE', *, *, #12134, .T. ) ;
#22977=CARTESIAN_POINT ( 'NONE',  ( -1.394453263437886604E-15, 14.00000000000002132, -123.7109808024214885 ) ) ;
#22978=EDGE_CURVE ( 'NONE', #21640, #12728, #36149, .T. ) ;
#22979=CARTESIAN_POINT ( 'NONE',  ( 2.340729813953370519E-16, 21.32270188528332255, -130.0141058028994507 ) ) ;
#22980=ORIENTED_EDGE ( 'NONE', *, *, #40244, .F. ) ;
#22981=ORIENTED_EDGE ( 'NONE', *, *, #11838, .F. ) ;
#22982=CARTESIAN_POINT ( 'NONE',  ( 0.9378221735089281585, 14.00000000000001243, -64.36007260463891555 ) ) ;
#22983=CARTESIAN_POINT ( 'NONE',  ( 3.310556943749999981, 15.58864905735837247, -118.4349391362327992 ) ) ;
#22984=ORIENTED_EDGE ( 'NONE', *, *, #9034, .F. ) ;
#22986=CARTESIAN_POINT ( 'NONE',  ( 3.500000000000001332, 17.50000000000002487, -130.1547308033774186 ) ) ;
#22987=CARTESIAN_POINT ( 'NONE',  ( -3.310556943750001313, 17.50000000000001421, -72.85160580289947063 ) ) ;
#22988=CARTESIAN_POINT ( 'NONE',  ( 3.500000000000001332, 17.50000000000002132, -118.4609808024215170 ) ) ;
#22989=CARTESIAN_POINT ( 'NONE',  ( 3.310556943750001313, 19.41135094264166483, -100.1807724695661364 ) ) ;
#22992=CARTESIAN_POINT ( 'NONE',  ( -3.500000000000002220, 15.47927405783632615, -72.87764746908815994 ) ) ;
#22993=FACE_OUTER_BOUND ( 'NONE', #8225, .T. ) ;
#22994=CARTESIAN_POINT ( 'NONE',  ( 2.340729813953370519E-16, 21.32270188528330479, -38.01410580289947916 ) ) ;
#22995=CARTESIAN_POINT ( 'NONE',  ( 1.655278471875001101, 20.36702641396249192, -96.18493913623279923 ) ) ;
#22996=CARTESIAN_POINT ( 'NONE',  ( -3.500000000000001332, 17.50000000000001421, -64.65473080337743284 ) ) ;
#22998=CARTESIAN_POINT ( 'NONE',  ( -3.310556943750000425, 19.41135094264166838, -118.9349391362327992 ) ) ;
#23005=CARTESIAN_POINT ( 'NONE',  ( 4.648177544792955347E-16, 21.00000000000002132, -118.9047308033774328 ) ) ;
#23006=CARTESIAN_POINT ( 'NONE',  ( 3.310556943750001313, 17.50000000000001776, -96.26410580289946495 ) ) ;
#23007=CARTESIAN_POINT ( 'NONE',  ( 3.500000000000000000, 15.47927405783632437, -62.54431413575483845 ) ) ;
#23014=ORIENTED_EDGE ( 'NONE', *, *, #3368, .T. ) ;
#23018=CARTESIAN_POINT ( 'NONE',  ( 1.655278471874998436, 14.63297358603753828, -26.43077246956613990 ) ) ;
#23019=ORIENTED_EDGE ( 'NONE', *, *, #27667, .F. ) ;
#23020=LINE ( 'NONE', #3879, #29132 ) ;
#23023=CARTESIAN_POINT ( 'NONE',  ( -0.9378221735089268263, 14.00000000000002309, -138.4493890021159928 ) ) ;
#23024=ORIENTED_EDGE ( 'NONE', *, *, #11218, .F. ) ;
#23026=CARTESIAN_POINT ( 'NONE',  ( -0.9378221735089310451, 14.00000000000002309, -114.7556390011600200 ) ) ;
#23028=CARTESIAN_POINT ( 'NONE',  ( -3.500000000000001332, 17.50000000000002132, -119.6547308033774328 ) ) ;
#23030=CARTESIAN_POINT ( 'NONE',  ( -1.655278471875002211, 14.63297358603755427, -136.6849391362327992 ) ) ;
#23031=CARTESIAN_POINT ( 'NONE',  ( -1.750000000000002220, 14.46891108675447413, -25.79431413575483845 ) ) ;
#23033=VECTOR ( 'NONE', #37164, 1000.000000000000000 ) ;
#23035=CARTESIAN_POINT ( 'NONE',  ( 0.9378221735089287137, 14.00000000000002665, -142.6663226036829997 ) ) ;
#23037=CARTESIAN_POINT ( 'NONE',  ( -3.500000000000001332, 17.50000000000002487, -139.9609808024215170 ) ) ;
#23039=CARTESIAN_POINT ( 'NONE',  ( 3.310556943750001313, 17.50000000000002132, -119.2641058028994792 ) ) ;
#23041=ORIENTED_EDGE ( 'NONE', *, *, #24318, .T. ) ;
#23044=CARTESIAN_POINT ( 'NONE',  ( 2.474675557024783212E-16, 21.54145188432739744, -89.21098080242151696 ) ) ;
#23045=CARTESIAN_POINT ( 'NONE',  ( -3.500000000000002220, 15.47927405783632082, -36.87764746908817415 ) ) ;
#23046=CARTESIAN_POINT ( 'NONE',  ( 1.655278471875001101, 20.36702641396248836, -53.09743913623281486 ) ) ;
#23047=CARTESIAN_POINT ( 'NONE',  ( 3.310556943750001313, 17.50000000000002132, -113.3516058028994564 ) ) ;
#23049=CARTESIAN_POINT ( 'NONE',  ( -3.500000000000001332, 17.50000000000001066, -34.65473080337742573 ) ) ;
#23052=CARTESIAN_POINT ( 'NONE',  ( 1.655278471875001101, 20.36702641396249902, -133.1849391362327992 ) ) ;
#23054=CARTESIAN_POINT ( 'NONE',  ( -1.749999999999999778, 20.53108891324554719, -29.82139747004410069 ) ) ;
#23055=DIRECTION ( 'NONE',  ( -0.000000000000000000, 1.259100132267607459E-16, -1.000000000000000000 ) ) ;
#23057=CARTESIAN_POINT ( 'NONE',  ( -1.655278471875002211, 14.63297358603754361, -61.68493913623279923 ) ) ;
#23059=CARTESIAN_POINT ( 'NONE',  ( 3.310556943749999981, 15.58864905735836537, -63.34743913623281486 ) ) ;
#23061=CARTESIAN_POINT ( 'NONE',  ( 3.310556943750001313, 19.41135094264166838, -87.26827246956612782 ) ) ;
#23062=EDGE_CURVE ( 'NONE', #20433, #31031, #22832, .T. ) ;
#23064=CYLINDRICAL_SURFACE ( 'NONE', #7069, 3.499999999999999556 ) ;
#23066=CARTESIAN_POINT ( 'NONE',  ( -3.310556943750000425, 19.41135094264166483, -46.84743913623280065 ) ) ;
#23068=CARTESIAN_POINT ( 'NONE',  ( 3.310556943750001313, 17.50000000000002132, -104.2641058028994649 ) ) ;
#23069=CARTESIAN_POINT ( 'NONE',  ( 0.9378221735089300459, 21.00000000000001066, -41.94938900211595012 ) ) ;
#23071=ORIENTED_EDGE ( 'NONE', *, *, #27063, .F. ) ;
#23073=VERTEX_POINT ( 'NONE', #10070 ) ;
#23075=CARTESIAN_POINT ( 'NONE',  ( -1.655278471875002211, 14.63297358603754361, -55.59743913623280065 ) ) ;
#23078=CARTESIAN_POINT ( 'NONE',  ( 1.750000000000001110, 20.53108891324555429, -76.29431413575484555 ) ) ;
#23083=CARTESIAN_POINT ( 'NONE',  ( 0.000000000000000000, 17.50000000000002487, -149.5231586289125687 ) ) ;
#23085=CARTESIAN_POINT ( 'NONE',  ( -1.750000000000002220, 14.46891108675447768, -44.79431413575483845 ) ) ;
#23086=CARTESIAN_POINT ( 'NONE',  ( 4.648177544792955347E-16, 21.00000000000002487, -133.9047308033774186 ) ) ;
#23087=CARTESIAN_POINT ( 'NONE',  ( 1.749999999999998224, 14.46891108675448123, -94.62764746908815994 ) ) ;
#23088=EDGE_CURVE ( 'NONE', #13712, #14781, #38994, .T. ) ;
#23090=CARTESIAN_POINT ( 'NONE',  ( 3.310556943750001313, 17.50000000000001066, -35.35160580289946353 ) ) ;
#23093=CARTESIAN_POINT ( 'NONE',  ( 1.655278471875001101, 20.36702641396249192, -89.18493913623279923 ) ) ;
#23094=CARTESIAN_POINT ( 'NONE',  ( 3.310556943750001313, 19.41135094264167549, -140.1807724695661364 ) ) ;
#23098=VECTOR ( 'NONE', #39856, 1000.000000000000000 ) ;
#23099=CARTESIAN_POINT ( 'NONE',  ( 3.310556943750001313, 17.50000000000002132, -128.3516058028994564 ) ) ;
#23100=CARTESIAN_POINT ( 'NONE',  ( 3.500000000000000000, 15.47927405783632615, -70.23806413671077564 ) ) ;
#23101=CARTESIAN_POINT ( 'NONE',  ( 1.655278471874998436, 14.63297358603754539, -92.43077246956613635 ) ) ;
#23103=FACE_OUTER_BOUND ( 'NONE', #41664, .T. ) ;
#23104=CARTESIAN_POINT ( 'NONE',  ( 3.500000000000001776, 19.52072594216371115, -77.07139747004409003 ) ) ;
#23106=CARTESIAN_POINT ( 'NONE',  ( -3.310556943750002201, 15.58864905735836892, -61.76827246956613493 ) ) ;
#23108=CARTESIAN_POINT ( 'NONE',  ( 3.405278471875001323, 17.50000000000002487, -143.2094183031384489 ) ) ;
#23110=CARTESIAN_POINT ( 'NONE',  ( 1.655278471874998436, 14.63297358603754361, -78.51827246956614204 ) ) ;
#23111=CARTESIAN_POINT ( 'NONE',  ( 0.000000000000000000, 17.50000000000002487, -149.5231586289125687 ) ) ;
#23113=CARTESIAN_POINT ( 'NONE',  ( 3.310556943749999981, 15.58864905735837247, -111.3474391362328078 ) ) ;
#23114=CARTESIAN_POINT ( 'NONE',  ( 2.340729813953370519E-16, 21.32270188528331190, -80.01410580289946495 ) ) ;
#23116=EDGE_LOOP ( 'NONE', ( #210, #11770, #33965, #25353 ) ) ;
#23118=CARTESIAN_POINT ( 'NONE',  ( -3.310556943750002201, 15.58864905735837425, -101.7682724695661278 ) ) ;
#23119=CARTESIAN_POINT ( 'NONE',  ( -7.424026671074350129E-16, 13.45854811567263809, -104.4047308033774186 ) ) ;
#23121=CARTESIAN_POINT ( 'NONE',  ( -3.500000000000002220, 15.47927405783632970, -94.57139747004409003 ) ) ;
#23124=CARTESIAN_POINT ( 'NONE',  ( -7.022189441860112050E-16, 13.67729811471672186, -58.51410580289947916 ) ) ;
#23125=( BOUNDED_CURVE ( )  B_SPLINE_CURVE ( 2, ( #38765, #38553, #16030, #41969, #26219, #22385, #19201, #15813, #39168 ),
 .UNSPECIFIED., .F., .T. ) 
 B_SPLINE_CURVE_WITH_KNOTS ( ( 3, 2, 2, 2, 3 ),
 ( 0.7895833333333333037, 0.7902777777777777457, 0.7916666666666666297, 0.7930555555555555136, 0.7937499999999999556 ),
 .UNSPECIFIED. ) 
 CURVE ( )  GEOMETRIC_REPRESENTATION_ITEM ( )  RATIONAL_B_SPLINE_CURVE ( ( 0.9330127018922194093, 0.9330127018922194093, 1.000000000000000000, 0.8660254037844387076, 1.000000000000000000, 0.8660254037844387076, 1.000000000000000000, 0.9330127018922194093, 0.9330127018922194093 ) ) 
 REPRESENTATION_ITEM ( '' )  );
#23126=CARTESIAN_POINT ( 'NONE',  ( -1.749999999999999778, 20.53108891324554719, -30.12764746908817770 ) ) ;
#23127=CARTESIAN_POINT ( 'NONE',  ( 3.310556943750001313, 17.50000000000002132, -123.2641058028994649 ) ) ;
#23128=CARTESIAN_POINT ( 'NONE',  ( 4.648177544792955347E-16, 21.00000000000002132, -118.2109808024215170 ) ) ;
#23132=CARTESIAN_POINT ( 'NONE',  ( 3.500000000000000000, 15.47927405783632970, -99.54431413575485976 ) ) ;
#23133=CARTESIAN_POINT ( 'NONE',  ( -0.9378221735089310451, 14.00000000000002132, -89.75563900116003424 ) ) ;
#23134=CARTESIAN_POINT ( 'NONE',  ( -7.022189441860112050E-16, 13.67729811471672186, -74.51410580289947916 ) ) ;
#23135=ORIENTED_EDGE ( 'NONE', *, *, #6395, .T. ) ;
#23136=ORIENTED_EDGE ( 'NONE', *, *, #40157, .F. ) ;
#23139=EDGE_CURVE ( 'NONE', #13827, #3209, #16062, .T. ) ;
#23140=CARTESIAN_POINT ( 'NONE',  ( 3.310556943750001313, 19.41135094264167549, -139.1807724695661364 ) ) ;
#23141=CARTESIAN_POINT ( 'NONE',  ( -0.9378221735089221633, 14.00000000000001599, -128.7556390011600342 ) ) ;
#23142=CARTESIAN_POINT ( 'NONE',  ( 3.500000000000000000, 15.47927405783633503, -141.5443141357548313 ) ) ;
#23145=CARTESIAN_POINT ( 'NONE',  ( -7.022189441860112050E-16, 13.67729811471671475, -36.60160580289946353 ) ) ;
#23146=CARTESIAN_POINT ( 'NONE',  ( 2.340729813953370519E-16, 21.32270188528331900, -103.1016058028994564 ) ) ;
#23147=CARTESIAN_POINT ( 'NONE',  ( 1.655278471875001101, 20.36702641396249902, -142.1849391362327992 ) ) ;
#23149=CARTESIAN_POINT ( 'NONE',  ( -7.424026671074350129E-16, 13.45854811567263809, -103.7109808024214885 ) ) ;
#23152=CARTESIAN_POINT ( 'NONE',  ( 3.500000000000000000, 15.47927405783632615, -92.23806413671076143 ) ) ;
#23158=CARTESIAN_POINT ( 'NONE',  ( -1.749999999999999778, 20.53108891324555074, -56.12764746908817415 ) ) ;
#23160=CARTESIAN_POINT ( 'NONE',  ( -3.500000000000002220, 15.47927405783632437, -46.57139747004410424 ) ) ;
#23161=CARTESIAN_POINT ( 'NONE',  ( -1.394453263437886604E-15, 14.00000000000001776, -82.40473080337743284 ) ) ;
#23162=CARTESIAN_POINT ( 'NONE',  ( -7.424026671074350129E-16, 13.45854811567263276, -43.40473080337743284 ) ) ;
#23164=CARTESIAN_POINT ( 'NONE',  ( 1.655278471874998436, 14.63297358603753828, -28.51827246956613493 ) ) ;
#23166=DIRECTION ( 'NONE',  ( 0.000000000000000000, 1.000000000000000000, 0.000000000000000000 ) ) ;
#23167=CYLINDRICAL_SURFACE ( 'NONE', #23754, 3.499999999999999556 ) ;
#23169=CARTESIAN_POINT ( 'NONE',  ( 0.9378221735089300459, 21.00000000000001066, -35.94938900211595723 ) ) ;
#23171=CARTESIAN_POINT ( 'NONE',  ( -1.655278471874999990, 20.36702641396249192, -83.93077246956615056 ) ) ;
#23173=ORIENTED_EDGE ( 'NONE', *, *, #40824, .F. ) ;
#23174=CARTESIAN_POINT ( 'NONE',  ( -1.394453263437886604E-15, 14.00000000000001066, -34.40473080337743284 ) ) ;
#23175=( BOUNDED_CURVE ( )  B_SPLINE_CURVE ( 2, ( #9829, #15789, #9399, #12160, #22362, #31935, #26, #2807, #9184 ),
 .UNSPECIFIED., .F., .T. ) 
 B_SPLINE_CURVE_WITH_KNOTS ( ( 3, 2, 2, 2, 3 ),
 ( 0.4145833333333333592, 0.4152777777777778012, 0.4166666666666666852, 0.4180555555555555691, 0.4187500000000000111 ),
 .UNSPECIFIED. ) 
 CURVE ( )  GEOMETRIC_REPRESENTATION_ITEM ( )  RATIONAL_B_SPLINE_CURVE ( ( 0.9330127018922194093, 0.9330127018922220739, 1.000000000000000000, 0.8660254037844387076, 1.000000000000000000, 0.8660254037844387076, 1.000000000000000000, 0.9330127018922194093, 0.9330127018922194093 ) ) 
 REPRESENTATION_ITEM ( '' )  );
#23176=DIRECTION ( 'NONE',  ( -0.000000000000000000, 1.259100132267607459E-16, -1.000000000000000000 ) ) ;
#23177=ORIENTED_EDGE ( 'NONE', *, *, #17976, .F. ) ;
#23179=CARTESIAN_POINT ( 'NONE',  ( -1.655278471875002211, 14.63297358603754716, -91.59743913623280775 ) ) ;
#23180=EDGE_CURVE ( 'NONE', #37225, #40441, #12634, .T. ) ;
#23181=ORIENTED_EDGE ( 'NONE', *, *, #7460, .F. ) ;
#23187=CARTESIAN_POINT ( 'NONE',  ( 3.310556943750001313, 19.41135094264166838, -125.1807724695661364 ) ) ;
#23189=CARTESIAN_POINT ( 'NONE',  ( -3.500000000000002220, 15.47927405783632970, -94.87764746908814573 ) ) ;
#23190=CARTESIAN_POINT ( 'NONE',  ( -3.310556943750001313, 17.50000000000001421, -53.85160580289946353 ) ) ;
#23191=CARTESIAN_POINT ( 'NONE',  ( 1.655278471874998436, 14.63297358603754894, -121.5182724695661278 ) ) ;
#23192=ORIENTED_EDGE ( 'NONE', *, *, #24236, .F. ) ;
#23193=EDGE_LOOP ( 'NONE', ( #24401, #6072, #18411, #20941 ) ) ;
#23194=CARTESIAN_POINT ( 'NONE',  ( 1.750000000000001110, 20.53108891324555785, -124.9880641367107614 ) ) ;
#23195=VECTOR ( 'NONE', #30217, 1000.000000000000000 ) ;
#23196=CARTESIAN_POINT ( 'NONE',  ( 3.310556943749999981, 15.58864905735836714, -69.43493913623279923 ) ) ;
#23197=CARTESIAN_POINT ( 'NONE',  ( -3.500000000000002220, 15.47927405783633503, -115.8776474690881884 ) ) ;
#23198=CARTESIAN_POINT ( 'NONE',  ( -3.310556943750001313, 17.50000000000001776, -99.76410580289947916 ) ) ;
#23202=CARTESIAN_POINT ( 'NONE',  ( -3.500000000000001332, 17.50000000000001421, -68.96098080242150274 ) ) ;
#23204=CARTESIAN_POINT ( 'NONE',  ( 2.340729813953370519E-16, 21.32270188528330479, -40.01410580289947916 ) ) ;
#23205=CARTESIAN_POINT ( 'NONE',  ( 3.310556943750001313, 19.41135094264166483, -94.26827246956612782 ) ) ;
#23206=CARTESIAN_POINT ( 'NONE',  ( 2.474675557024783212E-16, 21.54145188432739388, -58.90473080337743284 ) ) ;
#23208=CARTESIAN_POINT ( 'NONE',  ( -1.655278471874999990, 20.36702641396249547, -120.0182724695661278 ) ) ;
#23215=CARTESIAN_POINT ( 'NONE',  ( -1.655278471875002211, 14.63297358603754894, -100.5974391362328078 ) ) ;
#23216=DIRECTION ( 'NONE',  ( -0.000000000000000000, 1.259100132267607459E-16, -1.000000000000000000 ) ) ;
#23220=CARTESIAN_POINT ( 'NONE',  ( 1.750000000000001110, 20.53108891324555429, -81.29431413575484555 ) ) ;
#23221=CARTESIAN_POINT ( 'NONE',  ( -1.394453263437886604E-15, 14.00000000000002132, -112.4047308033774186 ) ) ;
#23222=ORIENTED_EDGE ( 'NONE', *, *, #37568, .F. ) ;
#23226=CARTESIAN_POINT ( 'NONE',  ( -3.310556943750002201, 15.58864905735836537, -29.68077246956614346 ) ) ;
#23228=CARTESIAN_POINT ( 'NONE',  ( -3.500000000000001332, 17.50000000000002132, -123.6547308033774186 ) ) ;
#23229=VECTOR ( 'NONE', #10346, 1000.000000000000000 ) ;
#23233=ORIENTED_EDGE ( 'NONE', *, *, #18638, .F. ) ;
#23234=CARTESIAN_POINT ( 'NONE',  ( -3.500000000000000000, 19.52072594216370405, -37.73806413671076854 ) ) ;
#23237=CARTESIAN_POINT ( 'NONE',  ( -0.9378221735089291577, 21.00000000000001776, -81.16632260368297125 ) ) ;
#23238=VECTOR ( 'NONE', #16214, 1000.000000000000000 ) ;
#23240=CARTESIAN_POINT ( 'NONE',  ( 3.310556943749999981, 15.58864905735837780, -137.4349391362327992 ) ) ;
#23241=CARTESIAN_POINT ( 'NONE',  ( -7.424026671074350129E-16, 13.45854811567263098, -25.71098080242151340 ) ) ;
#23247=CARTESIAN_POINT ( 'NONE',  ( 1.749999999999998224, 14.46891108675447590, -43.32139747004409713 ) ) ;
#23249=CARTESIAN_POINT ( 'NONE',  ( -3.500000000000001332, 17.50000000000002487, -133.9609808024214885 ) ) ;
#23250=CARTESIAN_POINT ( 'NONE',  ( 1.655278471875001101, 20.36702641396249547, -119.0974391362328078 ) ) ;
#23254=CARTESIAN_POINT ( 'NONE',  ( 2.474675557024783212E-16, 21.54145188432739744, -87.21098080242150274 ) ) ;
#23255=CARTESIAN_POINT ( 'NONE',  ( -1.394453263437886604E-15, 14.00000000000001776, -105.7109808024215027 ) ) ;
#23256=CARTESIAN_POINT ( 'NONE',  ( 3.310556943750001313, 17.50000000000001421, -52.26410580289947205 ) ) ;
#23257=CARTESIAN_POINT ( 'NONE',  ( 3.310556943750001313, 19.41135094264166838, -114.2682724695661136 ) ) ;
#23259=CARTESIAN_POINT ( 'NONE',  ( -3.500000000000000888, 19.52072594216370405, -29.73806413671076143 ) ) ;
#23260=CARTESIAN_POINT ( 'NONE',  ( 3.500000000000001332, 19.52072594216371826, -116.3776474690881741 ) ) ;
#23262=CARTESIAN_POINT ( 'NONE',  ( -3.310556943750000425, 19.41135094264167549, -135.9349391362327992 ) ) ;
#23265=DIRECTION ( 'NONE',  ( -0.000000000000000000, 1.259100132267607459E-16, -1.000000000000000000 ) ) ;
#23266=CARTESIAN_POINT ( 'NONE',  ( 3.310556943750001313, 17.50000000000001421, -65.35160580289945642 ) ) ;
#23269=CARTESIAN_POINT ( 'NONE',  ( 1.655278471875001101, 20.36702641396248836, -66.09743913623280775 ) ) ;
#23270=VERTEX_POINT ( 'NONE', #38575 ) ;
#23271=CARTESIAN_POINT ( 'NONE',  ( -3.310556943750000425, 19.41135094264166838, -84.93493913623279923 ) ) ;
#23272=EDGE_CURVE ( 'NONE', #3618, #7219, #5978, .T. ) ;
#23278=CARTESIAN_POINT ( 'NONE',  ( -1.655278471875002211, 14.63297358603754184, -47.59743913623280775 ) ) ;
#23281=CARTESIAN_POINT ( 'NONE',  ( 2.340729813953370519E-16, 21.32270188528331190, -99.01410580289946495 ) ) ;
#23288=CARTESIAN_POINT ( 'NONE',  ( -1.655278471875002211, 14.63297358603754184, -51.59743913623281486 ) ) ;
#23289=ORIENTED_EDGE ( 'NONE', *, *, #38085, .F. ) ;
#23290=VERTEX_POINT ( 'NONE', #36648 ) ;
#23291=( BOUNDED_CURVE ( )  B_SPLINE_CURVE ( 2, ( #5417, #11796, #12215, #24791, #37754, #8610, #38379, #21582, #18395 ),
 .UNSPECIFIED., .F., .T. ) 
 B_SPLINE_CURVE_WITH_KNOTS ( ( 3, 2, 2, 2, 3 ),
 ( 0.4062500000000000000, 0.4069444444444444420, 0.4083333333333333259, 0.4097222222222222099, 0.4104166666666666519 ),
 .UNSPECIFIED. ) 
 CURVE ( )  GEOMETRIC_REPRESENTATION_ITEM ( )  RATIONAL_B_SPLINE_CURVE ( ( 0.9330127018922194093, 0.9330127018922194093, 1.000000000000000000, 0.8660254037844387076, 1.000000000000000000, 0.8660254037844387076, 1.000000000000000000, 0.9330127018922194093, 0.9330127018922194093 ) ) 
 REPRESENTATION_ITEM ( '' )  );
#23293=CARTESIAN_POINT ( 'NONE',  ( 3.500000000000001332, 19.52072594216371826, -125.0713974700440900 ) ) ;
#23295=( BOUNDED_CURVE ( )  B_SPLINE_CURVE ( 2, ( #37604, #34829, #31842, #18877, #31635, #2711, #38230, #41006, #15697 ),
 .UNSPECIFIED., .F., .T. ) 
 B_SPLINE_CURVE_WITH_KNOTS ( ( 3, 2, 2, 2, 3 ),
 ( 0.7937499999999999556, 0.7944444444444443976, 0.7958333333333332815, 0.7972222222222222765, 0.7979166666666667185 ),
 .UNSPECIFIED. ) 
 CURVE ( )  GEOMETRIC_REPRESENTATION_ITEM ( )  RATIONAL_B_SPLINE_CURVE ( ( 0.9330127018922194093, 0.9330127018922194093, 1.000000000000000000, 0.8660254037844387076, 1.000000000000000000, 0.8660254037844387076, 1.000000000000000000, 0.9330127018922194093, 0.9330127018922194093 ) ) 
 REPRESENTATION_ITEM ( '' )  );
#23297=CARTESIAN_POINT ( 'NONE',  ( 4.648177544792955347E-16, 21.00000000000001421, -46.90473080337742573 ) ) ;
#23298=ORIENTED_EDGE ( 'NONE', *, *, #20819, .F. ) ;
#23300=CARTESIAN_POINT ( 'NONE',  ( -1.749999999999999778, 20.53108891324554719, -42.12764746908817415 ) ) ;
#23301=ADVANCED_FACE ( 'NONE', ( #11326 ), #20393, .T. ) ;
#23302=CARTESIAN_POINT ( 'NONE',  ( 4.286263797015737581E-16, 14.00000000000002487, -149.5231586289125687 ) ) ;
#23303=ADVANCED_FACE ( 'NONE', ( #22950 ), #29748, .T. ) ;
#23305=CARTESIAN_POINT ( 'NONE',  ( 1.750000000000001110, 20.53108891324555429, -94.29431413575484555 ) ) ;
#23308=CARTESIAN_POINT ( 'NONE',  ( 1.655278471875001101, 20.36702641396248481, -29.18493913623279568 ) ) ;
#23310=CARTESIAN_POINT ( 'NONE',  ( -0.9378221735089291577, 21.00000000000001776, -97.86007260463888713 ) ) ;
#23312=CARTESIAN_POINT ( 'NONE',  ( -3.310556943750001313, 17.50000000000001776, -80.85160580289945642 ) ) ;
#23313=CARTESIAN_POINT ( 'NONE',  ( -3.310556943750002645, 15.58864905735837780, -134.6807724695661364 ) ) ;
#23316=AXIS2_PLACEMENT_3D ( 'NONE', #18069, #34028, #15307 ) ;
#23319=CARTESIAN_POINT ( 'NONE',  ( -1.655278471875002211, 14.63297358603755249, -128.6849391362327992 ) ) ;
#23320=CARTESIAN_POINT ( 'NONE',  ( -0.9378221735089310451, 14.00000000000001599, -68.75563900116003424 ) ) ;
#23321=CARTESIAN_POINT ( 'NONE',  ( 2.340729813953370519E-16, 21.32270188528331190, -85.01410580289949337 ) ) ;
#23324=CARTESIAN_POINT ( 'NONE',  ( 1.750000000000001110, 20.53108891324555785, -126.2943141357548456 ) ) ;
#23325=CARTESIAN_POINT ( 'NONE',  ( -3.500000000000002220, 15.47927405783632615, -75.57139747004410424 ) ) ;
#23326=CARTESIAN_POINT ( 'NONE',  ( -3.310556943750000425, 19.41135094264166483, -61.93493913623281344 ) ) ;
#23330=CARTESIAN_POINT ( 'NONE',  ( 1.655278471875001101, 20.36702641396249192, -78.18493913623279923 ) ) ;
#23331=CARTESIAN_POINT ( 'NONE',  ( -3.500000000000002220, 15.47927405783632615, -59.87764746908817415 ) ) ;
#23333=CARTESIAN_POINT ( 'NONE',  ( 3.310556943750001313, 17.50000000000002132, -110.2641058028994649 ) ) ;
#23334=CARTESIAN_POINT ( 'NONE',  ( 1.655278471874998436, 14.63297358603754361, -79.43077246956615056 ) ) ;
#23335=CARTESIAN_POINT ( 'NONE',  ( 3.500000000000001332, 17.50000000000002487, -138.4609808024214885 ) ) ;
#23336=ORIENTED_EDGE ( 'NONE', *, *, #6689, .F. ) ;
#23337=CARTESIAN_POINT ( 'NONE',  ( -3.310556943750000425, 19.41135094264166838, -102.9349391362327992 ) ) ;
#23338=CARTESIAN_POINT ( 'NONE',  ( -3.500000000000000888, 19.52072594216371115, -100.7380641367107756 ) ) ;
#23340=CARTESIAN_POINT ( 'NONE',  ( 4.648177544792955347E-16, 21.00000000000002132, -104.9047308033774186 ) ) ;
#23341=CARTESIAN_POINT ( 'NONE',  ( 3.500000000000001332, 19.52072594216370760, -54.07139747004409713 ) ) ;
#23343=CARTESIAN_POINT ( 'NONE',  ( 3.310556943749999981, 15.58864905735836537, -63.34743913623281486 ) ) ;
#23345=CARTESIAN_POINT ( 'NONE',  ( 3.310556943749999981, 15.58864905735837247, -114.3474391362328078 ) ) ;
#23347=EDGE_CURVE ( 'NONE', #19989, #39287, #27483, .T. ) ;
#23350=VERTEX_POINT ( 'NONE', #26570 ) ;
#23351=ADVANCED_FACE ( 'NONE', ( #7425 ), #13170, .T. ) ;
#23355=CARTESIAN_POINT ( 'NONE',  ( -1.655278471875002211, 14.63297358603754539, -76.59743913623280775 ) ) ;
#23356=ORIENTED_EDGE ( 'NONE', *, *, #12855, .F. ) ;
#23360=ADVANCED_FACE ( 'NONE', ( #10407 ), #39530, .T. ) ;
#23361=ORIENTED_EDGE ( 'NONE', *, *, #17754, .T. ) ;
#23362=CARTESIAN_POINT ( 'NONE',  ( 3.310556943749999981, 15.58864905735837425, -133.3474391362328220 ) ) ;
#23364=EDGE_CURVE ( 'NONE', #2263, #13986, #3388, .T. ) ;
#23365=CARTESIAN_POINT ( 'NONE',  ( 3.500000000000000000, 15.47927405783632082, -41.23806413671076143 ) ) ;
#23366=CARTESIAN_POINT ( 'NONE',  ( -7.022189441860112050E-16, 13.67729811471671475, -39.60160580289946353 ) ) ;
#23367=CARTESIAN_POINT ( 'NONE',  ( -1.655278471874999990, 20.36702641396249192, -98.01827246956612782 ) ) ;
#23369=CARTESIAN_POINT ( 'NONE',  ( 1.655278471875001101, 20.36702641396248481, -25.09743913623281486 ) ) ;
#23371=CARTESIAN_POINT ( 'NONE',  ( -1.750000000000002220, 14.46891108675448478, -100.7943141357548456 ) ) ;
#23375=CARTESIAN_POINT ( 'NONE',  ( -3.500000000000001332, 17.50000000000001776, -91.65473080337743284 ) ) ;
#23377=( BOUNDED_CURVE ( )  B_SPLINE_CURVE ( 2, ( #28370, #27746, #37744, #8601, #37532, #27954, #40929, #12207, #18179 ),
 .UNSPECIFIED., .F., .F. ) 
 B_SPLINE_CURVE_WITH_KNOTS ( ( 3, 2, 2, 2, 3 ),
 ( 0.5520833333333333703, 0.5527777777777778123, 0.5541666666666666963, 0.5555555555555555802, 0.5562500000000000222 ),
 .UNSPECIFIED. ) 
 CURVE ( )  GEOMETRIC_REPRESENTATION_ITEM ( )  RATIONAL_B_SPLINE_CURVE ( ( 0.9330127018922194093, 0.9330127018922194093, 1.000000000000000000, 0.8660254037844387076, 1.000000000000000000, 0.8660254037844387076, 1.000000000000000000, 0.9330127018922194093, 0.9330127018922194093 ) ) 
 REPRESENTATION_ITEM ( '' )  );
#23380=CARTESIAN_POINT ( 'NONE',  ( 3.500000000000000000, 15.47927405783632615, -68.23806413671077564 ) ) ;
#23381=CARTESIAN_POINT ( 'NONE',  ( -1.749999999999999778, 20.53108891324555074, -52.12764746908816704 ) ) ;
#23383=DIRECTION ( 'NONE',  ( -0.000000000000000000, 1.259100132267607459E-16, -1.000000000000000000 ) ) ;
#23385=CARTESIAN_POINT ( 'NONE',  ( -7.424026671074350129E-16, 13.45854811567263276, -44.40473080337743994 ) ) ;
#23388=CARTESIAN_POINT ( 'NONE',  ( 3.310556943750001313, 17.50000000000001066, -29.35160580289947063 ) ) ;
#23390=DIRECTION ( 'NONE',  ( 0.000000000000000000, 1.000000000000000000, 0.000000000000000000 ) ) ;
#23391=CARTESIAN_POINT ( 'NONE',  ( -1.394453263437886604E-15, 14.00000000000001421, -56.71098080242150985 ) ) ;
#23393=CARTESIAN_POINT ( 'NONE',  ( -1.394453263437886604E-15, 14.00000000000001066, -36.40473080337743284 ) ) ;
#23395=CARTESIAN_POINT ( 'NONE',  ( -3.310556943750002201, 15.58864905735837070, -77.68077246956615056 ) ) ;
#23396=CARTESIAN_POINT ( 'NONE',  ( 0.9378221735089281585, 14.00000000000001066, -52.66632260368298546 ) ) ;
#23398=CARTESIAN_POINT ( 'NONE',  ( 0.000000000000000000, 17.50000000000002487, -149.5231586289125687 ) ) ;
#23399=CARTESIAN_POINT ( 'NONE',  ( -0.9378221735089291577, 21.00000000000001066, -45.16632260368299256 ) ) ;
#23402=CARTESIAN_POINT ( 'NONE',  ( -3.310556943750001313, 17.50000000000001776, -87.76410580289947916 ) ) ;
#23407=EDGE_CURVE ( 'NONE', #7031, #9419, #28828, .T. ) ;
#23409=CARTESIAN_POINT ( 'NONE',  ( 0.000000000000000000, 17.50000000000002487, -149.5231586289125687 ) ) ;
#23410=CARTESIAN_POINT ( 'NONE',  ( -3.310556943750002645, 15.58864905735837780, -126.6807724695661221 ) ) ;
#23413=CARTESIAN_POINT ( 'NONE',  ( -1.655278471875002211, 14.63297358603754184, -53.68493913623280633 ) ) ;
#23414=CARTESIAN_POINT ( 'NONE',  ( 2.340729813953370519E-16, 21.32270188528331900, -116.1016058028994848 ) ) ;
#23416=ORIENTED_EDGE ( 'NONE', *, *, #27764, .F. ) ;
#23417=CARTESIAN_POINT ( 'NONE',  ( -7.424026671074350129E-16, 13.45854811567264164, -123.4047308033774186 ) ) ;
#23418=CARTESIAN_POINT ( 'NONE',  ( -7.022189441860112050E-16, 13.67729811471671653, -40.51410580289947916 ) ) ;
#23419=CARTESIAN_POINT ( 'NONE',  ( 2.340729813953370519E-16, 21.32270188528330834, -73.10160580289948484 ) ) ;
#23420=CARTESIAN_POINT ( 'NONE',  ( 3.500000000000001776, 19.52072594216371826, -117.3776474690881599 ) ) ;
#23421=CARTESIAN_POINT ( 'NONE',  ( -7.022189441860112050E-16, 13.67729811471672541, -104.5141058028994507 ) ) ;
#23422=CARTESIAN_POINT ( 'NONE',  ( -1.394453263437886604E-15, 14.00000000000001066, -42.40473080337742573 ) ) ;
#23423=CARTESIAN_POINT ( 'NONE',  ( 0.000000000000000000, 17.50000000000002487, -149.5231586289125687 ) ) ;
#23425=CARTESIAN_POINT ( 'NONE',  ( -7.424026671074350129E-16, 13.45854811567263454, -67.71098080242151696 ) ) ;
#23426=CARTESIAN_POINT ( 'NONE',  ( -1.655278471875002211, 14.63297358603754006, -37.59743913623281486 ) ) ;
#23427=( BOUNDED_CURVE ( )  B_SPLINE_CURVE ( 2, ( #35454, #9084, #22064, #2071, #11850, #28646, #41635, #24849, #8661 ),
 .UNSPECIFIED., .F., .F. ) 
 B_SPLINE_CURVE_WITH_KNOTS ( ( 3, 2, 2, 2, 3 ),
 ( 0.1687500000000000111, 0.1694444444444444531, 0.1708333333333333370, 0.1722222222222222210, 0.1729166666666666630 ),
 .UNSPECIFIED. ) 
 CURVE ( )  GEOMETRIC_REPRESENTATION_ITEM ( )  RATIONAL_B_SPLINE_CURVE ( ( 0.9330127018922194093, 0.9330127018922194093, 1.000000000000000000, 0.8660254037844387076, 1.000000000000000000, 0.8660254037844387076, 1.000000000000000000, 0.9330127018922194093, 0.9330127018922194093 ) ) 
 REPRESENTATION_ITEM ( '' )  );
#23428=CARTESIAN_POINT ( 'NONE',  ( -3.310556943750000425, 19.41135094264166483, -94.93493913623278502 ) ) ;
#23429=AXIS2_PLACEMENT_3D ( 'NONE', #28688, #21890, #2540 ) ;
#23430=CARTESIAN_POINT ( 'NONE',  ( -3.500000000000002220, 15.47927405783632437, -60.57139747004410424 ) ) ;
#23432=CARTESIAN_POINT ( 'NONE',  ( -3.310556943750000425, 19.41135094264166838, -109.9349391362327992 ) ) ;
#23434=CARTESIAN_POINT ( 'NONE',  ( 1.655278471875001101, 20.36702641396248481, -42.18493913623279212 ) ) ;
#23436=CARTESIAN_POINT ( 'NONE',  ( -0.9378221735089310451, 14.00000000000001599, -60.75563900116002003 ) ) ;
#23440=CARTESIAN_POINT ( 'NONE',  ( 0.9378221735089281585, 14.00000000000001243, -61.66632260368298546 ) ) ;
#23441=CARTESIAN_POINT ( 'NONE',  ( -1.655278471874999990, 20.36702641396249192, -91.93077246956613635 ) ) ;
#23442=CARTESIAN_POINT ( 'NONE',  ( 4.648177544792955347E-16, 21.00000000000002487, -135.9047308033774186 ) ) ;
#23444=VERTEX_POINT ( 'NONE', #39108 ) ;
#23448=AXIS2_PLACEMENT_3D ( 'NONE', #16471, #12856, #9674 ) ;
#23449=DIRECTION ( 'NONE',  ( -0.000000000000000000, 1.259100132267607459E-16, -1.000000000000000000 ) ) ;
#23454=CARTESIAN_POINT ( 'NONE',  ( -1.655278471874999990, 20.36702641396248481, -26.93077246956613990 ) ) ;
#23455=ORIENTED_EDGE ( 'NONE', *, *, #37107, .T. ) ;
#23456=CARTESIAN_POINT ( 'NONE',  ( -1.750000000000002220, 14.46891108675448656, -109.4880641367107614 ) ) ;
#23461=VERTEX_POINT ( 'NONE', #23161 ) ;
#23465=FACE_OUTER_BOUND ( 'NONE', #12123, .T. ) ;
#23466=DIRECTION ( 'NONE',  ( 0.000000000000000000, 1.000000000000000000, 0.000000000000000000 ) ) ;
#23467=CARTESIAN_POINT ( 'NONE',  ( -3.500000000000001332, 17.50000000000001776, -74.96098080242151696 ) ) ;
#23468=CARTESIAN_POINT ( 'NONE',  ( -3.310556943750000425, 19.41135094264167549, -134.9349391362328277 ) ) ;
#23469=CARTESIAN_POINT ( 'NONE',  ( 1.750000000000001110, 20.53108891324554719, -30.29431413575484200 ) ) ;
#23471=CARTESIAN_POINT ( 'NONE',  ( -1.749999999999999778, 20.53108891324556140, -142.8213974700441042 ) ) ;
#23475=CARTESIAN_POINT ( 'NONE',  ( -3.500000000000002220, 15.47927405783633503, -133.8776474690881741 ) ) ;
#23476=CARTESIAN_POINT ( 'NONE',  ( -3.310556943750001313, 17.50000000000002132, -118.7641058028994792 ) ) ;
#23479=CARTESIAN_POINT ( 'NONE',  ( 0.000000000000000000, 17.50000000000002487, -149.5231586289125687 ) ) ;
#23480=CARTESIAN_POINT ( 'NONE',  ( 3.500000000000001776, 19.52072594216371115, -87.37764746908817415 ) ) ;
#23481=CARTESIAN_POINT ( 'NONE',  ( 4.648177544792955347E-16, 21.00000000000001776, -92.90473080337741862 ) ) ;
#23482=CARTESIAN_POINT ( 'NONE',  ( -1.655278471875002211, 14.63297358603754361, -55.59743913623280065 ) ) ;
#23483=CARTESIAN_POINT ( 'NONE',  ( 1.655278471875001101, 20.36702641396249547, -111.1849391362327992 ) ) ;
#23485=CARTESIAN_POINT ( 'NONE',  ( 1.750000000000001110, 20.53108891324554719, -27.98806413671076143 ) ) ;
#23488=CARTESIAN_POINT ( 'NONE',  ( 2.340729813953370519E-16, 21.32270188528331900, -128.1016058028994848 ) ) ;
#23489=VECTOR ( 'NONE', #30491, 1000.000000000000000 ) ;
#23492=CARTESIAN_POINT ( 'NONE',  ( 2.340729813953370519E-16, 21.32270188528330834, -63.10160580289946353 ) ) ;
#23494=CARTESIAN_POINT ( 'NONE',  ( -3.310556943750000425, 19.41135094264166128, -61.84743913623280065 ) ) ;
#23495=ORIENTED_EDGE ( 'NONE', *, *, #6136, .T. ) ;
#23496=CARTESIAN_POINT ( 'NONE',  ( -3.310556943750000425, 19.41135094264166838, -85.93493913623278502 ) ) ;
#23501=CARTESIAN_POINT ( 'NONE',  ( -3.310556943750001313, 17.50000000000001066, -46.76410580289947205 ) ) ;
#23504=CARTESIAN_POINT ( 'NONE',  ( 3.310556943750001313, 17.50000000000001776, -101.2641058028994792 ) ) ;
#23505=CARTESIAN_POINT ( 'NONE',  ( 1.749999999999998224, 14.46891108675447590, -53.32139747004409003 ) ) ;
#23506=ORIENTED_EDGE ( 'NONE', *, *, #16777, .T. ) ;
#23507=AXIS2_PLACEMENT_3D ( 'NONE', #18955, #31919, #26185 ) ;
#23509=ORIENTED_EDGE ( 'NONE', *, *, #11380, .T. ) ;
#23511=CARTESIAN_POINT ( 'NONE',  ( -1.655278471874999990, 20.36702641396248836, -54.93077246956613635 ) ) ;
#23512=ORIENTED_EDGE ( 'NONE', *, *, #11662, .F. ) ;
#23517=CARTESIAN_POINT ( 'NONE',  ( 4.286263797015737581E-16, 14.00000000000002487, -149.5231586289125687 ) ) ;
#23520=CARTESIAN_POINT ( 'NONE',  ( -3.500000000000002220, 15.47927405783632260, -44.87764746908818125 ) ) ;
#23521=CARTESIAN_POINT ( 'NONE',  ( -1.655278471875002211, 14.63297358603754184, -42.59743913623280065 ) ) ;
#23522=CARTESIAN_POINT ( 'NONE',  ( 7.367361408496833051E-14, 14.00000000000001776, -108.7109808024215027 ) ) ;
#23524=EDGE_CURVE ( 'NONE', #37080, #17995, #26996, .T. ) ;
#23525=CARTESIAN_POINT ( 'NONE',  ( 1.750000000000001110, 20.53108891324555785, -125.2943141357548456 ) ) ;
#23528=CARTESIAN_POINT ( 'NONE',  ( 3.310556943750001313, 19.41135094264165772, -31.26827246956613493 ) ) ;
#23529=CARTESIAN_POINT ( 'NONE',  ( 4.648177544792955347E-16, 21.00000000000001776, -97.90473080337743284 ) ) ;
#23530=CARTESIAN_POINT ( 'NONE',  ( 2.340729813953370519E-16, 21.32270188528331190, -85.10160580289947063 ) ) ;
#23531=CARTESIAN_POINT ( 'NONE',  ( 3.310556943750001313, 19.41135094264167549, -133.1807724695661364 ) ) ;
#23536=CARTESIAN_POINT ( 'NONE',  ( 3.310556943750001313, 19.41135094264166838, -126.2682724695661278 ) ) ;
#23538=CARTESIAN_POINT ( 'NONE',  ( 3.500000000000001332, 17.50000000000002487, -141.1547308033774186 ) ) ;
#23539=CARTESIAN_POINT ( 'NONE',  ( 3.310556943750001313, 17.50000000000001776, -86.26410580289947916 ) ) ;
#23541=CARTESIAN_POINT ( 'NONE',  ( 1.750000000000001110, 20.53108891324555429, -75.29431413575484555 ) ) ;
#23543=CARTESIAN_POINT ( 'NONE',  ( 1.749999999999998224, 14.46891108675447946, -74.32139747004410424 ) ) ;
#23544=CARTESIAN_POINT ( 'NONE',  ( 2.340729813953370519E-16, 21.32270188528331190, -57.10160580289946353 ) ) ;
#23548=CARTESIAN_POINT ( 'NONE',  ( 1.655278471874998436, 14.63297358603754361, -77.51827246956614204 ) ) ;
#23549=CARTESIAN_POINT ( 'NONE',  ( -3.310556943750001313, 17.50000000000002487, -138.8516058028994564 ) ) ;
#23551=CARTESIAN_POINT ( 'NONE',  ( -1.655278471874999990, 20.36702641396249547, -108.9307724695661506 ) ) ;
#23552=CARTESIAN_POINT ( 'NONE',  ( 3.310556943750001313, 19.41135094264166128, -74.18077246956613635 ) ) ;
#23553=ORIENTED_EDGE ( 'NONE', *, *, #40548, .T. ) ;
#23554=CARTESIAN_POINT ( 'NONE',  ( -1.655278471874999990, 20.36702641396249192, -100.0182724695661278 ) ) ;
#23555=CARTESIAN_POINT ( 'NONE',  ( 3.500000000000001332, 17.50000000000002132, -102.1547308033774186 ) ) ;
#23559=CARTESIAN_POINT ( 'NONE',  ( 1.750000000000001110, 20.53108891324555074, -57.98806413671076143 ) ) ;
#23561=CARTESIAN_POINT ( 'NONE',  ( 3.310556943750001313, 19.41135094264166483, -63.18077246956614346 ) ) ;
#23562=CARTESIAN_POINT ( 'NONE',  ( -3.500000000000000000, 19.52072594216371826, -113.0443141357548171 ) ) ;
#23563=CARTESIAN_POINT ( 'NONE',  ( -3.310556943750000425, 19.41135094264166838, -116.8474391362328078 ) ) ;
#23565=( BOUNDED_CURVE ( )  B_SPLINE_CURVE ( 2, ( #18431, #37787, #32028, #31190, #25453, #18645, #31398, #6080, #12039 ),
 .UNSPECIFIED., .F., .F. ) 
 B_SPLINE_CURVE_WITH_KNOTS ( ( 3, 2, 2, 2, 3 ),
 ( 0.9395833333333333259, 0.9402777777777777679, 0.9416666666666666519, 0.9430555555555555358, 0.9437499999999999778 ),
 .UNSPECIFIED. ) 
 CURVE ( )  GEOMETRIC_REPRESENTATION_ITEM ( )  RATIONAL_B_SPLINE_CURVE ( ( 0.9330127018922194093, 0.9330127018922194093, 1.000000000000000000, 0.8660254037844387076, 1.000000000000000000, 0.8660254037844387076, 1.000000000000000000, 0.9330127018922194093, 0.9330127018922194093 ) ) 
 REPRESENTATION_ITEM ( '' )  );
#23566=EDGE_CURVE ( 'NONE', #13587, #33623, #40761, .T. ) ;
#23569=( BOUNDED_CURVE ( )  B_SPLINE_CURVE ( 2, ( #20406, #17220, #4239, #6789, #19764, #23817, #30184, #7223, #194 ),
 .UNSPECIFIED., .F., .F. ) 
 B_SPLINE_CURVE_WITH_KNOTS ( ( 3, 2, 2, 2, 3 ),
 ( 0.5187500000000000444, 0.5194444444444444864, 0.5208333333333333703, 0.5222222222222222543, 0.5229166666666666963 ),
 .UNSPECIFIED. ) 
 CURVE ( )  GEOMETRIC_REPRESENTATION_ITEM ( )  RATIONAL_B_SPLINE_CURVE ( ( 0.9330127018922194093, 0.9330127018922194093, 1.000000000000000000, 0.8660254037844387076, 1.000000000000000000, 0.8660254037844387076, 1.000000000000000000, 0.9330127018922194093, 0.9330127018922194093 ) ) 
 REPRESENTATION_ITEM ( '' )  );
#23570=ORIENTED_EDGE ( 'NONE', *, *, #22560, .T. ) ;
#23573=CARTESIAN_POINT ( 'NONE',  ( -1.394453263437886604E-15, 14.00000000000001776, -89.71098080242148853 ) ) ;
#23574=CARTESIAN_POINT ( 'NONE',  ( -7.022189441860112050E-16, 13.67729811471672186, -70.51410580289947916 ) ) ;
#23575=VERTEX_POINT ( 'NONE', #8258 ) ;
#23577=DIRECTION ( 'NONE',  ( -0.000000000000000000, 1.259100132267607459E-16, -1.000000000000000000 ) ) ;
#23580=CARTESIAN_POINT ( 'NONE',  ( 3.310556943750001313, 17.50000000000002487, -138.2641058028994792 ) ) ;
#23582=CARTESIAN_POINT ( 'NONE',  ( 3.310556943749999981, 15.58864905735836182, -47.43493913623279923 ) ) ;
#23583=CARTESIAN_POINT ( 'NONE',  ( 0.9378221735089281585, 14.00000000000001066, -41.36007260463891555 ) ) ;
#23584=CARTESIAN_POINT ( 'NONE',  ( 1.655278471874998436, 14.63297358603753828, -39.51827246956612782 ) ) ;
#23585=CARTESIAN_POINT ( 'NONE',  ( -1.655278471875002211, 14.63297358603754894, -97.68493913623279923 ) ) ;
#23587=CARTESIAN_POINT ( 'NONE',  ( -3.310556943750001313, 17.50000000000001066, -24.76410580289947916 ) ) ;
#23589=CARTESIAN_POINT ( 'NONE',  ( -3.500000000000001332, 17.50000000000001776, -101.9609808024215170 ) ) ;
#23591=ADVANCED_FACE ( 'NONE', ( #8054 ), #4857, .T. ) ;
#23592=FACE_OUTER_BOUND ( 'NONE', #11467, .T. ) ;
#23593=CARTESIAN_POINT ( 'NONE',  ( -1.749999999999999778, 20.53108891324555429, -89.82139747004410424 ) ) ;
#23597=CARTESIAN_POINT ( 'NONE',  ( -1.394453263437886604E-15, 14.00000000000002132, -131.4047308033774186 ) ) ;
#23598=CARTESIAN_POINT ( 'NONE',  ( 3.500000000000001332, 17.50000000000001421, -51.46098080242150985 ) ) ;
#23600=CARTESIAN_POINT ( 'NONE',  ( -1.750000000000002220, 14.46891108675448834, -134.4880641367107614 ) ) ;
#23602=CARTESIAN_POINT ( 'NONE',  ( 3.500000000000000000, 15.47927405783632082, -42.23806413671075433 ) ) ;
#23604=CARTESIAN_POINT ( 'NONE',  ( 1.655278471875001101, 20.36702641396248481, -25.18493913623280633 ) ) ;
#23608=CARTESIAN_POINT ( 'NONE',  ( 0.9378221735089281585, 14.00000000000000888, -36.36007260463890844 ) ) ;
#23610=CARTESIAN_POINT ( 'NONE',  ( -3.310556943750000425, 19.41135094264166838, -74.84743913623280775 ) ) ;
#23611=CARTESIAN_POINT ( 'NONE',  ( -0.9378221735089310451, 14.00000000000002309, -133.7556390011600342 ) ) ;
#23613=CARTESIAN_POINT ( 'NONE',  ( -0.9378221735089310451, 14.00000000000002132, -97.75563900116003424 ) ) ;
#23614=EDGE_CURVE ( 'NONE', #33770, #12339, #33799, .T. ) ;
#23615=DIRECTION ( 'NONE',  ( -0.000000000000000000, 1.259100132267607459E-16, -1.000000000000000000 ) ) ;
#23618=CARTESIAN_POINT ( 'NONE',  ( 1.655278471874998436, 14.63297358603754539, -82.43077246956615056 ) ) ;
#23619=ORIENTED_EDGE ( 'NONE', *, *, #17839, .F. ) ;
#23620=ORIENTED_EDGE ( 'NONE', *, *, #29817, .T. ) ;
#23623=CARTESIAN_POINT ( 'NONE',  ( -1.394453263437886604E-15, 14.00000000000001421, -58.71098080242150985 ) ) ;
#23624=CARTESIAN_POINT ( 'NONE',  ( -3.310556943750000425, 19.41135094264166838, -124.8474391362328078 ) ) ;
#23625=ORIENTED_EDGE ( 'NONE', *, *, #22872, .F. ) ;
#23627=CARTESIAN_POINT ( 'NONE',  ( 3.310556943749999981, 15.58864905735836537, -55.43493913623281344 ) ) ;
#23628=CARTESIAN_POINT ( 'NONE',  ( 3.310556943750001313, 17.50000000000002132, -113.3516058028994564 ) ) ;
#23629=ORIENTED_EDGE ( 'NONE', *, *, #391, .T. ) ;
#23630=( BOUNDED_CURVE ( )  B_SPLINE_CURVE ( 2, ( #825, #26779, #39744, #10611, #33354, #11638, #18450, #8452, #31209 ),
 .UNSPECIFIED., .F., .F. ) 
 B_SPLINE_CURVE_WITH_KNOTS ( ( 3, 2, 2, 2, 3 ),
 ( 0.5770833333333332815, 0.5777777777777777235, 0.5791666666666667185, 0.5805555555555556024, 0.5812500000000000444 ),
 .UNSPECIFIED. ) 
 CURVE ( )  GEOMETRIC_REPRESENTATION_ITEM ( )  RATIONAL_B_SPLINE_CURVE ( ( 0.9330127018922194093, 0.9330127018922194093, 1.000000000000000000, 0.8660254037844387076, 1.000000000000000000, 0.8660254037844387076, 1.000000000000000000, 0.9330127018922194093, 0.9330127018922194093 ) ) 
 REPRESENTATION_ITEM ( '' )  );
#23631=EDGE_LOOP ( 'NONE', ( #36029, #19559, #8847, #4620 ) ) ;
#23632=CARTESIAN_POINT ( 'NONE',  ( -7.424026671074350129E-16, 13.45854811567264164, -126.4047308033774328 ) ) ;
#23633=CARTESIAN_POINT ( 'NONE',  ( -3.310556943750002645, 15.58864905735836714, -40.68077246956613635 ) ) ;
#23634=CARTESIAN_POINT ( 'NONE',  ( -1.655278471875002211, 14.63297358603754539, -67.68493913623279923 ) ) ;
#23635=CARTESIAN_POINT ( 'NONE',  ( 3.500000000000000000, 15.47927405783632970, -117.5443141357548171 ) ) ;
#23637=CARTESIAN_POINT ( 'NONE',  ( 1.655278471875001101, 20.36702641396249547, -103.0974391362328220 ) ) ;
#23638=CARTESIAN_POINT ( 'NONE',  ( 0.9378221735089281585, 14.00000000000002132, -98.36007260463891555 ) ) ;
#23642=CARTESIAN_POINT ( 'NONE',  ( 3.500000000000001776, 19.52072594216370760, -72.37764746908818836 ) ) ;
#23644=CARTESIAN_POINT ( 'NONE',  ( 0.9378221735089300459, 21.00000000000002132, -122.2556390011600485 ) ) ;
#23645=CARTESIAN_POINT ( 'NONE',  ( 1.655278471875001101, 20.36702641396248481, -39.09743913623281486 ) ) ;
#23646=CARTESIAN_POINT ( 'NONE',  ( -1.655278471875002211, 14.63297358603754716, -93.68493913623279923 ) ) ;
#23647=CARTESIAN_POINT ( 'NONE',  ( -1.750000000000002220, 14.46891108675447946, -58.48806413671076143 ) ) ;
#23649=CARTESIAN_POINT ( 'NONE',  ( -1.655278471875002211, 14.63297358603755072, -112.6849391362327992 ) ) ;
#23650=CARTESIAN_POINT ( 'NONE',  ( 3.310556943750001313, 17.50000000000001066, -44.35160580289947063 ) ) ;
#23653=EDGE_CURVE ( 'NONE', #4297, #12140, #30599, .T. ) ;
#23658=CARTESIAN_POINT ( 'NONE',  ( -7.022189441860112050E-16, 13.67729811471672363, -91.51410580289947916 ) ) ;
#23659=CARTESIAN_POINT ( 'NONE',  ( 1.749999999999998224, 14.46891108675447413, -39.32139747004409713 ) ) ;
#23662=ORIENTED_EDGE ( 'NONE', *, *, #26195, .F. ) ;
#23665=CARTESIAN_POINT ( 'NONE',  ( 1.749999999999998224, 14.46891108675447590, -46.62764746908818125 ) ) ;
#23666=ORIENTED_EDGE ( 'NONE', *, *, #30589, .T. ) ;
#23669=CARTESIAN_POINT ( 'NONE',  ( 3.310556943750001313, 17.50000000000001066, -28.26410580289947916 ) ) ;
#23670=EDGE_LOOP ( 'NONE', ( #20724, #41518, #27840, #22663 ) ) ;
#23675=ORIENTED_EDGE ( 'NONE', *, *, #39420, .T. ) ;
#23676=CARTESIAN_POINT ( 'NONE',  ( 4.648177544792955347E-16, 21.00000000000001066, -27.90473080337742928 ) ) ;
#23678=CARTESIAN_POINT ( 'NONE',  ( 1.655278471874998436, 14.63297358603755249, -142.4307724695661364 ) ) ;
#23679=CARTESIAN_POINT ( 'NONE',  ( -1.749999999999999778, 20.53108891324555429, -81.12764746908818836 ) ) ;
#23681=CARTESIAN_POINT ( 'NONE',  ( -1.394453263437886604E-15, 14.00000000000001421, -74.71098080242151696 ) ) ;
#23682=CARTESIAN_POINT ( 'NONE',  ( 3.310556943750001313, 17.50000000000002487, -131.3516058028994564 ) ) ;
#23683=CARTESIAN_POINT ( 'NONE',  ( 2.474675557024783212E-16, 21.54145188432739033, -27.21098080242151696 ) ) ;
#23685=CARTESIAN_POINT ( 'NONE',  ( 1.750000000000001110, 20.53108891324556140, -140.9880641367107614 ) ) ;
#23688=CARTESIAN_POINT ( 'NONE',  ( 1.750000000000001110, 20.53108891324556140, -131.2943141357548598 ) ) ;
#23689=CARTESIAN_POINT ( 'NONE',  ( -1.655278471875002211, 14.63297358603755072, -116.5974391362327935 ) ) ;
#23691=LINE ( 'NONE', #33242, #31340 ) ;
#23692=CARTESIAN_POINT ( 'NONE',  ( 3.500000000000001332, 17.50000000000001776, -83.46098080242150274 ) ) ;
#23694=CARTESIAN_POINT ( 'NONE',  ( -3.500000000000002220, 15.47927405783632970, -92.57139747004409003 ) ) ;
#23695=CARTESIAN_POINT ( 'NONE',  ( -7.022189441860112050E-16, 13.67729811471671653, -51.51410580289947916 ) ) ;
#23696=CARTESIAN_POINT ( 'NONE',  ( -3.310556943750000425, 19.41135094264166838, -111.9349391362327992 ) ) ;
#23700=CARTESIAN_POINT ( 'NONE',  ( -1.655278471875002211, 14.63297358603755249, -128.6849391362327992 ) ) ;
#23701=ADVANCED_FACE ( 'NONE', ( #40795 ), #24229, .T. ) ;
#23704=CARTESIAN_POINT ( 'NONE',  ( 3.500000000000001332, 19.52072594216371115, -86.07139747004409003 ) ) ;
#23705=CARTESIAN_POINT ( 'NONE',  ( -1.655278471874999990, 20.36702641396248836, -65.01827246956614204 ) ) ;
#23708=CARTESIAN_POINT ( 'NONE',  ( 1.655278471874998436, 14.63297358603754361, -79.51827246956614204 ) ) ;
#23713=CARTESIAN_POINT ( 'NONE',  ( -3.310556943750000425, 19.41135094264166128, -45.84743913623280775 ) ) ;
#23714=CARTESIAN_POINT ( 'NONE',  ( 2.340729813953370519E-16, 21.32270188528331900, -102.0141058028994649 ) ) ;
#23715=CARTESIAN_POINT ( 'NONE',  ( -1.394453263437886604E-15, 14.00000000000000711, -24.40473080337742928 ) ) ;
#23716=ORIENTED_EDGE ( 'NONE', *, *, #22527, .T. ) ;
#23718=ORIENTED_EDGE ( 'NONE', *, *, #40810, .T. ) ;
#23720=CARTESIAN_POINT ( 'NONE',  ( 2.340729813953370519E-16, 21.32270188528330834, -52.01410580289947205 ) ) ;
#23722=ORIENTED_EDGE ( 'NONE', *, *, #30557, .F. ) ;
#23724=CYLINDRICAL_SURFACE ( 'NONE', #38217, 3.499999999999999556 ) ;
#23725=CARTESIAN_POINT ( 'NONE',  ( 4.648177544792955347E-16, 21.00000000000001776, -91.90473080337741862 ) ) ;
#23727=FACE_OUTER_BOUND ( 'NONE', #583, .T. ) ;
#23730=CARTESIAN_POINT ( 'NONE',  ( 1.750000000000001110, 20.53108891324554719, -45.29431413575483845 ) ) ;
#23731=CARTESIAN_POINT ( 'NONE',  ( -3.500000000000002220, 15.47927405783633503, -133.5713974700441042 ) ) ;
#23734=CARTESIAN_POINT ( 'NONE',  ( 3.310556943749999981, 15.58864905735836182, -31.43493913623279923 ) ) ;
#23736=CARTESIAN_POINT ( 'NONE',  ( 3.310556943750001313, 17.50000000000001776, -82.35160580289945642 ) ) ;
#23737=CARTESIAN_POINT ( 'NONE',  ( -7.022189441860112050E-16, 13.67729811471672718, -131.5141058028994507 ) ) ;
#23740=CARTESIAN_POINT ( 'NONE',  ( -1.655278471874999990, 20.36702641396249547, -126.0182724695661278 ) ) ;
#23742=CARTESIAN_POINT ( 'NONE',  ( -1.655278471874999990, 20.36702641396249192, -85.93077246956613635 ) ) ;
#23743=CARTESIAN_POINT ( 'NONE',  ( 3.500000000000000000, 15.47927405783631727, -24.54431413575484910 ) ) ;
#23745=CARTESIAN_POINT ( 'NONE',  ( 3.500000000000001332, 19.52072594216371115, -89.07139747004409003 ) ) ;
#23746=CARTESIAN_POINT ( 'NONE',  ( -3.500000000000002220, 15.47927405783632615, -69.57139747004409003 ) ) ;
#23747=CARTESIAN_POINT ( 'NONE',  ( 3.310556943749999981, 15.58864905735836182, -51.43493913623279212 ) ) ;
#23748=( BOUNDED_CURVE ( )  B_SPLINE_CURVE ( 2, ( #10475, #26430, #36196, #26640, #9860, #33011, #23456, #54, #39177 ),
 .UNSPECIFIED., .F., .T. ) 
 B_SPLINE_CURVE_WITH_KNOTS ( ( 3, 2, 2, 2, 3 ),
 ( 0.2770833333333333481, 0.2777777777777777901, 0.2791666666666666741, 0.2805555555555555580, 0.2812500000000000000 ),
 .UNSPECIFIED. ) 
 CURVE ( )  GEOMETRIC_REPRESENTATION_ITEM ( )  RATIONAL_B_SPLINE_CURVE ( ( 0.9330127018922194093, 0.9330127018922194093, 1.000000000000000000, 0.8660254037844387076, 1.000000000000000000, 0.8660254037844387076, 1.000000000000000000, 0.9330127018922194093, 0.9330127018922194093 ) ) 
 REPRESENTATION_ITEM ( '' )  );
#23750=CARTESIAN_POINT ( 'NONE',  ( 1.749999999999998224, 14.46891108675448834, -137.6276474690881741 ) ) ;
#23752=CARTESIAN_POINT ( 'NONE',  ( 2.340729813953370519E-16, 21.32270188528331190, -82.10160580289945642 ) ) ;
#23753=CARTESIAN_POINT ( 'NONE',  ( -3.310556943750000425, 19.41135094264167549, -141.9349391362327708 ) ) ;
#23754=AXIS2_PLACEMENT_3D ( 'NONE', #18255, #1473, #18052 ) ;
#23756=CARTESIAN_POINT ( 'NONE',  ( 3.310556943750001313, 19.41135094264166838, -111.1807724695661506 ) ) ;
#23757=CARTESIAN_POINT ( 'NONE',  ( -3.310556943750002645, 15.58864905735837070, -73.68077246956615056 ) ) ;
#23758=ORIENTED_EDGE ( 'NONE', *, *, #21673, .T. ) ;
#23759=CARTESIAN_POINT ( 'NONE',  ( -3.310556943750000425, 19.41135094264166838, -95.93493913623279923 ) ) ;
#23760=CARTESIAN_POINT ( 'NONE',  ( -3.500000000000001332, 17.50000000000001776, -101.6547308033774328 ) ) ;
#23762=DIRECTION ( 'NONE',  ( 0.000000000000000000, 1.000000000000000000, 0.000000000000000000 ) ) ;
#23763=CARTESIAN_POINT ( 'NONE',  ( -0.9378221735089291577, 21.00000000000001776, -81.86007260463891555 ) ) ;
#23765=CARTESIAN_POINT ( 'NONE',  ( 3.310556943750001313, 19.41135094264166483, -59.18077246956614346 ) ) ;
#23766=CARTESIAN_POINT ( 'NONE',  ( -1.394453263437886604E-15, 14.00000000000002132, -109.7109808024215170 ) ) ;
#23767=CARTESIAN_POINT ( 'NONE',  ( -7.022189441860112050E-16, 13.67729811471672718, -114.5141058028994792 ) ) ;
#23772=EDGE_CURVE ( 'NONE', #22667, #6296, #21234, .T. ) ;
#23775=CARTESIAN_POINT ( 'NONE',  ( 3.500000000000001332, 17.50000000000002487, -131.1547308033774186 ) ) ;
#23777=CARTESIAN_POINT ( 'NONE',  ( 1.655278471874998436, 14.63297358603754361, -68.43077246956613635 ) ) ;
#23778=VERTEX_POINT ( 'NONE', #41223 ) ;
#23779=EDGE_LOOP ( 'NONE', ( #14628, #21833, #41882, #29031 ) ) ;
#23781=CARTESIAN_POINT ( 'NONE',  ( 3.500000000000001332, 17.50000000000001776, -83.46098080242150274 ) ) ;
#23785=ORIENTED_EDGE ( 'NONE', *, *, #40502, .T. ) ;
#23786=CARTESIAN_POINT ( 'NONE',  ( -1.655278471874999990, 20.36702641396249902, -137.9307724695661364 ) ) ;
#23787=VECTOR ( 'NONE', #22270, 1000.000000000000000 ) ;
#23788=CARTESIAN_POINT ( 'NONE',  ( -0.9378221735089291577, 21.00000000000002487, -131.8600726046389013 ) ) ;
#23789=CARTESIAN_POINT ( 'NONE',  ( -1.655278471875002211, 14.63297358603754184, -45.68493913623279923 ) ) ;
#23790=CARTESIAN_POINT ( 'NONE',  ( 3.500000000000000000, 15.47927405783633503, -134.5443141357548598 ) ) ;
#23791=CARTESIAN_POINT ( 'NONE',  ( -3.310556943750001313, 17.50000000000001066, -38.85160580289946353 ) ) ;
#23792=CARTESIAN_POINT ( 'NONE',  ( 1.655278471875001101, 20.36702641396249192, -99.18493913623279923 ) ) ;
#23796=EDGE_CURVE ( 'NONE', #29770, #13398, #26121, .T. ) ;
#23797=CARTESIAN_POINT ( 'NONE',  ( -3.310556943750000425, 19.41135094264165772, -25.84743913623280065 ) ) ;
#23799=CARTESIAN_POINT ( 'NONE',  ( 3.500000000000001332, 17.50000000000001776, -100.4609808024215027 ) ) ;
#23802=CARTESIAN_POINT ( 'NONE',  ( 1.749999999999998224, 14.46891108675448123, -92.32139747004409003 ) ) ;
#23803=CARTESIAN_POINT ( 'NONE',  ( 3.310556943750001313, 19.41135094264166483, -68.26827246956612782 ) ) ;
#23807=CARTESIAN_POINT ( 'NONE',  ( 3.500000000000001332, 17.50000000000002132, -110.4609808024215027 ) ) ;
#23808=CARTESIAN_POINT ( 'NONE',  ( -1.750000000000002220, 14.46891108675447768, -52.79431413575484555 ) ) ;
#23809=FACE_OUTER_BOUND ( 'NONE', #14777, .T. ) ;
#23811=( BOUNDED_CURVE ( )  B_SPLINE_CURVE ( 2, ( #25971, #35321, #22343, #35744, #5974, #38933, #6184, #16399, #9 ),
 .UNSPECIFIED., .F., .F. ) 
 B_SPLINE_CURVE_WITH_KNOTS ( ( 3, 2, 2, 2, 3 ),
 ( 0.4854166666666666630, 0.4861111111111111049, 0.4874999999999999889, 0.4888888888888888729, 0.4895833333333333148 ),
 .UNSPECIFIED. ) 
 CURVE ( )  GEOMETRIC_REPRESENTATION_ITEM ( )  RATIONAL_B_SPLINE_CURVE ( ( 0.9330127018922194093, 0.9330127018922194093, 1.000000000000000000, 0.8660254037844387076, 1.000000000000000000, 0.8660254037844387076, 1.000000000000000000, 0.9330127018922194093, 0.9330127018922194093 ) ) 
 REPRESENTATION_ITEM ( '' )  );
#23812=DIRECTION ( 'NONE',  ( -0.000000000000000000, 1.259100132267607459E-16, -1.000000000000000000 ) ) ;
#23814=CARTESIAN_POINT ( 'NONE',  ( -3.500000000000000888, 19.52072594216370405, -43.73806413671076143 ) ) ;
#23815=CARTESIAN_POINT ( 'NONE',  ( 0.9378221735089281585, 14.00000000000001243, -55.36007260463890844 ) ) ;
#23816=CARTESIAN_POINT ( 'NONE',  ( -3.310556943750001313, 17.50000000000001066, -27.85160580289947063 ) ) ;
#23817=CARTESIAN_POINT ( 'NONE',  ( -3.500000000000002220, 15.47927405783632793, -80.57139747004410424 ) ) ;
#23820=CARTESIAN_POINT ( 'NONE',  ( -3.500000000000002220, 15.47927405783633326, -106.8776474690881884 ) ) ;
#23822=CARTESIAN_POINT ( 'NONE',  ( -1.655278471874999990, 20.36702641396249192, -78.93077246956615056 ) ) ;
#23823=CARTESIAN_POINT ( 'NONE',  ( -1.394453263437886604E-15, 14.00000000000001776, -98.71098080242150274 ) ) ;
#23825=ORIENTED_EDGE ( 'NONE', *, *, #15287, .F. ) ;
#23826=DIRECTION ( 'NONE',  ( -0.000000000000000000, 1.259100132267607459E-16, -1.000000000000000000 ) ) ;
#23829=ORIENTED_EDGE ( 'NONE', *, *, #25320, .T. ) ;
#23831=CARTESIAN_POINT ( 'NONE',  ( 3.310556943749999981, 15.58864905735836892, -86.34743913623279354 ) ) ;
#23833=VERTEX_POINT ( 'NONE', #2504 ) ;
#23838=CARTESIAN_POINT ( 'NONE',  ( 1.655278471875001101, 20.36702641396249547, -126.0974391362328078 ) ) ;
#23839=CARTESIAN_POINT ( 'NONE',  ( 3.500000000000001332, 17.50000000000001421, -64.15473080337743284 ) ) ;
#23840=CARTESIAN_POINT ( 'NONE',  ( -1.655278471874999990, 20.36702641396248836, -56.01827246956612782 ) ) ;
#23841=CARTESIAN_POINT ( 'NONE',  ( -3.310556943750000425, 19.41135094264166838, -113.9349391362327850 ) ) ;
#23845=CARTESIAN_POINT ( 'NONE',  ( 3.500000000000001776, 19.52072594216371826, -124.0713974700440758 ) ) ;
#23847=EDGE_CURVE ( 'NONE', #15095, #8756, #38021, .T. ) ;
#23849=CARTESIAN_POINT ( 'NONE',  ( 3.310556943750001313, 19.41135094264165772, -40.18077246956614346 ) ) ;
#23850=CARTESIAN_POINT ( 'NONE',  ( 3.310556943750001313, 17.50000000000001421, -67.35160580289947063 ) ) ;
#23851=CARTESIAN_POINT ( 'NONE',  ( 1.749999999999998224, 14.46891108675448478, -119.6276474690881741 ) ) ;
#23852=CARTESIAN_POINT ( 'NONE',  ( 2.340729813953370519E-16, 21.32270188528331900, -102.0141058028994649 ) ) ;
#23853=CARTESIAN_POINT ( 'NONE',  ( 0.000000000000000000, 17.50000000000002487, -149.5231586289125687 ) ) ;
#23855=CARTESIAN_POINT ( 'NONE',  ( 4.286263797015737581E-16, 14.00000000000002487, -149.5231586289125687 ) ) ;
#23857=CARTESIAN_POINT ( 'NONE',  ( 3.500000000000001332, 17.50000000000001421, -72.46098080242151696 ) ) ;
#23859=CARTESIAN_POINT ( 'NONE',  ( -3.310556943750000425, 19.41135094264165772, -31.84743913623280420 ) ) ;
#23860=VECTOR ( 'NONE', #2645, 1000.000000000000114 ) ;
#23861=CARTESIAN_POINT ( 'NONE',  ( 3.310556943749999981, 15.58864905735836892, -90.43493913623278502 ) ) ;
#23862=CARTESIAN_POINT ( 'NONE',  ( -7.424026671074350129E-16, 13.45854811567263454, -57.40473080337743284 ) ) ;
#23863=DIRECTION ( 'NONE',  ( -0.000000000000000000, 1.259100132267607459E-16, -1.000000000000000000 ) ) ;
#23864=CARTESIAN_POINT ( 'NONE',  ( -3.310556943750002201, 15.58864905735837780, -113.7682724695661420 ) ) ;
#23865=CARTESIAN_POINT ( 'NONE',  ( 3.310556943750001313, 17.50000000000001066, -43.35160580289947063 ) ) ;
#23867=CARTESIAN_POINT ( 'NONE',  ( 3.500000000000001332, 17.50000000000002132, -127.4609808024215170 ) ) ;
#23872=CARTESIAN_POINT ( 'NONE',  ( 1.655278471874998436, 14.63297358603754539, -92.43077246956613635 ) ) ;
#23875=EDGE_LOOP ( 'NONE', ( #12411, #8728, #7973, #24108 ) ) ;
#23876=FACE_OUTER_BOUND ( 'NONE', #26422, .T. ) ;
#23881=VERTEX_POINT ( 'NONE', #24855 ) ;
#23882=CARTESIAN_POINT ( 'NONE',  ( 0.9378221735089300459, 21.00000000000002132, -117.9493890021159501 ) ) ;
#23886=ADVANCED_FACE ( 'NONE', ( #2713 ), #34415, .T. ) ;
#23891=CARTESIAN_POINT ( 'NONE',  ( -1.394453263437886604E-15, 14.00000000000001776, -98.71098080242150274 ) ) ;
#23893=CARTESIAN_POINT ( 'NONE',  ( -3.310556943750002645, 15.58864905735837958, -142.6807724695661364 ) ) ;
#23894=CARTESIAN_POINT ( 'NONE',  ( 0.9378221735089630196, 14.00000000000004086, -110.3600726046389013 ) ) ;
#23896=CARTESIAN_POINT ( 'NONE',  ( -1.750000000000002220, 14.46891108675448123, -74.79431413575484555 ) ) ;
#23897=CARTESIAN_POINT ( 'NONE',  ( 1.655278471874998436, 14.63297358603755072, -132.5182724695661420 ) ) ;
#23898=CARTESIAN_POINT ( 'NONE',  ( 3.500000000000000000, 15.47927405783632082, -29.54431413575483845 ) ) ;
#23900=CARTESIAN_POINT ( 'NONE',  ( -3.500000000000000888, 19.52072594216372181, -139.7380641367107330 ) ) ;
#23902=CARTESIAN_POINT ( 'NONE',  ( -3.500000000000002220, 15.47927405783633503, -135.8776474690881741 ) ) ;
#23903=CARTESIAN_POINT ( 'NONE',  ( 2.340729813953370519E-16, 21.32270188528331900, -117.0141058028994792 ) ) ;
#23906=CARTESIAN_POINT ( 'NONE',  ( -1.749999999999999778, 20.53108891324555429, -85.12764746908817415 ) ) ;
#23908=CARTESIAN_POINT ( 'NONE',  ( 2.340729813953370519E-16, 21.32270188528330834, -56.01410580289947916 ) ) ;
#23909=CARTESIAN_POINT ( 'NONE',  ( -7.022189441860112050E-16, 13.67729811471672541, -107.6016058028994706 ) ) ;
#23913=CARTESIAN_POINT ( 'NONE',  ( 3.310556943750001313, 19.41135094264166838, -129.2682724695661136 ) ) ;
#23916=CARTESIAN_POINT ( 'NONE',  ( 0.9378221735089300459, 21.00000000000001066, -27.25563900116002714 ) ) ;
#23917=LINE ( 'NONE', #27098, #22 ) ;
#23918=CARTESIAN_POINT ( 'NONE',  ( -3.310556943750001313, 17.50000000000001421, -63.85160580289946353 ) ) ;
#23920=AXIS2_PLACEMENT_3D ( 'NONE', #24583, #21799, #5003 ) ;
#23921=CARTESIAN_POINT ( 'NONE',  ( -3.310556943750000425, 19.41135094264166838, -82.93493913623278502 ) ) ;
#23926=CARTESIAN_POINT ( 'NONE',  ( 1.655278471875001101, 20.36702641396248481, -45.09743913623280775 ) ) ;
#23927=CARTESIAN_POINT ( 'NONE',  ( 1.655278471875001101, 20.36702641396249192, -101.0974391362328078 ) ) ;
#23932=ORIENTED_EDGE ( 'NONE', *, *, #40777, .T. ) ;
#23935=CARTESIAN_POINT ( 'NONE',  ( -7.022189441860112050E-16, 13.67729811471671653, -53.51410580289947205 ) ) ;
#23937=AXIS2_PLACEMENT_3D ( 'NONE', #34110, #4967, #24760 ) ;
#23940=( BOUNDED_CURVE ( )  B_SPLINE_CURVE ( 2, ( #32738, #3605, #16597, #29552, #26373, #25540, #417, #35308, #6172 ),
 .UNSPECIFIED., .F., .F. ) 
 B_SPLINE_CURVE_WITH_KNOTS ( ( 3, 2, 2, 2, 3 ),
 ( 0.8937500000000000444, 0.8944444444444444864, 0.8958333333333333703, 0.8972222222222222543, 0.8979166666666666963 ),
 .UNSPECIFIED. ) 
 CURVE ( )  GEOMETRIC_REPRESENTATION_ITEM ( )  RATIONAL_B_SPLINE_CURVE ( ( 0.9330127018922194093, 0.9330127018922194093, 1.000000000000000000, 0.8660254037844387076, 1.000000000000000000, 0.8660254037844387076, 1.000000000000000000, 0.9330127018922194093, 0.9330127018922194093 ) ) 
 REPRESENTATION_ITEM ( '' )  );
#23941=CARTESIAN_POINT ( 'NONE',  ( 4.648177544792955347E-16, 21.00000000000002132, -105.9047308033774186 ) ) ;
#23943=DIRECTION ( 'NONE',  ( -0.000000000000000000, 1.259100132267607459E-16, -1.000000000000000000 ) ) ;
#23945=ORIENTED_EDGE ( 'NONE', *, *, #2536, .T. ) ;
#23946=CARTESIAN_POINT ( 'NONE',  ( -1.750000000000002220, 14.46891108675447768, -45.79431413575483845 ) ) ;
#23948=ORIENTED_EDGE ( 'NONE', *, *, #31176, .F. ) ;
#23949=CYLINDRICAL_SURFACE ( 'NONE', #25764, 3.499999999999999556 ) ;
#23951=CARTESIAN_POINT ( 'NONE',  ( 2.340729813953370519E-16, 21.32270188528330479, -31.10160580289945642 ) ) ;
#23952=CARTESIAN_POINT ( 'NONE',  ( -1.749999999999999778, 20.53108891324555074, -53.12764746908817415 ) ) ;
#23953=CARTESIAN_POINT ( 'NONE',  ( 3.310556943750001313, 19.41135094264166483, -83.26827246956614204 ) ) ;
#23954=CARTESIAN_POINT ( 'NONE',  ( -3.310556943750000425, 19.41135094264167549, -135.8474391362328220 ) ) ;
#23958=CARTESIAN_POINT ( 'NONE',  ( -7.022189441860112050E-16, 13.67729811471672718, -128.6016058028994848 ) ) ;
#23959=CARTESIAN_POINT ( 'NONE',  ( -1.750000000000002220, 14.46891108675448123, -68.79431413575484555 ) ) ;
#23960=CARTESIAN_POINT ( 'NONE',  ( 2.340729813953370519E-16, 21.32270188528331190, -87.01410580289947916 ) ) ;
#23962=DIRECTION ( 'NONE',  ( -0.000000000000000000, 1.259100132267607459E-16, -1.000000000000000000 ) ) ;
#23963=CARTESIAN_POINT ( 'NONE',  ( 3.500000000000001332, 17.50000000000001776, -101.1547308033774328 ) ) ;
#23964=CARTESIAN_POINT ( 'NONE',  ( 3.500000000000001332, 19.52072594216370760, -67.07139747004409003 ) ) ;
#23965=CARTESIAN_POINT ( 'NONE',  ( 3.500000000000001332, 17.50000000000001421, -69.15473080337743284 ) ) ;
#23967=CARTESIAN_POINT ( 'NONE',  ( 2.340729813953370519E-16, 21.32270188528331190, -55.10160580289947063 ) ) ;
#23969=CARTESIAN_POINT ( 'NONE',  ( -3.500000000000000000, 19.52072594216370760, -67.73806413671076143 ) ) ;
#23970=CARTESIAN_POINT ( 'NONE',  ( -3.500000000000002220, 15.47927405783632437, -48.87764746908818125 ) ) ;
#23972=CARTESIAN_POINT ( 'NONE',  ( 1.655278471875001101, 20.36702641396249192, -80.18493913623279923 ) ) ;
#23973=CARTESIAN_POINT ( 'NONE',  ( -7.022189441860112050E-16, 13.67729811471672896, -142.6016058028994564 ) ) ;
#23975=CARTESIAN_POINT ( 'NONE',  ( -1.655278471874999990, 20.36702641396249192, -101.9307724695661364 ) ) ;
#23976=CARTESIAN_POINT ( 'NONE',  ( 1.655278471874998436, 14.63297358603754361, -74.43077246956613635 ) ) ;
#23978=CARTESIAN_POINT ( 'NONE',  ( 3.310556943750001313, 19.41135094264166838, -95.26827246956612782 ) ) ;
#23979=CARTESIAN_POINT ( 'NONE',  ( 3.500000000000000000, 15.47927405783632793, -100.2380641367107756 ) ) ;
#23981=DIRECTION ( 'NONE',  ( -0.000000000000000000, 1.259100132267607459E-16, -1.000000000000000000 ) ) ;
#23982=CARTESIAN_POINT ( 'NONE',  ( 4.648177544792955347E-16, 21.00000000000001066, -26.21098080242150985 ) ) ;
#23984=CARTESIAN_POINT ( 'NONE',  ( -3.310556943750000425, 19.41135094264166483, -58.84743913623280065 ) ) ;
#23986=CARTESIAN_POINT ( 'NONE',  ( 3.310556943750001313, 19.41135094264166838, -114.1807724695661364 ) ) ;
#23987=LINE ( 'NONE', #7597, #20987 ) ;
#23990=VERTEX_POINT ( 'NONE', #14505 ) ;
#23992=CARTESIAN_POINT ( 'NONE',  ( 3.500000000000000000, 15.47927405783633503, -131.2380641367107614 ) ) ;
#23994=CARTESIAN_POINT ( 'NONE',  ( -3.310556943750001313, 17.50000000000001421, -67.76410580289947916 ) ) ;
#23995=VERTEX_POINT ( 'NONE', #7914 ) ;
#23996=ORIENTED_EDGE ( 'NONE', *, *, #34698, .F. ) ;
#23998=LINE ( 'NONE', #8230, #41205 ) ;
#24005=CARTESIAN_POINT ( 'NONE',  ( -1.655278471875002211, 14.63297358603755249, -134.5974391362328220 ) ) ;
#24007=CARTESIAN_POINT ( 'NONE',  ( -3.310556943750001313, 17.50000000000001066, -43.85160580289947063 ) ) ;
#24009=CARTESIAN_POINT ( 'NONE',  ( 3.310556943749999981, 15.58864905735836182, -37.43493913623280633 ) ) ;
#24010=CARTESIAN_POINT ( 'NONE',  ( -3.310556943750000425, 19.41135094264166483, -95.93493913623279923 ) ) ;
#24011=( BOUNDED_CURVE ( )  B_SPLINE_CURVE ( 2, ( #6642, #3654, #10049, #13030, #6847, #20250, #16231, #39378, #19818 ),
 .UNSPECIFIED., .F., .T. ) 
 B_SPLINE_CURVE_WITH_KNOTS ( ( 3, 2, 2, 2, 3 ),
 ( 0.6020833333333333037, 0.6027777777777777457, 0.6041666666666666297, 0.6055555555555555136, 0.6062499999999999556 ),
 .UNSPECIFIED. ) 
 CURVE ( )  GEOMETRIC_REPRESENTATION_ITEM ( )  RATIONAL_B_SPLINE_CURVE ( ( 0.9330127018922194093, 0.9330127018922194093, 1.000000000000000000, 0.8660254037844387076, 1.000000000000000000, 0.8660254037844387076, 1.000000000000000000, 0.9330127018922194093, 0.9330127018922194093 ) ) 
 REPRESENTATION_ITEM ( '' )  );
#24013=CARTESIAN_POINT ( 'NONE',  ( 2.340729813953370519E-16, 21.32270188528330479, -26.01410580289947916 ) ) ;
#24014=CARTESIAN_POINT ( 'NONE',  ( 1.750000000000001110, 20.53108891324555429, -95.29431413575484555 ) ) ;
#24015=CARTESIAN_POINT ( 'NONE',  ( 3.500000000000001332, 17.50000000000002132, -124.4609808024215027 ) ) ;
#24016=CARTESIAN_POINT ( 'NONE',  ( 3.500000000000000000, 15.47927405783632615, -88.23806413671076143 ) ) ;
#24017=CARTESIAN_POINT ( 'NONE',  ( 1.655278471875001101, 20.36702641396248836, -69.18493913623279923 ) ) ;
#24020=CARTESIAN_POINT ( 'NONE',  ( 0.9378221735089630196, 14.00000000000004086, -110.6663226036829855 ) ) ;
#24021=CARTESIAN_POINT ( 'NONE',  ( 1.749999999999998224, 14.46891108675447590, -49.62764746908818125 ) ) ;
#24022=CARTESIAN_POINT ( 'NONE',  ( -0.9378221735089310451, 14.00000000000001066, -30.44938900211595012 ) ) ;
#24024=CARTESIAN_POINT ( 'NONE',  ( 1.750000000000001110, 20.53108891324555785, -103.2943141357548456 ) ) ;
#24025=EDGE_LOOP ( 'NONE', ( #5, #17338, #30070, #38285 ) ) ;
#24026=CARTESIAN_POINT ( 'NONE',  ( -1.749999999999999778, 20.53108891324555785, -114.8213974700440900 ) ) ;
#24028=CLOSED_SHELL ( 'NONE', ( #27955, #15493, #8694, #33282, #36892, #35534, #27904, #156, #12876, #27412, #15609, #30041, #30072, #18927, #2463, #6364, #34694, #32707, #14427, #4614, #12077, #1975, #32172, #8787, #28339, #12096, #21863, #38125, #40977, #13361, #23351, #7253, #14474, #2988, #30100, #13452, #22808, #25910, #36889, #27590, #2532, #37365, #4908, #9327, #23591, #34523, #39523, #21716, #15297, #35884, #34438, #13702, #7865, #31086, #34297, #648, #34942, #21002, #3079, #33661, #32624, #26144, #35708, #28682, #15349, #3810, #29200, #19174, #6255, #33681, #17459, #33263, #26973, #41507, #21471, #22770, #39104, #24830, #18067, #36107, #30287, #10025, #35477, #2514, #13887, #39285, #10594, #16631, #2208, #27100, #22003, #40401, #10385, #16598, #12344, #20215, #36687, #40253, #35280, #39256, #24799, #19781, #38701, #26140, #34005, #7761, #35057, #3783, #9823, #2318, #12404, #16617, #11721, #40533, #11165, #38319, #26050, #37844, #35260, #31047, #25083, #30795, #31783, #14917, #29876, #29388, #3181, #38052, #35754, #41257, #41719, #2696, #8955, #7497, #8260, #1406, #38740, #13988, #15252, #2104, #17223, #14191, #14310, #6349, #15816, #41343, #31319, #21768, #26295, #28455, #6505, #17286, #7021, #39403, #4041, #36600, #4342, #10324, #23701, #34489, #26933, #35817, #36322, #23360, #371, #31659, #28976, #11463, #4618, #8107, #3846, #19613, #35742, #10055, #22928, #176, #17413, #15720, #19417, #13380, #17605, #33135, #11478, #18441, #32651, #34824, #37074, #25384, #21212, #3563, #920, #35060, #40062, #31134, #32236, #14402, #36585, #12155, #3589, #38999, #33118, #29479, #3505, #38211, #5371, #19697, #17033, #39135, #14244, #18889, #39457, #33441, #20581, #29776, #35958, #25519, #1697, #19361, #40304, #13171, #18594, #40336, #18062, #1266, #6666, #7658, #9334, #30900, #16355, #38051, #28247, #23303, #3375, #33775, #20635, #23886, #11302, #6151, #11346, #20929, #1665, #3322, #37191, #20866, #41312, #14151, #22959, #35008, #18120, #23301 ) ) ;
#24029=CARTESIAN_POINT ( 'NONE',  ( -3.310556943750000425, 19.41135094264166128, -23.93493913623280278 ) ) ;
#24035=CARTESIAN_POINT ( 'NONE',  ( -3.310556943750000425, 19.41135094264166838, -76.84743913623280775 ) ) ;
#24037=CARTESIAN_POINT ( 'NONE',  ( 3.500000000000001332, 17.50000000000001776, -98.46098080242150274 ) ) ;
#24038=CARTESIAN_POINT ( 'NONE',  ( -0.9378221735089291577, 21.00000000000001776, -98.16632260368298546 ) ) ;
#24040=ORIENTED_EDGE ( 'NONE', *, *, #32132, .T. ) ;
#24042=CARTESIAN_POINT ( 'NONE',  ( 0.000000000000000000, 21.00000000000002487, -149.5231586289125687 ) ) ;
#24043=CARTESIAN_POINT ( 'NONE',  ( 3.310556943750001313, 17.50000000000001776, -87.26410580289947916 ) ) ;
#24052=DIRECTION ( 'NONE',  ( 0.000000000000000000, 1.000000000000000000, 0.000000000000000000 ) ) ;
#24053=CARTESIAN_POINT ( 'NONE',  ( 3.310556943750001313, 19.41135094264166128, -54.26827246956613493 ) ) ;
#24054=CARTESIAN_POINT ( 'NONE',  ( -1.655278471874999990, 20.36702641396249547, -116.0182724695661278 ) ) ;
#24055=ORIENTED_EDGE ( 'NONE', *, *, #17017, .T. ) ;
#24057=CARTESIAN_POINT ( 'NONE',  ( -1.750000000000002220, 14.46891108675448834, -125.4880641367107614 ) ) ;
#24058=( BOUNDED_CURVE ( )  B_SPLINE_CURVE ( 2, ( #35055, #18890, #31856, #2724, #41655, #25496, #9321, #35691, #36307 ),
 .UNSPECIFIED., .F., .T. ) 
 B_SPLINE_CURVE_WITH_KNOTS ( ( 3, 2, 2, 2, 3 ),
 ( 0.6979166666666666297, 0.6986111111111110716, 0.6999999999999999556, 0.7013888888888888395, 0.7020833333333332815 ),
 .UNSPECIFIED. ) 
 CURVE ( )  GEOMETRIC_REPRESENTATION_ITEM ( )  RATIONAL_B_SPLINE_CURVE ( ( 0.9330127018922194093, 0.9330127018922194093, 1.000000000000000000, 0.8660254037844387076, 1.000000000000000000, 0.8660254037844387076, 1.000000000000000000, 0.9330127018922194093, 0.9330127018922194093 ) ) 
 REPRESENTATION_ITEM ( '' )  );
#24060=CARTESIAN_POINT ( 'NONE',  ( -1.655278471874999990, 20.36702641396248481, -41.93077246956614346 ) ) ;
#24061=VECTOR ( 'NONE', #6331, 1000.000000000000000 ) ;
#24062=CARTESIAN_POINT ( 'NONE',  ( 1.655278471874998436, 14.63297358603754184, -66.51827246956612782 ) ) ;
#24063=CARTESIAN_POINT ( 'NONE',  ( 2.474675557024783212E-16, 21.54145188432740099, -112.2109808024215027 ) ) ;
#24064=CARTESIAN_POINT ( 'NONE',  ( -1.655278471874999990, 20.36702641396249192, -96.93077246956613635 ) ) ;
#24065=CARTESIAN_POINT ( 'NONE',  ( -3.500000000000000000, 19.52072594216370760, -47.73806413671076143 ) ) ;
#24067=CARTESIAN_POINT ( 'NONE',  ( -1.394453263437886604E-15, 14.00000000000001421, -70.40473080337741862 ) ) ;
#24069=CARTESIAN_POINT ( 'NONE',  ( 2.474675557024783212E-16, 21.54145188432739388, -71.21098080242150274 ) ) ;
#24070=LINE ( 'NONE', #33635, #21248 ) ;
#24071=CARTESIAN_POINT ( 'NONE',  ( 2.340729813953370519E-16, 21.32270188528330479, -30.01410580289948271 ) ) ;
#24072=CARTESIAN_POINT ( 'NONE',  ( 3.310556943749999981, 15.58864905735836892, -89.43493913623278502 ) ) ;
#24073=CARTESIAN_POINT ( 'NONE',  ( -1.750000000000002220, 14.46891108675447946, -57.48806413671076143 ) ) ;
#24074=CARTESIAN_POINT ( 'NONE',  ( 3.500000000000001332, 19.52072594216371115, -92.37764746908815994 ) ) ;
#24075=CARTESIAN_POINT ( 'NONE',  ( 3.310556943750001313, 19.41135094264166838, -110.2682724695661420 ) ) ;
#24076=CARTESIAN_POINT ( 'NONE',  ( 1.655278471874998436, 14.63297358603753828, -39.51827246956612782 ) ) ;
#24078=CARTESIAN_POINT ( 'NONE',  ( 7.785697387528201340E-15, 14.00000000000002487, -138.4047308033774470 ) ) ;
#24083=CARTESIAN_POINT ( 'NONE',  ( 1.655278471874998436, 14.63297358603754716, -95.43077246956613635 ) ) ;
#24086=ORIENTED_EDGE ( 'NONE', *, *, #9284, .T. ) ;
#24089=AXIS2_PLACEMENT_3D ( 'NONE', #26353, #39304, #9779 ) ;
#24090=CARTESIAN_POINT ( 'NONE',  ( -7.460324959392693302E-14, 21.00000000000001776, -85.90473080337741862 ) ) ;
#24094=EDGE_LOOP ( 'NONE', ( #3203, #33328, #23629, #25240 ) ) ;
#24101=EDGE_LOOP ( 'NONE', ( #6384, #5616, #8445, #27598 ) ) ;
#24103=CARTESIAN_POINT ( 'NONE',  ( 1.655278471875001101, 20.36702641396249902, -140.0974391362327935 ) ) ;
#24105=CARTESIAN_POINT ( 'NONE',  ( -0.9378221735089291577, 21.00000000000001066, -26.86007260463891555 ) ) ;
#24106=CARTESIAN_POINT ( 'NONE',  ( 1.655278471874998436, 14.63297358603755072, -131.5182724695661136 ) ) ;
#24107=CARTESIAN_POINT ( 'NONE',  ( 3.310556943749999981, 15.58864905735836537, -57.43493913623279212 ) ) ;
#24108=ORIENTED_EDGE ( 'NONE', *, *, #26909, .F. ) ;
#24110=CARTESIAN_POINT ( 'NONE',  ( 3.500000000000001332, 17.50000000000002487, -139.1547308033774186 ) ) ;
#24112=DIRECTION ( 'NONE',  ( 0.000000000000000000, 0.000000000000000000, 1.000000000000000000 ) ) ;
#24114=CARTESIAN_POINT ( 'NONE',  ( 2.474675557024783212E-16, 21.54145188432740810, -135.2109808024215170 ) ) ;
#24115=CARTESIAN_POINT ( 'NONE',  ( -7.022189441860112050E-16, 13.67729811471672718, -113.5141058028994792 ) ) ;
#24117=CARTESIAN_POINT ( 'NONE',  ( 0.9378221735089300459, 21.00000000000002132, -128.2556390011600342 ) ) ;
#24118=CARTESIAN_POINT ( 'NONE',  ( 1.750000000000001110, 20.53108891324555429, -85.29431413575483134 ) ) ;
#24121=CARTESIAN_POINT ( 'NONE',  ( -1.655278471875002211, 14.63297358603754184, -49.59743913623280775 ) ) ;
#24122=CARTESIAN_POINT ( 'NONE',  ( -7.022189441860112050E-16, 13.67729811471672541, -105.6016058028994422 ) ) ;
#24124=CARTESIAN_POINT ( 'NONE',  ( 4.648177544792955347E-16, 21.00000000000001776, -80.21098080242148853 ) ) ;
#24129=CARTESIAN_POINT ( 'NONE',  ( -3.310556943750000425, 19.41135094264166838, -126.9349391362327992 ) ) ;
#24131=DIRECTION ( 'NONE',  ( -0.000000000000000000, 1.259100132267607459E-16, -1.000000000000000000 ) ) ;
#24132=CARTESIAN_POINT ( 'NONE',  ( -3.500000000000001332, 17.50000000000002132, -116.9609808024215170 ) ) ;
#24133=CARTESIAN_POINT ( 'NONE',  ( 3.500000000000000000, 15.47927405783632437, -58.54431413575483845 ) ) ;
#24134=CARTESIAN_POINT ( 'NONE',  ( -1.655278471875002211, 14.63297358603754361, -60.68493913623279923 ) ) ;
#24136=CARTESIAN_POINT ( 'NONE',  ( -3.310556943750001313, 17.50000000000001776, -79.85160580289945642 ) ) ;
#24137=CARTESIAN_POINT ( 'NONE',  ( -1.394453263437886604E-15, 14.00000000000001421, -77.40473080337740441 ) ) ;
#24138=CARTESIAN_POINT ( 'NONE',  ( 3.500000000000001332, 17.50000000000001066, -44.46098080242151696 ) ) ;
#24142=CARTESIAN_POINT ( 'NONE',  ( 3.310556943750001313, 19.41135094264166128, -41.18077246956614346 ) ) ;
#24143=CARTESIAN_POINT ( 'NONE',  ( 3.310556943750001313, 19.41135094264166483, -100.1807724695661364 ) ) ;
#24150=CARTESIAN_POINT ( 'NONE',  ( -3.310556943750000425, 19.41135094264166128, -51.84743913623280775 ) ) ;
#24156=DIRECTION ( 'NONE',  ( 0.000000000000000000, 1.000000000000000000, 0.000000000000000000 ) ) ;
#24159=CARTESIAN_POINT ( 'NONE',  ( 3.500000000000001332, 17.50000000000001066, -38.46098080242150985 ) ) ;
#24161=CARTESIAN_POINT ( 'NONE',  ( 3.500000000000000000, 15.47927405783632615, -78.23806413671076143 ) ) ;
#24163=CARTESIAN_POINT ( 'NONE',  ( -1.655278471875002211, 14.63297358603754006, -30.68493913623279568 ) ) ;
#24164=CARTESIAN_POINT ( 'NONE',  ( -0.9378221735089291577, 21.00000000000001421, -53.16632260368298546 ) ) ;
#24165=CARTESIAN_POINT ( 'NONE',  ( 1.655278471874998436, 14.63297358603755072, -126.4307724695661364 ) ) ;
#24169=CARTESIAN_POINT ( 'NONE',  ( -3.310556943750000425, 19.41135094264166838, -123.9349391362327992 ) ) ;
#24171=CARTESIAN_POINT ( 'NONE',  ( 3.310556943749999981, 15.58864905735836892, -84.34743913623280775 ) ) ;
#24172=CARTESIAN_POINT ( 'NONE',  ( 1.750000000000001110, 20.53108891324554719, -45.98806413671076143 ) ) ;
#24173=CARTESIAN_POINT ( 'NONE',  ( 3.500000000000001332, 17.50000000000001421, -65.15473080337743284 ) ) ;
#24174=EDGE_CURVE ( 'NONE', #33342, #36084, #33172, .T. ) ;
#24175=CARTESIAN_POINT ( 'NONE',  ( -3.310556943750000425, 19.41135094264167549, -142.9349391362327992 ) ) ;
#24176=CARTESIAN_POINT ( 'NONE',  ( 1.750000000000001110, 20.53108891324555074, -69.98806413671077564 ) ) ;
#24177=CARTESIAN_POINT ( 'NONE',  ( 3.310556943750001313, 19.41135094264166483, -52.26827246956613493 ) ) ;
#24180=CARTESIAN_POINT ( 'NONE',  ( -1.749999999999999778, 20.53108891324555429, -99.12764746908817415 ) ) ;
#24181=CARTESIAN_POINT ( 'NONE',  ( 3.310556943750001313, 19.41135094264166483, -75.26827246956612782 ) ) ;
#24182=CARTESIAN_POINT ( 'NONE',  ( -3.310556943750002645, 15.58864905735837958, -138.7682724695661420 ) ) ;
#24184=CARTESIAN_POINT ( 'NONE',  ( 2.340729813953370519E-16, 21.32270188528331900, -104.0141058028994649 ) ) ;
#24185=CARTESIAN_POINT ( 'NONE',  ( -1.655278471874999990, 20.36702641396249192, -77.93077246956615056 ) ) ;
#24187=CARTESIAN_POINT ( 'NONE',  ( -1.655278471875002211, 14.63297358603754716, -94.68493913623279923 ) ) ;
#24188=( BOUNDED_CURVE ( )  B_SPLINE_CURVE ( 2, ( #25223, #22232, #28400, #11815, #28611, #2666, #41386, #22438, #31594 ),
 .UNSPECIFIED., .F., .F. ) 
 B_SPLINE_CURVE_WITH_KNOTS ( ( 3, 2, 2, 2, 3 ),
 ( 0.3104166666666666741, 0.3111111111111111160, 0.3125000000000000000, 0.3138888888888888840, 0.3145833333333333259 ),
 .UNSPECIFIED. ) 
 CURVE ( )  GEOMETRIC_REPRESENTATION_ITEM ( )  RATIONAL_B_SPLINE_CURVE ( ( 0.9330127018922194093, 0.9330127018922194093, 1.000000000000000000, 0.8660254037844387076, 1.000000000000000000, 0.8660254037844387076, 1.000000000000000000, 0.9330127018922194093, 0.9330127018922194093 ) ) 
 REPRESENTATION_ITEM ( '' )  );
#24190=CARTESIAN_POINT ( 'NONE',  ( -1.749999999999999778, 20.53108891324555429, -85.82139747004409003 ) ) ;
#24191=CARTESIAN_POINT ( 'NONE',  ( -0.9378221735089291577, 21.00000000000001421, -52.16632260368299256 ) ) ;
#24192=EDGE_CURVE ( 'NONE', #8481, #15295, #30199, .T. ) ;
#24194=CARTESIAN_POINT ( 'NONE',  ( 1.655278471874998436, 14.63297358603754006, -53.43077246956613635 ) ) ;
#24195=CARTESIAN_POINT ( 'NONE',  ( -3.695301148110399846E-14, 21.00000000000002132, -125.2109808024214885 ) ) ;
#24196=CARTESIAN_POINT ( 'NONE',  ( 2.340729813953370519E-16, 21.32270188528331900, -116.0141058028994649 ) ) ;
#24197=LINE ( 'NONE', #40348, #23033 ) ;
#24198=VERTEX_POINT ( 'NONE', #5331 ) ;
#24199=ORIENTED_EDGE ( 'NONE', *, *, #24293, .F. ) ;
#24201=VERTEX_POINT ( 'NONE', #2355 ) ;
#24202=CARTESIAN_POINT ( 'NONE',  ( -3.310556943750000425, 19.41135094264166128, -67.84743913623280775 ) ) ;
#24205=ORIENTED_EDGE ( 'NONE', *, *, #23180, .F. ) ;
#24206=CARTESIAN_POINT ( 'NONE',  ( -0.9378221735089310451, 14.00000000000001066, -29.44938900211595367 ) ) ;
#24209=VERTEX_POINT ( 'NONE', #37463 ) ;
#24210=CARTESIAN_POINT ( 'NONE',  ( -1.394453263437886604E-15, 14.00000000000001066, -50.40473080337741862 ) ) ;
#24211=CARTESIAN_POINT ( 'NONE',  ( -3.310556943750001313, 17.50000000000002487, -136.7641058028994792 ) ) ;
#24212=CARTESIAN_POINT ( 'NONE',  ( -0.9378221735089310451, 14.00000000000002309, -131.4493890021159359 ) ) ;
#24213=CARTESIAN_POINT ( 'NONE',  ( -7.022189441860112050E-16, 13.67729811471671653, -46.60160580289946353 ) ) ;
#24214=CARTESIAN_POINT ( 'NONE',  ( 1.655278471875001101, 20.36702641396248481, -34.18493913623279923 ) ) ;
#24215=CARTESIAN_POINT ( 'NONE',  ( 1.655278471875001101, 20.36702641396249192, -101.1849391362327992 ) ) ;
#24216=CARTESIAN_POINT ( 'NONE',  ( 3.310556943750001313, 17.50000000000002487, -138.3516058028994564 ) ) ;
#24218=CARTESIAN_POINT ( 'NONE',  ( -1.750000000000002220, 14.46891108675448478, -95.79431413575484555 ) ) ;
#24221=CARTESIAN_POINT ( 'NONE',  ( -3.500000000000001332, 17.50000000000001776, -83.65473080337743284 ) ) ;
#24222=CARTESIAN_POINT ( 'NONE',  ( 1.655278471875001101, 20.36702641396248836, -71.18493913623278502 ) ) ;
#24224=CARTESIAN_POINT ( 'NONE',  ( -1.394453263437886604E-15, 14.00000000000001776, -84.40473080337743284 ) ) ;
#24226=DIRECTION ( 'NONE',  ( -0.000000000000000000, 1.259100132267607459E-16, -1.000000000000000000 ) ) ;
#24227=CARTESIAN_POINT ( 'NONE',  ( -3.500000000000002220, 15.47927405783632260, -46.87764746908817415 ) ) ;
#24228=CARTESIAN_POINT ( 'NONE',  ( 1.655278471875001101, 20.36702641396249547, -121.0974391362328078 ) ) ;
#24229=CYLINDRICAL_SURFACE ( 'NONE', #16297, 3.499999999999999556 ) ;
#24231=ORIENTED_EDGE ( 'NONE', *, *, #12438, .F. ) ;
#24232=CARTESIAN_POINT ( 'NONE',  ( 3.500000000000000000, 15.47927405783632970, -115.2380641367107472 ) ) ;
#24236=EDGE_CURVE ( 'NONE', #31790, #2211, #4106, .T. ) ;
#24239=CARTESIAN_POINT ( 'NONE',  ( 3.310556943750001313, 19.41135094264166483, -74.18077246956612214 ) ) ;
#24240=CARTESIAN_POINT ( 'NONE',  ( 1.750000000000001110, 20.53108891324555785, -115.9880641367107614 ) ) ;
#24243=CARTESIAN_POINT ( 'NONE',  ( 1.749999999999998224, 14.46891108675448123, -88.62764746908817415 ) ) ;
#24244=CARTESIAN_POINT ( 'NONE',  ( 3.310556943750001313, 19.41135094264166483, -84.18077246956615056 ) ) ;
#24245=ORIENTED_EDGE ( 'NONE', *, *, #16302, .T. ) ;
#24246=EDGE_LOOP ( 'NONE', ( #250, #15227, #11732, #5665 ) ) ;
#24248=( BOUNDED_CURVE ( )  B_SPLINE_CURVE ( 2, ( #34270, #18110, #15348, #31080, #14913, #28298, #12125, #27881, #11711 ),
 .UNSPECIFIED., .F., .T. ) 
 B_SPLINE_CURVE_WITH_KNOTS ( ( 3, 2, 2, 2, 3 ),
 ( 0.9354166666666666741, 0.9361111111111111160, 0.9375000000000000000, 0.9388888888888888840, 0.9395833333333333259 ),
 .UNSPECIFIED. ) 
 CURVE ( )  GEOMETRIC_REPRESENTATION_ITEM ( )  RATIONAL_B_SPLINE_CURVE ( ( 0.9330127018922194093, 0.9330127018922194093, 1.000000000000000000, 0.8660254037844387076, 1.000000000000000000, 0.8660254037844387076, 1.000000000000000000, 0.9330127018922194093, 0.9330127018922194093 ) ) 
 REPRESENTATION_ITEM ( '' )  );
#24250=CARTESIAN_POINT ( 'NONE',  ( 3.500000000000001332, 19.52072594216371826, -102.3776474690881599 ) ) ;
#24251=EDGE_LOOP ( 'NONE', ( #2264, #14714, #2083, #1067 ) ) ;
#24252=DIRECTION ( 'NONE',  ( -0.000000000000000000, 1.259100132267607459E-16, -1.000000000000000000 ) ) ;
#24253=CARTESIAN_POINT ( 'NONE',  ( 3.310556943750001313, 19.41135094264166128, -51.26827246956612782 ) ) ;
#24254=CARTESIAN_POINT ( 'NONE',  ( -3.310556943750001313, 17.50000000000002132, -115.8516058028994706 ) ) ;
#24256=CARTESIAN_POINT ( 'NONE',  ( -3.500000000000001332, 17.50000000000002132, -121.6547308033774328 ) ) ;
#24257=CARTESIAN_POINT ( 'NONE',  ( -7.022189441860112050E-16, 13.67729811471671475, -38.51410580289947916 ) ) ;
#24258=CARTESIAN_POINT ( 'NONE',  ( -1.655278471874999990, 20.36702641396248836, -68.01827246956612782 ) ) ;
#24259=CARTESIAN_POINT ( 'NONE',  ( -3.500000000000002220, 15.47927405783633503, -112.8776474690881599 ) ) ;
#24261=CARTESIAN_POINT ( 'NONE',  ( -3.310556943750001313, 17.50000000000001776, -98.76410580289947916 ) ) ;
#24264=CARTESIAN_POINT ( 'NONE',  ( -0.9378221735089291577, 21.00000000000001066, -26.16632260368299256 ) ) ;
#24267=CARTESIAN_POINT ( 'NONE',  ( 3.500000000000000000, 15.47927405783632260, -65.54431413575484555 ) ) ;
#24268=LINE ( 'NONE', #5314, #32544 ) ;
#24269=CARTESIAN_POINT ( 'NONE',  ( -1.655278471874999990, 20.36702641396248481, -31.93077246956614701 ) ) ;
#24270=CARTESIAN_POINT ( 'NONE',  ( -3.310556943750000425, 19.41135094264166483, -89.93493913623278502 ) ) ;
#24271=CARTESIAN_POINT ( 'NONE',  ( -3.500000000000000888, 19.52072594216370760, -52.73806413671076143 ) ) ;
#24273=CARTESIAN_POINT ( 'NONE',  ( -3.310556943750002201, 15.58864905735837780, -111.7682724695661420 ) ) ;
#24274=CARTESIAN_POINT ( 'NONE',  ( 1.655278471874998436, 14.63297358603753828, -35.51827246956612782 ) ) ;
#24279=CARTESIAN_POINT ( 'NONE',  ( 1.750000000000001110, 20.53108891324555074, -48.29431413575484555 ) ) ;
#24280=CARTESIAN_POINT ( 'NONE',  ( -3.310556943750000425, 19.41135094264166838, -91.84743913623280775 ) ) ;
#24281=CARTESIAN_POINT ( 'NONE',  ( 3.500000000000001332, 19.52072594216371826, -117.0713974700440900 ) ) ;
#24284=CARTESIAN_POINT ( 'NONE',  ( 1.750000000000001110, 20.53108891324555074, -57.29431413575483845 ) ) ;
#24286=CARTESIAN_POINT ( 'NONE',  ( 4.648177544792955347E-16, 21.00000000000001066, -46.21098080242150274 ) ) ;
#24292=ORIENTED_EDGE ( 'NONE', *, *, #33438, .F. ) ;
#24293=EDGE_CURVE ( 'NONE', #17014, #5191, #40517, .T. ) ;
#24302=CARTESIAN_POINT ( 'NONE',  ( -0.9378221735089291577, 21.00000000000001066, -27.86007260463891200 ) ) ;
#24303=( BOUNDED_CURVE ( )  B_SPLINE_CURVE ( 2, ( #41698, #32115, #2352, #25538, #2980, #15971, #15123, #41916, #28292 ),
 .UNSPECIFIED., .F., .T. ) 
 B_SPLINE_CURVE_WITH_KNOTS ( ( 3, 2, 2, 2, 3 ),
 ( 0.9770833333333333037, 0.9777777777777777457, 0.9791666666666666297, 0.9805555555555555136, 0.9812499999999999556 ),
 .UNSPECIFIED. ) 
 CURVE ( )  GEOMETRIC_REPRESENTATION_ITEM ( )  RATIONAL_B_SPLINE_CURVE ( ( 0.9330127018922194093, 0.9330127018922194093, 1.000000000000000000, 0.8660254037844387076, 1.000000000000000000, 0.8660254037844387076, 1.000000000000000000, 0.9330127018922194093, 0.9330127018922194093 ) ) 
 REPRESENTATION_ITEM ( '' )  );
#24304=CYLINDRICAL_SURFACE ( 'NONE', #5830, 3.499999999999999556 ) ;
#24305=CARTESIAN_POINT ( 'NONE',  ( 3.310556943750001313, 19.41135094264167549, -135.1807724695661364 ) ) ;
#24306=CARTESIAN_POINT ( 'NONE',  ( 0.000000000000000000, 17.50000000000002487, -149.5231586289125687 ) ) ;
#24307=CARTESIAN_POINT ( 'NONE',  ( -3.500000000000002220, 15.47927405783632082, -26.57139747004409713 ) ) ;
#24308=CARTESIAN_POINT ( 'NONE',  ( 2.340729813953370519E-16, 21.32270188528332255, -131.1016058028994564 ) ) ;
#24309=CARTESIAN_POINT ( 'NONE',  ( -1.655278471875002211, 14.63297358603754361, -54.68493913623280633 ) ) ;
#24312=CARTESIAN_POINT ( 'NONE',  ( -3.500000000000000888, 19.52072594216372181, -141.7380641367107614 ) ) ;
#24315=EDGE_CURVE ( 'NONE', #16447, #40609, #18780, .T. ) ;
#24316=CARTESIAN_POINT ( 'NONE',  ( 1.655278471874998436, 14.63297358603754894, -110.4307724695661506 ) ) ;
#24318=EDGE_CURVE ( 'NONE', #25787, #37593, #30456, .T. ) ;
#24320=CARTESIAN_POINT ( 'NONE',  ( 3.500000000000001332, 17.50000000000001776, -80.46098080242150274 ) ) ;
#24322=CARTESIAN_POINT ( 'NONE',  ( -3.310556943750000425, 19.41135094264166128, -46.84743913623280065 ) ) ;
#24323=EDGE_CURVE ( 'NONE', #6435, #32641, #12, .T. ) ;
#24324=CARTESIAN_POINT ( 'NONE',  ( -1.655278471875002211, 14.63297358603754894, -107.6849391362327992 ) ) ;
#24325=CARTESIAN_POINT ( 'NONE',  ( -3.500000000000002220, 15.47927405783633503, -129.8776474690881741 ) ) ;
#24326=CARTESIAN_POINT ( 'NONE',  ( 4.648177544792955347E-16, 21.00000000000001776, -99.90473080337743284 ) ) ;
#24328=CARTESIAN_POINT ( 'NONE',  ( 1.655278471875001101, 20.36702641396249902, -130.1849391362327992 ) ) ;
#24331=CARTESIAN_POINT ( 'NONE',  ( 3.500000000000000000, 15.47927405783632082, -27.54431413575483845 ) ) ;
#24333=CARTESIAN_POINT ( 'NONE',  ( 3.310556943750001313, 17.50000000000001421, -59.35160580289947063 ) ) ;
#24335=CARTESIAN_POINT ( 'NONE',  ( -3.310556943750000425, 19.41135094264166838, -77.93493913623279923 ) ) ;
#24338=FACE_OUTER_BOUND ( 'NONE', #7872, .T. ) ;
#24339=DIRECTION ( 'NONE',  ( 0.000000000000000000, 1.000000000000000000, 0.000000000000000000 ) ) ;
#24342=CARTESIAN_POINT ( 'NONE',  ( 2.340729813953370519E-16, 21.32270188528330834, -41.01410580289948626 ) ) ;
#24343=CARTESIAN_POINT ( 'NONE',  ( -1.655278471875002211, 14.63297358603754894, -95.59743913623280775 ) ) ;
#24347=VERTEX_POINT ( 'NONE', #16390 ) ;
#24349=CARTESIAN_POINT ( 'NONE',  ( -7.022189441860112050E-16, 13.67729811471671653, -49.51410580289947205 ) ) ;
#24351=ORIENTED_EDGE ( 'NONE', *, *, #37565, .F. ) ;
#24352=CYLINDRICAL_SURFACE ( 'NONE', #12412, 3.499999999999999556 ) ;
#24356=CARTESIAN_POINT ( 'NONE',  ( 4.648177544792955347E-16, 21.00000000000001776, -89.21098080242148853 ) ) ;
#24357=CARTESIAN_POINT ( 'NONE',  ( 2.474675557024783212E-16, 21.54145188432739033, -39.21098080242150985 ) ) ;
#24358=CARTESIAN_POINT ( 'NONE',  ( 0.9378221735088952959, 21.00000000000003908, -86.25563900116000582 ) ) ;
#24359=CARTESIAN_POINT ( 'NONE',  ( 0.9378221735089281585, 14.00000000000002132, -119.3600726046389013 ) ) ;
#24360=VECTOR ( 'NONE', #37724, 1000.000000000000000 ) ;
#24362=CARTESIAN_POINT ( 'NONE',  ( 3.310556943750001313, 19.41135094264165772, -25.26827246956613138 ) ) ;
#24363=CARTESIAN_POINT ( 'NONE',  ( -0.9378221735089310451, 14.00000000000002132, -106.4493890021159501 ) ) ;
#24364=CARTESIAN_POINT ( 'NONE',  ( -1.655278471874999990, 20.36702641396249547, -128.9307724695661364 ) ) ;
#24367=EDGE_CURVE ( 'NONE', #37828, #32296, #29333, .T. ) ;
#24368=CARTESIAN_POINT ( 'NONE',  ( -0.9378221735089310451, 14.00000000000001599, -75.44938900211593591 ) ) ;
#24369=EDGE_CURVE ( 'NONE', #35272, #19314, #17175, .T. ) ;
#24370=CARTESIAN_POINT ( 'NONE',  ( 3.310556943749999981, 15.58864905735837425, -123.4349391362327992 ) ) ;
#24371=CARTESIAN_POINT ( 'NONE',  ( -3.500000000000001332, 17.50000000000001421, -55.65473080337743284 ) ) ;
#24372=CARTESIAN_POINT ( 'NONE',  ( 1.749999999999998224, 14.46891108675447413, -36.32139747004409003 ) ) ;
#24373=CARTESIAN_POINT ( 'NONE',  ( -1.394453263437886604E-15, 14.00000000000002132, -115.4047308033774186 ) ) ;
#24375=CARTESIAN_POINT ( 'NONE',  ( 3.500000000000000000, 15.47927405783632437, -67.23806413671076143 ) ) ;
#24376=CARTESIAN_POINT ( 'NONE',  ( -1.749999999999999778, 20.53108891324555074, -67.82139747004409003 ) ) ;
#24377=CARTESIAN_POINT ( 'NONE',  ( -7.022189441860112050E-16, 13.67729811471671830, -51.60160580289946353 ) ) ;
#24380=CARTESIAN_POINT ( 'NONE',  ( -1.655278471875002211, 14.63297358603754539, -74.68493913623279923 ) ) ;
#24382=CARTESIAN_POINT ( 'NONE',  ( 3.310556943750001313, 19.41135094264166838, -103.1807724695661364 ) ) ;
#24383=CARTESIAN_POINT ( 'NONE',  ( 2.340729813953370519E-16, 21.32270188528331190, -78.01410580289946495 ) ) ;
#24385=CARTESIAN_POINT ( 'NONE',  ( -1.655278471875002211, 14.63297358603754894, -97.68493913623279923 ) ) ;
#24387=CARTESIAN_POINT ( 'NONE',  ( -0.9378221735089291577, 21.00000000000001066, -33.16632260368298546 ) ) ;
#24390=CARTESIAN_POINT ( 'NONE',  ( 1.655278471874998436, 14.63297358603754184, -54.43077246956613635 ) ) ;
#24391=CARTESIAN_POINT ( 'NONE',  ( 0.000000000000000000, 21.00000000000002487, -149.5231586289125687 ) ) ;
#24392=CARTESIAN_POINT ( 'NONE',  ( 3.310556943750001313, 17.50000000000002132, -109.2641058028994649 ) ) ;
#24393=CARTESIAN_POINT ( 'NONE',  ( 0.9378221735089281585, 14.00000000000001776, -84.66632260368297125 ) ) ;
#24394=VECTOR ( 'NONE', #8041, 1000.000000000000000 ) ;
#24395=ORIENTED_EDGE ( 'NONE', *, *, #7707, .F. ) ;
#24398=ORIENTED_EDGE ( 'NONE', *, *, #42045, .T. ) ;
#24399=CARTESIAN_POINT ( 'NONE',  ( -3.500000000000002220, 15.47927405783633503, -109.8776474690881599 ) ) ;
#24400=CARTESIAN_POINT ( 'NONE',  ( 3.310556943749999981, 15.58864905735836714, -68.34743913623280775 ) ) ;
#24401=ORIENTED_EDGE ( 'NONE', *, *, #17519, .F. ) ;
#24403=CARTESIAN_POINT ( 'NONE',  ( -1.750000000000002220, 14.46891108675447590, -29.48806413671076143 ) ) ;
#24409=EDGE_CURVE ( 'NONE', #16185, #18793, #9801, .T. ) ;
#24410=ORIENTED_EDGE ( 'NONE', *, *, #11157, .T. ) ;
#24412=CARTESIAN_POINT ( 'NONE',  ( -7.022189441860112050E-16, 13.67729811471672896, -128.5141058028994507 ) ) ;
#24413=CARTESIAN_POINT ( 'NONE',  ( -1.750000000000002220, 14.46891108675448834, -131.4880641367107614 ) ) ;
#24414=CARTESIAN_POINT ( 'NONE',  ( -1.655278471875002211, 14.63297358603754184, -40.68493913623279212 ) ) ;
#24415=CARTESIAN_POINT ( 'NONE',  ( -3.310556943750002645, 15.58864905735836537, -32.76827246956613493 ) ) ;
#24416=EDGE_CURVE ( 'NONE', #6760, #11127, #34799, .T. ) ;
#24417=CARTESIAN_POINT ( 'NONE',  ( -7.022189441860112050E-16, 13.67729811471672363, -92.60160580289947063 ) ) ;
#24418=CARTESIAN_POINT ( 'NONE',  ( 1.655278471875001101, 20.36702641396249902, -142.0974391362327935 ) ) ;
#24420=( BOUNDED_CURVE ( )  B_SPLINE_CURVE ( 2, ( #36430, #13884, #7295, #19836, #26652, #29618, #36643, #39611, #20057 ),
 .UNSPECIFIED., .F., .T. ) 
 B_SPLINE_CURVE_WITH_KNOTS ( ( 3, 2, 2, 2, 3 ),
 ( 0.06041666666666666713, 0.06111111111111110911, 0.06250000000000000000, 0.06388888888888888395, 0.06458333333333333981 ),
 .UNSPECIFIED. ) 
 CURVE ( )  GEOMETRIC_REPRESENTATION_ITEM ( )  RATIONAL_B_SPLINE_CURVE ( ( 0.9330127018922194093, 0.9330127018922194093, 1.000000000000000000, 0.8660254037844387076, 1.000000000000000000, 0.8660254037844387076, 1.000000000000000000, 0.9330127018922187432, 0.9330127018922194093 ) ) 
 REPRESENTATION_ITEM ( '' )  );
#24421=CARTESIAN_POINT ( 'NONE',  ( -3.310556943750002645, 15.58864905735837958, -138.7682724695661420 ) ) ;
#24422=CARTESIAN_POINT ( 'NONE',  ( 3.500000000000001332, 17.50000000000002132, -121.4609808024215170 ) ) ;
#24423=CARTESIAN_POINT ( 'NONE',  ( -7.424026671074350129E-16, 13.45854811567263809, -95.71098080242150274 ) ) ;
#24425=CARTESIAN_POINT ( 'NONE',  ( 3.500000000000001332, 19.52072594216370760, -64.37764746908817415 ) ) ;
#24426=CARTESIAN_POINT ( 'NONE',  ( 3.500000000000000000, 15.47927405783632615, -85.23806413671076143 ) ) ;
#24427=CARTESIAN_POINT ( 'NONE',  ( -3.310556943750000425, 19.41135094264166483, -70.93493913623278502 ) ) ;
#24431=CARTESIAN_POINT ( 'NONE',  ( -3.500000000000002220, 15.47927405783633503, -119.8776474690881884 ) ) ;
#24432=CARTESIAN_POINT ( 'NONE',  ( -7.424026671074350129E-16, 13.45854811567263276, -48.71098080242150985 ) ) ;
#24433=CARTESIAN_POINT ( 'NONE',  ( 1.655278471875001101, 20.36702641396249547, -117.0974391362327935 ) ) ;
#24436=VERTEX_POINT ( 'NONE', #37009 ) ;
#24437=AXIS2_PLACEMENT_3D ( 'NONE', #24306, #40465, #24933 ) ;
#24438=CARTESIAN_POINT ( 'NONE',  ( 1.749999999999998224, 14.46891108675448478, -112.3213974700441042 ) ) ;
#24440=CARTESIAN_POINT ( 'NONE',  ( -3.500000000000000000, 19.52072594216371115, -83.73806413671076143 ) ) ;
#24444=CARTESIAN_POINT ( 'NONE',  ( -1.655278471875002211, 14.63297358603754539, -73.59743913623280775 ) ) ;
#24445=CARTESIAN_POINT ( 'NONE',  ( -3.500000000000000000, 19.52072594216371115, -97.04431413575484555 ) ) ;
#24446=CARTESIAN_POINT ( 'NONE',  ( 0.9378221735089300459, 21.00000000000001421, -69.25563900116003424 ) ) ;
#24447=ORIENTED_EDGE ( 'NONE', *, *, #17448, .T. ) ;
#24449=CARTESIAN_POINT ( 'NONE',  ( 3.500000000000000000, 15.47927405783631727, -25.54431413575483489 ) ) ;
#24450=CARTESIAN_POINT ( 'NONE',  ( -1.655278471874999990, 20.36702641396249192, -84.93077246956613635 ) ) ;
#24451=ORIENTED_EDGE ( 'NONE', *, *, #2117, .F. ) ;
#24453=VECTOR ( 'NONE', #1879, 1000.000000000000000 ) ;
#24460=CARTESIAN_POINT ( 'NONE',  ( 3.310556943750001313, 17.50000000000001421, -51.35160580289946353 ) ) ;
#24462=CARTESIAN_POINT ( 'NONE',  ( -3.310556943750001313, 17.50000000000002132, -111.8516058028994564 ) ) ;
#24464=CARTESIAN_POINT ( 'NONE',  ( 2.340729813953370519E-16, 21.32270188528330479, -36.01410580289947205 ) ) ;
#24465=CARTESIAN_POINT ( 'NONE',  ( -3.310556943750000425, 19.41135094264166128, -65.93493913623279923 ) ) ;
#24466=CARTESIAN_POINT ( 'NONE',  ( 3.500000000000001332, 17.50000000000002132, -111.4609808024215027 ) ) ;
#24468=CARTESIAN_POINT ( 'NONE',  ( -1.655278471875002211, 14.63297358603754716, -94.59743913623280775 ) ) ;
#24469=CARTESIAN_POINT ( 'NONE',  ( -1.394453263437886604E-15, 14.00000000000001776, -98.40473080337743284 ) ) ;
#24470=CARTESIAN_POINT ( 'NONE',  ( -1.394453263437886604E-15, 14.00000000000001066, -52.40473080337743284 ) ) ;
#24473=CARTESIAN_POINT ( 'NONE',  ( -7.424026671074350129E-16, 13.45854811567263454, -64.71098080242150274 ) ) ;
#24475=CARTESIAN_POINT ( 'NONE',  ( -0.9378221735089310451, 14.00000000000001066, -43.75563900116002714 ) ) ;
#24476=CARTESIAN_POINT ( 'NONE',  ( 2.340729813953370519E-16, 21.32270188528330479, -33.01410580289947205 ) ) ;
#24477=CARTESIAN_POINT ( 'NONE',  ( -3.310556943750002645, 15.58864905735837247, -92.76827246956611361 ) ) ;
#24478=CARTESIAN_POINT ( 'NONE',  ( 1.750000000000001110, 20.53108891324555074, -51.98806413671076854 ) ) ;
#24480=CARTESIAN_POINT ( 'NONE',  ( -1.655278471874999990, 20.36702641396249547, -108.0182724695661278 ) ) ;
#24481=CARTESIAN_POINT ( 'NONE',  ( -3.310556943750002201, 15.58864905735836537, -37.76827246956612782 ) ) ;
#24483=CARTESIAN_POINT ( 'NONE',  ( 4.648177544792955347E-16, 21.00000000000001421, -53.21098080242150274 ) ) ;
#24487=CARTESIAN_POINT ( 'NONE',  ( 3.500000000000000000, 15.47927405783632082, -48.54431413575484555 ) ) ;
#24489=CARTESIAN_POINT ( 'NONE',  ( 3.310556943749999981, 15.58864905735836892, -86.34743913623279354 ) ) ;
#24495=CARTESIAN_POINT ( 'NONE',  ( 3.500000000000001332, 17.50000000000002487, -133.1547308033774186 ) ) ;
#24500=( BOUNDED_CURVE ( )  B_SPLINE_CURVE ( 2, ( #34966, #41151, #24782, #34344, #41355, #5204, #2849, #11574, #41568 ),
 .UNSPECIFIED., .F., .F. ) 
 B_SPLINE_CURVE_WITH_KNOTS ( ( 3, 2, 2, 2, 3 ),
 ( 0.6062499999999999556, 0.6069444444444443976, 0.6083333333333332815, 0.6097222222222222765, 0.6104166666666667185 ),
 .UNSPECIFIED. ) 
 CURVE ( )  GEOMETRIC_REPRESENTATION_ITEM ( )  RATIONAL_B_SPLINE_CURVE ( ( 0.9330127018922194093, 0.9330127018922194093, 1.000000000000000000, 0.8660254037844387076, 1.000000000000000000, 0.8660254037844387076, 1.000000000000000000, 0.9330127018922194093, 0.9330127018922194093 ) ) 
 REPRESENTATION_ITEM ( '' )  );
#24501=ORIENTED_EDGE ( 'NONE', *, *, #18655, .F. ) ;
#24503=CARTESIAN_POINT ( 'NONE',  ( 4.648177544792955347E-16, 21.00000000000001421, -68.21098080242148853 ) ) ;
#24508=VERTEX_POINT ( 'NONE', #20627 ) ;
#24510=CARTESIAN_POINT ( 'NONE',  ( 3.500000000000000000, 15.47927405783633503, -140.2380641367107614 ) ) ;
#24511=CARTESIAN_POINT ( 'NONE',  ( -3.310556943750002645, 15.58864905735837958, -137.6807724695661364 ) ) ;
#24514=CARTESIAN_POINT ( 'NONE',  ( 2.340729813953370519E-16, 21.32270188528331900, -128.1016058028994848 ) ) ;
#24515=CARTESIAN_POINT ( 'NONE',  ( -1.655278471874999990, 20.36702641396248836, -58.01827246956613493 ) ) ;
#24518=CARTESIAN_POINT ( 'NONE',  ( 2.474675557024783212E-16, 21.54145188432740810, -133.9047308033774186 ) ) ;
#24519=VECTOR ( 'NONE', #20530, 1000.000000000000000 ) ;
#24521=CARTESIAN_POINT ( 'NONE',  ( 1.750000000000001110, 20.53108891324556140, -130.2943141357548598 ) ) ;
#24522=CARTESIAN_POINT ( 'NONE',  ( 3.310556943750001313, 19.41135094264166838, -114.1807724695661364 ) ) ;
#24525=EDGE_CURVE ( 'NONE', #36839, #167, #37529, .T. ) ;
#24527=CARTESIAN_POINT ( 'NONE',  ( 1.749999999999998224, 14.46891108675447946, -78.62764746908817415 ) ) ;
#24529=CARTESIAN_POINT ( 'NONE',  ( 1.655278471875001101, 20.36702641396248836, -49.09743913623280775 ) ) ;
#24530=CARTESIAN_POINT ( 'NONE',  ( -3.310556943750001313, 17.50000000000002132, -104.8516058028994564 ) ) ;
#24531=CARTESIAN_POINT ( 'NONE',  ( 3.500000000000001332, 19.52072594216371826, -111.0713974700441042 ) ) ;
#24534=CARTESIAN_POINT ( 'NONE',  ( 2.340729813953370519E-16, 21.32270188528331900, -125.1016058028994564 ) ) ;
#24537=CARTESIAN_POINT ( 'NONE',  ( 0.9378221735089128375, 21.00000000000003553, -123.9493890021159359 ) ) ;
#24538=CARTESIAN_POINT ( 'NONE',  ( -1.394453263437886604E-15, 14.00000000000002132, -130.4047308033774186 ) ) ;
#24539=CARTESIAN_POINT ( 'NONE',  ( -1.655278471875002211, 14.63297358603754361, -57.68493913623279212 ) ) ;
#24541=ORIENTED_EDGE ( 'NONE', *, *, #23139, .F. ) ;
#24542=CARTESIAN_POINT ( 'NONE',  ( 3.310556943749999981, 15.58864905735836714, -79.43493913623279923 ) ) ;
#24546=FACE_OUTER_BOUND ( 'NONE', #25865, .T. ) ;
#24548=CARTESIAN_POINT ( 'NONE',  ( 3.310556943749999981, 15.58864905735836182, -38.34743913623281486 ) ) ;
#24550=( BOUNDED_CURVE ( )  B_SPLINE_CURVE ( 2, ( #29742, #6780, #19542, #39102, #185, #3383, #26152, #32514, #26782 ),
 .UNSPECIFIED., .F., .T. ) 
 B_SPLINE_CURVE_WITH_KNOTS ( ( 3, 2, 2, 2, 3 ),
 ( 0.5437499999999999556, 0.5444444444444443976, 0.5458333333333332815, 0.5472222222222222765, 0.5479166666666667185 ),
 .UNSPECIFIED. ) 
 CURVE ( )  GEOMETRIC_REPRESENTATION_ITEM ( )  RATIONAL_B_SPLINE_CURVE ( ( 0.9330127018922194093, 0.9330127018922194093, 1.000000000000000000, 0.8660254037844387076, 1.000000000000000000, 0.8660254037844387076, 1.000000000000000000, 0.9330127018922194093, 0.9330127018922194093 ) ) 
 REPRESENTATION_ITEM ( '' )  );
#24553=ORIENTED_EDGE ( 'NONE', *, *, #13750, .F. ) ;
#24555=CARTESIAN_POINT ( 'NONE',  ( 3.310556943750001313, 17.50000000000001066, -45.26410580289947916 ) ) ;
#24556=EDGE_CURVE ( 'NONE', #29085, #4773, #7440, .T. ) ;
#24560=CARTESIAN_POINT ( 'NONE',  ( 4.648177544792955347E-16, 21.00000000000001776, -94.21098080242150274 ) ) ;
#24563=CARTESIAN_POINT ( 'NONE',  ( -3.500000000000000000, 19.52072594216371826, -104.7380641367107472 ) ) ;
#24566=CARTESIAN_POINT ( 'NONE',  ( -1.750000000000002220, 14.46891108675447590, -38.79431413575484555 ) ) ;
#24567=CARTESIAN_POINT ( 'NONE',  ( 0.000000000000000000, 17.50000000000002487, -149.5231586289125687 ) ) ;
#24568=CARTESIAN_POINT ( 'NONE',  ( -1.394453263437886604E-15, 14.00000000000001066, -28.40473080337742928 ) ) ;
#24570=CARTESIAN_POINT ( 'NONE',  ( 1.750000000000001110, 20.53108891324556140, -143.2943141357548313 ) ) ;
#24571=CARTESIAN_POINT ( 'NONE',  ( -1.749999999999999778, 20.53108891324555785, -106.8213974700441042 ) ) ;
#24572=CARTESIAN_POINT ( 'NONE',  ( -1.655278471874999990, 20.36702641396249902, -129.9307724695661364 ) ) ;
#24575=EDGE_CURVE ( 'NONE', #30090, #5717, #39767, .T. ) ;
#24578=CARTESIAN_POINT ( 'NONE',  ( 3.310556943750001313, 19.41135094264166838, -125.2682724695661136 ) ) ;
#24581=CARTESIAN_POINT ( 'NONE',  ( -1.749999999999999778, 20.53108891324554719, -36.82139747004409003 ) ) ;
#24582=CARTESIAN_POINT ( 'NONE',  ( 4.648177544792955347E-16, 21.00000000000002132, -114.9047308033774186 ) ) ;
#24583=CARTESIAN_POINT ( 'NONE',  ( 0.000000000000000000, 17.50000000000002487, -149.5231586289125687 ) ) ;
#24584=CARTESIAN_POINT ( 'NONE',  ( 4.648177544792955347E-16, 21.00000000000001421, -66.90473080337743284 ) ) ;
#24585=CARTESIAN_POINT ( 'NONE',  ( -3.500000000000001332, 17.50000000000001421, -67.65473080337743284 ) ) ;
#24587=CARTESIAN_POINT ( 'NONE',  ( 2.340729813953370519E-16, 21.32270188528331190, -54.10160580289946353 ) ) ;
#24590=CARTESIAN_POINT ( 'NONE',  ( -7.022189441860112050E-16, 13.67729811471672186, -74.60160580289947063 ) ) ;
#24592=CARTESIAN_POINT ( 'NONE',  ( -1.655278471874999990, 20.36702641396249547, -104.9307724695661364 ) ) ;
#24593=CARTESIAN_POINT ( 'NONE',  ( -3.310556943750001313, 17.50000000000001421, -69.76410580289947916 ) ) ;
#24595=CARTESIAN_POINT ( 'NONE',  ( -3.310556943750002201, 15.58864905735837425, -96.76827246956612782 ) ) ;
#24597=CARTESIAN_POINT ( 'NONE',  ( 3.500000000000000000, 15.47927405783632082, -26.54431413575483845 ) ) ;
#24598=FACE_OUTER_BOUND ( 'NONE', #16500, .T. ) ;
#24599=CARTESIAN_POINT ( 'NONE',  ( 1.655278471875001101, 20.36702641396248836, -55.09743913623281486 ) ) ;
#24600=AXIS2_PLACEMENT_3D ( 'NONE', #38807, #10091, #9681 ) ;
#24602=CARTESIAN_POINT ( 'NONE',  ( -7.022189441860112050E-16, 13.67729811471672718, -111.5141058028994649 ) ) ;
#24603=ORIENTED_EDGE ( 'NONE', *, *, #37588, .T. ) ;
#24608=CARTESIAN_POINT ( 'NONE',  ( 1.655278471875001101, 20.36702641396248836, -64.09743913623280775 ) ) ;
#24609=EDGE_CURVE ( 'NONE', #19056, #1595, #30706, .T. ) ;
#24614=CONICAL_SURFACE ( 'NONE', #11012, 577.3502691896253509, 0.5235987755982987046 ) ;
#24616=EDGE_CURVE ( 'NONE', #9312, #39182, #41892, .T. ) ;
#24621=CARTESIAN_POINT ( 'NONE',  ( -3.310556943750002201, 15.58864905735837780, -129.6807724695661364 ) ) ;
#24623=CARTESIAN_POINT ( 'NONE',  ( -1.655278471874999990, 20.36702641396248481, -38.01827246956612782 ) ) ;
#24624=CARTESIAN_POINT ( 'NONE',  ( -3.310556943750000425, 19.41135094264165772, -30.93493913623279923 ) ) ;
#24626=CARTESIAN_POINT ( 'NONE',  ( -3.310556943750002645, 15.58864905735837247, -92.76827246956611361 ) ) ;
#24627=CARTESIAN_POINT ( 'NONE',  ( -3.500000000000002220, 15.47927405783632082, -26.57139747004410069 ) ) ;
#24628=ORIENTED_EDGE ( 'NONE', *, *, #36588, .F. ) ;
#24631=CARTESIAN_POINT ( 'NONE',  ( 1.655278471875001101, 20.36702641396249902, -138.1849391362327992 ) ) ;
#24633=CARTESIAN_POINT ( 'NONE',  ( -7.424026671074350129E-16, 13.45854811567263809, -98.71098080242150274 ) ) ;
#24634=CARTESIAN_POINT ( 'NONE',  ( 7.785697387528201340E-15, 14.00000000000002487, -136.4047308033774186 ) ) ;
#24635=CARTESIAN_POINT ( 'NONE',  ( -7.022189441860112050E-16, 13.67729811471671830, -59.51410580289948626 ) ) ;
#24636=CARTESIAN_POINT ( 'NONE',  ( 4.648177544792955347E-16, 21.00000000000001421, -59.90473080337743284 ) ) ;
#24637=CARTESIAN_POINT ( 'NONE',  ( 2.474675557024783212E-16, 21.54145188432739744, -87.90473080337741862 ) ) ;
#24638=CARTESIAN_POINT ( 'NONE',  ( -7.022189441860112050E-16, 13.67729811471672186, -69.60160580289947063 ) ) ;
#24640=CARTESIAN_POINT ( 'NONE',  ( 4.648177544792955347E-16, 21.00000000000001776, -83.90473080337743284 ) ) ;
#24642=CARTESIAN_POINT ( 'NONE',  ( 1.750000000000001110, 20.53108891324555074, -49.29431413575484555 ) ) ;
#24643=CARTESIAN_POINT ( 'NONE',  ( 3.310556943750001313, 19.41135094264166838, -120.1807724695661364 ) ) ;
#24644=CARTESIAN_POINT ( 'NONE',  ( 4.286263797015737581E-16, 14.00000000000002487, -149.5231586289125687 ) ) ;
#24647=VERTEX_POINT ( 'NONE', #1683 ) ;
#24648=CARTESIAN_POINT ( 'NONE',  ( -1.749999999999999778, 20.53108891324555785, -112.8213974700440900 ) ) ;
#24652=CARTESIAN_POINT ( 'NONE',  ( 3.500000000000001332, 17.50000000000001066, -37.46098080242150985 ) ) ;
#24655=CARTESIAN_POINT ( 'NONE',  ( -7.022189441860112050E-16, 13.67729811471672186, -71.51410580289947916 ) ) ;
#24656=FACE_OUTER_BOUND ( 'NONE', #4047, .T. ) ;
#24657=CARTESIAN_POINT ( 'NONE',  ( 3.500000000000000000, 15.47927405783632615, -69.54431413575484555 ) ) ;
#24660=CARTESIAN_POINT ( 'NONE',  ( -3.500000000000000000, 19.52072594216371826, -104.0443141357548171 ) ) ;
#24664=CARTESIAN_POINT ( 'NONE',  ( -1.655278471875002211, 14.63297358603754539, -80.59743913623280775 ) ) ;
#24666=EDGE_LOOP ( 'NONE', ( #25264, #9003, #21726, #8079, #7555, #4420, #29821, #14297, #8549, #23356, #25861, #2473, #8221, #33750, #8379, #10386, #31396, #29567, #7708, #283, #7606, #37870, #29505, #8425, #20101, #12358, #24501, #27332, #30338, #1377, #39659, #25548, #21045, #34904, #18203, #18942, #1688, #23722, #41398, #30410, #26487, #847, #36887, #13972, #7281, #7391, #4734, #30154, #2778, #38923, #21147, #32332, #23024, #18773, #19789, #20632, #25398, #22660, #13205, #14249, #9332, #16964, #589, #14763, #742, #9153, #28929, #24768, #36195, #38413, #40878, #34223, #24928, #31909, #26527, #511, #40972, #40084, #41277, #17391, #27318, #26760, #25446, #21507, #9597, #21773, #27434, #19997, #12121, #14673, #17495, #3108, #19715, #27696, #39215, #7012, #26071, #29917, #8526, #23948, #17181, #27378, #20422, #22038, #20307, #36475, #8853, #23289, #13239, #39444, #8592, #12765, #25026, #37523, #37485, #13284, #25448, #1736, #15547, #21917, #37062, #36538, #38727, #20741, #3758, #10205, #31123, #13837, #13994, #6742, #1944, #39823, #16555, #8965, #23825, #33913, #5031, #15452, #38616, #5546, #24351, #11835, #14808, #32744, #22297, #7650, #22722, #10890, #2942, #34645, #18166, #16301, #41966, #37778, #17073, #11875, #5067, #3301, #27028, #34480, #5238, #37371, #39531, #28427, #22148, #6390, #39653, #21672, #15355, #7074, #4084, #36185, #27643, #37636, #25601, #3316, #28812, #1800, #15752, #31236, #27227, #6239, #3047, #23619, #38246, #6648, #31276, #22981, #7980, #6451, #27492, #10859, #22039, #6974, #3565, #16406, #6917, #24231, #2293, #11610, #7056, #37518, #40808, #8480, #17216, #31917, #18113, #23222, #32127, #12529, #36579, #13409, #29348, #36097, #7826, #16501, #13540, #527, #22503, #41150, #38880, #32645, #5452, #24199, #26697, #1635, #25539, #39069, #14408, #30127, #4919, #5126, #29234, #33764, #13483, #18749, #8319, #25659, #19092, #24292, #14821, #26321, #10846, #15990 ) ) ;
#24670=CARTESIAN_POINT ( 'NONE',  ( 3.500000000000001332, 19.52072594216371826, -129.0713974700441042 ) ) ;
#24671=( BOUNDED_CURVE ( )  B_SPLINE_CURVE ( 2, ( #38570, #3671, #2843, #26438, #64, #16046, #41773, #16657, #26024 ),
 .UNSPECIFIED., .F., .T. ) 
 B_SPLINE_CURVE_WITH_KNOTS ( ( 3, 2, 2, 2, 3 ),
 ( 0.02291666666666666852, 0.02361111111111111049, 0.02500000000000000139, 0.02638888888888888881, 0.02708333333333333426 ),
 .UNSPECIFIED. ) 
 CURVE ( )  GEOMETRIC_REPRESENTATION_ITEM ( )  RATIONAL_B_SPLINE_CURVE ( ( 0.9330127018922194093, 0.9330127018922195203, 1.000000000000000000, 0.8660254037844387076, 1.000000000000000000, 0.8660254037844387076, 1.000000000000000000, 0.9330127018922191873, 0.9330127018922194093 ) ) 
 REPRESENTATION_ITEM ( '' )  );
#24672=( BOUNDED_CURVE ( )  B_SPLINE_CURVE ( 2, ( #37962, #27758, #2443, #21584, #21796, #28381, #40729, #38168, #40529 ),
 .UNSPECIFIED., .F., .F. ) 
 B_SPLINE_CURVE_WITH_KNOTS ( ( 3, 2, 2, 2, 3 ),
 ( 0.07291666666666667129, 0.07361111111111111327, 0.07499999999999999722, 0.07638888888888889506, 0.07708333333333333703 ),
 .UNSPECIFIED. ) 
 CURVE ( )  GEOMETRIC_REPRESENTATION_ITEM ( )  RATIONAL_B_SPLINE_CURVE ( ( 0.9330127018922194093, 0.9330127018922200755, 1.000000000000000000, 0.8660254037844387076, 1.000000000000000000, 0.8660254037844387076, 1.000000000000000000, 0.9330127018922194093, 0.9330127018922194093 ) ) 
 REPRESENTATION_ITEM ( '' )  );
#24673=CARTESIAN_POINT ( 'NONE',  ( -1.394453263437886604E-15, 14.00000000000002132, -126.4047308033774186 ) ) ;
#24674=CARTESIAN_POINT ( 'NONE',  ( 1.655278471874998436, 14.63297358603754006, -51.51827246956612782 ) ) ;
#24675=CARTESIAN_POINT ( 'NONE',  ( 1.655278471875001101, 20.36702641396249547, -108.1849391362327992 ) ) ;
#24677=CARTESIAN_POINT ( 'NONE',  ( 3.310556943750001313, 19.41135094264165772, -34.18077246956615056 ) ) ;
#24678=CARTESIAN_POINT ( 'NONE',  ( -3.310556943750001313, 17.50000000000001421, -58.85160580289947063 ) ) ;
#24679=CARTESIAN_POINT ( 'NONE',  ( 3.500000000000000000, 15.47927405783632970, -112.5443141357548456 ) ) ;
#24681=CARTESIAN_POINT ( 'NONE',  ( 1.655278471875001101, 20.36702641396249192, -97.09743913623280775 ) ) ;
#24683=CARTESIAN_POINT ( 'NONE',  ( -1.750000000000002220, 14.46891108675447946, -56.48806413671076143 ) ) ;
#24686=CARTESIAN_POINT ( 'NONE',  ( 1.750000000000001110, 20.53108891324555074, -66.29431413575484555 ) ) ;
#24688=CARTESIAN_POINT ( 'NONE',  ( 3.310556943750001313, 19.41135094264165772, -34.18077246956615056 ) ) ;
#24689=CARTESIAN_POINT ( 'NONE',  ( 3.500000000000000000, 15.47927405783632260, -54.23806413671076854 ) ) ;
#24690=CARTESIAN_POINT ( 'NONE',  ( 0.9378221735089281585, 14.00000000000001776, -92.66632260368298546 ) ) ;
#24691=CARTESIAN_POINT ( 'NONE',  ( 1.655278471874998436, 14.63297358603754894, -109.5182724695661420 ) ) ;
#24692=CARTESIAN_POINT ( 'NONE',  ( 2.340729813953370519E-16, 21.32270188528330834, -39.10160580289946353 ) ) ;
#24694=CARTESIAN_POINT ( 'NONE',  ( 0.9378221735089281585, 14.00000000000001243, -66.36007260463890134 ) ) ;
#24700=CARTESIAN_POINT ( 'NONE',  ( 2.340729813953370519E-16, 21.32270188528331190, -88.01410580289947916 ) ) ;
#24703=ORIENTED_EDGE ( 'NONE', *, *, #4765, .F. ) ;
#24713=VERTEX_POINT ( 'NONE', #40599 ) ;
#24715=AXIS2_PLACEMENT_3D ( 'NONE', #18567, #30548, #10989 ) ;
#24717=CARTESIAN_POINT ( 'NONE',  ( 0.000000000000000000, 17.50000000000002487, -149.5231586289125687 ) ) ;
#24721=CARTESIAN_POINT ( 'NONE',  ( 4.648177544792955347E-16, 21.00000000000002132, -108.9047308033774328 ) ) ;
#24722=CARTESIAN_POINT ( 'NONE',  ( 0.9378221735089302680, 14.00000000000002132, -140.3600726046389013 ) ) ;
#24723=CARTESIAN_POINT ( 'NONE',  ( 3.310556943750001313, 17.50000000000002487, -138.2641058028994792 ) ) ;
#24727=CARTESIAN_POINT ( 'NONE',  ( 2.340729813953370519E-16, 21.32270188528331900, -124.1016058028994706 ) ) ;
#24728=CARTESIAN_POINT ( 'NONE',  ( 1.655278471874998436, 14.63297358603754184, -58.51827246956613493 ) ) ;
#24731=CARTESIAN_POINT ( 'NONE',  ( -3.500000000000002220, 15.47927405783633503, -136.5713974700440758 ) ) ;
#24733=CARTESIAN_POINT ( 'NONE',  ( 1.655278471875001101, 20.36702641396249192, -79.18493913623279923 ) ) ;
#24734=CARTESIAN_POINT ( 'NONE',  ( 3.500000000000000000, 15.47927405783633503, -127.5443141357548313 ) ) ;
#24735=CARTESIAN_POINT ( 'NONE',  ( 1.655278471874998436, 14.63297358603754894, -114.4307724695661364 ) ) ;
#24739=CARTESIAN_POINT ( 'NONE',  ( 3.500000000000001776, 19.52072594216371115, -79.37764746908817415 ) ) ;
#24740=CARTESIAN_POINT ( 'NONE',  ( 0.9378221735089281585, 14.00000000000002132, -103.3600726046389013 ) ) ;
#24741=CARTESIAN_POINT ( 'NONE',  ( 3.310556943750001313, 19.41135094264166128, -49.18077246956614346 ) ) ;
#24742=CARTESIAN_POINT ( 'NONE',  ( -3.310556943750000425, 19.41135094264166838, -106.9349391362327850 ) ) ;
#24743=DIRECTION ( 'NONE',  ( -0.000000000000000000, 1.259100132267607459E-16, -1.000000000000000000 ) ) ;
#24747=CARTESIAN_POINT ( 'NONE',  ( 3.310556943750001313, 19.41135094264166838, -123.2682724695661278 ) ) ;
#24750=CARTESIAN_POINT ( 'NONE',  ( 0.9378221735089286026, 21.00000000000002842, -142.9493890021159643 ) ) ;
#24753=CARTESIAN_POINT ( 'NONE',  ( -3.500000000000001332, 17.50000000000001776, -100.9609808024215170 ) ) ;
#24754=CARTESIAN_POINT ( 'NONE',  ( 1.655278471874998436, 14.63297358603754184, -58.51827246956613493 ) ) ;
#24755=ORIENTED_EDGE ( 'NONE', *, *, #14219, .T. ) ;
#24756=CARTESIAN_POINT ( 'NONE',  ( -1.655278471875002211, 14.63297358603754539, -72.68493913623279923 ) ) ;
#24757=LINE ( 'NONE', #25385, #13568 ) ;
#24758=VECTOR ( 'NONE', #10153, 1000.000000000000000 ) ;
#24759=CARTESIAN_POINT ( 'NONE',  ( 4.286263797015737581E-16, 14.00000000000002487, -149.5231586289125687 ) ) ;
#24760=DIRECTION ( 'NONE',  ( 0.000000000000000000, 1.000000000000000000, 0.000000000000000000 ) ) ;
#24762=EDGE_CURVE ( 'NONE', #37080, #5763, #34545, .T. ) ;
#24764=CARTESIAN_POINT ( 'NONE',  ( 1.655278471874998436, 14.63297358603753828, -37.43077246956613635 ) ) ;
#24768=ORIENTED_EDGE ( 'NONE', *, *, #10865, .F. ) ;
#24770=CARTESIAN_POINT ( 'NONE',  ( -3.310556943750002645, 15.58864905735836714, -44.68077246956615056 ) ) ;
#24771=VERTEX_POINT ( 'NONE', #4872 ) ;
#24772=VERTEX_POINT ( 'NONE', #17848 ) ;
#24774=DIRECTION ( 'NONE',  ( -0.000000000000000000, 1.259100132267607459E-16, -1.000000000000000000 ) ) ;
#24776=CARTESIAN_POINT ( 'NONE',  ( 3.500000000000001332, 19.52072594216371826, -113.0713974700440900 ) ) ;
#24778=CARTESIAN_POINT ( 'NONE',  ( 1.750000000000001110, 20.53108891324555429, -89.29431413575483134 ) ) ;
#24779=CARTESIAN_POINT ( 'NONE',  ( -1.750000000000002220, 14.46891108675447768, -40.79431413575483845 ) ) ;
#24780=FACE_OUTER_BOUND ( 'NONE', #16151, .T. ) ;
#24782=CARTESIAN_POINT ( 'NONE',  ( 1.749999999999998224, 14.46891108675447946, -70.62764746908817415 ) ) ;
#24784=CARTESIAN_POINT ( 'NONE',  ( 3.500000000000001332, 19.52072594216371115, -96.37764746908815994 ) ) ;
#24786=CARTESIAN_POINT ( 'NONE',  ( 1.655278471874998436, 14.63297358603753651, -24.51827246956613138 ) ) ;
#24788=CARTESIAN_POINT ( 'NONE',  ( 3.310556943750001313, 17.50000000000002132, -128.2641058028994792 ) ) ;
#24791=CARTESIAN_POINT ( 'NONE',  ( 3.500000000000000000, 15.47927405783632793, -94.23806413671074722 ) ) ;
#24792=CARTESIAN_POINT ( 'NONE',  ( -1.655278471875002211, 14.63297358603755072, -121.6849391362327992 ) ) ;
#24794=CARTESIAN_POINT ( 'NONE',  ( -1.749999999999999778, 20.53108891324554719, -37.82139747004409003 ) ) ;
#24795=CARTESIAN_POINT ( 'NONE',  ( 0.9378221735089300459, 21.00000000000001066, -45.94938900211594301 ) ) ;
#24797=CARTESIAN_POINT ( 'NONE',  ( -1.655278471874999990, 20.36702641396249902, -141.0182724695661420 ) ) ;
#24798=CARTESIAN_POINT ( 'NONE',  ( 3.500000000000001332, 17.50000000000001066, -29.46098080242151696 ) ) ;
#24799=ADVANCED_FACE ( 'NONE', ( #18688 ), #8475, .T. ) ;
#24800=CARTESIAN_POINT ( 'NONE',  ( -7.022189441860112050E-16, 13.67729811471671830, -47.60160580289946353 ) ) ;
#24803=CARTESIAN_POINT ( 'NONE',  ( -1.655278471875002211, 14.63297358603754539, -75.68493913623279923 ) ) ;
#24805=CARTESIAN_POINT ( 'NONE',  ( -3.310556943750000425, 19.41135094264166838, -105.8474391362327935 ) ) ;
#24806=CARTESIAN_POINT ( 'NONE',  ( 3.310556943750001313, 17.50000000000001421, -68.26410580289947916 ) ) ;
#24808=( BOUNDED_CURVE ( )  B_SPLINE_CURVE ( 2, ( #24470, #37440, #21273, #30427, #31255, #1503, #4896, #2118, #14481 ),
 .UNSPECIFIED., .F., .T. ) 
 B_SPLINE_CURVE_WITH_KNOTS ( ( 3, 2, 2, 2, 3 ),
 ( 0.7562499999999999778, 0.7569444444444444198, 0.7583333333333333037, 0.7597222222222221877, 0.7604166666666666297 ),
 .UNSPECIFIED. ) 
 CURVE ( )  GEOMETRIC_REPRESENTATION_ITEM ( )  RATIONAL_B_SPLINE_CURVE ( ( 0.9330127018922194093, 0.9330127018922194093, 1.000000000000000000, 0.8660254037844387076, 1.000000000000000000, 0.8660254037844387076, 1.000000000000000000, 0.9330127018922194093, 0.9330127018922194093 ) ) 
 REPRESENTATION_ITEM ( '' )  );
#24809=CARTESIAN_POINT ( 'NONE',  ( 3.310556943750001313, 19.41135094264166838, -90.26827246956612782 ) ) ;
#24812=CARTESIAN_POINT ( 'NONE',  ( 0.000000000000000000, 17.50000000000002487, -149.5231586289125687 ) ) ;
#24814=CARTESIAN_POINT ( 'NONE',  ( -1.655278471875002211, 14.63297358603754361, -57.59743913623280065 ) ) ;
#24815=CYLINDRICAL_SURFACE ( 'NONE', #33516, 3.499999999999999556 ) ;
#24816=CARTESIAN_POINT ( 'NONE',  ( -3.310556943750001313, 17.50000000000002132, -109.7641058028994649 ) ) ;
#24817=AXIS2_PLACEMENT_3D ( 'NONE', #32349, #19376, #22779 ) ;
#24822=EDGE_LOOP ( 'NONE', ( #30725, #37779, #2315, #13186 ) ) ;
#24824=CARTESIAN_POINT ( 'NONE',  ( 3.310556943750001313, 17.50000000000001421, -65.26410580289946495 ) ) ;
#24826=VERTEX_POINT ( 'NONE', #21870 ) ;
#24827=EDGE_CURVE ( 'NONE', #3414, #1125, #10329, .T. ) ;
#24830=ADVANCED_FACE ( 'NONE', ( #40807 ), #5712, .T. ) ;
#24833=ORIENTED_EDGE ( 'NONE', *, *, #26271, .T. ) ;
#24835=CARTESIAN_POINT ( 'NONE',  ( 3.310556943749999981, 15.58864905735837425, -132.3474391362328220 ) ) ;
#24837=CARTESIAN_POINT ( 'NONE',  ( -3.310556943750002645, 15.58864905735836714, -40.76827246956613493 ) ) ;
#24838=CARTESIAN_POINT ( 'NONE',  ( 1.655278471875001101, 20.36702641396248481, -33.18493913623279923 ) ) ;
#24839=CARTESIAN_POINT ( 'NONE',  ( -3.310556943750001313, 17.50000000000001776, -92.85160580289947063 ) ) ;
#24840=CARTESIAN_POINT ( 'NONE',  ( 1.750000000000001110, 20.53108891324554719, -24.98806413671077209 ) ) ;
#24842=EDGE_CURVE ( 'NONE', #4210, #38089, #21039, .T. ) ;
#24844=CARTESIAN_POINT ( 'NONE',  ( -1.655278471875002211, 14.63297358603755427, -139.6849391362327708 ) ) ;
#24847=CARTESIAN_POINT ( 'NONE',  ( 3.500000000000000000, 15.47927405783632793, -87.23806413671076143 ) ) ;
#24848=CARTESIAN_POINT ( 'NONE',  ( 3.310556943749999981, 15.58864905735836537, -59.34743913623280775 ) ) ;
#24849=CARTESIAN_POINT ( 'NONE',  ( -0.9378221735089310451, 14.00000000000002309, -122.4493890021159501 ) ) ;
#24850=CARTESIAN_POINT ( 'NONE',  ( 3.500000000000001776, 19.52072594216371115, -83.07139747004410424 ) ) ;
#24851=CARTESIAN_POINT ( 'NONE',  ( 1.655278471875001101, 20.36702641396248836, -64.18493913623279923 ) ) ;
#24854=CARTESIAN_POINT ( 'NONE',  ( -3.310556943750001313, 17.50000000000002132, -121.7641058028994792 ) ) ;
#24855=CARTESIAN_POINT ( 'NONE',  ( -1.394453263437886604E-15, 14.00000000000002132, -130.4047308033774186 ) ) ;
#24858=CARTESIAN_POINT ( 'NONE',  ( -3.500000000000002220, 15.47927405783633503, -115.5713974700440900 ) ) ;
#24859=CARTESIAN_POINT ( 'NONE',  ( -1.394453263437886604E-15, 14.00000000000001066, -28.40473080337742928 ) ) ;
#24860=( NAMED_UNIT ( * ) PLANE_ANGLE_UNIT ( ) SI_UNIT ( $, .RADIAN. ) );
#24864=CARTESIAN_POINT ( 'NONE',  ( 3.310556943750001313, 17.50000000000001421, -69.26410580289947916 ) ) ;
#24865=DIRECTION ( 'NONE',  ( 0.000000000000000000, 1.000000000000000000, 0.000000000000000000 ) ) ;
#24868=CARTESIAN_POINT ( 'NONE',  ( 1.655278471875001101, 20.36702641396248481, -25.09743913623281486 ) ) ;
#24870=CARTESIAN_POINT ( 'NONE',  ( -1.655278471875002211, 14.63297358603754539, -78.59743913623280775 ) ) ;
#24872=ORIENTED_EDGE ( 'NONE', *, *, #3252, .T. ) ;
#24873=CARTESIAN_POINT ( 'NONE',  ( 4.648177544792955347E-16, 21.00000000000002132, -128.2109808024214885 ) ) ;
#24876=CARTESIAN_POINT ( 'NONE',  ( -1.394453263437886604E-15, 14.00000000000001776, -102.7109808024215027 ) ) ;
#24880=CARTESIAN_POINT ( 'NONE',  ( 1.655278471874998436, 14.63297358603754006, -49.51827246956613493 ) ) ;
#24881=CARTESIAN_POINT ( 'NONE',  ( -7.022189441860112050E-16, 13.67729811471672718, -109.6016058028994564 ) ) ;
#24882=ORIENTED_EDGE ( 'NONE', *, *, #36346, .T. ) ;
#24883=CARTESIAN_POINT ( 'NONE',  ( 3.310556943750001313, 19.41135094264165772, -37.18077246956613635 ) ) ;
#24884=CARTESIAN_POINT ( 'NONE',  ( -7.022189441860112050E-16, 13.67729811471671830, -58.60160580289947063 ) ) ;
#24885=CARTESIAN_POINT ( 'NONE',  ( 3.500000000000001776, 19.52072594216371826, -110.3776474690881884 ) ) ;
#24887=CARTESIAN_POINT ( 'NONE',  ( -7.022189441860112050E-16, 13.67729811471672363, -92.51410580289949337 ) ) ;
#24892=CARTESIAN_POINT ( 'NONE',  ( -3.500000000000001332, 17.50000000000001421, -64.96098080242150274 ) ) ;
#24893=EDGE_CURVE ( 'NONE', #18307, #9218, #11436, .T. ) ;
#24895=CARTESIAN_POINT ( 'NONE',  ( -7.022189441860112050E-16, 13.67729811471671475, -28.51410580289948271 ) ) ;
#24897=CARTESIAN_POINT ( 'NONE',  ( -7.424026671074350129E-16, 13.45854811567263454, -56.40473080337743284 ) ) ;
#24900=CARTESIAN_POINT ( 'NONE',  ( 3.310556943749999981, 15.58864905735837247, -109.4349391362327992 ) ) ;
#24901=CARTESIAN_POINT ( 'NONE',  ( -1.655278471874999990, 20.36702641396248481, -40.01827246956612782 ) ) ;
#24903=CARTESIAN_POINT ( 'NONE',  ( 3.500000000000001332, 17.50000000000002487, -135.4609808024214885 ) ) ;
#24906=CARTESIAN_POINT ( 'NONE',  ( 4.648177544792955347E-16, 21.00000000000001421, -50.21098080242150985 ) ) ;
#24908=CARTESIAN_POINT ( 'NONE',  ( 1.655278471875001101, 20.36702641396249192, -87.09743913623280775 ) ) ;
#24909=CARTESIAN_POINT ( 'NONE',  ( -3.500000000000002220, 15.47927405783633503, -135.5713974700441042 ) ) ;
#24911=ORIENTED_EDGE ( 'NONE', *, *, #7707, .T. ) ;
#24913=CARTESIAN_POINT ( 'NONE',  ( 0.9378221735089281585, 14.00000000000002132, -109.6663226036829855 ) ) ;
#24922=( BOUNDED_CURVE ( )  B_SPLINE_CURVE ( 2, ( #12184, #34735, #24969, #25176, #8791, #14767, #21761, #27935, #11553 ),
 .UNSPECIFIED., .F., .T. ) 
 B_SPLINE_CURVE_WITH_KNOTS ( ( 3, 2, 2, 2, 3 ),
 ( 0.3645833333333333148, 0.3652777777777777568, 0.3666666666666666408, 0.3680555555555555802, 0.3687500000000000222 ),
 .UNSPECIFIED. ) 
 CURVE ( )  GEOMETRIC_REPRESENTATION_ITEM ( )  RATIONAL_B_SPLINE_CURVE ( ( 0.9330127018922194093, 0.9330127018922194093, 1.000000000000000000, 0.8660254037844387076, 1.000000000000000000, 0.8660254037844387076, 1.000000000000000000, 0.9330127018922194093, 0.9330127018922194093 ) ) 
 REPRESENTATION_ITEM ( '' )  );
#24923=( BOUNDED_CURVE ( )  B_SPLINE_CURVE ( 2, ( #2078, #22273, #41644, #25482, #38446, #21438, #9308, #35246, #19088 ),
 .UNSPECIFIED., .F., .F. ) 
 B_SPLINE_CURVE_WITH_KNOTS ( ( 3, 2, 2, 2, 3 ),
 ( 0.2187500000000000000, 0.2194444444444444420, 0.2208333333333333259, 0.2222222222222222099, 0.2229166666666666796 ),
 .UNSPECIFIED. ) 
 CURVE ( )  GEOMETRIC_REPRESENTATION_ITEM ( )  RATIONAL_B_SPLINE_CURVE ( ( 0.9330127018922194093, 0.9330127018922194093, 1.000000000000000000, 0.8660254037844387076, 1.000000000000000000, 0.8660254037844387076, 1.000000000000000000, 0.9330127018922180770, 0.9330127018922194093 ) ) 
 REPRESENTATION_ITEM ( '' )  );
#24928=ORIENTED_EDGE ( 'NONE', *, *, #28007, .F. ) ;
#24930=DIRECTION ( 'NONE',  ( 0.000000000000000000, 1.000000000000000000, 0.000000000000000000 ) ) ;
#24932=CARTESIAN_POINT ( 'NONE',  ( 3.310556943750001313, 19.41135094264167549, -138.1807724695661648 ) ) ;
#24933=DIRECTION ( 'NONE',  ( 0.000000000000000000, 1.000000000000000000, 0.000000000000000000 ) ) ;
#24936=CARTESIAN_POINT ( 'NONE',  ( -1.394453263437886604E-15, 14.00000000000001421, -54.71098080242151696 ) ) ;
#24937=CARTESIAN_POINT ( 'NONE',  ( -7.022189441860112050E-16, 13.67729811471672718, -123.6016058028994564 ) ) ;
#24938=CARTESIAN_POINT ( 'NONE',  ( 3.310556943750001313, 19.41135094264166128, -57.26827246956612782 ) ) ;
#24941=CARTESIAN_POINT ( 'NONE',  ( 1.750000000000001110, 20.53108891324556140, -137.9880641367107614 ) ) ;
#24943=CARTESIAN_POINT ( 'NONE',  ( 1.655278471875001101, 20.36702641396249192, -78.18493913623279923 ) ) ;
#24944=CARTESIAN_POINT ( 'NONE',  ( -3.500000000000002220, 15.47927405783633503, -128.8776474690881741 ) ) ;
#24945=CARTESIAN_POINT ( 'NONE',  ( 1.655278471875001101, 20.36702641396249547, -111.0974391362328078 ) ) ;
#24950=CARTESIAN_POINT ( 'NONE',  ( 3.500000000000000000, 15.47927405783632437, -79.54431413575483134 ) ) ;
#24951=CARTESIAN_POINT ( 'NONE',  ( 3.500000000000001332, 19.52072594216371826, -103.0713974700440900 ) ) ;
#24952=CARTESIAN_POINT ( 'NONE',  ( -3.310556943750000425, 19.41135094264165772, -45.84743913623280775 ) ) ;
#24953=CARTESIAN_POINT ( 'NONE',  ( 3.310556943750001313, 17.50000000000002132, -103.3516058028994564 ) ) ;
#24956=CARTESIAN_POINT ( 'NONE',  ( -0.9378221735089310451, 14.00000000000001599, -72.44938900211595012 ) ) ;
#24957=VERTEX_POINT ( 'NONE', #8016 ) ;
#24958=CARTESIAN_POINT ( 'NONE',  ( 3.310556943749999981, 15.58864905735837425, -123.4349391362327992 ) ) ;
#24962=CARTESIAN_POINT ( 'NONE',  ( -1.394453263437886604E-15, 14.00000000000001066, -32.40473080337742573 ) ) ;
#24963=CARTESIAN_POINT ( 'NONE',  ( -1.750000000000002220, 14.46891108675448123, -71.48806413671076143 ) ) ;
#24967=CARTESIAN_POINT ( 'NONE',  ( 3.310556943750001313, 19.41135094264166838, -75.26827246956612782 ) ) ;
#24969=CARTESIAN_POINT ( 'NONE',  ( 1.749999999999998224, 14.46891108675448301, -99.32139747004409003 ) ) ;
#24972=CARTESIAN_POINT ( 'NONE',  ( -1.655278471874999990, 20.36702641396248481, -32.93077246956614346 ) ) ;
#24975=ORIENTED_EDGE ( 'NONE', *, *, #26192, .T. ) ;
#24978=CARTESIAN_POINT ( 'NONE',  ( 3.310556943750001313, 19.41135094264166128, -47.18077246956614346 ) ) ;
#24979=VERTEX_POINT ( 'NONE', #27376 ) ;
#24980=ORIENTED_EDGE ( 'NONE', *, *, #1469, .F. ) ;
#24984=CARTESIAN_POINT ( 'NONE',  ( 4.648177544792955347E-16, 21.00000000000001421, -62.90473080337742573 ) ) ;
#24985=CARTESIAN_POINT ( 'NONE',  ( 0.000000000000000000, 21.00000000000002487, -149.5231586289125687 ) ) ;
#24986=CARTESIAN_POINT ( 'NONE',  ( 1.749999999999998224, 14.46891108675447413, -37.62764746908817415 ) ) ;
#24987=CARTESIAN_POINT ( 'NONE',  ( 3.500000000000000000, 15.47927405783632793, -86.54431413575483134 ) ) ;
#24988=CARTESIAN_POINT ( 'NONE',  ( 4.286263797015737581E-16, 14.00000000000002487, -149.5231586289125687 ) ) ;
#24991=CARTESIAN_POINT ( 'NONE',  ( 1.655278471875001101, 20.36702641396248481, -26.18493913623279212 ) ) ;
#24993=CARTESIAN_POINT ( 'NONE',  ( -3.310556943750002645, 15.58864905735837780, -126.6807724695661221 ) ) ;
#24994=EDGE_CURVE ( 'NONE', #11063, #41241, #24197, .T. ) ;
#24997=( BOUNDED_CURVE ( )  B_SPLINE_CURVE ( 2, ( #30588, #27197, #33141, #33789, #30166, #13798, #1043, #14431, #27406 ),
 .UNSPECIFIED., .F., .F. ) 
 B_SPLINE_CURVE_WITH_KNOTS ( ( 3, 2, 2, 2, 3 ),
 ( 0.3562500000000000111, 0.3569444444444444531, 0.3583333333333333370, 0.3597222222222222210, 0.3604166666666666630 ),
 .UNSPECIFIED. ) 
 CURVE ( )  GEOMETRIC_REPRESENTATION_ITEM ( )  RATIONAL_B_SPLINE_CURVE ( ( 0.9330127018922194093, 0.9330127018922194093, 1.000000000000000000, 0.8660254037844387076, 1.000000000000000000, 0.8660254037844387076, 1.000000000000000000, 0.9330127018922194093, 0.9330127018922194093 ) ) 
 REPRESENTATION_ITEM ( '' )  );
#24999=CARTESIAN_POINT ( 'NONE',  ( 3.310556943750001313, 19.41135094264166838, -121.2682724695661420 ) ) ;
#25000=CARTESIAN_POINT ( 'NONE',  ( 0.000000000000000000, 17.50000000000002487, -149.5231586289125687 ) ) ;
#25001=CARTESIAN_POINT ( 'NONE',  ( 2.474675557024783212E-16, 21.54145188432739033, -35.90473080337743284 ) ) ;
#25004=CARTESIAN_POINT ( 'NONE',  ( -3.310556943750001313, 17.50000000000002487, -139.8516058028994564 ) ) ;
#25005=CARTESIAN_POINT ( 'NONE',  ( 1.749999999999998224, 14.46891108675447413, -29.62764746908817770 ) ) ;
#25006=CARTESIAN_POINT ( 'NONE',  ( -7.022189441860112050E-16, 13.67729811471671830, -48.60160580289947774 ) ) ;
#25008=CARTESIAN_POINT ( 'NONE',  ( 4.648177544792955347E-16, 21.00000000000002132, -104.2109808024215027 ) ) ;
#25009=CARTESIAN_POINT ( 'NONE',  ( 3.310556943749999981, 15.58864905735836714, -72.43493913623278502 ) ) ;
#25011=CARTESIAN_POINT ( 'NONE',  ( -3.310556943750000425, 19.41135094264166838, -97.84743913623280775 ) ) ;
#25012=CARTESIAN_POINT ( 'NONE',  ( 3.310556943750001313, 17.50000000000001421, -69.26410580289947916 ) ) ;
#25014=ORIENTED_EDGE ( 'NONE', *, *, #9584, .F. ) ;
#25015=CARTESIAN_POINT ( 'NONE',  ( 3.310556943750001313, 19.41135094264166838, -93.26827246956612782 ) ) ;
#25017=CARTESIAN_POINT ( 'NONE',  ( 3.500000000000001332, 19.52072594216370760, -67.37764746908817415 ) ) ;
#25018=CARTESIAN_POINT ( 'NONE',  ( -3.500000000000001332, 17.50000000000001776, -84.96098080242150274 ) ) ;
#25019=CARTESIAN_POINT ( 'NONE',  ( 1.750000000000001110, 20.53108891324555785, -117.2943141357548313 ) ) ;
#25020=CARTESIAN_POINT ( 'NONE',  ( 3.310556943750001313, 17.50000000000001421, -54.26410580289947916 ) ) ;
#25021=CARTESIAN_POINT ( 'NONE',  ( 4.648177544792955347E-16, 21.00000000000001066, -24.90473080337743284 ) ) ;
#25022=CARTESIAN_POINT ( 'NONE',  ( -7.022189441860112050E-16, 13.67729811471672541, -108.5141058028994649 ) ) ;
#25026=ORIENTED_EDGE ( 'NONE', *, *, #34964, .F. ) ;
#25028=CARTESIAN_POINT ( 'NONE',  ( 3.310556943750001313, 19.41135094264166128, -64.18077246956613635 ) ) ;
#25030=ORIENTED_EDGE ( 'NONE', *, *, #2271, .T. ) ;
#25038=CARTESIAN_POINT ( 'NONE',  ( 1.655278471875001101, 20.36702641396249902, -131.0974391362328220 ) ) ;
#25039=CARTESIAN_POINT ( 'NONE',  ( -3.500000000000001332, 17.50000000000002132, -128.6547308033774186 ) ) ;
#25040=CARTESIAN_POINT ( 'NONE',  ( 1.655278471875001101, 20.36702641396248481, -41.18493913623279212 ) ) ;
#25041=CARTESIAN_POINT ( 'NONE',  ( -3.310556943750000425, 19.41135094264165772, -25.93493913623279212 ) ) ;
#25042=CARTESIAN_POINT ( 'NONE',  ( 3.310556943750001313, 17.50000000000001776, -95.35160580289945642 ) ) ;
#25043=CARTESIAN_POINT ( 'NONE',  ( 3.500000000000001776, 19.52072594216370405, -25.07139747004409713 ) ) ;
#25044=ORIENTED_EDGE ( 'NONE', *, *, #34698, .T. ) ;
#25047=CARTESIAN_POINT ( 'NONE',  ( 3.310556943749999981, 15.58864905735837780, -138.4349391362327708 ) ) ;
#25050=CARTESIAN_POINT ( 'NONE',  ( 3.500000000000001332, 17.50000000000002487, -132.1547308033774186 ) ) ;
#25051=CARTESIAN_POINT ( 'NONE',  ( 2.474675557024783212E-16, 21.54145188432739744, -80.90473080337743284 ) ) ;
#25052=CARTESIAN_POINT ( 'NONE',  ( 3.310556943750001313, 19.41135094264166483, -65.26827246956614204 ) ) ;
#25055=CARTESIAN_POINT ( 'NONE',  ( 3.500000000000000000, 15.47927405783632082, -47.54431413575484555 ) ) ;
#25057=EDGE_LOOP ( 'NONE', ( #25014, #39815, #35951, #1443 ) ) ;
#25059=CARTESIAN_POINT ( 'NONE',  ( -7.022189441860112050E-16, 13.67729811471672896, -120.5141058028994792 ) ) ;
#25064=CARTESIAN_POINT ( 'NONE',  ( 1.750000000000001110, 20.53108891324555785, -109.9880641367107614 ) ) ;
#25065=LINE ( 'NONE', #28449, #24061 ) ;
#25067=CARTESIAN_POINT ( 'NONE',  ( 0.9378221735089300459, 21.00000000000001421, -65.25563900116003424 ) ) ;
#25069=CARTESIAN_POINT ( 'NONE',  ( 1.655278471874998436, 14.63297358603754361, -73.43077246956613635 ) ) ;
#25070=LINE ( 'NONE', #28454, #25963 ) ;
#25071=CARTESIAN_POINT ( 'NONE',  ( 4.648177544792955347E-16, 21.00000000000002132, -122.9047308033774044 ) ) ;
#25073=ORIENTED_EDGE ( 'NONE', *, *, #3480, .T. ) ;
#25074=DIRECTION ( 'NONE',  ( -0.000000000000000000, 1.259100132267607459E-16, -1.000000000000000000 ) ) ;
#25075=CARTESIAN_POINT ( 'NONE',  ( -3.310556943750002645, 15.58864905735837070, -80.68077246956613635 ) ) ;
#25076=ORIENTED_EDGE ( 'NONE', *, *, #4139, .T. ) ;
#25077=ORIENTED_EDGE ( 'NONE', *, *, #17543, .T. ) ;
#25078=CARTESIAN_POINT ( 'NONE',  ( -1.394453263437886604E-15, 14.00000000000001066, -48.40473080337742573 ) ) ;
#25079=EDGE_CURVE ( 'NONE', #36084, #11305, #37784, .T. ) ;
#25081=LINE ( 'NONE', #5088, #4273 ) ;
#25083=ADVANCED_FACE ( 'NONE', ( #29326 ), #12546, .T. ) ;
#25084=DIRECTION ( 'NONE',  ( -0.000000000000000000, 1.259100132267607459E-16, -1.000000000000000000 ) ) ;
#25085=CARTESIAN_POINT ( 'NONE',  ( -3.310556943750001313, 17.50000000000001066, -46.85160580289945642 ) ) ;
#25086=CARTESIAN_POINT ( 'NONE',  ( 3.310556943750001313, 17.50000000000002132, -111.3516058028994564 ) ) ;
#25087=ORIENTED_EDGE ( 'NONE', *, *, #40725, .T. ) ;
#25089=CARTESIAN_POINT ( 'NONE',  ( -3.310556943750000425, 19.41135094264165772, -36.84743913623281486 ) ) ;
#25090=CARTESIAN_POINT ( 'NONE',  ( 3.310556943750001313, 19.41135094264166128, -61.26827246956612782 ) ) ;
#25091=CARTESIAN_POINT ( 'NONE',  ( 3.500000000000000000, 15.47927405783632793, -106.5443141357548313 ) ) ;
#25093=CARTESIAN_POINT ( 'NONE',  ( 3.310556943750001313, 19.41135094264166483, -92.18077246956612214 ) ) ;
#25094=CARTESIAN_POINT ( 'NONE',  ( 1.750000000000001110, 20.53108891324555429, -96.98806413671076143 ) ) ;
#25096=CARTESIAN_POINT ( 'NONE',  ( 3.500000000000001332, 19.52072594216371115, -85.07139747004407582 ) ) ;
#25099=CARTESIAN_POINT ( 'NONE',  ( 1.750000000000001110, 20.53108891324555074, -62.29431413575483845 ) ) ;
#25101=CARTESIAN_POINT ( 'NONE',  ( -3.310556943750002645, 15.58864905735836537, -26.68077246956614346 ) ) ;
#25102=EDGE_CURVE ( 'NONE', #3232, #2623, #39132, .T. ) ;
#25103=CARTESIAN_POINT ( 'NONE',  ( -1.750000000000002220, 14.46891108675447768, -51.48806413671076854 ) ) ;
#25104=CARTESIAN_POINT ( 'NONE',  ( 1.749999999999998224, 14.46891108675447946, -77.62764746908817415 ) ) ;
#25105=CARTESIAN_POINT ( 'NONE',  ( -3.310556943750002201, 15.58864905735837425, -108.7682724695661420 ) ) ;
#25106=CARTESIAN_POINT ( 'NONE',  ( 3.310556943749999981, 15.58864905735836182, -31.43493913623279923 ) ) ;
#25108=CARTESIAN_POINT ( 'NONE',  ( 4.648177544792955347E-16, 21.00000000000002487, -130.2109808024214885 ) ) ;
#25111=CARTESIAN_POINT ( 'NONE',  ( 0.000000000000000000, 21.00000000000002487, -149.5231586289125687 ) ) ;
#25113=CARTESIAN_POINT ( 'NONE',  ( -1.655278471874999990, 20.36702641396249192, -87.93077246956613635 ) ) ;
#25115=VECTOR ( 'NONE', #8995, 1000.000000000000000 ) ;
#25118=CARTESIAN_POINT ( 'NONE',  ( -3.500000000000000000, 19.52072594216370760, -50.73806413671077564 ) ) ;
#25122=CARTESIAN_POINT ( 'NONE',  ( -1.655278471875002211, 14.63297358603754894, -97.59743913623280775 ) ) ;
#25124=VERTEX_POINT ( 'NONE', #18926 ) ;
#25126=ORIENTED_EDGE ( 'NONE', *, *, #38769, .T. ) ;
#25130=CARTESIAN_POINT ( 'NONE',  ( 4.286263797015737581E-16, 14.00000000000002487, -149.5231586289125687 ) ) ;
#25133=EDGE_CURVE ( 'NONE', #12462, #12520, #17424, .T. ) ;
#25135=CARTESIAN_POINT ( 'NONE',  ( 3.500000000000001332, 17.50000000000001776, -91.15473080337743284 ) ) ;
#25137=CARTESIAN_POINT ( 'NONE',  ( -7.022189441860112050E-16, 13.67729811471672896, -136.5141058028994792 ) ) ;
#25138=CARTESIAN_POINT ( 'NONE',  ( 1.749999999999998224, 14.46891108675448656, -133.6276474690881741 ) ) ;
#25139=EDGE_LOOP ( 'NONE', ( #9648, #31426, #24040, #29782 ) ) ;
#25140=CARTESIAN_POINT ( 'NONE',  ( 1.750000000000001110, 20.53108891324555074, -72.98806413671076143 ) ) ;
#25141=CARTESIAN_POINT ( 'NONE',  ( 3.310556943750001313, 17.50000000000002132, -123.3516058028994564 ) ) ;
#25142=CARTESIAN_POINT ( 'NONE',  ( -3.310556943750001313, 17.50000000000001421, -50.85160580289946353 ) ) ;
#25145=CARTESIAN_POINT ( 'NONE',  ( 3.500000000000001776, 19.52072594216372181, -136.0713974700441042 ) ) ;
#25148=CARTESIAN_POINT ( 'NONE',  ( -1.655278471874999990, 20.36702641396249192, -77.01827246956612782 ) ) ;
#25149=CARTESIAN_POINT ( 'NONE',  ( 1.749999999999998224, 14.46891108675448478, -120.6276474690881741 ) ) ;
#25150=CARTESIAN_POINT ( 'NONE',  ( -1.655278471874999990, 20.36702641396249547, -108.9307724695661506 ) ) ;
#25151=CARTESIAN_POINT ( 'NONE',  ( 0.9378221735089281585, 14.00000000000001776, -81.36007260463891555 ) ) ;
#25154=CARTESIAN_POINT ( 'NONE',  ( 1.749999999999998224, 14.46891108675448123, -81.62764746908818836 ) ) ;
#25156=CARTESIAN_POINT ( 'NONE',  ( 1.655278471875001101, 20.36702641396248481, -45.09743913623280775 ) ) ;
#25158=CARTESIAN_POINT ( 'NONE',  ( -1.655278471874999990, 20.36702641396249192, -102.0182724695661278 ) ) ;
#25159=CARTESIAN_POINT ( 'NONE',  ( 4.648177544792955347E-16, 21.00000000000001776, -83.21098080242150274 ) ) ;
#25160=CARTESIAN_POINT ( 'NONE',  ( 0.000000000000000000, 17.50000000000002487, -149.5231586289125687 ) ) ;
#25161=VERTEX_POINT ( 'NONE', #12332 ) ;
#25162=CARTESIAN_POINT ( 'NONE',  ( -1.655278471875002211, 14.63297358603755249, -123.6849391362327992 ) ) ;
#25163=LINE ( 'NONE', #13019, #41757 ) ;
#25167=CARTESIAN_POINT ( 'NONE',  ( -0.9378221735089310451, 14.00000000000001599, -57.44938900211595723 ) ) ;
#25170=ORIENTED_EDGE ( 'NONE', *, *, #28515, .F. ) ;
#25171=( BOUNDED_CURVE ( )  B_SPLINE_CURVE ( 2, ( #11800, #34142, #17571, #15003, #1403, #40325, #24172, #24795, #37142 ),
 .UNSPECIFIED., .F., .T. ) 
 B_SPLINE_CURVE_WITH_KNOTS ( ( 3, 2, 2, 2, 3 ),
 ( 0.8062500000000000222, 0.8069444444444444642, 0.8083333333333333481, 0.8097222222222222321, 0.8104166666666666741 ),
 .UNSPECIFIED. ) 
 CURVE ( )  GEOMETRIC_REPRESENTATION_ITEM ( )  RATIONAL_B_SPLINE_CURVE ( ( 0.9330127018922194093, 0.9330127018922194093, 1.000000000000000000, 0.8660254037844387076, 1.000000000000000000, 0.8660254037844387076, 1.000000000000000000, 0.9330127018922194093, 0.9330127018922194093 ) ) 
 REPRESENTATION_ITEM ( '' )  );
#25172=CARTESIAN_POINT ( 'NONE',  ( 2.340729813953370519E-16, 21.32270188528331190, -73.10160580289948484 ) ) ;
#25176=CARTESIAN_POINT ( 'NONE',  ( 3.500000000000000000, 15.47927405783632970, -99.23806413671076143 ) ) ;
#25179=CARTESIAN_POINT ( 'NONE',  ( 4.648177544792955347E-16, 21.00000000000001421, -70.21098080242150274 ) ) ;
#25181=CARTESIAN_POINT ( 'NONE',  ( 3.310556943749999981, 15.58864905735836182, -35.34743913623280775 ) ) ;
#25182=CARTESIAN_POINT ( 'NONE',  ( 3.500000000000000000, 15.47927405783632970, -107.2380641367107614 ) ) ;
#25188=CARTESIAN_POINT ( 'NONE',  ( 1.655278471875001101, 20.36702641396248836, -49.09743913623280775 ) ) ;
#25189=VERTEX_POINT ( 'NONE', #39115 ) ;
#25192=CARTESIAN_POINT ( 'NONE',  ( -7.424026671074350129E-16, 13.45854811567263098, -24.71098080242150985 ) ) ;
#25194=CARTESIAN_POINT ( 'NONE',  ( 3.500000000000000000, 15.47927405783632082, -43.54431413575483845 ) ) ;
#25195=CARTESIAN_POINT ( 'NONE',  ( -1.749999999999999778, 20.53108891324554719, -32.12764746908818125 ) ) ;
#25196=CARTESIAN_POINT ( 'NONE',  ( 4.286263797015737581E-16, 14.00000000000002487, -149.5231586289125687 ) ) ;
#25197=CARTESIAN_POINT ( 'NONE',  ( 3.500000000000001332, 17.50000000000001776, -82.46098080242150274 ) ) ;
#25200=CARTESIAN_POINT ( 'NONE',  ( 1.750000000000001110, 20.53108891324556140, -142.2943141357548313 ) ) ;
#25201=LINE ( 'NONE', #21787, #41520 ) ;
#25202=CARTESIAN_POINT ( 'NONE',  ( -3.310556943750002645, 15.58864905735837780, -121.6807724695661364 ) ) ;
#25205=CARTESIAN_POINT ( 'NONE',  ( -7.022189441860112050E-16, 13.67729811471672718, -116.6016058028994564 ) ) ;
#25206=CARTESIAN_POINT ( 'NONE',  ( 4.648177544792955347E-16, 21.00000000000001421, -55.90473080337743284 ) ) ;
#25207=CARTESIAN_POINT ( 'NONE',  ( -3.500000000000001332, 17.50000000000001066, -35.65473080337743284 ) ) ;
#25209=CARTESIAN_POINT ( 'NONE',  ( -3.310556943750000425, 19.41135094264167549, -140.9349391362327708 ) ) ;
#25211=DIRECTION ( 'NONE',  ( 0.000000000000000000, 1.000000000000000000, 0.000000000000000000 ) ) ;
#25212=CARTESIAN_POINT ( 'NONE',  ( 1.655278471874998436, 14.63297358603754006, -46.51827246956613493 ) ) ;
#25214=CARTESIAN_POINT ( 'NONE',  ( -0.9378221735089310451, 14.00000000000001599, -72.75563900116003424 ) ) ;
#25215=CARTESIAN_POINT ( 'NONE',  ( -3.310556943750001313, 17.50000000000001421, -69.85160580289947063 ) ) ;
#25217=CARTESIAN_POINT ( 'NONE',  ( 3.310556943750001313, 17.50000000000001421, -72.26410580289947916 ) ) ;
#25220=CARTESIAN_POINT ( 'NONE',  ( 1.655278471874998436, 14.63297358603754539, -89.51827246956612782 ) ) ;
#25222=CARTESIAN_POINT ( 'NONE',  ( 4.648177544792955347E-16, 21.00000000000001421, -67.21098080242148853 ) ) ;
#25223=CARTESIAN_POINT ( 'NONE',  ( 4.648177544792955347E-16, 21.00000000000002132, -106.2109808024215027 ) ) ;
#25224=CARTESIAN_POINT ( 'NONE',  ( 3.310556943749999981, 15.58864905735836182, -49.34743913623280775 ) ) ;
#25226=CARTESIAN_POINT ( 'NONE',  ( -3.310556943750000425, 19.41135094264166838, -110.8474391362328078 ) ) ;
#25228=VERTEX_POINT ( 'NONE', #6790 ) ;
#25230=EDGE_LOOP ( 'NONE', ( #40797, #1938, #13864 ) ) ;
#25232=EDGE_CURVE ( 'NONE', #14931, #15239, #4367, .T. ) ;
#25233=CARTESIAN_POINT ( 'NONE',  ( 3.310556943750001313, 19.41135094264166128, -65.18077246956615056 ) ) ;
#25234=ORIENTED_EDGE ( 'NONE', *, *, #16302, .F. ) ;
#25235=ORIENTED_EDGE ( 'NONE', *, *, #33436, .T. ) ;
#25240=ORIENTED_EDGE ( 'NONE', *, *, #29986, .T. ) ;
#25242=CARTESIAN_POINT ( 'NONE',  ( -1.749999999999999778, 20.53108891324555074, -55.12764746908817415 ) ) ;
#25243=CARTESIAN_POINT ( 'NONE',  ( -3.310556943750002201, 15.58864905735837780, -132.6807724695661364 ) ) ;
#25246=CARTESIAN_POINT ( 'NONE',  ( -1.655278471875002211, 14.63297358603754184, -41.68493913623279212 ) ) ;
#25247=CARTESIAN_POINT ( 'NONE',  ( 3.310556943750001313, 19.41135094264165772, -30.26827246956613493 ) ) ;
#25248=CARTESIAN_POINT ( 'NONE',  ( 3.310556943750001313, 19.41135094264166483, -95.26827246956612782 ) ) ;
#25249=CARTESIAN_POINT ( 'NONE',  ( -3.310556943750000425, 19.41135094264167549, -142.8474391362327935 ) ) ;
#25253=CARTESIAN_POINT ( 'NONE',  ( 3.310556943749999981, 15.58864905735837425, -132.4349391362327992 ) ) ;
#25255=CARTESIAN_POINT ( 'NONE',  ( 3.500000000000001332, 17.50000000000001066, -28.15473080337743639 ) ) ;
#25256=CARTESIAN_POINT ( 'NONE',  ( 4.648177544792955347E-16, 21.00000000000002132, -123.2109808024214885 ) ) ;
#25257=CARTESIAN_POINT ( 'NONE',  ( 1.749999999999998224, 14.46891108675447946, -79.32139747004410424 ) ) ;
#25258=CARTESIAN_POINT ( 'NONE',  ( -3.310556943750002201, 15.58864905735836892, -63.76827246956613493 ) ) ;
#25260=CARTESIAN_POINT ( 'NONE',  ( -1.750000000000002220, 14.46891108675449011, -136.7943141357548598 ) ) ;
#25261=FACE_OUTER_BOUND ( 'NONE', #27018, .T. ) ;
#25262=CARTESIAN_POINT ( 'NONE',  ( 1.655278471875001101, 20.36702641396249192, -88.18493913623279923 ) ) ;
#25263=CARTESIAN_POINT ( 'NONE',  ( 4.648177544792955347E-16, 21.00000000000002487, -129.9047308033774186 ) ) ;
#25264=ORIENTED_EDGE ( 'NONE', *, *, #26875, .T. ) ;
#25265=CARTESIAN_POINT ( 'NONE',  ( -3.310556943750001313, 17.50000000000002132, -112.7641058028994792 ) ) ;
#25269=CARTESIAN_POINT ( 'NONE',  ( -3.500000000000001332, 17.50000000000002132, -110.6547308033774328 ) ) ;
#25270=CARTESIAN_POINT ( 'NONE',  ( -0.9378221735089288247, 14.00000000000002309, -139.7556390011600342 ) ) ;
#25272=CARTESIAN_POINT ( 'NONE',  ( -1.749999999999999778, 20.53108891324554719, -32.82139747004410424 ) ) ;
#25274=CARTESIAN_POINT ( 'NONE',  ( 3.310556943750001313, 17.50000000000001421, -66.26410580289947916 ) ) ;
#25275=DIRECTION ( 'NONE',  ( -0.000000000000000000, 1.259100132267607459E-16, -1.000000000000000000 ) ) ;
#25276=DIRECTION ( 'NONE',  ( 0.000000000000000000, 1.000000000000000000, 0.000000000000000000 ) ) ;
#25277=AXIS2_PLACEMENT_3D ( 'NONE', #18418, #15233, #33958 ) ;
#25279=ORIENTED_EDGE ( 'NONE', *, *, #32501, .F. ) ;
#25280=CARTESIAN_POINT ( 'NONE',  ( 3.310556943750001313, 17.50000000000001066, -25.26410580289947916 ) ) ;
#25281=CARTESIAN_POINT ( 'NONE',  ( 4.648177544792955347E-16, 21.00000000000002132, -105.2109808024215027 ) ) ;
#25283=CARTESIAN_POINT ( 'NONE',  ( -3.310556943750000425, 19.41135094264166483, -77.84743913623280775 ) ) ;
#25284=EDGE_LOOP ( 'NONE', ( #41187, #10313, #12246, #21003 ) ) ;
#25286=CARTESIAN_POINT ( 'NONE',  ( -3.500000000000000000, 19.52072594216370760, -53.73806413671077564 ) ) ;
#25292=( BOUNDED_CURVE ( )  B_SPLINE_CURVE ( 2, ( #26526, #359, #6741, #16949, #23335, #35679, #16331, #568, #787 ),
 .UNSPECIFIED., .F., .F. ) 
 B_SPLINE_CURVE_WITH_KNOTS ( ( 3, 2, 2, 2, 3 ),
 ( 0.03958333333333333842, 0.04027777777777778040, 0.04166666666666666435, 0.04305555555555555525, 0.04375000000000000416 ),
 .UNSPECIFIED. ) 
 CURVE ( )  GEOMETRIC_REPRESENTATION_ITEM ( )  RATIONAL_B_SPLINE_CURVE ( ( 0.9330127018922192983, 0.9330127018922196314, 1.000000000000000000, 0.8660254037844387076, 1.000000000000000000, 0.8660254037844387076, 1.000000000000000000, 0.9330127018922189652, 0.9330127018922192983 ) ) 
 REPRESENTATION_ITEM ( '' )  );
#25293=DIRECTION ( 'NONE',  ( -0.000000000000000000, 1.259100132267607459E-16, -1.000000000000000000 ) ) ;
#25294=CARTESIAN_POINT ( 'NONE',  ( -3.310556943750002645, 15.58864905735836714, -45.76827246956613493 ) ) ;
#25295=CARTESIAN_POINT ( 'NONE',  ( 1.655278471874998436, 14.63297358603754716, -108.5182724695661420 ) ) ;
#25297=CARTESIAN_POINT ( 'NONE',  ( -3.310556943750000425, 19.41135094264165772, -32.84743913623280775 ) ) ;
#25298=CARTESIAN_POINT ( 'NONE',  ( -7.022189441860112050E-16, 13.67729811471671830, -59.60160580289947063 ) ) ;
#25299=CARTESIAN_POINT ( 'NONE',  ( -3.500000000000002220, 15.47927405783632970, -104.8776474690881741 ) ) ;
#25301=CARTESIAN_POINT ( 'NONE',  ( 1.655278471875001101, 20.36702641396249192, -92.09743913623280775 ) ) ;
#25302=CARTESIAN_POINT ( 'NONE',  ( -7.424026671074350129E-16, 13.45854811567263809, -98.40473080337741862 ) ) ;
#25303=CARTESIAN_POINT ( 'NONE',  ( -0.9378221735089291577, 21.00000000000002132, -108.8600726046389155 ) ) ;
#25306=CARTESIAN_POINT ( 'NONE',  ( 3.500000000000001332, 17.50000000000001421, -57.46098080242150985 ) ) ;
#25308=CARTESIAN_POINT ( 'NONE',  ( -1.655278471874999990, 20.36702641396248481, -26.93077246956613990 ) ) ;
#25309=CARTESIAN_POINT ( 'NONE',  ( -7.424026671074350129E-16, 13.45854811567263276, -47.40473080337742573 ) ) ;
#25312=CARTESIAN_POINT ( 'NONE',  ( 3.310556943750001313, 17.50000000000002132, -106.3516058028994564 ) ) ;
#25313=CARTESIAN_POINT ( 'NONE',  ( 3.310556943750001313, 19.41135094264166128, -35.26827246956614204 ) ) ;
#25316=CARTESIAN_POINT ( 'NONE',  ( 1.749999999999998224, 14.46891108675447590, -50.32139747004409003 ) ) ;
#25320=EDGE_CURVE ( 'NONE', #24508, #23995, #21506, .T. ) ;
#25322=CARTESIAN_POINT ( 'NONE',  ( 3.310556943749999981, 15.58864905735836892, -89.34743913623279354 ) ) ;
#25323=ORIENTED_EDGE ( 'NONE', *, *, #1436, .T. ) ;
#25328=CARTESIAN_POINT ( 'NONE',  ( 1.750000000000001110, 20.53108891324555785, -109.2943141357548456 ) ) ;
#25329=ORIENTED_EDGE ( 'NONE', *, *, #8067, .F. ) ;
#25332=CARTESIAN_POINT ( 'NONE',  ( 3.310556943749999981, 15.58864905735836892, -94.34743913623280775 ) ) ;
#25334=ORIENTED_EDGE ( 'NONE', *, *, #36562, .F. ) ;
#25335=CARTESIAN_POINT ( 'NONE',  ( 0.000000000000000000, 21.00000000000002487, -149.5231586289125687 ) ) ;
#25336=ORIENTED_EDGE ( 'NONE', *, *, #18911, .T. ) ;
#25337=CARTESIAN_POINT ( 'NONE',  ( 3.500000000000000000, 15.47927405783633503, -139.5443141357548313 ) ) ;
#25339=CARTESIAN_POINT ( 'NONE',  ( 0.000000000000000000, 17.50000000000002487, -149.5231586289125687 ) ) ;
#25342=VERTEX_POINT ( 'NONE', #20197 ) ;
#25344=CARTESIAN_POINT ( 'NONE',  ( -1.836030130193217234E-14, 21.00000000000002487, -134.9047308033774186 ) ) ;
#25345=FACE_OUTER_BOUND ( 'NONE', #18213, .T. ) ;
#25346=EDGE_CURVE ( 'NONE', #21152, #6760, #32068, .T. ) ;
#25347=CARTESIAN_POINT ( 'NONE',  ( 3.310556943749999981, 15.58864905735837425, -131.3474391362327935 ) ) ;
#25349=VERTEX_POINT ( 'NONE', #39759 ) ;
#25350=CARTESIAN_POINT ( 'NONE',  ( -0.9378221735089291577, 21.00000000000001066, -31.86007260463891200 ) ) ;
#25351=CARTESIAN_POINT ( 'NONE',  ( 3.310556943750001313, 17.50000000000002132, -124.3516058028994564 ) ) ;
#25352=CARTESIAN_POINT ( 'NONE',  ( -1.655278471874999990, 20.36702641396248836, -48.01827246956613493 ) ) ;
#25353=ORIENTED_EDGE ( 'NONE', *, *, #18651, .T. ) ;
#25355=CARTESIAN_POINT ( 'NONE',  ( -3.500000000000002220, 15.47927405783633503, -135.5713974700441042 ) ) ;
#25358=CARTESIAN_POINT ( 'NONE',  ( -1.655278471875002211, 14.63297358603754539, -79.68493913623279923 ) ) ;
#25359=CARTESIAN_POINT ( 'NONE',  ( -3.500000000000000888, 19.52072594216371826, -123.0443141357548313 ) ) ;
#25360=CARTESIAN_POINT ( 'NONE',  ( -1.655278471874999990, 20.36702641396249547, -106.9307724695661364 ) ) ;
#25361=( BOUNDED_CURVE ( )  B_SPLINE_CURVE ( 2, ( #24224, #17830, #37194, #1048, #37397, #27819, #40791, #7632, #24640 ),
 .UNSPECIFIED., .F., .T. ) 
 B_SPLINE_CURVE_WITH_KNOTS ( ( 3, 2, 2, 2, 3 ),
 ( 0.4895833333333333148, 0.4902777777777777568, 0.4916666666666666408, 0.4930555555555555802, 0.4937500000000000222 ),
 .UNSPECIFIED. ) 
 CURVE ( )  GEOMETRIC_REPRESENTATION_ITEM ( )  RATIONAL_B_SPLINE_CURVE ( ( 0.9330127018922194093, 0.9330127018922194093, 1.000000000000000000, 0.8660254037844387076, 1.000000000000000000, 0.8660254037844387076, 1.000000000000000000, 0.9330127018922194093, 0.9330127018922194093 ) ) 
 REPRESENTATION_ITEM ( '' )  );
#25362=CARTESIAN_POINT ( 'NONE',  ( 3.500000000000001332, 19.52072594216371115, -81.07139747004410424 ) ) ;
#25366=CARTESIAN_POINT ( 'NONE',  ( -3.500000000000001332, 17.50000000000001776, -74.96098080242151696 ) ) ;
#25367=CARTESIAN_POINT ( 'NONE',  ( 0.9378221735089281585, 14.00000000000001066, -51.66632260368298546 ) ) ;
#25368=CARTESIAN_POINT ( 'NONE',  ( 3.310556943750001313, 17.50000000000001066, -45.26410580289947916 ) ) ;
#25369=CARTESIAN_POINT ( 'NONE',  ( -3.310556943750002645, 15.58864905735837425, -102.7682724695661278 ) ) ;
#25371=CARTESIAN_POINT ( 'NONE',  ( 3.500000000000000000, 15.47927405783632260, -62.23806413671076854 ) ) ;
#25372=DIRECTION ( 'NONE',  ( -0.000000000000000000, 1.259100132267607459E-16, -1.000000000000000000 ) ) ;
#25374=CARTESIAN_POINT ( 'NONE',  ( -1.655278471874999990, 20.36702641396249547, -125.0182724695661278 ) ) ;
#25375=CARTESIAN_POINT ( 'NONE',  ( -0.9378221735089310451, 14.00000000000002132, -91.75563900116003424 ) ) ;
#25379=CARTESIAN_POINT ( 'NONE',  ( 0.9378221735089300459, 21.00000000000001421, -60.25563900116002714 ) ) ;
#25383=CARTESIAN_POINT ( 'NONE',  ( 3.310556943750001313, 19.41135094264166838, -76.26827246956612782 ) ) ;
#25384=ADVANCED_FACE ( 'NONE', ( #10197 ), #23167, .T. ) ;
#25385=CARTESIAN_POINT ( 'NONE',  ( 0.000000000000000000, 21.00000000000002487, -149.5231586289125687 ) ) ;
#25391=CARTESIAN_POINT ( 'NONE',  ( 3.310556943750001313, 19.41135094264166128, -32.18077246956614346 ) ) ;
#25396=CARTESIAN_POINT ( 'NONE',  ( -3.500000000000000000, 19.52072594216370760, -58.04431413575484555 ) ) ;
#25397=ORIENTED_EDGE ( 'NONE', *, *, #35354, .T. ) ;
#25398=ORIENTED_EDGE ( 'NONE', *, *, #11891, .F. ) ;
#25399=CARTESIAN_POINT ( 'NONE',  ( 0.000000000000000000, 17.50000000000002487, -149.5231586289125687 ) ) ;
#25403=CARTESIAN_POINT ( 'NONE',  ( -1.749999999999999778, 20.53108891324554719, -34.12764746908818125 ) ) ;
#25404=CARTESIAN_POINT ( 'NONE',  ( 3.500000000000001332, 19.52072594216371115, -82.37764746908818836 ) ) ;
#25407=CARTESIAN_POINT ( 'NONE',  ( 0.9378221735089281585, 14.00000000000001066, -41.66632260368298546 ) ) ;
#25409=CARTESIAN_POINT ( 'NONE',  ( 1.750000000000001110, 20.53108891324556140, -138.2943141357548313 ) ) ;
#25412=CARTESIAN_POINT ( 'NONE',  ( 2.340729813953370519E-16, 21.32270188528331900, -122.0141058028994792 ) ) ;
#25415=CARTESIAN_POINT ( 'NONE',  ( 1.749999999999998224, 14.46891108675448301, -97.62764746908817415 ) ) ;
#25416=( BOUNDED_CURVE ( )  B_SPLINE_CURVE ( 2, ( #2650, #12219, #25420, #13064, #19029, #2445, #39009, #5637, #16268 ),
 .UNSPECIFIED., .F., .T. ) 
 B_SPLINE_CURVE_WITH_KNOTS ( ( 3, 2, 2, 2, 3 ),
 ( 0.1770833333333333426, 0.1777777777777777846, 0.1791666666666666685, 0.1805555555555555525, 0.1812499999999999944 ),
 .UNSPECIFIED. ) 
 CURVE ( )  GEOMETRIC_REPRESENTATION_ITEM ( )  RATIONAL_B_SPLINE_CURVE ( ( 0.9330127018922194093, 0.9330127018922194093, 1.000000000000000000, 0.8660254037844387076, 1.000000000000000000, 0.8660254037844387076, 1.000000000000000000, 0.9330127018922194093, 0.9330127018922194093 ) ) 
 REPRESENTATION_ITEM ( '' )  );
#25417=CARTESIAN_POINT ( 'NONE',  ( 1.655278471874998436, 14.63297358603754894, -115.5182724695661278 ) ) ;
#25419=CARTESIAN_POINT ( 'NONE',  ( 3.500000000000000000, 15.47927405783632082, -30.23806413671076143 ) ) ;
#25420=CARTESIAN_POINT ( 'NONE',  ( -1.749999999999999778, 20.53108891324555785, -121.8213974700441042 ) ) ;
#25423=CARTESIAN_POINT ( 'NONE',  ( 3.310556943750001313, 19.41135094264167549, -139.2682724695661420 ) ) ;
#25425=CARTESIAN_POINT ( 'NONE',  ( 3.500000000000001332, 19.52072594216370405, -29.37764746908817770 ) ) ;
#25426=CARTESIAN_POINT ( 'NONE',  ( -3.310556943750002201, 15.58864905735836714, -47.76827246956612782 ) ) ;
#25428=CARTESIAN_POINT ( 'NONE',  ( -0.9378221735089310451, 14.00000000000002309, -114.4493890021159501 ) ) ;
#25429=ADVANCED_BREP_SHAPE_REPRESENTATION ( '', ( #38463, #40442 ), #34335 ) ;
#25430=CARTESIAN_POINT ( 'NONE',  ( -3.310556943750002645, 15.58864905735837070, -71.76827246956612782 ) ) ;
#25432=CARTESIAN_POINT ( 'NONE',  ( 3.310556943749999981, 15.58864905735836714, -69.34743913623282197 ) ) ;
#25434=CARTESIAN_POINT ( 'NONE',  ( -1.655278471875002211, 14.63297358603754716, -90.68493913623279923 ) ) ;
#25438=CARTESIAN_POINT ( 'NONE',  ( 4.286263797015737581E-16, 14.00000000000002487, -149.5231586289125687 ) ) ;
#25439=DIRECTION ( 'NONE',  ( -0.000000000000000000, 1.259100132267607459E-16, -1.000000000000000000 ) ) ;
#25440=CARTESIAN_POINT ( 'NONE',  ( -3.310556943750000425, 19.41135094264166483, -49.84743913623280065 ) ) ;
#25442=CARTESIAN_POINT ( 'NONE',  ( 3.310556943749999981, 15.58864905735837070, -105.3474391362328078 ) ) ;
#25443=DIRECTION ( 'NONE',  ( -0.000000000000000000, 1.259100132267607459E-16, -1.000000000000000000 ) ) ;
#25445=VECTOR ( 'NONE', #29529, 1000.000000000000000 ) ;
#25446=ORIENTED_EDGE ( 'NONE', *, *, #37588, .F. ) ;
#25448=ORIENTED_EDGE ( 'NONE', *, *, #23566, .F. ) ;
#25450=CARTESIAN_POINT ( 'NONE',  ( 3.310556943749999981, 15.58864905735836537, -62.34743913623280775 ) ) ;
#25453=CARTESIAN_POINT ( 'NONE',  ( 3.500000000000001332, 17.50000000000001066, -30.46098080242151696 ) ) ;
#25457=VECTOR ( 'NONE', #15485, 1000.000000000000000 ) ;
#25460=CARTESIAN_POINT ( 'NONE',  ( -3.310556943750002201, 15.58864905735837780, -123.6807724695661506 ) ) ;
#25461=CARTESIAN_POINT ( 'NONE',  ( -3.500000000000002220, 15.47927405783633503, -128.5713974700441042 ) ) ;
#25462=CARTESIAN_POINT ( 'NONE',  ( 1.655278471875001101, 20.36702641396248481, -37.18493913623280633 ) ) ;
#25464=CARTESIAN_POINT ( 'NONE',  ( 1.655278471874998436, 14.63297358603753828, -26.51827246956613138 ) ) ;
#25465=CARTESIAN_POINT ( 'NONE',  ( 2.340729813953370519E-16, 21.32270188528331190, -90.10160580289947063 ) ) ;
#25466=CARTESIAN_POINT ( 'NONE',  ( 2.340729813953370519E-16, 21.32270188528332255, -139.0141058028994792 ) ) ;
#25469=CARTESIAN_POINT ( 'NONE',  ( -3.310556943750002645, 15.58864905735837780, -133.7682724695661420 ) ) ;
#25473=CARTESIAN_POINT ( 'NONE',  ( -1.394453263437886604E-15, 14.00000000000001421, -75.71098080242151696 ) ) ;
#25475=CARTESIAN_POINT ( 'NONE',  ( 3.500000000000000000, 15.47927405783632437, -79.23806413671077564 ) ) ;
#25477=CARTESIAN_POINT ( 'NONE',  ( -7.022189441860112050E-16, 13.67729811471672186, -62.60160580289945642 ) ) ;
#25480=CARTESIAN_POINT ( 'NONE',  ( -1.394453263437886604E-15, 14.00000000000001066, -47.71098080242150274 ) ) ;
#25481=CARTESIAN_POINT ( 'NONE',  ( -1.655278471874999990, 20.36702641396249192, -88.01827246956612782 ) ) ;
#25482=CARTESIAN_POINT ( 'NONE',  ( -3.500000000000000000, 19.52072594216371826, -116.7380641367107472 ) ) ;
#25483=CARTESIAN_POINT ( 'NONE',  ( -3.310556943750002201, 15.58864905735837780, -112.6807724695661364 ) ) ;
#25487=ORIENTED_EDGE ( 'NONE', *, *, #8280, .F. ) ;
#25488=CARTESIAN_POINT ( 'NONE',  ( 1.750000000000001110, 20.53108891324555785, -108.9880641367107614 ) ) ;
#25491=CARTESIAN_POINT ( 'NONE',  ( -1.394453263437886604E-15, 14.00000000000001421, -67.71098080242148853 ) ) ;
#25492=CARTESIAN_POINT ( 'NONE',  ( -0.9378221735089310451, 14.00000000000001066, -26.75563900116003069 ) ) ;
#25495=CARTESIAN_POINT ( 'NONE',  ( 2.340729813953370519E-16, 21.32270188528331190, -65.01410580289946495 ) ) ;
#25496=CARTESIAN_POINT ( 'NONE',  ( 3.500000000000001332, 19.52072594216370760, -59.37764746908817415 ) ) ;
#25501=CARTESIAN_POINT ( 'NONE',  ( -0.9378221735089291577, 21.00000000000002132, -105.1663226036829997 ) ) ;
#25502=CARTESIAN_POINT ( 'NONE',  ( -1.655278471874999990, 20.36702641396249192, -79.93077246956615056 ) ) ;
#25503=VERTEX_POINT ( 'NONE', #4660 ) ;
#25505=CARTESIAN_POINT ( 'NONE',  ( -1.749999999999999778, 20.53108891324555074, -48.82139747004410424 ) ) ;
#25507=CARTESIAN_POINT ( 'NONE',  ( -7.022189441860112050E-16, 13.67729811471673074, -142.5141058028994792 ) ) ;
#25509=AXIS2_PLACEMENT_3D ( 'NONE', #18799, #2629, #28154 ) ;
#25511=CARTESIAN_POINT ( 'NONE',  ( 3.310556943750001313, 19.41135094264165772, -44.26827246956613493 ) ) ;
#25512=CARTESIAN_POINT ( 'NONE',  ( 1.655278471875001101, 20.36702641396249547, -102.1849391362327992 ) ) ;
#25513=ORIENTED_EDGE ( 'NONE', *, *, #25915, .T. ) ;
#25514=CARTESIAN_POINT ( 'NONE',  ( 3.310556943749999981, 15.58864905735836182, -29.34743913623280775 ) ) ;
#25515=CARTESIAN_POINT ( 'NONE',  ( 1.655278471874998436, 14.63297358603754184, -60.51827246956613493 ) ) ;
#25516=CARTESIAN_POINT ( 'NONE',  ( 3.500000000000001332, 17.50000000000002132, -106.4609808024215027 ) ) ;
#25518=CARTESIAN_POINT ( 'NONE',  ( -1.750000000000002220, 14.46891108675448478, -96.48806413671076143 ) ) ;
#25519=ADVANCED_FACE ( 'NONE', ( #14662 ), #11253, .T. ) ;
#25520=DIRECTION ( 'NONE',  ( -0.000000000000000000, 1.259100132267607459E-16, -1.000000000000000000 ) ) ;
#25524=CARTESIAN_POINT ( 'NONE',  ( -3.500000000000000888, 19.52072594216370760, -59.04431413575483134 ) ) ;
#25526=CARTESIAN_POINT ( 'NONE',  ( 1.655278471874998436, 14.63297358603753828, -27.43077246956614346 ) ) ;
#25527=CARTESIAN_POINT ( 'NONE',  ( 3.500000000000000000, 15.47927405783632082, -49.23806413671076143 ) ) ;
#25529=CARTESIAN_POINT ( 'NONE',  ( 1.655278471875001101, 20.36702641396248481, -33.18493913623279923 ) ) ;
#25531=DIRECTION ( 'NONE',  ( -0.000000000000000000, 1.259100132267607459E-16, -1.000000000000000000 ) ) ;
#25532=CARTESIAN_POINT ( 'NONE',  ( -0.9378221735089299349, 14.00000000000002487, -141.7556390011600342 ) ) ;
#25536=CARTESIAN_POINT ( 'NONE',  ( 1.655278471875001101, 20.36702641396249192, -80.09743913623280775 ) ) ;
#25538=CARTESIAN_POINT ( 'NONE',  ( -3.500000000000000000, 19.52072594216370405, -25.73806413671075788 ) ) ;
#25539=ORIENTED_EDGE ( 'NONE', *, *, #23347, .F. ) ;
#25540=CARTESIAN_POINT ( 'NONE',  ( -3.500000000000002220, 15.47927405783632082, -35.57139747004409003 ) ) ;
#25541=CARTESIAN_POINT ( 'NONE',  ( 3.500000000000001332, 19.52072594216371826, -108.0713974700441042 ) ) ;
#25542=( BOUNDED_CURVE ( )  B_SPLINE_CURVE ( 2, ( #36542, #29944, #4214, #10176, #595, #17197, #13154, #13571, #30158 ),
 .UNSPECIFIED., .F., .F. ) 
 B_SPLINE_CURVE_WITH_KNOTS ( ( 3, 2, 2, 2, 3 ),
 ( 0.2687499999999999889, 0.2694444444444444309, 0.2708333333333333148, 0.2722222222222221988, 0.2729166666666666963 ),
 .UNSPECIFIED. ) 
 CURVE ( )  GEOMETRIC_REPRESENTATION_ITEM ( )  RATIONAL_B_SPLINE_CURVE ( ( 0.9330127018922194093, 0.9330127018922194093, 1.000000000000000000, 0.8660254037844387076, 1.000000000000000000, 0.8660254037844387076, 1.000000000000000000, 0.9330127018922167448, 0.9330127018922194093 ) ) 
 REPRESENTATION_ITEM ( '' )  );
#25546=CARTESIAN_POINT ( 'NONE',  ( -3.310556943750000425, 19.41135094264166483, -97.84743913623280775 ) ) ;
#25548=ORIENTED_EDGE ( 'NONE', *, *, #42041, .F. ) ;
#25549=CARTESIAN_POINT ( 'NONE',  ( -1.394453263437886604E-15, 14.00000000000002132, -121.4047308033774328 ) ) ;
#25553=CARTESIAN_POINT ( 'NONE',  ( 0.000000000000000000, 17.50000000000002487, -149.5231586289125687 ) ) ;
#25556=VERTEX_POINT ( 'NONE', #30605 ) ;
#25559=CARTESIAN_POINT ( 'NONE',  ( -3.310556943750002645, 15.58864905735837780, -133.6807724695661648 ) ) ;
#25560=CARTESIAN_POINT ( 'NONE',  ( -1.394453263437886604E-15, 14.00000000000002132, -132.4047308033774186 ) ) ;
#25563=CARTESIAN_POINT ( 'NONE',  ( -3.310556943750000425, 19.41135094264166838, -124.9349391362327850 ) ) ;
#25564=CARTESIAN_POINT ( 'NONE',  ( -3.310556943750000425, 19.41135094264166128, -50.93493913623280633 ) ) ;
#25566=CARTESIAN_POINT ( 'NONE',  ( -1.750000000000002220, 14.46891108675448834, -131.4880641367107614 ) ) ;
#25568=CARTESIAN_POINT ( 'NONE',  ( -1.655278471875002211, 14.63297358603754539, -76.68493913623279923 ) ) ;
#25569=CARTESIAN_POINT ( 'NONE',  ( -1.750000000000002220, 14.46891108675448834, -123.7943141357548456 ) ) ;
#25570=CARTESIAN_POINT ( 'NONE',  ( -3.310556943750001313, 17.50000000000002132, -105.7641058028994649 ) ) ;
#25571=CARTESIAN_POINT ( 'NONE',  ( 4.648177544792955347E-16, 21.00000000000002132, -107.9047308033774328 ) ) ;
#25574=CARTESIAN_POINT ( 'NONE',  ( 1.749999999999998224, 14.46891108675447946, -75.62764746908817415 ) ) ;
#25575=CARTESIAN_POINT ( 'NONE',  ( -1.394453263437886604E-15, 14.00000000000002132, -126.4047308033774186 ) ) ;
#25576=CARTESIAN_POINT ( 'NONE',  ( -3.310556943750001313, 17.50000000000001066, -44.76410580289947916 ) ) ;
#25577=CARTESIAN_POINT ( 'NONE',  ( 1.655278471874998436, 14.63297358603754716, -99.51827246956612782 ) ) ;
#25579=CARTESIAN_POINT ( 'NONE',  ( -3.500000000000002220, 15.47927405783632437, -66.57139747004409003 ) ) ;
#25582=CARTESIAN_POINT ( 'NONE',  ( 3.310556943750001313, 17.50000000000002132, -115.3516058028994706 ) ) ;
#25587=CARTESIAN_POINT ( 'NONE',  ( 3.500000000000001332, 17.50000000000002132, -107.4609808024215027 ) ) ;
#25592=CARTESIAN_POINT ( 'NONE',  ( 2.340729813953370519E-16, 21.32270188528331190, -75.10160580289947063 ) ) ;
#25593=EDGE_CURVE ( 'NONE', #21522, #31803, #37820, .T. ) ;
#25598=CARTESIAN_POINT ( 'NONE',  ( 1.655278471874998436, 14.63297358603753828, -36.43077246956613635 ) ) ;
#25601=ORIENTED_EDGE ( 'NONE', *, *, #3927, .F. ) ;
#25603=CARTESIAN_POINT ( 'NONE',  ( -3.500000000000000000, 19.52072594216371826, -138.7380641367107614 ) ) ;
#25608=CARTESIAN_POINT ( 'NONE',  ( 0.000000000000000000, 17.50000000000002487, -149.5231586289125687 ) ) ;
#25609=CARTESIAN_POINT ( 'NONE',  ( 3.500000000000000000, 15.47927405783632970, -121.2380641367107472 ) ) ;
#25611=CARTESIAN_POINT ( 'NONE',  ( -1.749999999999999778, 20.53108891324554719, -31.12764746908817770 ) ) ;
#25613=( BOUNDED_CURVE ( )  B_SPLINE_CURVE ( 2, ( #26943, #14803, #23750, #40538, #7798, #7580, #30120, #37149, #996 ),
 .UNSPECIFIED., .F., .T. ) 
 B_SPLINE_CURVE_WITH_KNOTS ( ( 3, 2, 2, 2, 3 ),
 ( 0.04791666666666666990, 0.04861111111111111188, 0.05000000000000000278, 0.05138888888888888673, 0.05208333333333333565 ),
 .UNSPECIFIED. ) 
 CURVE ( )  GEOMETRIC_REPRESENTATION_ITEM ( )  RATIONAL_B_SPLINE_CURVE ( ( 0.9330127018922192983, 0.9330127018922196314, 1.000000000000000000, 0.8660254037844387076, 1.000000000000000000, 0.8660254037844387076, 1.000000000000000000, 0.9330127018922189652, 0.9330127018922192983 ) ) 
 REPRESENTATION_ITEM ( '' )  );
#25614=DIRECTION ( 'NONE',  ( -0.000000000000000000, 1.259100132267607459E-16, -1.000000000000000000 ) ) ;
#25616=EDGE_CURVE ( 'NONE', #15608, #24508, #14682, .T. ) ;
#25617=CARTESIAN_POINT ( 'NONE',  ( 4.648177544792955347E-16, 21.00000000000002132, -118.2109808024215170 ) ) ;
#25619=CARTESIAN_POINT ( 'NONE',  ( -1.750000000000002220, 14.46891108675449011, -138.7943141357548313 ) ) ;
#25621=CARTESIAN_POINT ( 'NONE',  ( 1.655278471875001101, 20.36702641396249547, -124.0974391362328078 ) ) ;
#25625=CARTESIAN_POINT ( 'NONE',  ( 1.749999999999998224, 14.46891108675448123, -93.62764746908815994 ) ) ;
#25627=CARTESIAN_POINT ( 'NONE',  ( -1.655278471875002211, 14.63297358603754361, -57.59743913623280065 ) ) ;
#25628=CARTESIAN_POINT ( 'NONE',  ( -3.310556943750000425, 19.41135094264166838, -117.9349391362327992 ) ) ;
#25629=CARTESIAN_POINT ( 'NONE',  ( 0.000000000000000000, 17.50000000000002487, -149.5231586289125687 ) ) ;
#25630=CARTESIAN_POINT ( 'NONE',  ( 3.500000000000001332, 17.50000000000001066, -32.15473080337742573 ) ) ;
#25631=CARTESIAN_POINT ( 'NONE',  ( 1.750000000000001110, 20.53108891324555429, -91.98806413671076143 ) ) ;
#25633=CARTESIAN_POINT ( 'NONE',  ( -1.655278471875002211, 14.63297358603755249, -133.6849391362327992 ) ) ;
#25636=CARTESIAN_POINT ( 'NONE',  ( -7.022189441860112050E-16, 13.67729811471671830, -49.60160580289946353 ) ) ;
#25638=CARTESIAN_POINT ( 'NONE',  ( 0.000000000000000000, 17.49999999999998934, 153.5815388724490163 ) ) ;
#25639=CARTESIAN_POINT ( 'NONE',  ( 3.310556943750001313, 19.41135094264166128, -71.26827246956612782 ) ) ;
#25641=CARTESIAN_POINT ( 'NONE',  ( 3.310556943750001313, 19.41135094264166128, -63.18077246956614346 ) ) ;
#25643=CARTESIAN_POINT ( 'NONE',  ( -3.310556943750000425, 19.41135094264166838, -88.93493913623281344 ) ) ;
#25646=CARTESIAN_POINT ( 'NONE',  ( 4.648177544792955347E-16, 21.00000000000002132, -108.2109808024215170 ) ) ;
#25648=CARTESIAN_POINT ( 'NONE',  ( -1.749999999999999778, 20.53108891324554719, -42.12764746908817415 ) ) ;
#25649=CARTESIAN_POINT ( 'NONE',  ( -3.310556943750001313, 17.50000000000001421, -50.76410580289947205 ) ) ;
#25651=CARTESIAN_POINT ( 'NONE',  ( -1.655278471875002211, 14.63297358603754894, -103.5974391362328220 ) ) ;
#25652=ORIENTED_EDGE ( 'NONE', *, *, #16758, .T. ) ;
#25655=ORIENTED_EDGE ( 'NONE', *, *, #22150, .T. ) ;
#25657=CARTESIAN_POINT ( 'NONE',  ( 3.310556943749999981, 15.58864905735836537, -58.34743913623280775 ) ) ;
#25658=ORIENTED_EDGE ( 'NONE', *, *, #10341, .T. ) ;
#25659=ORIENTED_EDGE ( 'NONE', *, *, #35404, .F. ) ;
#25660=CARTESIAN_POINT ( 'NONE',  ( 0.000000000000000000, 21.00000000000002487, -149.5231586289125687 ) ) ;
#25664=ORIENTED_EDGE ( 'NONE', *, *, #32184, .T. ) ;
#25666=CARTESIAN_POINT ( 'NONE',  ( -0.9378221735089268263, 14.00000000000002309, -138.7556390011600342 ) ) ;
#25667=CARTESIAN_POINT ( 'NONE',  ( 3.310556943750001313, 17.50000000000002132, -123.2641058028994649 ) ) ;
#25669=( BOUNDED_CURVE ( )  B_SPLINE_CURVE ( 2, ( #11458, #27630, #40602, #24449, #1888, #37418, #31033, #21251, #27837 ),
 .UNSPECIFIED., .F., .T. ) 
 B_SPLINE_CURVE_WITH_KNOTS ( ( 3, 2, 2, 2, 3 ),
 ( 0.9812499999999999556, 0.9819444444444443976, 0.9833333333333332815, 0.9847222222222222765, 0.9854166666666667185 ),
 .UNSPECIFIED. ) 
 CURVE ( )  GEOMETRIC_REPRESENTATION_ITEM ( )  RATIONAL_B_SPLINE_CURVE ( ( 0.9330127018922194093, 0.9330127018922194093, 1.000000000000000000, 0.8660254037844387076, 1.000000000000000000, 0.8660254037844387076, 1.000000000000000000, 0.9330127018922194093, 0.9330127018922194093 ) ) 
 REPRESENTATION_ITEM ( '' )  );
#25670=EDGE_CURVE ( 'NONE', #1932, #25189, #1388, .T. ) ;
#25672=CARTESIAN_POINT ( 'NONE',  ( -7.022189441860112050E-16, 13.67729811471671475, -33.60160580289946353 ) ) ;
#25673=CARTESIAN_POINT ( 'NONE',  ( 3.310556943750001313, 17.50000000000001066, -26.35160580289947063 ) ) ;
#25674=CARTESIAN_POINT ( 'NONE',  ( 3.310556943750001313, 19.41135094264166483, -90.26827246956612782 ) ) ;
#25675=CARTESIAN_POINT ( 'NONE',  ( 3.310556943750001313, 19.41135094264167549, -137.1807724695661364 ) ) ;
#25678=CARTESIAN_POINT ( 'NONE',  ( 0.9378221735089281585, 14.00000000000002132, -114.3600726046389013 ) ) ;
#25679=CARTESIAN_POINT ( 'NONE',  ( 3.310556943750001313, 17.50000000000002487, -135.3516058028994564 ) ) ;
#25680=CARTESIAN_POINT ( 'NONE',  ( 1.750000000000001110, 20.53108891324555074, -69.98806413671077564 ) ) ;
#25682=CARTESIAN_POINT ( 'NONE',  ( -3.500000000000001332, 17.50000000000001776, -92.96098080242151696 ) ) ;
#25683=CARTESIAN_POINT ( 'NONE',  ( 1.750000000000001110, 20.53108891324555429, -78.98806413671076143 ) ) ;
#25684=CARTESIAN_POINT ( 'NONE',  ( 1.655278471874998436, 14.63297358603754184, -66.51827246956612782 ) ) ;
#25687=CARTESIAN_POINT ( 'NONE',  ( -1.750000000000002220, 14.46891108675447946, -58.48806413671076143 ) ) ;
#25688=CARTESIAN_POINT ( 'NONE',  ( -3.310556943750001313, 17.50000000000001776, -87.85160580289947063 ) ) ;
#25690=CARTESIAN_POINT ( 'NONE',  ( -3.310556943750000425, 19.41135094264166838, -115.8474391362327935 ) ) ;
#25693=ORIENTED_EDGE ( 'NONE', *, *, #9130, .F. ) ;
#25694=CARTESIAN_POINT ( 'NONE',  ( 1.749999999999998224, 14.46891108675448478, -110.3213974700441042 ) ) ;
#25697=CARTESIAN_POINT ( 'NONE',  ( -1.749999999999999778, 20.53108891324555074, -68.12764746908817415 ) ) ;
#25701=CARTESIAN_POINT ( 'NONE',  ( 1.655278471875001101, 20.36702641396248836, -68.09743913623280775 ) ) ;
#25703=CARTESIAN_POINT ( 'NONE',  ( 1.655278471875001101, 20.36702641396249547, -122.0974391362328078 ) ) ;
#25707=ORIENTED_EDGE ( 'NONE', *, *, #13613, .T. ) ;
#25709=CARTESIAN_POINT ( 'NONE',  ( -3.500000000000002220, 15.47927405783633326, -103.8776474690881599 ) ) ;
#25710=CARTESIAN_POINT ( 'NONE',  ( 3.310556943749999981, 15.58864905735836714, -76.34743913623280775 ) ) ;
#25715=CARTESIAN_POINT ( 'NONE',  ( -7.022189441860112050E-16, 13.67729811471673074, -140.5141058028994792 ) ) ;
#25718=CARTESIAN_POINT ( 'NONE',  ( 1.655278471875001101, 20.36702641396248481, -43.18493913623279212 ) ) ;
#25719=CARTESIAN_POINT ( 'NONE',  ( 3.310556943749999981, 15.58864905735837070, -102.4349391362328134 ) ) ;
#25722=CARTESIAN_POINT ( 'NONE',  ( 1.655278471875001101, 20.36702641396248481, -28.09743913623280420 ) ) ;
#25724=CARTESIAN_POINT ( 'NONE',  ( 1.750000000000001110, 20.53108891324555785, -107.2943141357548456 ) ) ;
#25727=CARTESIAN_POINT ( 'NONE',  ( 2.474675557024783212E-16, 21.54145188432739744, -94.90473080337743284 ) ) ;
#25728=CARTESIAN_POINT ( 'NONE',  ( -1.749999999999999778, 20.53108891324555785, -108.8213974700441042 ) ) ;
#25731=CARTESIAN_POINT ( 'NONE',  ( -1.749999999999999778, 20.53108891324555074, -57.12764746908817415 ) ) ;
#25733=CARTESIAN_POINT ( 'NONE',  ( -1.655278471875002211, 14.63297358603754006, -27.59743913623280420 ) ) ;
#25734=CARTESIAN_POINT ( 'NONE',  ( 3.500000000000001776, 19.52072594216370760, -47.07139747004410424 ) ) ;
#25735=CARTESIAN_POINT ( 'NONE',  ( -0.9378221735089291577, 21.00000000000001066, -46.16632260368297835 ) ) ;
#25737=CARTESIAN_POINT ( 'NONE',  ( 1.655278471874998436, 14.63297358603753828, -31.51827246956613493 ) ) ;
#25740=CARTESIAN_POINT ( 'NONE',  ( 4.648177544792955347E-16, 21.00000000000002132, -121.2109808024215170 ) ) ;
#25744=CARTESIAN_POINT ( 'NONE',  ( -1.655278471875002211, 14.63297358603754716, -81.59743913623280775 ) ) ;
#25746=VERTEX_POINT ( 'NONE', #29077 ) ;
#25748=CARTESIAN_POINT ( 'NONE',  ( 1.750000000000001110, 20.53108891324555785, -107.9880641367107614 ) ) ;
#25752=CARTESIAN_POINT ( 'NONE',  ( -1.655278471874999990, 20.36702641396249192, -92.93077246956613635 ) ) ;
#25754=FACE_OUTER_BOUND ( 'NONE', #25057, .T. ) ;
#25755=ORIENTED_EDGE ( 'NONE', *, *, #31403, .T. ) ;
#25758=CARTESIAN_POINT ( 'NONE',  ( -1.394453263437886604E-15, 14.00000000000001421, -66.71098080242148853 ) ) ;
#25762=CARTESIAN_POINT ( 'NONE',  ( -3.500000000000001332, 17.50000000000001776, -88.65473080337743284 ) ) ;
#25763=DIRECTION ( 'NONE',  ( -0.000000000000000000, 1.259100132267607459E-16, -1.000000000000000000 ) ) ;
#25764=AXIS2_PLACEMENT_3D ( 'NONE', #36696, #4153, #11177 ) ;
#25765=CARTESIAN_POINT ( 'NONE',  ( -3.310556943750001313, 17.50000000000002487, -132.7641058028994507 ) ) ;
#25767=CARTESIAN_POINT ( 'NONE',  ( -7.022189441860112050E-16, 13.67729811471672718, -117.6016058028994564 ) ) ;
#25768=CARTESIAN_POINT ( 'NONE',  ( -3.310556943750000425, 19.41135094264166128, -51.93493913623279923 ) ) ;
#25770=CARTESIAN_POINT ( 'NONE',  ( -3.500000000000001332, 17.50000000000002487, -131.6547308033774186 ) ) ;
#25772=CARTESIAN_POINT ( 'NONE',  ( 1.655278471875001101, 20.36702641396248836, -72.18493913623279923 ) ) ;
#25773=CARTESIAN_POINT ( 'NONE',  ( -3.500000000000000888, 19.52072594216371826, -125.0443141357548456 ) ) ;
#25774=CARTESIAN_POINT ( 'NONE',  ( -1.655278471875002211, 14.63297358603754894, -106.5974391362328078 ) ) ;
#25775=DIRECTION ( 'NONE',  ( -0.000000000000000000, 1.259100132267607459E-16, -1.000000000000000000 ) ) ;
#25778=CARTESIAN_POINT ( 'NONE',  ( 2.474675557024783212E-16, 21.54145188432739388, -74.21098080242151696 ) ) ;
#25781=CARTESIAN_POINT ( 'NONE',  ( -3.310556943750000425, 19.41135094264165772, -44.84743913623280775 ) ) ;
#25782=CARTESIAN_POINT ( 'NONE',  ( 1.655278471875001101, 20.36702641396249547, -102.1849391362327992 ) ) ;
#25783=( BOUNDED_CURVE ( )  B_SPLINE_CURVE ( 2, ( #28938, #9389, #31925, #38522, #22564, #2582, #12998, #22352, #29140 ),
 .UNSPECIFIED., .F., .T. ) 
 B_SPLINE_CURVE_WITH_KNOTS ( ( 3, 2, 2, 2, 3 ),
 ( 0.01874999999999999931, 0.01944444444444444475, 0.02083333333333333218, 0.02222222222222222307, 0.02291666666666666852 ),
 .UNSPECIFIED. ) 
 CURVE ( )  GEOMETRIC_REPRESENTATION_ITEM ( )  RATIONAL_B_SPLINE_CURVE ( ( 0.9330127018922194093, 0.9330127018922194093, 1.000000000000000000, 0.8660254037844387076, 1.000000000000000000, 0.8660254037844387076, 1.000000000000000000, 0.9330127018922191873, 0.9330127018922194093 ) ) 
 REPRESENTATION_ITEM ( '' )  );
#25784=CARTESIAN_POINT ( 'NONE',  ( -0.9378221735089310451, 14.00000000000002132, -82.75563900116002003 ) ) ;
#25785=CARTESIAN_POINT ( 'NONE',  ( 3.500000000000000000, 15.47927405783632260, -67.23806413671077564 ) ) ;
#25787=VERTEX_POINT ( 'NONE', #22081 ) ;
#25788=CARTESIAN_POINT ( 'NONE',  ( -7.022189441860112050E-16, 13.67729811471672896, -116.6016058028994564 ) ) ;
#25794=CARTESIAN_POINT ( 'NONE',  ( 3.310556943749999981, 15.58864905735837070, -97.34743913623280775 ) ) ;
#25795=DIRECTION ( 'NONE',  ( -0.000000000000000000, 1.259100132267607459E-16, -1.000000000000000000 ) ) ;
#25797=VERTEX_POINT ( 'NONE', #35050 ) ;
#25798=FACE_OUTER_BOUND ( 'NONE', #25284, .T. ) ;
#25800=CARTESIAN_POINT ( 'NONE',  ( -3.500000000000002220, 15.47927405783633503, -126.8776474690881741 ) ) ;
#25801=CARTESIAN_POINT ( 'NONE',  ( 3.500000000000000000, 15.47927405783632615, -80.23806413671076143 ) ) ;
#25805=CARTESIAN_POINT ( 'NONE',  ( -1.655278471874999990, 20.36702641396248481, -33.93077246956615056 ) ) ;
#25806=EDGE_CURVE ( 'NONE', #18214, #11305, #12720, .T. ) ;
#25807=CARTESIAN_POINT ( 'NONE',  ( 1.749999999999998224, 14.46891108675448301, -107.3213974700441042 ) ) ;
#25812=EDGE_LOOP ( 'NONE', ( #26007, #6003, #4196, #23829 ) ) ;
#25813=VECTOR ( 'NONE', #21862, 1000.000000000000000 ) ;
#25815=DIRECTION ( 'NONE',  ( -0.000000000000000000, 1.259100132267607459E-16, -1.000000000000000000 ) ) ;
#25818=CARTESIAN_POINT ( 'NONE',  ( 1.749999999999998224, 14.46891108675448478, -116.3213974700440900 ) ) ;
#25819=CARTESIAN_POINT ( 'NONE',  ( -3.500000000000000000, 19.52072594216370405, -34.04431413575484555 ) ) ;
#25820=CARTESIAN_POINT ( 'NONE',  ( -3.310556943750000425, 19.41135094264167549, -133.9349391362327992 ) ) ;
#25821=CARTESIAN_POINT ( 'NONE',  ( -3.500000000000002220, 15.47927405783632082, -30.87764746908818481 ) ) ;
#25825=CARTESIAN_POINT ( 'NONE',  ( 3.500000000000000000, 15.47927405783632082, -41.54431413575483845 ) ) ;
#25827=CARTESIAN_POINT ( 'NONE',  ( -3.500000000000002220, 15.47927405783633503, -138.8776474690881741 ) ) ;
#25828=LINE ( 'NONE', #37956, #34707 ) ;
#25829=CARTESIAN_POINT ( 'NONE',  ( 3.310556943750001313, 19.41135094264166838, -125.1807724695661364 ) ) ;
#25832=CARTESIAN_POINT ( 'NONE',  ( 2.474675557024783212E-16, 21.54145188432739744, -90.21098080242150274 ) ) ;
#25833=CARTESIAN_POINT ( 'NONE',  ( -1.394453263437886604E-15, 14.00000000000001066, -45.40473080337742573 ) ) ;
#25834=CARTESIAN_POINT ( 'NONE',  ( -7.022189441860112050E-16, 13.67729811471671830, -56.51410580289947205 ) ) ;
#25835=CARTESIAN_POINT ( 'NONE',  ( 1.655278471875001101, 20.36702641396249547, -118.1849391362327850 ) ) ;
#25837=CARTESIAN_POINT ( 'NONE',  ( -1.749999999999999778, 20.53108891324554719, -32.82139747004410424 ) ) ;
#25838=CARTESIAN_POINT ( 'NONE',  ( 7.367361408496833051E-14, 14.00000000000001776, -108.7109808024215027 ) ) ;
#25840=CARTESIAN_POINT ( 'NONE',  ( -1.655278471874999990, 20.36702641396249902, -136.0182724695661420 ) ) ;
#25843=CARTESIAN_POINT ( 'NONE',  ( -3.310556943750000425, 19.41135094264166128, -45.93493913623279923 ) ) ;
#25844=FACE_OUTER_BOUND ( 'NONE', #14361, .T. ) ;
#25845=CARTESIAN_POINT ( 'NONE',  ( 1.655278471874998436, 14.63297358603754361, -69.51827246956612782 ) ) ;
#25848=CARTESIAN_POINT ( 'NONE',  ( -7.022189441860112050E-16, 13.67729811471671830, -66.51410580289947916 ) ) ;
#25850=CARTESIAN_POINT ( 'NONE',  ( 2.340729813953370519E-16, 21.32270188528331190, -87.10160580289947063 ) ) ;
#25852=CARTESIAN_POINT ( 'NONE',  ( 4.286263797015737581E-16, 14.00000000000002487, -149.5231586289125687 ) ) ;
#25853=FACE_OUTER_BOUND ( 'NONE', #24025, .T. ) ;
#25855=CARTESIAN_POINT ( 'NONE',  ( 2.340729813953370519E-16, 21.32270188528331190, -48.01410580289946495 ) ) ;
#25856=EDGE_CURVE ( 'NONE', #24209, #6382, #2997, .T. ) ;
#25858=CARTESIAN_POINT ( 'NONE',  ( 1.655278471875001101, 20.36702641396249547, -104.0974391362328220 ) ) ;
#25859=ORIENTED_EDGE ( 'NONE', *, *, #11191, .T. ) ;
#25861=ORIENTED_EDGE ( 'NONE', *, *, #40810, .F. ) ;
#25863=CARTESIAN_POINT ( 'NONE',  ( -3.310556943750001313, 17.50000000000001421, -59.76410580289947916 ) ) ;
#25864=( BOUNDED_CURVE ( )  B_SPLINE_CURVE ( 2, ( #2934, #15923, #3148, #153, #13135, #26747, #19722, #37307, #19935 ),
 .UNSPECIFIED., .F., .T. ) 
 B_SPLINE_CURVE_WITH_KNOTS ( ( 3, 2, 2, 2, 3 ),
 ( 0.8145833333333333259, 0.8152777777777777679, 0.8166666666666666519, 0.8180555555555555358, 0.8187499999999999778 ),
 .UNSPECIFIED. ) 
 CURVE ( )  GEOMETRIC_REPRESENTATION_ITEM ( )  RATIONAL_B_SPLINE_CURVE ( ( 0.9330127018922194093, 0.9330127018922194093, 1.000000000000000000, 0.8660254037844387076, 1.000000000000000000, 0.8660254037844387076, 1.000000000000000000, 0.9330127018922194093, 0.9330127018922194093 ) ) 
 REPRESENTATION_ITEM ( '' )  );
#25865=EDGE_LOOP ( 'NONE', ( #6508, #28309, #42018, #33969 ) ) ;
#25866=ORIENTED_EDGE ( 'NONE', *, *, #7390, .T. ) ;
#25868=CARTESIAN_POINT ( 'NONE',  ( 4.648177544792955347E-16, 21.00000000000001421, -48.21098080242150274 ) ) ;
#25870=FACE_OUTER_BOUND ( 'NONE', #18221, .T. ) ;
#25872=CARTESIAN_POINT ( 'NONE',  ( -1.394453263437886604E-15, 14.00000000000001066, -38.71098080242150985 ) ) ;
#25873=CARTESIAN_POINT ( 'NONE',  ( 3.310556943750001313, 17.50000000000002132, -126.2641058028994792 ) ) ;
#25876=EDGE_CURVE ( 'NONE', #12197, #20737, #19306, .T. ) ;
#25878=CARTESIAN_POINT ( 'NONE',  ( 3.310556943750001313, 19.41135094264165772, -34.26827246956613493 ) ) ;
#25879=CARTESIAN_POINT ( 'NONE',  ( 2.340729813953370519E-16, 21.32270188528330479, -28.10160580289947418 ) ) ;
#25880=CARTESIAN_POINT ( 'NONE',  ( 2.340729813953370519E-16, 21.32270188528331190, -86.10160580289948484 ) ) ;
#25881=CARTESIAN_POINT ( 'NONE',  ( -7.022189441860112050E-16, 13.67729811471672896, -141.5141058028994792 ) ) ;
#25884=CARTESIAN_POINT ( 'NONE',  ( 3.500000000000001332, 17.50000000000002132, -114.1547308033774328 ) ) ;
#25885=CARTESIAN_POINT ( 'NONE',  ( -3.310556943750000425, 19.41135094264167549, -135.9349391362327992 ) ) ;
#25888=CARTESIAN_POINT ( 'NONE',  ( -1.749999999999999778, 20.53108891324555429, -76.12764746908817415 ) ) ;
#25889=CARTESIAN_POINT ( 'NONE',  ( 1.749999999999998224, 14.46891108675448656, -126.6276474690881741 ) ) ;
#25890=CARTESIAN_POINT ( 'NONE',  ( 3.500000000000001332, 17.50000000000001421, -73.15473080337743284 ) ) ;
#25891=CARTESIAN_POINT ( 'NONE',  ( -7.022189441860112050E-16, 13.67729811471672186, -58.60160580289947063 ) ) ;
#25895=CARTESIAN_POINT ( 'NONE',  ( -7.022189441860112050E-16, 13.67729811471672363, -84.60160580289947063 ) ) ;
#25896=CARTESIAN_POINT ( 'NONE',  ( 1.655278471875001101, 20.36702641396249902, -143.1849391362327992 ) ) ;
#25897=CARTESIAN_POINT ( 'NONE',  ( 2.340729813953370519E-16, 21.32270188528331900, -116.0141058028994792 ) ) ;
#25898=CARTESIAN_POINT ( 'NONE',  ( -3.310556943750002645, 15.58864905735837070, -79.68077246956613635 ) ) ;
#25901=CARTESIAN_POINT ( 'NONE',  ( -3.500000000000001332, 17.50000000000002132, -106.6547308033774186 ) ) ;
#25903=CARTESIAN_POINT ( 'NONE',  ( -1.750000000000002220, 14.46891108675448301, -94.48806413671076143 ) ) ;
#25906=CARTESIAN_POINT ( 'NONE',  ( -1.394453263437886604E-15, 14.00000000000001421, -65.71098080242150274 ) ) ;
#25908=CARTESIAN_POINT ( 'NONE',  ( 1.655278471874998436, 14.63297358603754184, -66.43077246956613635 ) ) ;
#25910=ADVANCED_FACE ( 'NONE', ( #5706 ), #9317, .T. ) ;
#25912=CARTESIAN_POINT ( 'NONE',  ( 3.310556943749999981, 15.58864905735837247, -121.3474391362328078 ) ) ;
#25915=EDGE_CURVE ( 'NONE', #14868, #9312, #25864, .T. ) ;
#25918=CARTESIAN_POINT ( 'NONE',  ( -0.9378221735089310451, 14.00000000000001066, -42.75563900116002714 ) ) ;
#25920=CARTESIAN_POINT ( 'NONE',  ( 3.310556943749999981, 15.58864905735836714, -74.34743913623279354 ) ) ;
#25924=AXIS2_PLACEMENT_3D ( 'NONE', #35608, #16465, #3275 ) ;
#25926=CARTESIAN_POINT ( 'NONE',  ( -1.655278471875002211, 14.63297358603755427, -142.5974391362327935 ) ) ;
#25929=CARTESIAN_POINT ( 'NONE',  ( -1.655278471874999990, 20.36702641396248481, -46.01827246956613493 ) ) ;
#25930=CARTESIAN_POINT ( 'NONE',  ( -3.310556943750001313, 17.50000000000001776, -101.8516058028994706 ) ) ;
#25932=CARTESIAN_POINT ( 'NONE',  ( 3.310556943750001313, 19.41135094264165772, -30.18077246956614701 ) ) ;
#25934=CARTESIAN_POINT ( 'NONE',  ( 3.500000000000000000, 15.47927405783632970, -109.5443141357548313 ) ) ;
#25937=CARTESIAN_POINT ( 'NONE',  ( 0.000000000000000000, 21.00000000000002487, -149.5231586289125687 ) ) ;
#25938=CARTESIAN_POINT ( 'NONE',  ( 3.500000000000001332, 17.50000000000001776, -97.15473080337743284 ) ) ;
#25939=CARTESIAN_POINT ( 'NONE',  ( 0.000000000000000000, 21.00000000000002487, -149.5231586289125687 ) ) ;
#25942=CARTESIAN_POINT ( 'NONE',  ( 1.749999999999998224, 14.46891108675447768, -58.62764746908817415 ) ) ;
#25944=DIRECTION ( 'NONE',  ( 0.000000000000000000, 1.000000000000000000, 0.000000000000000000 ) ) ;
#25946=CARTESIAN_POINT ( 'NONE',  ( 1.750000000000001110, 20.53108891324555074, -50.98806413671076854 ) ) ;
#25948=CARTESIAN_POINT ( 'NONE',  ( -3.310556943750001313, 17.50000000000001066, -34.85160580289946353 ) ) ;
#25952=EDGE_CURVE ( 'NONE', #33816, #16704, #38895, .T. ) ;
#25954=CYLINDRICAL_SURFACE ( 'NONE', #15857, 3.499999999999999556 ) ;
#25955=CARTESIAN_POINT ( 'NONE',  ( -3.310556943750001313, 17.50000000000001776, -83.76410580289947916 ) ) ;
#25956=DIRECTION ( 'NONE',  ( 0.000000000000000000, 1.000000000000000000, 0.000000000000000000 ) ) ;
#25957=ORIENTED_EDGE ( 'NONE', *, *, #100, .F. ) ;
#25958=CARTESIAN_POINT ( 'NONE',  ( -3.500000000000002220, 15.47927405783633503, -123.8776474690881741 ) ) ;
#25960=CARTESIAN_POINT ( 'NONE',  ( 0.9378221735089300459, 21.00000000000002132, -107.9493890021159501 ) ) ;
#25963=VECTOR ( 'NONE', #2091, 1000.000000000000000 ) ;
#25965=CARTESIAN_POINT ( 'NONE',  ( -7.022189441860112050E-16, 13.67729811471672363, -89.51410580289949337 ) ) ;
#25967=VERTEX_POINT ( 'NONE', #21135 ) ;
#25968=FACE_OUTER_BOUND ( 'NONE', #35650, .T. ) ;
#25969=VERTEX_POINT ( 'NONE', #34108 ) ;
#25971=CARTESIAN_POINT ( 'NONE',  ( 4.648177544792955347E-16, 21.00000000000001776, -84.90473080337743284 ) ) ;
#25973=CYLINDRICAL_SURFACE ( 'NONE', #11733, 3.499999999999999556 ) ;
#25975=CARTESIAN_POINT ( 'NONE',  ( -3.310556943750001313, 17.50000000000002487, -133.7641058028994507 ) ) ;
#25977=CARTESIAN_POINT ( 'NONE',  ( 3.500000000000001332, 19.52072594216370405, -28.37764746908817770 ) ) ;
#25978=CARTESIAN_POINT ( 'NONE',  ( -1.655278471874999990, 20.36702641396249547, -122.0182724695661278 ) ) ;
#25979=CARTESIAN_POINT ( 'NONE',  ( 3.310556943749999981, 15.58864905735836182, -48.43493913623279923 ) ) ;
#25980=VERTEX_POINT ( 'NONE', #30924 ) ;
#25981=CARTESIAN_POINT ( 'NONE',  ( 3.500000000000001332, 17.50000000000002487, -131.1547308033774186 ) ) ;
#25982=VECTOR ( 'NONE', #15838, 1000.000000000000000 ) ;
#25983=CARTESIAN_POINT ( 'NONE',  ( -3.310556943750001313, 17.50000000000001421, -69.85160580289947063 ) ) ;
#25984=CARTESIAN_POINT ( 'NONE',  ( -3.500000000000002220, 15.47927405783633503, -121.8776474690881884 ) ) ;
#25985=EDGE_CURVE ( 'NONE', #167, #33769, #1141, .T. ) ;
#25986=CARTESIAN_POINT ( 'NONE',  ( 1.655278471874998436, 14.63297358603754716, -107.4307724695661506 ) ) ;
#25988=DIRECTION ( 'NONE',  ( 0.000000000000000000, 1.000000000000000000, 0.000000000000000000 ) ) ;
#25991=CARTESIAN_POINT ( 'NONE',  ( 1.750000000000001110, 20.53108891324555429, -75.29431413575484555 ) ) ;
#25992=CARTESIAN_POINT ( 'NONE',  ( 0.9378221735089300459, 21.00000000000002132, -125.9493890021159643 ) ) ;
#25993=CARTESIAN_POINT ( 'NONE',  ( 3.310556943750001313, 19.41135094264165772, -44.18077246956614346 ) ) ;
#25994=CARTESIAN_POINT ( 'NONE',  ( -7.022189441860112050E-16, 13.67729811471672363, -93.60160580289948484 ) ) ;
#25995=CARTESIAN_POINT ( 'NONE',  ( 2.474675557024783212E-16, 21.54145188432739388, -63.90473080337742573 ) ) ;
#25997=CARTESIAN_POINT ( 'NONE',  ( 3.310556943749999981, 15.58864905735837247, -118.4349391362327850 ) ) ;
#25998=DIRECTION ( 'NONE',  ( -0.000000000000000000, 1.259100132267607459E-16, -1.000000000000000000 ) ) ;
#26002=CARTESIAN_POINT ( 'NONE',  ( 3.500000000000001332, 19.52072594216371115, -79.37764746908817415 ) ) ;
#26004=CARTESIAN_POINT ( 'NONE',  ( 3.310556943750001313, 17.50000000000001776, -98.26410580289947916 ) ) ;
#26007=ORIENTED_EDGE ( 'NONE', *, *, #8193, .F. ) ;
#26009=CARTESIAN_POINT ( 'NONE',  ( -1.749999999999999778, 20.53108891324555785, -127.1276474690881741 ) ) ;
#26010=CARTESIAN_POINT ( 'NONE',  ( 4.286263797015737581E-16, 14.00000000000002487, -149.5231586289125687 ) ) ;
#26011=CARTESIAN_POINT ( 'NONE',  ( -1.836030130193217234E-14, 21.00000000000002487, -135.2109808024214885 ) ) ;
#26014=CARTESIAN_POINT ( 'NONE',  ( -3.310556943750001313, 17.50000000000001066, -29.76410580289948271 ) ) ;
#26015=CYLINDRICAL_SURFACE ( 'NONE', #37290, 3.499999999999999556 ) ;
#26019=CARTESIAN_POINT ( 'NONE',  ( -1.750000000000002220, 14.46891108675449011, -138.4880641367107614 ) ) ;
#26023=CARTESIAN_POINT ( 'NONE',  ( -3.500000000000000000, 19.52072594216371826, -115.0443141357548313 ) ) ;
#26024=CARTESIAN_POINT ( 'NONE',  ( -4.299564228933483745E-15, 21.00000000000002842, -140.2109808024215170 ) ) ;
#26025=CARTESIAN_POINT ( 'NONE',  ( 3.500000000000001332, 17.50000000000002132, -117.1547308033774328 ) ) ;
#26027=CARTESIAN_POINT ( 'NONE',  ( -1.655278471875002211, 14.63297358603755249, -133.6849391362327992 ) ) ;
#26028=CARTESIAN_POINT ( 'NONE',  ( -1.750000000000002220, 14.46891108675447590, -33.79431413575484555 ) ) ;
#26032=( BOUNDED_CURVE ( )  B_SPLINE_CURVE ( 2, ( #30361, #14202, #13782, #26972, #23781, #36747, #40145, #30571, #14412 ),
 .UNSPECIFIED., .F., .F. ) 
 B_SPLINE_CURVE_WITH_KNOTS ( ( 3, 2, 2, 2, 3 ),
 ( 0.4979166666666666741, 0.4986111111111111160, 0.5000000000000000000, 0.5013888888888888840, 0.5020833333333333259 ),
 .UNSPECIFIED. ) 
 CURVE ( )  GEOMETRIC_REPRESENTATION_ITEM ( )  RATIONAL_B_SPLINE_CURVE ( ( 0.9330127018922194093, 0.9330127018922194093, 1.000000000000000000, 0.8660254037844387076, 1.000000000000000000, 0.8660254037844387076, 1.000000000000000000, 0.9330127018922194093, 0.9330127018922194093 ) ) 
 REPRESENTATION_ITEM ( '' )  );
#26033=CARTESIAN_POINT ( 'NONE',  ( -1.394453263437886604E-15, 14.00000000000001066, -40.40473080337742573 ) ) ;
#26035=CARTESIAN_POINT ( 'NONE',  ( 3.500000000000001776, 19.52072594216372181, -141.3776474690881741 ) ) ;
#26036=CARTESIAN_POINT ( 'NONE',  ( 3.310556943750001313, 17.50000000000002132, -121.2641058028994792 ) ) ;
#26041=CARTESIAN_POINT ( 'NONE',  ( 3.500000000000001332, 17.50000000000001776, -90.46098080242151696 ) ) ;
#26042=CARTESIAN_POINT ( 'NONE',  ( -3.500000000000000000, 19.52072594216370405, -45.73806413671076143 ) ) ;
#26043=CARTESIAN_POINT ( 'NONE',  ( 2.340729813953370519E-16, 21.32270188528330834, -57.01410580289947916 ) ) ;
#26044=CARTESIAN_POINT ( 'NONE',  ( -3.310556943750001313, 17.50000000000002132, -114.8516058028994706 ) ) ;
#26045=CARTESIAN_POINT ( 'NONE',  ( 3.500000000000001776, 19.52072594216370405, -30.07139747004410069 ) ) ;
#26046=CARTESIAN_POINT ( 'NONE',  ( 4.286263797015737581E-16, 14.00000000000002487, -149.5231586289125687 ) ) ;
#26048=CARTESIAN_POINT ( 'NONE',  ( 1.655278471874998436, 14.63297358603755072, -134.5182724695661420 ) ) ;
#26050=ADVANCED_FACE ( 'NONE', ( #11551 ), #15599, .T. ) ;
#26052=CARTESIAN_POINT ( 'NONE',  ( -0.9378221735089291577, 21.00000000000001421, -66.86007260463890134 ) ) ;
#26053=CARTESIAN_POINT ( 'NONE',  ( 4.648177544792955347E-16, 21.00000000000002132, -118.2109808024215170 ) ) ;
#26055=CARTESIAN_POINT ( 'NONE',  ( -3.310556943750002645, 15.58864905735837070, -69.76827246956612782 ) ) ;
#26057=CARTESIAN_POINT ( 'NONE',  ( -1.655278471874999990, 20.36702641396248836, -65.93077246956613635 ) ) ;
#26058=VERTEX_POINT ( 'NONE', #21345 ) ;
#26059=CARTESIAN_POINT ( 'NONE',  ( -1.655278471875002211, 14.63297358603754716, -85.68493913623278502 ) ) ;
#26062=LINE ( 'NONE', #16282, #40362 ) ;
#26063=CARTESIAN_POINT ( 'NONE',  ( -0.9378221735089310451, 14.00000000000001066, -41.75563900116002714 ) ) ;
#26064=CARTESIAN_POINT ( 'NONE',  ( 2.340729813953370519E-16, 21.32270188528331190, -52.01410580289947205 ) ) ;
#26066=CARTESIAN_POINT ( 'NONE',  ( 1.655278471875001101, 20.36702641396249547, -103.0974391362328220 ) ) ;
#26067=CARTESIAN_POINT ( 'NONE',  ( 0.000000000000000000, 17.50000000000002487, -149.5231586289125687 ) ) ;
#26071=ORIENTED_EDGE ( 'NONE', *, *, #5631, .F. ) ;
#26073=CARTESIAN_POINT ( 'NONE',  ( 3.310556943750001313, 19.41135094264166128, -58.18077246956614346 ) ) ;
#26075=ORIENTED_EDGE ( 'NONE', *, *, #9535, .T. ) ;
#26076=DIRECTION ( 'NONE',  ( -0.000000000000000000, 1.259100132267607459E-16, -1.000000000000000000 ) ) ;
#26077=DIRECTION ( 'NONE',  ( 0.000000000000000000, 1.000000000000000000, 0.000000000000000000 ) ) ;
#26080=CARTESIAN_POINT ( 'NONE',  ( 3.500000000000000000, 15.47927405783633326, -114.5443141357548171 ) ) ;
#26083=CARTESIAN_POINT ( 'NONE',  ( -1.655278471875002211, 14.63297358603755249, -126.5974391362328078 ) ) ;
#26087=CARTESIAN_POINT ( 'NONE',  ( 2.340729813953370519E-16, 21.32270188528330479, -33.10160580289945642 ) ) ;
#26088=CARTESIAN_POINT ( 'NONE',  ( -1.655278471874999990, 20.36702641396248481, -25.01827246956613138 ) ) ;
#26089=CARTESIAN_POINT ( 'NONE',  ( 3.310556943750001313, 19.41135094264166483, -88.26827246956612782 ) ) ;
#26090=CARTESIAN_POINT ( 'NONE',  ( 1.655278471874998436, 14.63297358603755249, -137.4307724695661364 ) ) ;
#26094=CARTESIAN_POINT ( 'NONE',  ( -1.394453263437886604E-15, 14.00000000000001776, -100.4047308033774328 ) ) ;
#26095=CARTESIAN_POINT ( 'NONE',  ( 2.340729813953370519E-16, 21.32270188528332255, -131.1016058028994564 ) ) ;
#26096=CARTESIAN_POINT ( 'NONE',  ( 4.648177544792955347E-16, 21.00000000000001421, -56.21098080242151696 ) ) ;
#26097=CARTESIAN_POINT ( 'NONE',  ( 2.340729813953370519E-16, 21.32270188528331190, -93.01410580289949337 ) ) ;
#26098=DIRECTION ( 'NONE',  ( -0.000000000000000000, 1.259100132267607459E-16, -1.000000000000000000 ) ) ;
#26099=CARTESIAN_POINT ( 'NONE',  ( -3.500000000000000000, 19.52072594216371115, -93.04431413575484555 ) ) ;
#26100=CARTESIAN_POINT ( 'NONE',  ( 3.500000000000001332, 19.52072594216371826, -111.3776474690881599 ) ) ;
#26101=CARTESIAN_POINT ( 'NONE',  ( -3.500000000000000888, 19.52072594216370760, -72.73806413671076143 ) ) ;
#26102=CARTESIAN_POINT ( 'NONE',  ( -7.022189441860112050E-16, 13.67729811471672186, -59.60160580289947063 ) ) ;
#26106=CARTESIAN_POINT ( 'NONE',  ( 2.340729813953370519E-16, 21.32270188528331190, -87.10160580289945642 ) ) ;
#26108=CARTESIAN_POINT ( 'NONE',  ( 3.310556943750001313, 17.50000000000002132, -113.2641058028994792 ) ) ;
#26109=CARTESIAN_POINT ( 'NONE',  ( -3.310556943750000425, 19.41135094264166483, -79.84743913623279354 ) ) ;
#26110=CARTESIAN_POINT ( 'NONE',  ( 4.648177544792955347E-16, 21.00000000000001776, -96.90473080337741862 ) ) ;
#26112=CARTESIAN_POINT ( 'NONE',  ( 1.655278471874998436, 14.63297358603754716, -104.5182724695661278 ) ) ;
#26113=CARTESIAN_POINT ( 'NONE',  ( -1.750000000000002220, 14.46891108675448478, -102.4880641367107756 ) ) ;
#26114=VECTOR ( 'NONE', #10184, 1000.000000000000000 ) ;
#26117=DIRECTION ( 'NONE',  ( -0.000000000000000000, 1.259100132267607459E-16, -1.000000000000000000 ) ) ;
#26120=CARTESIAN_POINT ( 'NONE',  ( 2.340729813953370519E-16, 21.32270188528331190, -68.01410580289947916 ) ) ;
#26121=( BOUNDED_CURVE ( )  B_SPLINE_CURVE ( 2, ( #5485, #12282, #18675, #18461, #38448, #15915, #22275, #41862, #28862 ),
 .UNSPECIFIED., .F., .F. ) 
 B_SPLINE_CURVE_WITH_KNOTS ( ( 3, 2, 2, 2, 3 ),
 ( 0.9062500000000000000, 0.9069444444444444420, 0.9083333333333333259, 0.9097222222222222099, 0.9104166666666666519 ),
 .UNSPECIFIED. ) 
 CURVE ( )  GEOMETRIC_REPRESENTATION_ITEM ( )  RATIONAL_B_SPLINE_CURVE ( ( 0.9330127018922194093, 0.9330127018922194093, 1.000000000000000000, 0.8660254037844387076, 1.000000000000000000, 0.8660254037844387076, 1.000000000000000000, 0.9330127018922194093, 0.9330127018922194093 ) ) 
 REPRESENTATION_ITEM ( '' )  );
#26123=EDGE_CURVE ( 'NONE', #25503, #3199, #6015, .T. ) ;
#26124=CARTESIAN_POINT ( 'NONE',  ( -1.655278471875002211, 14.63297358603755072, -121.5974391362328078 ) ) ;
#26126=EDGE_CURVE ( 'NONE', #9158, #24772, #11760, .T. ) ;
#26131=CARTESIAN_POINT ( 'NONE',  ( -1.394453263437886604E-15, 14.00000000000001066, -39.40473080337742573 ) ) ;
#26133=CARTESIAN_POINT ( 'NONE',  ( -3.310556943750001313, 17.50000000000001776, -75.76410580289946495 ) ) ;
#26134=ORIENTED_EDGE ( 'NONE', *, *, #36903, .T. ) ;
#26137=CARTESIAN_POINT ( 'NONE',  ( -1.655278471874999990, 20.36702641396249902, -138.9307724695661364 ) ) ;
#26140=ADVANCED_FACE ( 'NONE', ( #21759 ), #37723, .T. ) ;
#26141=CARTESIAN_POINT ( 'NONE',  ( 1.750000000000001110, 20.53108891324556140, -134.2943141357548598 ) ) ;
#26142=CARTESIAN_POINT ( 'NONE',  ( -3.310556943750001313, 17.50000000000001066, -43.85160580289947063 ) ) ;
#26143=CARTESIAN_POINT ( 'NONE',  ( -3.310556943750000425, 19.41135094264166838, -105.9349391362328134 ) ) ;
#26144=ADVANCED_FACE ( 'NONE', ( #2409 ), #15396, .T. ) ;
#26145=CARTESIAN_POINT ( 'NONE',  ( 3.310556943750001313, 19.41135094264165772, -27.18077246956613990 ) ) ;
#26148=CARTESIAN_POINT ( 'NONE',  ( 1.749999999999998224, 14.46891108675448301, -103.6276474690881741 ) ) ;
#26150=CARTESIAN_POINT ( 'NONE',  ( 3.500000000000001332, 17.50000000000002487, -142.1547308033774186 ) ) ;
#26151=CARTESIAN_POINT ( 'NONE',  ( -3.500000000000001332, 17.50000000000001776, -88.65473080337743284 ) ) ;
#26152=CARTESIAN_POINT ( 'NONE',  ( -1.750000000000002220, 14.46891108675448123, -77.79431413575484555 ) ) ;
#26155=CARTESIAN_POINT ( 'NONE',  ( -7.424026671074350129E-16, 13.45854811567263454, -61.71098080242150274 ) ) ;
#26157=CARTESIAN_POINT ( 'NONE',  ( -1.749999999999999778, 20.53108891324554719, -25.12764746908817415 ) ) ;
#26158=CARTESIAN_POINT ( 'NONE',  ( 1.750000000000001110, 20.53108891324554719, -42.98806413671076143 ) ) ;
#26160=CARTESIAN_POINT ( 'NONE',  ( 1.655278471875001101, 20.36702641396248481, -29.18493913623279568 ) ) ;
#26162=CYLINDRICAL_SURFACE ( 'NONE', #15183, 3.499999999999999556 ) ;
#26167=CARTESIAN_POINT ( 'NONE',  ( -7.022189441860112050E-16, 13.67729811471672363, -82.51410580289947916 ) ) ;
#26171=( BOUNDED_CURVE ( )  B_SPLINE_CURVE ( 2, ( #41900, #25303, #25728, #15524, #19337, #18496, #38691, #9131, #28480 ),
 .UNSPECIFIED., .F., .F. ) 
 B_SPLINE_CURVE_WITH_KNOTS ( ( 3, 2, 2, 2, 3 ),
 ( 0.2854166666666666519, 0.2861111111111110938, 0.2874999999999999778, 0.2888888888888888618, 0.2895833333333333592 ),
 .UNSPECIFIED. ) 
 CURVE ( )  GEOMETRIC_REPRESENTATION_ITEM ( )  RATIONAL_B_SPLINE_CURVE ( ( 0.9330127018922194093, 0.9330127018922194093, 1.000000000000000000, 0.8660254037844387076, 1.000000000000000000, 0.8660254037844387076, 1.000000000000000000, 0.9330127018922167448, 0.9330127018922194093 ) ) 
 REPRESENTATION_ITEM ( '' )  );
#26172=CARTESIAN_POINT ( 'NONE',  ( 3.500000000000001332, 17.50000000000002132, -108.1547308033774186 ) ) ;
#26176=CARTESIAN_POINT ( 'NONE',  ( -3.310556943750002645, 15.58864905735837247, -88.68077246956613635 ) ) ;
#26179=AXIS2_PLACEMENT_3D ( 'NONE', #4589, #40106, #7155 ) ;
#26184=CARTESIAN_POINT ( 'NONE',  ( -0.9378221735089291577, 21.00000000000001776, -88.86007260463890134 ) ) ;
#26185=DIRECTION ( 'NONE',  ( 0.000000000000000000, 1.000000000000000000, 0.000000000000000000 ) ) ;
#26186=CARTESIAN_POINT ( 'NONE',  ( 1.655278471874998436, 14.63297358603755072, -133.4307724695661364 ) ) ;
#26189=CARTESIAN_POINT ( 'NONE',  ( -1.394453263437886604E-15, 14.00000000000001421, -64.40473080337743284 ) ) ;
#26190=CARTESIAN_POINT ( 'NONE',  ( -3.310556943750000425, 19.41135094264166838, -121.9349391362327850 ) ) ;
#26191=VERTEX_POINT ( 'NONE', #37927 ) ;
#26192=EDGE_CURVE ( 'NONE', #15295, #27367, #24757, .T. ) ;
#26193=EDGE_LOOP ( 'NONE', ( #22153, #27116, #36686, #34156 ) ) ;
#26194=CARTESIAN_POINT ( 'NONE',  ( 2.474675557024783212E-16, 21.54145188432740810, -132.9047308033774186 ) ) ;
#26195=EDGE_CURVE ( 'NONE', #23270, #32852, #8700, .T. ) ;
#26196=CARTESIAN_POINT ( 'NONE',  ( 2.340729813953370519E-16, 21.32270188528330834, -71.10160580289947063 ) ) ;
#26197=CARTESIAN_POINT ( 'NONE',  ( 2.474675557024783212E-16, 21.54145188432740099, -119.2109808024215170 ) ) ;
#26198=CARTESIAN_POINT ( 'NONE',  ( -3.310556943750000425, 19.41135094264166483, -100.8474391362328220 ) ) ;
#26200=CARTESIAN_POINT ( 'NONE',  ( 7.785697387528201340E-15, 14.00000000000002487, -138.7109808024215170 ) ) ;
#26202=CARTESIAN_POINT ( 'NONE',  ( -3.500000000000001332, 17.50000000000001421, -72.96098080242151696 ) ) ;
#26204=CARTESIAN_POINT ( 'NONE',  ( 3.310556943750001313, 17.50000000000001066, -38.26410580289947916 ) ) ;
#26205=CARTESIAN_POINT ( 'NONE',  ( 3.310556943750001313, 17.50000000000001776, -94.35160580289947063 ) ) ;
#26206=CARTESIAN_POINT ( 'NONE',  ( -7.424026671074350129E-16, 13.45854811567263454, -63.40473080337742573 ) ) ;
#26209=CARTESIAN_POINT ( 'NONE',  ( 3.310556943750001313, 19.41135094264166838, -116.2682724695661278 ) ) ;
#26210=CARTESIAN_POINT ( 'NONE',  ( 3.500000000000000000, 15.47927405783633503, -127.5443141357548456 ) ) ;
#26214=CARTESIAN_POINT ( 'NONE',  ( 4.648177544792955347E-16, 21.00000000000002132, -120.2109808024215170 ) ) ;
#26215=CARTESIAN_POINT ( 'NONE',  ( -1.655278471875002211, 14.63297358603754894, -96.59743913623280775 ) ) ;
#26219=CARTESIAN_POINT ( 'NONE',  ( 3.500000000000001332, 17.50000000000001421, -48.15473080337742573 ) ) ;
#26220=CARTESIAN_POINT ( 'NONE',  ( 4.648177544792955347E-16, 21.00000000000001066, -44.90473080337743994 ) ) ;
#26222=CARTESIAN_POINT ( 'NONE',  ( -3.500000000000002220, 15.47927405783633503, -134.8776474690881741 ) ) ;
#26225=CARTESIAN_POINT ( 'NONE',  ( -3.310556943750001313, 17.50000000000001066, -27.76410580289947916 ) ) ;
#26226=ORIENTED_EDGE ( 'NONE', *, *, #15769, .T. ) ;
#26232=CARTESIAN_POINT ( 'NONE',  ( -0.9378221735089310451, 14.00000000000002132, -99.75563900116003424 ) ) ;
#26235=CARTESIAN_POINT ( 'NONE',  ( -3.500000000000000000, 19.52072594216371115, -86.04431413575483134 ) ) ;
#26236=DIRECTION ( 'NONE',  ( 0.000000000000000000, 1.000000000000000000, 0.000000000000000000 ) ) ;
#26238=CARTESIAN_POINT ( 'NONE',  ( 3.500000000000001332, 17.50000000000002132, -119.1547308033774328 ) ) ;
#26241=CARTESIAN_POINT ( 'NONE',  ( 1.655278471874998436, 14.63297358603755249, -136.5182724695661420 ) ) ;
#26242=CARTESIAN_POINT ( 'NONE',  ( -3.500000000000002220, 15.47927405783632082, -25.87764746908817415 ) ) ;
#26244=CARTESIAN_POINT ( 'NONE',  ( 3.500000000000000000, 15.47927405783632082, -32.54431413575484555 ) ) ;
#26247=CARTESIAN_POINT ( 'NONE',  ( 1.750000000000001110, 20.53108891324556140, -141.2943141357548313 ) ) ;
#26248=CARTESIAN_POINT ( 'NONE',  ( 1.655278471874998436, 14.63297358603754894, -119.4307724695661364 ) ) ;
#26251=CARTESIAN_POINT ( 'NONE',  ( 0.000000000000000000, 17.50000000000002487, -149.5231586289125687 ) ) ;
#26252=CARTESIAN_POINT ( 'NONE',  ( -3.500000000000000888, 19.52072594216371115, -93.04431413575483134 ) ) ;
#26254=CARTESIAN_POINT ( 'NONE',  ( 1.655278471874998436, 14.63297358603754006, -52.43077246956613635 ) ) ;
#26255=CARTESIAN_POINT ( 'NONE',  ( 1.655278471874998436, 14.63297358603754894, -113.5182724695661278 ) ) ;
#26257=CARTESIAN_POINT ( 'NONE',  ( -7.424026671074350129E-16, 13.45854811567263098, -30.40473080337742573 ) ) ;
#26260=CARTESIAN_POINT ( 'NONE',  ( -7.022189441860112050E-16, 13.67729811471672896, -133.6016058028994564 ) ) ;
#26262=CARTESIAN_POINT ( 'NONE',  ( -3.500000000000000000, 19.52072594216370760, -66.73806413671076143 ) ) ;
#26264=CARTESIAN_POINT ( 'NONE',  ( -3.310556943750000425, 19.41135094264166128, -61.93493913623280633 ) ) ;
#26266=CARTESIAN_POINT ( 'NONE',  ( -7.022189441860112050E-16, 13.67729811471671830, -62.51410580289947205 ) ) ;
#26267=ORIENTED_EDGE ( 'NONE', *, *, #35208, .T. ) ;
#26269=CARTESIAN_POINT ( 'NONE',  ( -1.655278471874999990, 20.36702641396249192, -88.01827246956612782 ) ) ;
#26271=EDGE_CURVE ( 'NONE', #18011, #28293, #13056, .T. ) ;
#26274=CARTESIAN_POINT ( 'NONE',  ( 3.310556943750001313, 17.50000000000001066, -45.26410580289947916 ) ) ;
#26276=CARTESIAN_POINT ( 'NONE',  ( -1.655278471874999990, 20.36702641396249547, -103.9307724695661364 ) ) ;
#26277=ORIENTED_EDGE ( 'NONE', *, *, #100, .T. ) ;
#26281=CARTESIAN_POINT ( 'NONE',  ( 2.340729813953370519E-16, 21.32270188528330834, -60.01410580289947916 ) ) ;
#26282=ORIENTED_EDGE ( 'NONE', *, *, #30999, .T. ) ;
#26284=( BOUNDED_CURVE ( )  B_SPLINE_CURVE ( 2, ( #25256, #38222, #5473, #12057, #21847, #34821, #34404, #9083, #31831 ),
 .UNSPECIFIED., .F., .T. ) 
 B_SPLINE_CURVE_WITH_KNOTS ( ( 3, 2, 2, 2, 3 ),
 ( 0.1687500000000000111, 0.1694444444444444531, 0.1708333333333333370, 0.1722222222222222210, 0.1729166666666666630 ),
 .UNSPECIFIED. ) 
 CURVE ( )  GEOMETRIC_REPRESENTATION_ITEM ( )  RATIONAL_B_SPLINE_CURVE ( ( 0.9330127018922194093, 0.9330127018922194093, 1.000000000000000000, 0.8660254037844387076, 1.000000000000000000, 0.8660254037844387076, 1.000000000000000000, 0.9330127018922194093, 0.9330127018922194093 ) ) 
 REPRESENTATION_ITEM ( '' )  );
#26285=CARTESIAN_POINT ( 'NONE',  ( 3.405278471875001323, 17.50000000000002487, -143.4062933026604583 ) ) ;
#26288=( BOUNDED_CURVE ( )  B_SPLINE_CURVE ( 2, ( #40633, #24694, #8513, #37246, #27662, #31478, #6375, #35515, #16176 ),
 .UNSPECIFIED., .F., .T. ) 
 B_SPLINE_CURVE_WITH_KNOTS ( ( 3, 2, 2, 2, 3 ),
 ( 0.6395833333333332815, 0.6402777777777777235, 0.6416666666666667185, 0.6430555555555556024, 0.6437500000000000444 ),
 .UNSPECIFIED. ) 
 CURVE ( )  GEOMETRIC_REPRESENTATION_ITEM ( )  RATIONAL_B_SPLINE_CURVE ( ( 0.9330127018922194093, 0.9330127018922194093, 1.000000000000000000, 0.8660254037844387076, 1.000000000000000000, 0.8660254037844387076, 1.000000000000000000, 0.9330127018922194093, 0.9330127018922194093 ) ) 
 REPRESENTATION_ITEM ( '' )  );
#26292=VERTEX_POINT ( 'NONE', #32579 ) ;
#26293=CARTESIAN_POINT ( 'NONE',  ( 4.648177544792955347E-16, 21.00000000000001066, -39.21098080242150985 ) ) ;
#26294=CARTESIAN_POINT ( 'NONE',  ( 3.310556943749999981, 15.58864905735837425, -127.3474391362328078 ) ) ;
#26295=ADVANCED_FACE ( 'NONE', ( #28759 ), #252, .T. ) ;
#26296=CARTESIAN_POINT ( 'NONE',  ( 3.602337597214540226E-14, 14.00000000000002132, -117.4047308033774328 ) ) ;
#26298=CARTESIAN_POINT ( 'NONE',  ( -3.310556943750000425, 19.41135094264165772, -32.93493913623279923 ) ) ;
#26299=CARTESIAN_POINT ( 'NONE',  ( 4.648177544792955347E-16, 21.00000000000002132, -117.2109808024215170 ) ) ;
#26300=CARTESIAN_POINT ( 'NONE',  ( -7.022189441860112050E-16, 13.67729811471672363, -87.60160580289947063 ) ) ;
#26301=CARTESIAN_POINT ( 'NONE',  ( -3.310556943750002645, 15.58864905735837958, -141.6807724695661648 ) ) ;
#26305=CARTESIAN_POINT ( 'NONE',  ( -3.310556943750001313, 17.50000000000002132, -127.8516058028994422 ) ) ;
#26306=CARTESIAN_POINT ( 'NONE',  ( -7.022189441860112050E-16, 13.67729811471672363, -93.51410580289947916 ) ) ;
#26307=CARTESIAN_POINT ( 'NONE',  ( 0.9378221735089281585, 14.00000000000000711, -24.66632260368298546 ) ) ;
#26308=CARTESIAN_POINT ( 'NONE',  ( -0.9378221735089310451, 14.00000000000002132, -92.75563900116002003 ) ) ;
#26309=CARTESIAN_POINT ( 'NONE',  ( 1.749999999999998224, 14.46891108675448478, -111.6276474690881884 ) ) ;
#26310=CARTESIAN_POINT ( 'NONE',  ( 1.749999999999998224, 14.46891108675447946, -75.32139747004410424 ) ) ;
#26311=CARTESIAN_POINT ( 'NONE',  ( 3.310556943750001313, 19.41135094264166483, -58.26827246956613493 ) ) ;
#26315=CARTESIAN_POINT ( 'NONE',  ( -3.310556943750000425, 19.41135094264166483, -84.93493913623279923 ) ) ;
#26318=CARTESIAN_POINT ( 'NONE',  ( 1.655278471874998436, 14.63297358603754716, -106.4307724695661364 ) ) ;
#26319=CARTESIAN_POINT ( 'NONE',  ( 3.310556943749999981, 15.58864905735836714, -79.34743913623282197 ) ) ;
#26320=CARTESIAN_POINT ( 'NONE',  ( -1.749999999999999778, 20.53108891324555429, -96.82139747004409003 ) ) ;
#26321=ORIENTED_EDGE ( 'NONE', *, *, #2372, .F. ) ;
#26322=CARTESIAN_POINT ( 'NONE',  ( 3.310556943750001313, 17.50000000000002132, -102.3516058028994564 ) ) ;
#26323=CARTESIAN_POINT ( 'NONE',  ( -3.500000000000002220, 15.47927405783632970, -104.5713974700440900 ) ) ;
#26325=DIRECTION ( 'NONE',  ( -0.000000000000000000, 1.259100132267607459E-16, -1.000000000000000000 ) ) ;
#26326=CARTESIAN_POINT ( 'NONE',  ( 1.750000000000001110, 20.53108891324555785, -104.9880641367107614 ) ) ;
#26327=CARTESIAN_POINT ( 'NONE',  ( -1.394453263437886604E-15, 14.00000000000001421, -58.40473080337741862 ) ) ;
#26329=CARTESIAN_POINT ( 'NONE',  ( -1.655278471875002211, 14.63297358603754361, -58.59743913623280065 ) ) ;
#26331=CARTESIAN_POINT ( 'NONE',  ( -1.655278471874999990, 20.36702641396249547, -122.9307724695661506 ) ) ;
#26336=DIRECTION ( 'NONE',  ( -0.000000000000000000, 1.259100132267607459E-16, -1.000000000000000000 ) ) ;
#26337=CARTESIAN_POINT ( 'NONE',  ( -1.394453263437886604E-15, 14.00000000000000711, -24.71098080242150985 ) ) ;
#26338=CARTESIAN_POINT ( 'NONE',  ( -7.022189441860112050E-16, 13.67729811471672186, -71.51410580289947916 ) ) ;
#26340=ORIENTED_EDGE ( 'NONE', *, *, #24416, .T. ) ;
#26343=CARTESIAN_POINT ( 'NONE',  ( 1.655278471874998436, 14.63297358603755249, -139.4307724695661364 ) ) ;
#26344=CARTESIAN_POINT ( 'NONE',  ( -3.500000000000002220, 15.47927405783633503, -128.8776474690881741 ) ) ;
#26346=CARTESIAN_POINT ( 'NONE',  ( 2.340729813953370519E-16, 21.32270188528330479, -39.10160580289947063 ) ) ;
#26347=CARTESIAN_POINT ( 'NONE',  ( 1.655278471874998436, 14.63297358603754716, -103.5182724695661278 ) ) ;
#26349=CARTESIAN_POINT ( 'NONE',  ( 2.340729813953370519E-16, 21.32270188528332255, -143.1016058028994564 ) ) ;
#26351=CARTESIAN_POINT ( 'NONE',  ( 3.500000000000001332, 17.50000000000002132, -102.4609808024215027 ) ) ;
#26353=CARTESIAN_POINT ( 'NONE',  ( 0.000000000000000000, 17.50000000000002487, -149.5231586289125687 ) ) ;
#26354=CARTESIAN_POINT ( 'NONE',  ( 2.474675557024783212E-16, 21.54145188432739744, -91.90473080337743284 ) ) ;
#26358=CARTESIAN_POINT ( 'NONE',  ( 1.750000000000001110, 20.53108891324555074, -56.29431413575483845 ) ) ;
#26361=CARTESIAN_POINT ( 'NONE',  ( -3.500000000000001332, 17.50000000000001066, -42.65473080337743284 ) ) ;
#26363=CARTESIAN_POINT ( 'NONE',  ( 1.655278471875001101, 20.36702641396248481, -26.18493913623279212 ) ) ;
#26365=CARTESIAN_POINT ( 'NONE',  ( 3.500000000000000000, 15.47927405783632615, -75.23806413671076143 ) ) ;
#26368=CARTESIAN_POINT ( 'NONE',  ( 3.500000000000001332, 19.52072594216370405, -36.07139747004409003 ) ) ;
#26370=CARTESIAN_POINT ( 'NONE',  ( -3.310556943750000425, 19.41135094264166838, -83.84743913623279354 ) ) ;
#26372=ORIENTED_EDGE ( 'NONE', *, *, #10968, .T. ) ;
#26373=CARTESIAN_POINT ( 'NONE',  ( -3.500000000000001332, 17.50000000000001066, -35.65473080337743284 ) ) ;
#26374=CARTESIAN_POINT ( 'NONE',  ( 1.750000000000001110, 20.53108891324555429, -80.29431413575484555 ) ) ;
#26375=ORIENTED_EDGE ( 'NONE', *, *, #30553, .F. ) ;
#26376=CARTESIAN_POINT ( 'NONE',  ( -0.9378221735089640188, 20.99999999999999645, -88.16632260368298546 ) ) ;
#26377=CARTESIAN_POINT ( 'NONE',  ( -1.655278471874999990, 20.36702641396249192, -90.93077246956613635 ) ) ;
#26378=EDGE_CURVE ( 'NONE', #28825, #38312, #23125, .T. ) ;
#26383=CARTESIAN_POINT ( 'NONE',  ( 4.286263797015737581E-16, 14.00000000000002487, -149.5231586289125687 ) ) ;
#26386=CARTESIAN_POINT ( 'NONE',  ( -3.310556943750000425, 19.41135094264166838, -127.8474391362328078 ) ) ;
#26387=ORIENTED_EDGE ( 'NONE', *, *, #8465, .F. ) ;
#26389=CARTESIAN_POINT ( 'NONE',  ( -1.655278471875002211, 14.63297358603754184, -51.68493913623279923 ) ) ;
#26390=CARTESIAN_POINT ( 'NONE',  ( -1.655278471874999990, 20.36702641396249547, -119.0182724695661278 ) ) ;
#26394=CARTESIAN_POINT ( 'NONE',  ( -3.500000000000001332, 17.50000000000002487, -130.6547308033774186 ) ) ;
#26395=EDGE_CURVE ( 'NONE', #28207, #26790, #10076, .T. ) ;
#26396=CARTESIAN_POINT ( 'NONE',  ( -7.022189441860112050E-16, 13.67729811471672186, -69.60160580289947063 ) ) ;
#26397=CARTESIAN_POINT ( 'NONE',  ( 1.750000000000001110, 20.53108891324555785, -116.2943141357548313 ) ) ;
#26398=CARTESIAN_POINT ( 'NONE',  ( 2.340729813953370519E-16, 21.32270188528331190, -100.0141058028994792 ) ) ;
#26402=CARTESIAN_POINT ( 'NONE',  ( -1.749999999999999778, 20.53108891324555074, -69.12764746908817415 ) ) ;
#26404=CARTESIAN_POINT ( 'NONE',  ( -3.310556943750001313, 17.50000000000001066, -36.76410580289947205 ) ) ;
#26405=( BOUNDED_CURVE ( )  B_SPLINE_CURVE ( 2, ( #3775, #36315, #7823, #23992, #23775, #39502, #1226, #16761, #36961 ),
 .UNSPECIFIED., .F., .T. ) 
 B_SPLINE_CURVE_WITH_KNOTS ( ( 3, 2, 2, 2, 3 ),
 ( 0.09791666666666666574, 0.09861111111111110772, 0.1000000000000000056, 0.1013888888888888895, 0.1020833333333333315 ),
 .UNSPECIFIED. ) 
 CURVE ( )  GEOMETRIC_REPRESENTATION_ITEM ( )  RATIONAL_B_SPLINE_CURVE ( ( 0.9330127018922194093, 0.9330127018922194093, 1.000000000000000000, 0.8660254037844387076, 1.000000000000000000, 0.8660254037844387076, 1.000000000000000000, 0.9330127018922194093, 0.9330127018922194093 ) ) 
 REPRESENTATION_ITEM ( '' )  );
#26406=CARTESIAN_POINT ( 'NONE',  ( -3.310556943750002645, 15.58864905735837425, -96.76827246956612782 ) ) ;
#26407=CARTESIAN_POINT ( 'NONE',  ( 3.500000000000001776, 19.52072594216370760, -57.07139747004409713 ) ) ;
#26408=CARTESIAN_POINT ( 'NONE',  ( 3.310556943749999981, 15.58864905735837247, -119.4349391362328134 ) ) ;
#26410=CARTESIAN_POINT ( 'NONE',  ( -0.9378221735089291577, 21.00000000000001421, -62.86007260463890844 ) ) ;
#26415=CARTESIAN_POINT ( 'NONE',  ( -3.310556943750000425, 19.41135094264166838, -99.84743913623282197 ) ) ;
#26416=CARTESIAN_POINT ( 'NONE',  ( -1.394453263437886604E-15, 14.00000000000001066, -39.40473080337742573 ) ) ;
#26419=CARTESIAN_POINT ( 'NONE',  ( -0.9378221735089310451, 14.00000000000002132, -87.44938900211595012 ) ) ;
#26420=CARTESIAN_POINT ( 'NONE',  ( 3.500000000000001332, 19.52072594216371115, -81.37764746908818836 ) ) ;
#26422=EDGE_LOOP ( 'NONE', ( #42034, #40141, #18598, #27879 ) ) ;
#26423=CARTESIAN_POINT ( 'NONE',  ( -1.750000000000002220, 14.46891108675448834, -134.7943141357548598 ) ) ;
#26426=CARTESIAN_POINT ( 'NONE',  ( -3.310556943750001313, 17.50000000000001066, -28.76410580289948271 ) ) ;
#26427=EDGE_CURVE ( 'NONE', #8887, #13926, #35054, .T. ) ;
#26429=ORIENTED_EDGE ( 'NONE', *, *, #29040, .T. ) ;
#26430=CARTESIAN_POINT ( 'NONE',  ( -0.9378221735089291577, 21.00000000000002132, -109.8600726046389155 ) ) ;
#26436=DIRECTION ( 'NONE',  ( -0.000000000000000000, 1.259100132267607459E-16, -1.000000000000000000 ) ) ;
#26438=CARTESIAN_POINT ( 'NONE',  ( 3.500000000000000000, 15.47927405783633503, -140.5443141357548313 ) ) ;
#26439=CARTESIAN_POINT ( 'NONE',  ( -1.394453263437886604E-15, 14.00000000000001776, -104.7109808024215027 ) ) ;
#26440=CARTESIAN_POINT ( 'NONE',  ( -7.022189441860112050E-16, 13.67729811471672896, -137.6016058028994564 ) ) ;
#26441=CARTESIAN_POINT ( 'NONE',  ( -1.749999999999999778, 20.53108891324554719, -28.12764746908817770 ) ) ;
#26447=CARTESIAN_POINT ( 'NONE',  ( -1.749999999999999778, 20.53108891324556140, -136.1276474690881741 ) ) ;
#26448=CARTESIAN_POINT ( 'NONE',  ( 3.310556943749999981, 15.58864905735837247, -117.3474391362328078 ) ) ;
#26451=FACE_OUTER_BOUND ( 'NONE', #16765, .T. ) ;
#26452=CARTESIAN_POINT ( 'NONE',  ( -3.500000000000000888, 19.52072594216371115, -86.04431413575484555 ) ) ;
#26454=CARTESIAN_POINT ( 'NONE',  ( -1.394453263437886604E-15, 14.00000000000001066, -36.71098080242150985 ) ) ;
#26455=CARTESIAN_POINT ( 'NONE',  ( -1.655278471874999990, 20.36702641396248836, -52.93077246956613635 ) ) ;
#26456=CARTESIAN_POINT ( 'NONE',  ( 3.310556943750001313, 17.50000000000002132, -111.3516058028994564 ) ) ;
#26457=CARTESIAN_POINT ( 'NONE',  ( -1.394453263437886604E-15, 14.00000000000001066, -38.71098080242150985 ) ) ;
#26458=CARTESIAN_POINT ( 'NONE',  ( -1.750000000000002220, 14.46891108675447590, -27.48806413671076143 ) ) ;
#26461=EDGE_CURVE ( 'NONE', #41331, #4210, #15552, .T. ) ;
#26462=CARTESIAN_POINT ( 'NONE',  ( 3.310556943750001313, 17.50000000000002487, -133.3516058028994564 ) ) ;
#26464=CARTESIAN_POINT ( 'NONE',  ( -3.500000000000000000, 19.52072594216370405, -29.73806413671076143 ) ) ;
#26466=CARTESIAN_POINT ( 'NONE',  ( 2.340729813953370519E-16, 21.32270188528330834, -66.10160580289945642 ) ) ;
#26468=CARTESIAN_POINT ( 'NONE',  ( 3.310556943749999981, 15.58864905735836537, -67.34743913623280775 ) ) ;
#26470=CARTESIAN_POINT ( 'NONE',  ( 3.310556943750001313, 19.41135094264166838, -88.26827246956612782 ) ) ;
#26472=CARTESIAN_POINT ( 'NONE',  ( 4.648177544792955347E-16, 21.00000000000002132, -103.9047308033774186 ) ) ;
#26475=CARTESIAN_POINT ( 'NONE',  ( 3.310556943749999981, 15.58864905735836182, -46.34743913623280065 ) ) ;
#26477=CARTESIAN_POINT ( 'NONE',  ( 1.655278471875001101, 20.36702641396249192, -98.09743913623280775 ) ) ;
#26481=ORIENTED_EDGE ( 'NONE', *, *, #15248, .T. ) ;
#26486=CARTESIAN_POINT ( 'NONE',  ( -1.655278471875002211, 14.63297358603754361, -56.59743913623280065 ) ) ;
#26487=ORIENTED_EDGE ( 'NONE', *, *, #27246, .F. ) ;
#26488=ORIENTED_EDGE ( 'NONE', *, *, #14712, .F. ) ;
#26489=CYLINDRICAL_SURFACE ( 'NONE', #2210, 3.499999999999999556 ) ;
#26491=CARTESIAN_POINT ( 'NONE',  ( 3.500000000000000000, 15.47927405783632082, -31.54431413575484200 ) ) ;
#26494=CARTESIAN_POINT ( 'NONE',  ( 1.750000000000001110, 20.53108891324555785, -114.2943141357548313 ) ) ;
#26497=CARTESIAN_POINT ( 'NONE',  ( 1.750000000000001110, 20.53108891324554719, -42.29431413575483845 ) ) ;
#26498=CARTESIAN_POINT ( 'NONE',  ( 3.310556943749999981, 15.58864905735836182, -44.34743913623280065 ) ) ;
#26499=CARTESIAN_POINT ( 'NONE',  ( 3.500000000000000000, 15.47927405783631727, -23.54431413575484910 ) ) ;
#26500=CARTESIAN_POINT ( 'NONE',  ( -3.500000000000001332, 17.50000000000002132, -117.6547308033774328 ) ) ;
#26502=CARTESIAN_POINT ( 'NONE',  ( 3.310556943750001313, 17.50000000000001066, -30.35160580289947418 ) ) ;
#26504=CARTESIAN_POINT ( 'NONE',  ( -3.310556943750001313, 17.50000000000001776, -82.85160580289947063 ) ) ;
#26505=CARTESIAN_POINT ( 'NONE',  ( -7.022189441860112050E-16, 13.67729811471672718, -135.5141058028994792 ) ) ;
#26507=DIRECTION ( 'NONE',  ( 0.8660254037844367092, -0.000000000000000000, 0.5000000000000034417 ) ) ;
#26508=CARTESIAN_POINT ( 'NONE',  ( -1.394453263437886604E-15, 14.00000000000001066, -34.40473080337743284 ) ) ;
#26510=CARTESIAN_POINT ( 'NONE',  ( -3.310556943750000425, 19.41135094264166838, -127.9349391362327850 ) ) ;
#26511=CARTESIAN_POINT ( 'NONE',  ( 4.648177544792955347E-16, 21.00000000000001421, -69.21098080242148853 ) ) ;
#26512=CARTESIAN_POINT ( 'NONE',  ( -3.310556943750000425, 19.41135094264166483, -85.84743913623279354 ) ) ;
#26513=CARTESIAN_POINT ( 'NONE',  ( 4.286263797015737581E-16, 14.00000000000002487, -149.5231586289125687 ) ) ;
#26515=CARTESIAN_POINT ( 'NONE',  ( 3.500000000000001332, 19.52072594216371826, -126.3776474690881599 ) ) ;
#26516=CARTESIAN_POINT ( 'NONE',  ( 3.500000000000001332, 17.50000000000001776, -77.15473080337741862 ) ) ;
#26517=CARTESIAN_POINT ( 'NONE',  ( -3.310556943750001313, 17.50000000000001421, -59.85160580289947063 ) ) ;
#26521=CARTESIAN_POINT ( 'NONE',  ( -3.310556943750001313, 17.50000000000001776, -81.85160580289945642 ) ) ;
#26522=DIRECTION ( 'NONE',  ( 0.000000000000000000, 1.000000000000000000, 0.000000000000000000 ) ) ;
#26524=CARTESIAN_POINT ( 'NONE',  ( -3.310556943750001313, 17.50000000000002132, -110.7641058028994649 ) ) ;
#26525=CARTESIAN_POINT ( 'NONE',  ( 1.655278471875001101, 20.36702641396249192, -81.09743913623280775 ) ) ;
#26526=CARTESIAN_POINT ( 'NONE',  ( 7.785697387528201340E-15, 14.00000000000002487, -138.7109808024215170 ) ) ;
#26527=ORIENTED_EDGE ( 'NONE', *, *, #39617, .F. ) ;
#26529=CARTESIAN_POINT ( 'NONE',  ( 3.310556943749999981, 15.58864905735837070, -100.4349391362327992 ) ) ;
#26530=CARTESIAN_POINT ( 'NONE',  ( 3.500000000000001332, 17.50000000000002132, -103.1547308033774186 ) ) ;
#26533=CARTESIAN_POINT ( 'NONE',  ( -3.500000000000002220, 15.47927405783632082, -37.87764746908817415 ) ) ;
#26537=CARTESIAN_POINT ( 'NONE',  ( 3.310556943750001313, 17.50000000000001421, -60.26410580289947916 ) ) ;
#26538=CARTESIAN_POINT ( 'NONE',  ( -3.310556943750002645, 15.58864905735837780, -114.6807724695661364 ) ) ;
#26540=( BOUNDED_CURVE ( )  B_SPLINE_CURVE ( 2, ( #35619, #19453, #23054, #26464, #39418, #22222, #24403, #24206, #40764 ),
 .UNSPECIFIED., .F., .T. ) 
 B_SPLINE_CURVE_WITH_KNOTS ( ( 3, 2, 2, 2, 3 ),
 ( 0.9437499999999999778, 0.9444444444444444198, 0.9458333333333333037, 0.9472222222222221877, 0.9479166666666666297 ),
 .UNSPECIFIED. ) 
 CURVE ( )  GEOMETRIC_REPRESENTATION_ITEM ( )  RATIONAL_B_SPLINE_CURVE ( ( 0.9330127018922194093, 0.9330127018922194093, 1.000000000000000000, 0.8660254037844387076, 1.000000000000000000, 0.8660254037844387076, 1.000000000000000000, 0.9330127018922194093, 0.9330127018922194093 ) ) 
 REPRESENTATION_ITEM ( '' )  );
#26546=CARTESIAN_POINT ( 'NONE',  ( 1.655278471874998436, 14.63297358603754361, -72.43077246956613635 ) ) ;
#26553=CARTESIAN_POINT ( 'NONE',  ( 1.655278471874998436, 14.63297358603755072, -133.4307724695661364 ) ) ;
#26556=CARTESIAN_POINT ( 'NONE',  ( -7.022189441860112050E-16, 13.67729811471671475, -35.60160580289946353 ) ) ;
#26557=CARTESIAN_POINT ( 'NONE',  ( -3.310556943750001313, 17.50000000000001776, -99.85160580289947063 ) ) ;
#26559=CARTESIAN_POINT ( 'NONE',  ( -1.655278471875002211, 14.63297358603753828, -24.59743913623281486 ) ) ;
#26561=CARTESIAN_POINT ( 'NONE',  ( 2.474675557024783212E-16, 21.54145188432740099, -104.2109808024215027 ) ) ;
#26564=CARTESIAN_POINT ( 'NONE',  ( -3.500000000000000888, 19.52072594216371115, -90.73806413671074722 ) ) ;
#26568=CARTESIAN_POINT ( 'NONE',  ( -1.750000000000002220, 14.46891108675447946, -54.79431413575484555 ) ) ;
#26570=CARTESIAN_POINT ( 'NONE',  ( 4.648177544792955347E-16, 21.00000000000001776, -95.21098080242150274 ) ) ;
#26571=ORIENTED_EDGE ( 'NONE', *, *, #31176, .T. ) ;
#26572=CARTESIAN_POINT ( 'NONE',  ( 2.474675557024783212E-16, 21.54145188432739033, -43.90473080337743284 ) ) ;
#26574=CARTESIAN_POINT ( 'NONE',  ( 3.310556943749999981, 15.58864905735836004, -25.43493913623279212 ) ) ;
#26576=CYLINDRICAL_SURFACE ( 'NONE', #6372, 3.499999999999999556 ) ;
#26577=CARTESIAN_POINT ( 'NONE',  ( -0.9378221735089291577, 21.00000000000001421, -60.86007260463890134 ) ) ;
#26580=CARTESIAN_POINT ( 'NONE',  ( 3.500000000000000000, 15.47927405783632082, -36.23806413671076854 ) ) ;
#26582=CARTESIAN_POINT ( 'NONE',  ( 3.310556943750001313, 17.50000000000001776, -75.26410580289947916 ) ) ;
#26583=LINE ( 'NONE', #12976, #3253 ) ;
#26585=CARTESIAN_POINT ( 'NONE',  ( 0.000000000000000000, 21.00000000000002487, -149.5231586289125687 ) ) ;
#26587=ORIENTED_EDGE ( 'NONE', *, *, #6396, .T. ) ;
#26588=CARTESIAN_POINT ( 'NONE',  ( 0.000000000000000000, 17.50000000000002487, -149.5231586289125687 ) ) ;
#26589=CARTESIAN_POINT ( 'NONE',  ( 3.310556943750001313, 19.41135094264166483, -91.18077246956613635 ) ) ;
#26592=ORIENTED_EDGE ( 'NONE', *, *, #25133, .F. ) ;
#26595=CYLINDRICAL_SURFACE ( 'NONE', #2241, 3.499999999999999556 ) ;
#26596=CARTESIAN_POINT ( 'NONE',  ( -7.022189441860112050E-16, 13.67729811471672718, -124.5141058028994649 ) ) ;
#26599=CARTESIAN_POINT ( 'NONE',  ( 2.340729813953370519E-16, 21.32270188528330834, -53.10160580289946353 ) ) ;
#26600=CARTESIAN_POINT ( 'NONE',  ( 3.310556943750001313, 17.50000000000002132, -118.3516058028994706 ) ) ;
#26601=EDGE_LOOP ( 'NONE', ( #38613, #17540, #37427, #33015 ) ) ;
#26602=( BOUNDED_CURVE ( )  B_SPLINE_CURVE ( 2, ( #13883, #17076, #33869, #27073, #33670, #17503, #39833, #36641, #26862 ),
 .UNSPECIFIED., .F., .T. ) 
 B_SPLINE_CURVE_WITH_KNOTS ( ( 3, 2, 2, 2, 3 ),
 ( 0.04791666666666666990, 0.04861111111111111188, 0.05000000000000000278, 0.05138888888888888673, 0.05208333333333333565 ),
 .UNSPECIFIED. ) 
 CURVE ( )  GEOMETRIC_REPRESENTATION_ITEM ( )  RATIONAL_B_SPLINE_CURVE ( ( 0.9330127018922192983, 0.9330127018922196314, 1.000000000000000000, 0.8660254037844387076, 1.000000000000000000, 0.8660254037844387076, 1.000000000000000000, 0.9330127018922189652, 0.9330127018922192983 ) ) 
 REPRESENTATION_ITEM ( '' )  );
#26603=ORIENTED_EDGE ( 'NONE', *, *, #37825, .T. ) ;
#26604=CARTESIAN_POINT ( 'NONE',  ( 1.750000000000001110, 20.53108891324555785, -123.9880641367107614 ) ) ;
#26605=CARTESIAN_POINT ( 'NONE',  ( 3.310556943749999981, 15.58864905735836182, -37.34743913623281486 ) ) ;
#26606=CARTESIAN_POINT ( 'NONE',  ( 1.655278471874998436, 14.63297358603754361, -73.51827246956612782 ) ) ;
#26607=CARTESIAN_POINT ( 'NONE',  ( 3.500000000000001332, 17.50000000000002132, -116.4609808024215170 ) ) ;
#26608=CARTESIAN_POINT ( 'NONE',  ( 3.310556943749999981, 15.58864905735837070, -103.3474391362328220 ) ) ;
#26611=CARTESIAN_POINT ( 'NONE',  ( 7.367361408496833051E-14, 14.00000000000001776, -93.40473080337741862 ) ) ;
#26613=CARTESIAN_POINT ( 'NONE',  ( -1.750000000000002220, 14.46891108675448123, -67.79431413575484555 ) ) ;
#26614=CARTESIAN_POINT ( 'NONE',  ( -1.394453263437886604E-15, 14.00000000000002132, -122.7109808024214885 ) ) ;
#26615=CARTESIAN_POINT ( 'NONE',  ( -7.022189441860112050E-16, 13.67729811471671475, -35.51410580289947205 ) ) ;
#26616=CARTESIAN_POINT ( 'NONE',  ( -3.310556943750000425, 19.41135094264166483, -97.93493913623278502 ) ) ;
#26617=CARTESIAN_POINT ( 'NONE',  ( 1.750000000000001110, 20.53108891324555074, -60.98806413671076143 ) ) ;
#26618=CARTESIAN_POINT ( 'NONE',  ( -1.394453263437886604E-15, 14.00000000000001421, -77.40473080337740441 ) ) ;
#26619=CARTESIAN_POINT ( 'NONE',  ( 3.310556943750001313, 17.50000000000002132, -111.3516058028994564 ) ) ;
#26620=CARTESIAN_POINT ( 'NONE',  ( -3.310556943750002201, 15.58864905735836714, -43.76827246956613493 ) ) ;
#26622=CARTESIAN_POINT ( 'NONE',  ( -8.715332896486792803E-15, 21.00000000000002842, -137.9047308033774186 ) ) ;
#26626=CARTESIAN_POINT ( 'NONE',  ( -3.500000000000001332, 17.50000000000001066, -23.65473080337743284 ) ) ;
#26627=CARTESIAN_POINT ( 'NONE',  ( -7.022189441860112050E-16, 13.67729811471672363, -92.51410580289947916 ) ) ;
#26630=DIRECTION ( 'NONE',  ( -0.000000000000000000, 1.259100132267607459E-16, -1.000000000000000000 ) ) ;
#26632=CARTESIAN_POINT ( 'NONE',  ( 1.749999999999998224, 14.46891108675448656, -123.3213974700441042 ) ) ;
#26637=CARTESIAN_POINT ( 'NONE',  ( -7.022189441860112050E-16, 13.67729811471671653, -27.51410580289948271 ) ) ;
#26638=ORIENTED_EDGE ( 'NONE', *, *, #26271, .F. ) ;
#26639=EDGE_CURVE ( 'NONE', #31756, #5090, #5900, .T. ) ;
#26640=CARTESIAN_POINT ( 'NONE',  ( -3.500000000000000000, 19.52072594216371826, -109.7380641367107614 ) ) ;
#26646=ORIENTED_EDGE ( 'NONE', *, *, #37306, .T. ) ;
#26647=CARTESIAN_POINT ( 'NONE',  ( 1.749999999999998224, 14.46891108675448656, -135.3213974700441042 ) ) ;
#26649=CARTESIAN_POINT ( 'NONE',  ( 3.310556943750001313, 17.50000000000002487, -143.2641058028994792 ) ) ;
#26652=CARTESIAN_POINT ( 'NONE',  ( -3.500000000000001332, 17.50000000000002487, -135.9609808024214885 ) ) ;
#26653=CARTESIAN_POINT ( 'NONE',  ( -3.310556943750001313, 17.50000000000002487, -134.8516058028994564 ) ) ;
#26654=CARTESIAN_POINT ( 'NONE',  ( -1.749999999999999778, 20.53108891324554719, -29.12764746908817770 ) ) ;
#26656=CARTESIAN_POINT ( 'NONE',  ( 3.500000000000001332, 17.50000000000002487, -142.1547308033774186 ) ) ;
#26658=CARTESIAN_POINT ( 'NONE',  ( 1.750000000000001110, 20.53108891324556140, -136.2943141357548598 ) ) ;
#26659=CARTESIAN_POINT ( 'NONE',  ( -7.022189441860112050E-16, 13.67729811471672718, -119.5141058028994934 ) ) ;
#26663=CARTESIAN_POINT ( 'NONE',  ( 3.500000000000001332, 17.50000000000001776, -84.46098080242150274 ) ) ;
#26665=CARTESIAN_POINT ( 'NONE',  ( 2.340729813953370519E-16, 21.32270188528330834, -54.01410580289947916 ) ) ;
#26667=CARTESIAN_POINT ( 'NONE',  ( 1.655278471874998436, 14.63297358603754894, -110.5182724695661420 ) ) ;
#26669=CARTESIAN_POINT ( 'NONE',  ( 3.500000000000000000, 15.47927405783632082, -27.23806413671076143 ) ) ;
#26672=CARTESIAN_POINT ( 'NONE',  ( 3.310556943750001313, 17.50000000000002132, -129.3516058028994564 ) ) ;
#26675=CARTESIAN_POINT ( 'NONE',  ( -1.394453263437886604E-15, 14.00000000000001421, -58.71098080242150985 ) ) ;
#26676=CARTESIAN_POINT ( 'NONE',  ( 2.340729813953370519E-16, 21.32270188528330834, -65.10160580289947063 ) ) ;
#26678=CARTESIAN_POINT ( 'NONE',  ( 2.340729813953370519E-16, 21.32270188528330834, -62.01410580289947205 ) ) ;
#26680=CARTESIAN_POINT ( 'NONE',  ( 1.655278471875001101, 20.36702641396249192, -88.18493913623279923 ) ) ;
#26682=CARTESIAN_POINT ( 'NONE',  ( 1.750000000000001110, 20.53108891324554719, -44.29431413575483845 ) ) ;
#26684=CARTESIAN_POINT ( 'NONE',  ( -1.394453263437886604E-15, 14.00000000000001421, -54.71098080242150985 ) ) ;
#26685=VECTOR ( 'NONE', #23863, 1000.000000000000000 ) ;
#26687=CARTESIAN_POINT ( 'NONE',  ( -7.022189441860112050E-16, 13.67729811471671830, -43.51410580289947916 ) ) ;
#26688=AXIS2_PLACEMENT_3D ( 'NONE', #22877, #35843, #20102 ) ;
#26690=CARTESIAN_POINT ( 'NONE',  ( -1.394453263437886604E-15, 14.00000000000001776, -98.40473080337743284 ) ) ;
#26695=CARTESIAN_POINT ( 'NONE',  ( -3.310556943750000425, 19.41135094264166128, -53.84743913623281486 ) ) ;
#26697=ORIENTED_EDGE ( 'NONE', *, *, #4550, .F. ) ;
#26698=DIRECTION ( 'NONE',  ( 0.000000000000000000, 1.000000000000000000, 0.000000000000000000 ) ) ;
#26699=CARTESIAN_POINT ( 'NONE',  ( -0.9378221735088960731, 14.00000000000000000, -95.75563900116003424 ) ) ;
#26701=CARTESIAN_POINT ( 'NONE',  ( 0.9378221735089281585, 14.00000000000002132, -113.6663226036829997 ) ) ;
#26703=ORIENTED_EDGE ( 'NONE', *, *, #20638, .T. ) ;
#26705=CARTESIAN_POINT ( 'NONE',  ( -1.749999999999999778, 20.53108891324554719, -45.12764746908818125 ) ) ;
#26706=CARTESIAN_POINT ( 'NONE',  ( -3.310556943750001313, 17.50000000000001066, -42.76410580289947916 ) ) ;
#26707=CARTESIAN_POINT ( 'NONE',  ( 4.648177544792955347E-16, 21.00000000000002132, -108.2109808024215170 ) ) ;
#26708=CARTESIAN_POINT ( 'NONE',  ( -0.9378221735089310451, 14.00000000000002309, -133.4493890021159359 ) ) ;
#26709=CARTESIAN_POINT ( 'NONE',  ( 3.500000000000001332, 17.50000000000001776, -94.46098080242151696 ) ) ;
#26711=CARTESIAN_POINT ( 'NONE',  ( 1.655278471875001101, 20.36702641396248481, -32.18493913623279923 ) ) ;
#26712=CARTESIAN_POINT ( 'NONE',  ( 2.340729813953370519E-16, 21.32270188528330479, -25.10160580289946708 ) ) ;
#26714=CARTESIAN_POINT ( 'NONE',  ( 3.310556943750001313, 19.41135094264166483, -84.26827246956612782 ) ) ;
#26715=CARTESIAN_POINT ( 'NONE',  ( -3.310556943750001313, 17.50000000000002487, -132.7641058028994507 ) ) ;
#26722=CARTESIAN_POINT ( 'NONE',  ( 0.9378221735089300459, 21.00000000000001776, -85.25563900116002003 ) ) ;
#26723=CARTESIAN_POINT ( 'NONE',  ( 2.340729813953370519E-16, 21.32270188528332255, -130.1016058028994280 ) ) ;
#26724=CARTESIAN_POINT ( 'NONE',  ( 0.9378221735089294908, 14.00000000000002665, -141.3600726046389298 ) ) ;
#26725=CARTESIAN_POINT ( 'NONE',  ( 3.310556943750001313, 17.50000000000001776, -88.26410580289947916 ) ) ;
#26726=CARTESIAN_POINT ( 'NONE',  ( 1.750000000000001110, 20.53108891324554719, -24.29431413575484910 ) ) ;
#26727=CARTESIAN_POINT ( 'NONE',  ( 3.500000000000001332, 19.52072594216371115, -75.37764746908817415 ) ) ;
#26728=DIRECTION ( 'NONE',  ( -0.000000000000000000, 1.259100132267607459E-16, -1.000000000000000000 ) ) ;
#26729=CARTESIAN_POINT ( 'NONE',  ( 3.500000000000000000, 15.47927405783632437, -77.23806413671076143 ) ) ;
#26730=CARTESIAN_POINT ( 'NONE',  ( 3.310556943749999981, 15.58864905735836537, -60.43493913623279923 ) ) ;
#26731=( BOUNDED_CURVE ( )  B_SPLINE_CURVE ( 2, ( #6389, #17739, #11155, #21347, #20930, #4760, #30713, #40495, #40695 ),
 .UNSPECIFIED., .F., .T. ) 
 B_SPLINE_CURVE_WITH_KNOTS ( ( 3, 2, 2, 2, 3 ),
 ( 0.9395833333333333259, 0.9402777777777777679, 0.9416666666666666519, 0.9430555555555555358, 0.9437499999999999778 ),
 .UNSPECIFIED. ) 
 CURVE ( )  GEOMETRIC_REPRESENTATION_ITEM ( )  RATIONAL_B_SPLINE_CURVE ( ( 0.9330127018922194093, 0.9330127018922194093, 1.000000000000000000, 0.8660254037844387076, 1.000000000000000000, 0.8660254037844387076, 1.000000000000000000, 0.9330127018922194093, 0.9330127018922194093 ) ) 
 REPRESENTATION_ITEM ( '' )  );
#26733=CARTESIAN_POINT ( 'NONE',  ( 1.743066579297357930E-14, 14.00000000000002132, -135.4047308033774186 ) ) ;
#26735=CARTESIAN_POINT ( 'NONE',  ( -1.655278471875002211, 14.63297358603754539, -77.68493913623279923 ) ) ;
#26736=CARTESIAN_POINT ( 'NONE',  ( -3.310556943750001313, 17.50000000000002487, -140.8516058028994564 ) ) ;
#26738=CARTESIAN_POINT ( 'NONE',  ( -3.310556943750002201, 15.58864905735837425, -108.6807724695661648 ) ) ;
#26739=CARTESIAN_POINT ( 'NONE',  ( 3.310556943749999981, 15.58864905735836892, -82.34743913623280775 ) ) ;
#26740=CARTESIAN_POINT ( 'NONE',  ( 1.750000000000001110, 20.53108891324555074, -56.98806413671076143 ) ) ;
#26741=ORIENTED_EDGE ( 'NONE', *, *, #20482, .F. ) ;
#26742=CARTESIAN_POINT ( 'NONE',  ( -3.310556943750000425, 19.41135094264166838, -101.9349391362327850 ) ) ;
#26743=CARTESIAN_POINT ( 'NONE',  ( -7.424026671074350129E-16, 13.45854811567263809, -103.4047308033774328 ) ) ;
#26746=CARTESIAN_POINT ( 'NONE',  ( 0.000000000000000000, 21.00000000000002487, -149.5231586289125687 ) ) ;
#26747=CARTESIAN_POINT ( 'NONE',  ( 3.500000000000001332, 19.52072594216370405, -45.37764746908817415 ) ) ;
#26749=CARTESIAN_POINT ( 'NONE',  ( -1.655278471874999990, 20.36702641396248836, -60.93077246956614346 ) ) ;
#26750=CARTESIAN_POINT ( 'NONE',  ( 2.340729813953370519E-16, 21.32270188528331900, -117.0141058028994792 ) ) ;
#26751=CARTESIAN_POINT ( 'NONE',  ( 4.648177544792955347E-16, 21.00000000000002132, -107.2109808024215027 ) ) ;
#26757=CARTESIAN_POINT ( 'NONE',  ( 4.286263797015737581E-16, 14.00000000000002487, -149.5231586289125687 ) ) ;
#26759=CARTESIAN_POINT ( 'NONE',  ( 3.310556943750001313, 19.41135094264166128, -66.18077246956613635 ) ) ;
#26760=ORIENTED_EDGE ( 'NONE', *, *, #1068, .F. ) ;
#26761=ORIENTED_EDGE ( 'NONE', *, *, #41610, .F. ) ;
#26762=DIRECTION ( 'NONE',  ( -0.000000000000000000, 1.259100132267607459E-16, -1.000000000000000000 ) ) ;
#26766=ORIENTED_EDGE ( 'NONE', *, *, #2022, .F. ) ;
#26767=CARTESIAN_POINT ( 'NONE',  ( 3.310556943750001313, 19.41135094264167549, -137.1807724695661364 ) ) ;
#26768=DIRECTION ( 'NONE',  ( -0.000000000000000000, 1.259100132267607459E-16, -1.000000000000000000 ) ) ;
#26769=CARTESIAN_POINT ( 'NONE',  ( 3.310556943750001313, 17.50000000000001066, -44.35160580289947063 ) ) ;
#26771=CARTESIAN_POINT ( 'NONE',  ( 3.310556943750001313, 19.41135094264165772, -39.26827246956613493 ) ) ;
#26773=CARTESIAN_POINT ( 'NONE',  ( 3.310556943750001313, 17.50000000000001776, -96.35160580289945642 ) ) ;
#26775=CARTESIAN_POINT ( 'NONE',  ( -1.655278471875002211, 14.63297358603753828, -25.59743913623280065 ) ) ;
#26777=CARTESIAN_POINT ( 'NONE',  ( 0.9378221735089300459, 21.00000000000002132, -121.2556390011600485 ) ) ;
#26778=CARTESIAN_POINT ( 'NONE',  ( 3.500000000000000000, 15.47927405783632793, -100.5443141357548313 ) ) ;
#26779=CARTESIAN_POINT ( 'NONE',  ( -0.9378221735089291577, 21.00000000000001421, -73.86007260463891555 ) ) ;
#26781=CARTESIAN_POINT ( 'NONE',  ( 3.500000000000000000, 15.47927405783632615, -91.23806413671076143 ) ) ;
#26782=CARTESIAN_POINT ( 'NONE',  ( -1.394453263437886604E-15, 14.00000000000001421, -77.71098080242148853 ) ) ;
#26785=CARTESIAN_POINT ( 'NONE',  ( -3.500000000000001332, 17.50000000000002132, -119.9609808024215170 ) ) ;
#26786=CARTESIAN_POINT ( 'NONE',  ( -7.424026671074350129E-16, 13.45854811567263276, -51.71098080242150985 ) ) ;
#26787=CARTESIAN_POINT ( 'NONE',  ( -3.500000000000000000, 19.52072594216370760, -46.73806413671076143 ) ) ;
#26788=CARTESIAN_POINT ( 'NONE',  ( -1.749999999999999778, 20.53108891324556140, -134.8213974700441042 ) ) ;
#26789=( BOUNDED_CURVE ( )  B_SPLINE_CURVE ( 2, ( #23676, #24302, #36857, #8125, #21104, #7718, #4519, #17501, #30464 ),
 .UNSPECIFIED., .F., .T. ) 
 B_SPLINE_CURVE_WITH_KNOTS ( ( 3, 2, 2, 2, 3 ),
 ( 0.9604166666666666963, 0.9611111111111111382, 0.9625000000000000222, 0.9638888888888889062, 0.9645833333333333481 ),
 .UNSPECIFIED. ) 
 CURVE ( )  GEOMETRIC_REPRESENTATION_ITEM ( )  RATIONAL_B_SPLINE_CURVE ( ( 0.9330127018922194093, 0.9330127018922194093, 1.000000000000000000, 0.8660254037844387076, 1.000000000000000000, 0.8660254037844387076, 1.000000000000000000, 0.9330127018922194093, 0.9330127018922194093 ) ) 
 REPRESENTATION_ITEM ( '' )  );
#26790=VERTEX_POINT ( 'NONE', #38858 ) ;
#26791=CARTESIAN_POINT ( 'NONE',  ( -1.750000000000002220, 14.46891108675447768, -43.48806413671076143 ) ) ;
#26792=CARTESIAN_POINT ( 'NONE',  ( 4.648177544792955347E-16, 21.00000000000001421, -59.21098080242150274 ) ) ;
#26794=CARTESIAN_POINT ( 'NONE',  ( 1.655278471874998436, 14.63297358603753828, -27.51827246956613138 ) ) ;
#26795=DIRECTION ( 'NONE',  ( 0.000000000000000000, 1.000000000000000000, 0.000000000000000000 ) ) ;
#26798=CARTESIAN_POINT ( 'NONE',  ( 3.500000000000001332, 19.52072594216371826, -120.0713974700441042 ) ) ;
#26800=CARTESIAN_POINT ( 'NONE',  ( 2.340729813953370519E-16, 21.32270188528331190, -77.01410580289947916 ) ) ;
#26801=CARTESIAN_POINT ( 'NONE',  ( 0.000000000000000000, 17.50000000000002487, -149.5231586289125687 ) ) ;
#26807=CARTESIAN_POINT ( 'NONE',  ( 3.310556943749999981, 15.58864905735836892, -87.34743913623280775 ) ) ;
#26809=VERTEX_POINT ( 'NONE', #26733 ) ;
#26812=CARTESIAN_POINT ( 'NONE',  ( -1.749999999999999778, 20.53108891324555074, -59.12764746908817415 ) ) ;
#26813=CARTESIAN_POINT ( 'NONE',  ( 1.655278471875001101, 20.36702641396249547, -125.0974391362328078 ) ) ;
#26815=CARTESIAN_POINT ( 'NONE',  ( -3.310556943750001313, 17.50000000000001421, -51.85160580289946353 ) ) ;
#26817=CARTESIAN_POINT ( 'NONE',  ( -3.310556943750002645, 15.58864905735837780, -116.7682724695661278 ) ) ;
#26820=CARTESIAN_POINT ( 'NONE',  ( -3.500000000000000888, 19.52072594216371826, -125.7380641367107472 ) ) ;
#26821=CARTESIAN_POINT ( 'NONE',  ( 3.310556943750001313, 17.50000000000001066, -42.26410580289947916 ) ) ;
#26822=CARTESIAN_POINT ( 'NONE',  ( 3.310556943750001313, 17.50000000000001421, -65.35160580289945642 ) ) ;
#26823=CARTESIAN_POINT ( 'NONE',  ( 3.500000000000001332, 17.50000000000002132, -117.4609808024215170 ) ) ;
#26824=CARTESIAN_POINT ( 'NONE',  ( 3.310556943750001313, 19.41135094264166838, -103.1807724695661506 ) ) ;
#26825=CARTESIAN_POINT ( 'NONE',  ( 4.648177544792955347E-16, 21.00000000000001066, -44.90473080337743284 ) ) ;
#26828=CARTESIAN_POINT ( 'NONE',  ( -3.500000000000001332, 17.50000000000001421, -71.96098080242151696 ) ) ;
#26829=CARTESIAN_POINT ( 'NONE',  ( -1.394453263437886604E-15, 14.00000000000001066, -26.71098080242150985 ) ) ;
#26830=CARTESIAN_POINT ( 'NONE',  ( -7.022189441860112050E-16, 13.67729811471671475, -38.51410580289947916 ) ) ;
#26831=CARTESIAN_POINT ( 'NONE',  ( 3.310556943749999981, 15.58864905735836892, -94.43493913623279923 ) ) ;
#26832=CARTESIAN_POINT ( 'NONE',  ( 3.500000000000001776, 19.52072594216370760, -59.07139747004410424 ) ) ;
#26833=CARTESIAN_POINT ( 'NONE',  ( 3.310556943749999981, 15.58864905735837247, -113.4349391362327992 ) ) ;
#26834=CARTESIAN_POINT ( 'NONE',  ( 3.310556943750001313, 19.41135094264166128, -41.26827246956612072 ) ) ;
#26836=CARTESIAN_POINT ( 'NONE',  ( -1.394453263437886604E-15, 14.00000000000001421, -60.71098080242150985 ) ) ;
#26840=DIRECTION ( 'NONE',  ( 0.000000000000000000, 1.000000000000000000, 0.000000000000000000 ) ) ;
#26841=CARTESIAN_POINT ( 'NONE',  ( 1.655278471875001101, 20.36702641396249192, -94.09743913623280775 ) ) ;
#26842=CARTESIAN_POINT ( 'NONE',  ( -3.500000000000002220, 15.47927405783632082, -36.57139747004409003 ) ) ;
#26846=CARTESIAN_POINT ( 'NONE',  ( -1.394453263437886604E-15, 14.00000000000001421, -69.40473080337741862 ) ) ;
#26848=VECTOR ( 'NONE', #29849, 1000.000000000000000 ) ;
#26849=CARTESIAN_POINT ( 'NONE',  ( 4.648177544792955347E-16, 21.00000000000002132, -112.9047308033774186 ) ) ;
#26850=ORIENTED_EDGE ( 'NONE', *, *, #37381, .T. ) ;
#26853=CARTESIAN_POINT ( 'NONE',  ( -3.310556943750002201, 15.58864905735836537, -30.68077246956614346 ) ) ;
#26854=ORIENTED_EDGE ( 'NONE', *, *, #476, .T. ) ;
#26855=CARTESIAN_POINT ( 'NONE',  ( -1.394453263437886604E-15, 14.00000000000002132, -123.4047308033774044 ) ) ;
#26862=CARTESIAN_POINT ( 'NONE',  ( -8.715332896486792803E-15, 21.00000000000002842, -136.9047308033774470 ) ) ;
#26863=CARTESIAN_POINT ( 'NONE',  ( -1.394453263437886604E-15, 14.00000000000001421, -80.71098080242148853 ) ) ;
#26864=DIRECTION ( 'NONE',  ( -0.000000000000000000, 1.259100132267607459E-16, -1.000000000000000000 ) ) ;
#26865=CARTESIAN_POINT ( 'NONE',  ( -1.655278471875002211, 14.63297358603755249, -131.6849391362327992 ) ) ;
#26866=CARTESIAN_POINT ( 'NONE',  ( 1.750000000000001110, 20.53108891324554719, -27.29431413575483845 ) ) ;
#26868=CARTESIAN_POINT ( 'NONE',  ( 1.750000000000001110, 20.53108891324556140, -141.9880641367107614 ) ) ;
#26872=CARTESIAN_POINT ( 'NONE',  ( 1.750000000000001110, 20.53108891324556140, -133.2943141357548598 ) ) ;
#26873=CARTESIAN_POINT ( 'NONE',  ( 1.655278471875001101, 20.36702641396249547, -117.0974391362327935 ) ) ;
#26875=EDGE_CURVE ( 'NONE', #12093, #39830, #561, .T. ) ;
#26877=CARTESIAN_POINT ( 'NONE',  ( 1.749999999999998224, 14.46891108675448123, -83.62764746908818836 ) ) ;
#26878=DIRECTION ( 'NONE',  ( -0.000000000000000000, 1.259100132267607459E-16, -1.000000000000000000 ) ) ;
#26879=CARTESIAN_POINT ( 'NONE',  ( -1.655278471875002211, 14.63297358603754361, -54.59743913623281486 ) ) ;
#26880=CARTESIAN_POINT ( 'NONE',  ( -1.655278471874999990, 20.36702641396249547, -113.0182724695661278 ) ) ;
#26882=CARTESIAN_POINT ( 'NONE',  ( 3.500000000000001332, 19.52072594216370405, -38.37764746908817415 ) ) ;
#26883=CARTESIAN_POINT ( 'NONE',  ( 3.500000000000000000, 15.47927405783632082, -28.23806413671076143 ) ) ;
#26886=CARTESIAN_POINT ( 'NONE',  ( 3.310556943750001313, 17.50000000000002132, -127.3516058028994422 ) ) ;
#26889=CARTESIAN_POINT ( 'NONE',  ( 3.500000000000001332, 17.50000000000001776, -86.15473080337743284 ) ) ;
#26890=CARTESIAN_POINT ( 'NONE',  ( -3.310556943750001313, 17.50000000000001421, -62.85160580289946353 ) ) ;
#26893=CARTESIAN_POINT ( 'NONE',  ( -1.655278471874999990, 20.36702641396249192, -81.01827246956614204 ) ) ;
#26896=CYLINDRICAL_SURFACE ( 'NONE', #18614, 3.499999999999999556 ) ;
#26898=CARTESIAN_POINT ( 'NONE',  ( 3.310556943750001313, 19.41135094264166483, -47.18077246956614346 ) ) ;
#26900=CARTESIAN_POINT ( 'NONE',  ( -1.655278471875002211, 14.63297358603754894, -100.5974391362328078 ) ) ;
#26901=CARTESIAN_POINT ( 'NONE',  ( 3.500000000000001332, 19.52072594216370405, -42.07139747004409713 ) ) ;
#26902=( BOUNDED_CURVE ( )  B_SPLINE_CURVE ( 2, ( #21108, #24105, #1545, #30680, #27900, #24307, #5351, #1754, #8753 ),
 .UNSPECIFIED., .F., .F. ) 
 B_SPLINE_CURVE_WITH_KNOTS ( ( 3, 2, 2, 2, 3 ),
 ( 0.9687500000000000000, 0.9694444444444444420, 0.9708333333333333259, 0.9722222222222222099, 0.9729166666666666519 ),
 .UNSPECIFIED. ) 
 CURVE ( )  GEOMETRIC_REPRESENTATION_ITEM ( )  RATIONAL_B_SPLINE_CURVE ( ( 0.9330127018922194093, 0.9330127018922194093, 1.000000000000000000, 0.8660254037844387076, 1.000000000000000000, 0.8660254037844387076, 1.000000000000000000, 0.9330127018922194093, 0.9330127018922194093 ) ) 
 REPRESENTATION_ITEM ( '' )  );
#26903=ORIENTED_EDGE ( 'NONE', *, *, #31200, .F. ) ;
#26906=ORIENTED_EDGE ( 'NONE', *, *, #21673, .F. ) ;
#26908=CARTESIAN_POINT ( 'NONE',  ( -1.655278471874999990, 20.36702641396248836, -52.93077246956613635 ) ) ;
#26909=EDGE_CURVE ( 'NONE', #3024, #10427, #22904, .T. ) ;
#26910=ORIENTED_EDGE ( 'NONE', *, *, #28215, .T. ) ;
#26912=CARTESIAN_POINT ( 'NONE',  ( 4.648177544792955347E-16, 21.00000000000001776, -93.21098080242150274 ) ) ;
#26916=DIRECTION ( 'NONE',  ( -0.000000000000000000, 1.259100132267607459E-16, -1.000000000000000000 ) ) ;
#26918=VERTEX_POINT ( 'NONE', #352 ) ;
#26920=CARTESIAN_POINT ( 'NONE',  ( -3.500000000000002220, 15.47927405783632260, -42.87764746908817415 ) ) ;
#26921=CARTESIAN_POINT ( 'NONE',  ( -1.749999999999999778, 20.53108891324556140, -133.8213974700441042 ) ) ;
#26922=CARTESIAN_POINT ( 'NONE',  ( 3.500000000000001332, 17.50000000000002132, -119.1547308033774328 ) ) ;
#26924=CARTESIAN_POINT ( 'NONE',  ( 1.655278471874998436, 14.63297358603753828, -29.51827246956613493 ) ) ;
#26926=CARTESIAN_POINT ( 'NONE',  ( -3.310556943750002645, 15.58864905735837247, -81.76827246956614204 ) ) ;
#26927=CARTESIAN_POINT ( 'NONE',  ( 2.340729813953370519E-16, 21.32270188528332255, -135.0141058028994507 ) ) ;
#26930=CARTESIAN_POINT ( 'NONE',  ( 4.648177544792955347E-16, 21.00000000000001066, -38.90473080337743284 ) ) ;
#26932=CARTESIAN_POINT ( 'NONE',  ( -3.310556943750000425, 19.41135094264166838, -126.9349391362328134 ) ) ;
#26933=ADVANCED_FACE ( 'NONE', ( #13330 ), #39260, .T. ) ;
#26934=AXIS2_PLACEMENT_3D ( 'NONE', #18850, #2685, #21830 ) ;
#26935=LINE ( 'NONE', #20545, #35683 ) ;
#26936=CARTESIAN_POINT ( 'NONE',  ( 1.655278471874998436, 14.63297358603754539, -88.43077246956613635 ) ) ;
#26938=CARTESIAN_POINT ( 'NONE',  ( 0.9378221735088952959, 21.00000000000003908, -100.9493890021159643 ) ) ;
#26939=CARTESIAN_POINT ( 'NONE',  ( -1.394453263437886604E-15, 14.00000000000000711, -25.40473080337742928 ) ) ;
#26940=CARTESIAN_POINT ( 'NONE',  ( 3.500000000000001332, 17.50000000000001421, -72.15473080337743284 ) ) ;
#26941=CARTESIAN_POINT ( 'NONE',  ( 2.340729813953370519E-16, 21.32270188528331190, -52.10160580289946353 ) ) ;
#26943=CARTESIAN_POINT ( 'NONE',  ( 7.785697387528201340E-15, 14.00000000000002487, -137.7109808024215170 ) ) ;
#26945=CARTESIAN_POINT ( 'NONE',  ( -1.655278471875002211, 14.63297358603754716, -81.68493913623279923 ) ) ;
#26946=CARTESIAN_POINT ( 'NONE',  ( 3.310556943750001313, 19.41135094264167549, -138.2682724695661420 ) ) ;
#26948=CARTESIAN_POINT ( 'NONE',  ( 1.655278471874998436, 14.63297358603754716, -107.4307724695661506 ) ) ;
#26949=CARTESIAN_POINT ( 'NONE',  ( 1.655278471874998436, 14.63297358603754361, -76.43077246956615056 ) ) ;
#26950=CARTESIAN_POINT ( 'NONE',  ( -1.749999999999999778, 20.53108891324555785, -115.8213974700440900 ) ) ;
#26951=ORIENTED_EDGE ( 'NONE', *, *, #24369, .T. ) ;
#26952=CARTESIAN_POINT ( 'NONE',  ( 3.310556943750001313, 19.41135094264166838, -98.26827246956612782 ) ) ;
#26953=CARTESIAN_POINT ( 'NONE',  ( -7.424026671074350129E-16, 13.45854811567263809, -100.4047308033774470 ) ) ;
#26956=CARTESIAN_POINT ( 'NONE',  ( 3.500000000000000000, 15.47927405783632082, -51.23806413671076854 ) ) ;
#26958=CARTESIAN_POINT ( 'NONE',  ( -3.310556943750000425, 19.41135094264166483, -60.84743913623280775 ) ) ;
#26959=CARTESIAN_POINT ( 'NONE',  ( -0.9378221735089291577, 21.00000000000001421, -68.86007260463890134 ) ) ;
#26960=CARTESIAN_POINT ( 'NONE',  ( 1.655278471874998436, 14.63297358603754894, -117.4307724695661364 ) ) ;
#26962=ORIENTED_EDGE ( 'NONE', *, *, #22215, .T. ) ;
#26963=ORIENTED_EDGE ( 'NONE', *, *, #12203, .T. ) ;
#26967=CARTESIAN_POINT ( 'NONE',  ( -7.022189441860112050E-16, 13.67729811471671830, -66.51410580289947916 ) ) ;
#26971=CARTESIAN_POINT ( 'NONE',  ( -3.500000000000001332, 17.50000000000001776, -86.96098080242151696 ) ) ;
#26972=CARTESIAN_POINT ( 'NONE',  ( 3.500000000000000000, 15.47927405783632793, -83.54431413575483134 ) ) ;
#26973=ADVANCED_FACE ( 'NONE', ( #1824 ), #17370, .T. ) ;
#26976=ORIENTED_EDGE ( 'NONE', *, *, #10529, .T. ) ;
#26977=CARTESIAN_POINT ( 'NONE',  ( -3.310556943750000425, 19.41135094264167549, -137.8474391362328220 ) ) ;
#26979=CARTESIAN_POINT ( 'NONE',  ( -1.655278471875002211, 14.63297358603754184, -47.68493913623279923 ) ) ;
#26980=CARTESIAN_POINT ( 'NONE',  ( 3.310556943750001313, 19.41135094264165772, -37.26827246956612072 ) ) ;
#26981=CARTESIAN_POINT ( 'NONE',  ( -3.310556943750002645, 15.58864905735837425, -100.7682724695661278 ) ) ;
#26982=( BOUNDED_CURVE ( )  B_SPLINE_CURVE ( 2, ( #13429, #18986, #41750, #12606, #25587, #7696, #7272, #16843, #39811 ),
 .UNSPECIFIED., .F., .F. ) 
 B_SPLINE_CURVE_WITH_KNOTS ( ( 3, 2, 2, 2, 3 ),
 ( 0.2979166666666666630, 0.2986111111111111049, 0.2999999999999999889, 0.3013888888888888729, 0.3020833333333333148 ),
 .UNSPECIFIED. ) 
 CURVE ( )  GEOMETRIC_REPRESENTATION_ITEM ( )  RATIONAL_B_SPLINE_CURVE ( ( 0.9330127018922194093, 0.9330127018922194093, 1.000000000000000000, 0.8660254037844387076, 1.000000000000000000, 0.8660254037844387076, 1.000000000000000000, 0.9330127018922194093, 0.9330127018922194093 ) ) 
 REPRESENTATION_ITEM ( '' )  );
#26984=CARTESIAN_POINT ( 'NONE',  ( 1.655278471875001101, 20.36702641396249902, -143.1849391362327992 ) ) ;
#26986=CARTESIAN_POINT ( 'NONE',  ( 3.500000000000001332, 17.50000000000002132, -103.4609808024215027 ) ) ;
#26987=CARTESIAN_POINT ( 'NONE',  ( 4.286263797015737581E-16, 14.00000000000002487, -149.5231586289125687 ) ) ;
#26989=CARTESIAN_POINT ( 'NONE',  ( 2.474675557024783212E-16, 21.54145188432739744, -89.90473080337744705 ) ) ;
#26990=CARTESIAN_POINT ( 'NONE',  ( 3.310556943750001313, 17.50000000000001421, -68.35160580289947063 ) ) ;
#26992=CARTESIAN_POINT ( 'NONE',  ( 4.648177544792955347E-16, 21.00000000000002132, -111.9047308033774186 ) ) ;
#26994=CARTESIAN_POINT ( 'NONE',  ( 1.750000000000001110, 20.53108891324555074, -53.29431413575484555 ) ) ;
#26995=CARTESIAN_POINT ( 'NONE',  ( -1.394453263437886604E-15, 14.00000000000001421, -73.71098080242150274 ) ) ;
#26996=LINE ( 'NONE', #24644, #9524 ) ;
#26997=CARTESIAN_POINT ( 'NONE',  ( 4.648177544792955347E-16, 21.00000000000001776, -95.21098080242150274 ) ) ;
#27000=CARTESIAN_POINT ( 'NONE',  ( 3.500000000000001332, 17.50000000000001066, -45.15473080337743994 ) ) ;
#27003=CARTESIAN_POINT ( 'NONE',  ( -3.310556943750001313, 17.50000000000001066, -26.85160580289947063 ) ) ;
#27004=CARTESIAN_POINT ( 'NONE',  ( 1.750000000000001110, 20.53108891324555429, -74.98806413671076143 ) ) ;
#27007=CARTESIAN_POINT ( 'NONE',  ( 4.648177544792955347E-16, 21.00000000000001066, -35.90473080337743284 ) ) ;
#27009=CARTESIAN_POINT ( 'NONE',  ( 1.655278471875001101, 20.36702641396249192, -78.09743913623280775 ) ) ;
#27010=CARTESIAN_POINT ( 'NONE',  ( 4.648177544792955347E-16, 21.00000000000002132, -115.9047308033774328 ) ) ;
#27011=ORIENTED_EDGE ( 'NONE', *, *, #7387, .T. ) ;
#27013=CARTESIAN_POINT ( 'NONE',  ( -3.500000000000002220, 15.47927405783632437, -44.87764746908817415 ) ) ;
#27015=EDGE_CURVE ( 'NONE', #31391, #37632, #41389, .T. ) ;
#27016=CARTESIAN_POINT ( 'NONE',  ( 0.9378221735089281585, 14.00000000000001776, -88.66632260368298546 ) ) ;
#27017=CARTESIAN_POINT ( 'NONE',  ( -7.022189441860112050E-16, 13.67729811471672363, -86.51410580289947916 ) ) ;
#27018=EDGE_LOOP ( 'NONE', ( #8017, #7969, #19563, #34742 ) ) ;
#27019=VERTEX_POINT ( 'NONE', #30967 ) ;
#27023=CARTESIAN_POINT ( 'NONE',  ( -1.655278471875002211, 14.63297358603755249, -128.5974391362328220 ) ) ;
#27024=ORIENTED_EDGE ( 'NONE', *, *, #37825, .F. ) ;
#27026=CARTESIAN_POINT ( 'NONE',  ( 1.655278471875001101, 20.36702641396248836, -55.18493913623280633 ) ) ;
#27027=CARTESIAN_POINT ( 'NONE',  ( 3.310556943749999981, 15.58864905735837247, -112.4349391362327992 ) ) ;
#27028=ORIENTED_EDGE ( 'NONE', *, *, #18651, .F. ) ;
#27029=VERTEX_POINT ( 'NONE', #20340 ) ;
#27030=CARTESIAN_POINT ( 'NONE',  ( -3.500000000000000888, 19.52072594216371826, -123.7380641367107614 ) ) ;
#27031=( BOUNDED_CURVE ( )  B_SPLINE_CURVE ( 2, ( #6008, #36180, #13428, #20031, #9843, #26002, #32779, #3645, #10244 ),
 .UNSPECIFIED., .F., .T. ) 
 B_SPLINE_CURVE_WITH_KNOTS ( ( 3, 2, 2, 2, 3 ),
 ( 0.5312500000000000000, 0.5319444444444444420, 0.5333333333333333259, 0.5347222222222222099, 0.5354166666666666519 ),
 .UNSPECIFIED. ) 
 CURVE ( )  GEOMETRIC_REPRESENTATION_ITEM ( )  RATIONAL_B_SPLINE_CURVE ( ( 0.9330127018922194093, 0.9330127018922194093, 1.000000000000000000, 0.8660254037844387076, 1.000000000000000000, 0.8660254037844387076, 1.000000000000000000, 0.9330127018922194093, 0.9330127018922194093 ) ) 
 REPRESENTATION_ITEM ( '' )  );
#27032=CARTESIAN_POINT ( 'NONE',  ( 3.310556943750001313, 19.41135094264165772, -41.18077246956613635 ) ) ;
#27033=CARTESIAN_POINT ( 'NONE',  ( 2.340729813953370519E-16, 21.32270188528330834, -66.10160580289945642 ) ) ;
#27034=CARTESIAN_POINT ( 'NONE',  ( -3.500000000000001332, 17.50000000000002132, -118.9609808024215170 ) ) ;
#27035=CARTESIAN_POINT ( 'NONE',  ( -3.310556943750001313, 17.50000000000002132, -103.7641058028994649 ) ) ;
#27036=CARTESIAN_POINT ( 'NONE',  ( 1.750000000000001110, 20.53108891324555074, -59.98806413671076143 ) ) ;
#27040=CARTESIAN_POINT ( 'NONE',  ( 1.749999999999998224, 14.46891108675447946, -70.62764746908817415 ) ) ;
#27041=CARTESIAN_POINT ( 'NONE',  ( 3.500000000000001332, 19.52072594216371115, -100.3776474690881741 ) ) ;
#27042=CARTESIAN_POINT ( 'NONE',  ( 1.655278471874998436, 14.63297358603753828, -37.43077246956613635 ) ) ;
#27043=CARTESIAN_POINT ( 'NONE',  ( -1.655278471875002211, 14.63297358603754716, -90.68493913623279923 ) ) ;
#27044=CARTESIAN_POINT ( 'NONE',  ( 3.500000000000001332, 17.50000000000001421, -58.15473080337743284 ) ) ;
#27045=FACE_OUTER_BOUND ( 'NONE', #22596, .T. ) ;
#27046=CARTESIAN_POINT ( 'NONE',  ( -3.310556943750000425, 19.41135094264166838, -113.9349391362327850 ) ) ;
#27047=CARTESIAN_POINT ( 'NONE',  ( -1.655278471875002211, 14.63297358603754184, -43.68493913623279212 ) ) ;
#27049=CARTESIAN_POINT ( 'NONE',  ( 4.648177544792955347E-16, 21.00000000000001421, -62.90473080337742573 ) ) ;
#27053=CARTESIAN_POINT ( 'NONE',  ( 0.000000000000000000, 21.00000000000002487, -149.5231586289125687 ) ) ;
#27054=CARTESIAN_POINT ( 'NONE',  ( 1.655278471874998436, 14.63297358603754539, -93.43077246956613635 ) ) ;
#27056=ORIENTED_EDGE ( 'NONE', *, *, #19979, .T. ) ;
#27062=CARTESIAN_POINT ( 'NONE',  ( 0.9378221735089300459, 21.00000000000001421, -73.94938900211595012 ) ) ;
#27063=EDGE_CURVE ( 'NONE', #36906, #41331, #25613, .T. ) ;
#27066=CARTESIAN_POINT ( 'NONE',  ( 1.749999999999998224, 14.46891108675448123, -82.32139747004410424 ) ) ;
#27070=ORIENTED_EDGE ( 'NONE', *, *, #7921, .T. ) ;
#27073=CARTESIAN_POINT ( 'NONE',  ( 3.500000000000000000, 15.47927405783633503, -137.2380641367107614 ) ) ;
#27075=CARTESIAN_POINT ( 'NONE',  ( 4.648177544792955347E-16, 21.00000000000001421, -63.90473080337742573 ) ) ;
#27076=CARTESIAN_POINT ( 'NONE',  ( -3.310556943750002645, 15.58864905735837780, -128.7682724695661136 ) ) ;
#27077=CARTESIAN_POINT ( 'NONE',  ( 1.749999999999998224, 14.46891108675447413, -27.62764746908817770 ) ) ;
#27079=CARTESIAN_POINT ( 'NONE',  ( -3.500000000000001332, 17.50000000000002487, -141.6547308033774186 ) ) ;
#27082=CARTESIAN_POINT ( 'NONE',  ( 3.500000000000001332, 17.50000000000002487, -133.4609808024214885 ) ) ;
#27083=CARTESIAN_POINT ( 'NONE',  ( -1.655278471875002211, 14.63297358603755072, -115.5974391362327935 ) ) ;
#27086=CARTESIAN_POINT ( 'NONE',  ( 3.500000000000001332, 17.50000000000001776, -88.46098080242151696 ) ) ;
#27089=CARTESIAN_POINT ( 'NONE',  ( 1.655278471874998436, 14.63297358603754006, -53.43077246956613635 ) ) ;
#27090=CARTESIAN_POINT ( 'NONE',  ( -1.655278471875002211, 14.63297358603754894, -104.6849391362327992 ) ) ;
#27094=CARTESIAN_POINT ( 'NONE',  ( 2.340729813953370519E-16, 21.32270188528332255, -130.1016058028994564 ) ) ;
#27097=CARTESIAN_POINT ( 'NONE',  ( 0.000000000000000000, 17.50000000000002487, -149.5231586289125687 ) ) ;
#27098=CARTESIAN_POINT ( 'NONE',  ( 4.286263797015737581E-16, 14.00000000000002487, -149.5231586289125687 ) ) ;
#27099=CARTESIAN_POINT ( 'NONE',  ( 3.310556943750001313, 19.41135094264166128, -66.26827246956612782 ) ) ;
#27100=ADVANCED_FACE ( 'NONE', ( #14383 ), #20773, .T. ) ;
#27101=ORIENTED_EDGE ( 'NONE', *, *, #12682, .T. ) ;
#27102=CARTESIAN_POINT ( 'NONE',  ( 1.655278471874998436, 14.63297358603754539, -81.51827246956614204 ) ) ;
#27107=CARTESIAN_POINT ( 'NONE',  ( 1.655278471875001101, 20.36702641396248481, -43.09743913623280065 ) ) ;
#27108=CARTESIAN_POINT ( 'NONE',  ( -1.655278471874999990, 20.36702641396249192, -100.9307724695661364 ) ) ;
#27110=ORIENTED_EDGE ( 'NONE', *, *, #25806, .T. ) ;
#27114=CARTESIAN_POINT ( 'NONE',  ( 3.310556943750001313, 17.50000000000001421, -51.26410580289947205 ) ) ;
#27116=ORIENTED_EDGE ( 'NONE', *, *, #33220, .F. ) ;
#27119=CARTESIAN_POINT ( 'NONE',  ( -1.750000000000002220, 14.46891108675448478, -95.79431413575484555 ) ) ;
#27121=LINE ( 'NONE', #33501, #15684 ) ;
#27122=ORIENTED_EDGE ( 'NONE', *, *, #36555, .T. ) ;
#27123=CARTESIAN_POINT ( 'NONE',  ( -3.500000000000001332, 17.50000000000001066, -41.96098080242150985 ) ) ;
#27126=AXIS2_PLACEMENT_3D ( 'NONE', #2122, #5107, #40424 ) ;
#27127=AXIS2_PLACEMENT_3D ( 'NONE', #17708, #30678, #23466 ) ;
#27129=CARTESIAN_POINT ( 'NONE',  ( -3.310556943750000425, 19.41135094264165772, -26.93493913623279568 ) ) ;
#27131=CARTESIAN_POINT ( 'NONE',  ( -7.022189441860112050E-16, 13.67729811471672186, -80.60160580289947063 ) ) ;
#27132=CARTESIAN_POINT ( 'NONE',  ( 1.655278471875001101, 20.36702641396249902, -135.0974391362328220 ) ) ;
#27135=CARTESIAN_POINT ( 'NONE',  ( 0.9378221735089281585, 14.00000000000000711, -24.36007260463890844 ) ) ;
#27136=CARTESIAN_POINT ( 'NONE',  ( 1.655278471875001101, 20.36702641396249547, -127.1849391362327992 ) ) ;
#27137=FACE_OUTER_BOUND ( 'NONE', #1374, .T. ) ;
#27138=CARTESIAN_POINT ( 'NONE',  ( 1.655278471875001101, 20.36702641396249192, -85.09743913623279354 ) ) ;
#27139=CARTESIAN_POINT ( 'NONE',  ( -1.394453263437886604E-15, 14.00000000000001776, -87.40473080337743284 ) ) ;
#27140=CARTESIAN_POINT ( 'NONE',  ( -7.460324959392693302E-14, 21.00000000000001776, -100.9047308033774186 ) ) ;
#27141=CARTESIAN_POINT ( 'NONE',  ( 1.749999999999998224, 14.46891108675447235, -25.32139747004409713 ) ) ;
#27142=CARTESIAN_POINT ( 'NONE',  ( 3.500000000000000000, 15.47927405783632437, -69.23806413671077564 ) ) ;
#27144=CARTESIAN_POINT ( 'NONE',  ( -3.310556943750001313, 17.50000000000001421, -55.85160580289947063 ) ) ;
#27148=CARTESIAN_POINT ( 'NONE',  ( 3.310556943749999981, 15.58864905735836714, -80.43493913623281344 ) ) ;
#27149=CARTESIAN_POINT ( 'NONE',  ( 3.310556943750001313, 19.41135094264167549, -139.2682724695661420 ) ) ;
#27152=CARTESIAN_POINT ( 'NONE',  ( -3.310556943750002201, 15.58864905735837425, -106.6807724695661364 ) ) ;
#27153=CARTESIAN_POINT ( 'NONE',  ( 3.310556943749999981, 15.58864905735836714, -75.34743913623280775 ) ) ;
#27154=CARTESIAN_POINT ( 'NONE',  ( -1.394453263437886604E-15, 14.00000000000001776, -100.7109808024215027 ) ) ;
#27155=ORIENTED_EDGE ( 'NONE', *, *, #36555, .F. ) ;
#27156=CARTESIAN_POINT ( 'NONE',  ( 1.655278471874998436, 14.63297358603754716, -95.51827246956612782 ) ) ;
#27157=CARTESIAN_POINT ( 'NONE',  ( -7.424026671074350129E-16, 13.45854811567263809, -99.40473080337743284 ) ) ;
#27158=( BOUNDED_CURVE ( )  B_SPLINE_CURVE ( 2, ( #30945, #27951, #2217, #41352, #30732, #8181, #14782, #27743, #40714 ),
 .UNSPECIFIED., .F., .T. ) 
 B_SPLINE_CURVE_WITH_KNOTS ( ( 3, 2, 2, 2, 3 ),
 ( 0.2562499999999999778, 0.2569444444444444198, 0.2583333333333333592, 0.2597222222222222432, 0.2604166666666666852 ),
 .UNSPECIFIED. ) 
 CURVE ( )  GEOMETRIC_REPRESENTATION_ITEM ( )  RATIONAL_B_SPLINE_CURVE ( ( 0.9330127018922194093, 0.9330127018922194093, 1.000000000000000000, 0.8660254037844387076, 1.000000000000000000, 0.8660254037844387076, 1.000000000000000000, 0.9330127018922194093, 0.9330127018922194093 ) ) 
 REPRESENTATION_ITEM ( '' )  );
#27163=CARTESIAN_POINT ( 'NONE',  ( -3.310556943750001313, 17.50000000000001421, -62.76410580289947205 ) ) ;
#27164=CARTESIAN_POINT ( 'NONE',  ( -1.394453263437886604E-15, 14.00000000000001421, -68.40473080337741862 ) ) ;
#27165=CARTESIAN_POINT ( 'NONE',  ( 3.310556943749999981, 15.58864905735837247, -117.3474391362328078 ) ) ;
#27166=DIRECTION ( 'NONE',  ( -0.000000000000000000, 1.259100132267607459E-16, -1.000000000000000000 ) ) ;
#27170=EDGE_LOOP ( 'NONE', ( #37734, #27479, #21460, #16604 ) ) ;
#27174=CARTESIAN_POINT ( 'NONE',  ( 1.655278471875001101, 20.36702641396248836, -70.09743913623280775 ) ) ;
#27176=ORIENTED_EDGE ( 'NONE', *, *, #18858, .T. ) ;
#27178=CARTESIAN_POINT ( 'NONE',  ( -0.9378221735089310451, 14.00000000000002132, -86.75563900116003424 ) ) ;
#27183=CARTESIAN_POINT ( 'NONE',  ( 0.000000000000000000, 17.50000000000002487, -149.5231586289125687 ) ) ;
#27184=CARTESIAN_POINT ( 'NONE',  ( 1.655278471874998436, 14.63297358603755072, -135.4307724695661364 ) ) ;
#27185=AXIS2_PLACEMENT_3D ( 'NONE', #5182, #5383, #18362 ) ;
#27186=CARTESIAN_POINT ( 'NONE',  ( 4.648177544792955347E-16, 21.00000000000001776, -74.90473080337743284 ) ) ;
#27187=CARTESIAN_POINT ( 'NONE',  ( -1.655278471875002211, 14.63297358603754184, -46.68493913623279923 ) ) ;
#27188=CARTESIAN_POINT ( 'NONE',  ( -1.394453263437886604E-15, 14.00000000000001066, -46.71098080242149564 ) ) ;
#27189=CARTESIAN_POINT ( 'NONE',  ( -1.655278471874999990, 20.36702641396248481, -38.01827246956612782 ) ) ;
#27190=CARTESIAN_POINT ( 'NONE',  ( 1.655278471875001101, 20.36702641396249192, -100.1849391362327992 ) ) ;
#27194=CARTESIAN_POINT ( 'NONE',  ( 3.310556943750001313, 17.50000000000001066, -25.26410580289947916 ) ) ;
#27195=DIRECTION ( 'NONE',  ( 0.000000000000000000, 1.000000000000000000, 0.000000000000000000 ) ) ;
#27196=CARTESIAN_POINT ( 'NONE',  ( 3.500000000000000000, 15.47927405783632793, -97.54431413575484555 ) ) ;
#27197=CARTESIAN_POINT ( 'NONE',  ( 0.9378221735089281585, 14.00000000000002132, -100.3600726046389013 ) ) ;
#27199=CARTESIAN_POINT ( 'NONE',  ( -1.750000000000002220, 14.46891108675448301, -84.48806413671076143 ) ) ;
#27201=CARTESIAN_POINT ( 'NONE',  ( 3.310556943749999981, 15.58864905735836537, -67.43493913623279923 ) ) ;
#27205=CARTESIAN_POINT ( 'NONE',  ( 0.000000000000000000, 17.50000000000002487, -149.5231586289125687 ) ) ;
#27206=CARTESIAN_POINT ( 'NONE',  ( 1.749999999999998224, 14.46891108675447590, -50.62764746908816704 ) ) ;
#27207=CARTESIAN_POINT ( 'NONE',  ( -1.394453263437886604E-15, 14.00000000000001066, -46.40473080337741862 ) ) ;
#27209=CARTESIAN_POINT ( 'NONE',  ( 0.000000000000000000, 17.50000000000002487, -149.5231586289125687 ) ) ;
#27212=CARTESIAN_POINT ( 'NONE',  ( 1.749999999999998224, 14.46891108675448478, -114.3213974700440900 ) ) ;
#27214=CARTESIAN_POINT ( 'NONE',  ( 3.310556943750001313, 19.41135094264166128, -24.26827246956612782 ) ) ;
#27215=CARTESIAN_POINT ( 'NONE',  ( 0.000000000000000000, 17.50000000000002487, -143.4609808024215170 ) ) ;
#27217=CARTESIAN_POINT ( 'NONE',  ( 0.9378221735089281585, 14.00000000000002132, -102.3600726046388871 ) ) ;
#27219=CARTESIAN_POINT ( 'NONE',  ( 3.310556943749999981, 15.58864905735836714, -75.34743913623282197 ) ) ;
#27221=VECTOR ( 'NONE', #32473, 1000.000000000000114 ) ;
#27222=CARTESIAN_POINT ( 'NONE',  ( -1.394453263437886604E-15, 14.00000000000002132, -127.4047308033774186 ) ) ;
#27223=CARTESIAN_POINT ( 'NONE',  ( -1.394453263437886604E-15, 14.00000000000001776, -90.40473080337741862 ) ) ;
#27225=CARTESIAN_POINT ( 'NONE',  ( -3.500000000000001332, 17.50000000000002132, -120.6547308033774328 ) ) ;
#27226=CARTESIAN_POINT ( 'NONE',  ( -3.310556943750000425, 19.41135094264166483, -83.84743913623280775 ) ) ;
#27227=ORIENTED_EDGE ( 'NONE', *, *, #29239, .F. ) ;
#27229=VECTOR ( 'NONE', #20106, 1000.000000000000000 ) ;
#27231=( BOUNDED_CURVE ( )  B_SPLINE_CURVE ( 2, ( #41377, #37553, #15221, #6058, #8407, #31166, #12226, #25214, #15644 ),
 .UNSPECIFIED., .F., .T. ) 
 B_SPLINE_CURVE_WITH_KNOTS ( ( 3, 2, 2, 2, 3 ),
 ( 0.5854166666666666963, 0.5861111111111111382, 0.5875000000000000222, 0.5888888888888889062, 0.5895833333333333481 ),
 .UNSPECIFIED. ) 
 CURVE ( )  GEOMETRIC_REPRESENTATION_ITEM ( )  RATIONAL_B_SPLINE_CURVE ( ( 0.9330127018922194093, 0.9330127018922194093, 1.000000000000000000, 0.8660254037844387076, 1.000000000000000000, 0.8660254037844387076, 1.000000000000000000, 0.9330127018922194093, 0.9330127018922194093 ) ) 
 REPRESENTATION_ITEM ( '' )  );
#27235=EDGE_CURVE ( 'NONE', #39182, #18829, #2240, .T. ) ;
#27237=CARTESIAN_POINT ( 'NONE',  ( 3.310556943750001313, 17.50000000000001421, -56.35160580289947063 ) ) ;
#27238=CARTESIAN_POINT ( 'NONE',  ( 1.655278471875001101, 20.36702641396249547, -113.1849391362327992 ) ) ;
#27239=ORIENTED_EDGE ( 'NONE', *, *, #1977, .T. ) ;
#27240=CARTESIAN_POINT ( 'NONE',  ( -1.749999999999999778, 20.53108891324555785, -127.8213974700440900 ) ) ;
#27242=CARTESIAN_POINT ( 'NONE',  ( 1.655278471875001101, 20.36702641396248481, -42.09743913623280065 ) ) ;
#27243=CARTESIAN_POINT ( 'NONE',  ( -3.310556943750001313, 17.50000000000001421, -68.85160580289947063 ) ) ;
#27244=CARTESIAN_POINT ( 'NONE',  ( -3.500000000000001332, 17.50000000000002132, -111.9609808024215027 ) ) ;
#27245=CARTESIAN_POINT ( 'NONE',  ( -7.022189441860112050E-16, 13.67729811471672541, -99.51410580289946495 ) ) ;
#27246=EDGE_CURVE ( 'NONE', #15516, #27029, #12305, .T. ) ;
#27247=CARTESIAN_POINT ( 'NONE',  ( 3.500000000000001332, 19.52072594216371115, -98.07139747004407582 ) ) ;
#27252=CARTESIAN_POINT ( 'NONE',  ( 1.749999999999998224, 14.46891108675447946, -71.62764746908817415 ) ) ;
#27253=CARTESIAN_POINT ( 'NONE',  ( 0.000000000000000000, 17.50000000000002487, -149.5231586289125687 ) ) ;
#27254=CARTESIAN_POINT ( 'NONE',  ( -3.310556943750001313, 17.50000000000001066, -34.76410580289947205 ) ) ;
#27255=AXIS2_PLACEMENT_3D ( 'NONE', #27342, #18392, #1184 ) ;
#27256=CARTESIAN_POINT ( 'NONE',  ( -1.655278471874999990, 20.36702641396249192, -93.01827246956612782 ) ) ;
#27257=EDGE_CURVE ( 'NONE', #20942, #4773, #3611, .T. ) ;
#27258=CARTESIAN_POINT ( 'NONE',  ( -3.500000000000000888, 19.52072594216370760, -60.73806413671076854 ) ) ;
#27259=CARTESIAN_POINT ( 'NONE',  ( -3.310556943750001313, 17.50000000000002132, -113.8516058028994706 ) ) ;
#27260=CARTESIAN_POINT ( 'NONE',  ( -1.655278471874999990, 20.36702641396248481, -36.01827246956612782 ) ) ;
#27266=CARTESIAN_POINT ( 'NONE',  ( 0.000000000000000000, 17.50000000000002487, -149.5231586289125687 ) ) ;
#27267=CARTESIAN_POINT ( 'NONE',  ( -1.655278471874999990, 20.36702641396249192, -90.93077246956613635 ) ) ;
#27268=CARTESIAN_POINT ( 'NONE',  ( 4.648177544792955347E-16, 21.00000000000001066, -35.90473080337743284 ) ) ;
#27271=CARTESIAN_POINT ( 'NONE',  ( 3.500000000000001332, 19.52072594216370760, -57.37764746908817415 ) ) ;
#27273=CARTESIAN_POINT ( 'NONE',  ( 0.000000000000000000, 17.50000000000002487, -149.5231586289125687 ) ) ;
#27274=ORIENTED_EDGE ( 'NONE', *, *, #8067, .T. ) ;
#27279=CARTESIAN_POINT ( 'NONE',  ( 0.000000000000000000, 17.50000000000002487, -149.5231586289125687 ) ) ;
#27283=ORIENTED_EDGE ( 'NONE', *, *, #5845, .T. ) ;
#27284=CARTESIAN_POINT ( 'NONE',  ( -1.394453263437886604E-15, 14.00000000000001066, -53.71098080242150985 ) ) ;
#27285=( BOUNDED_CURVE ( )  B_SPLINE_CURVE ( 2, ( #3390, #6584, #35722, #4018, #29113, #10410, #19549, #13811, #29321 ),
 .UNSPECIFIED., .F., .F. ) 
 B_SPLINE_CURVE_WITH_KNOTS ( ( 3, 2, 2, 2, 3 ),
 ( 0.09375000000000000000, 0.09444444444444444198, 0.09583333333333333981, 0.09722222222222222376, 0.09791666666666666574 ),
 .UNSPECIFIED. ) 
 CURVE ( )  GEOMETRIC_REPRESENTATION_ITEM ( )  RATIONAL_B_SPLINE_CURVE ( ( 0.9330127018922194093, 0.9330127018922194093, 1.000000000000000000, 0.8660254037844387076, 1.000000000000000000, 0.8660254037844387076, 1.000000000000000000, 0.9330127018922194093, 0.9330127018922194093 ) ) 
 REPRESENTATION_ITEM ( '' )  );
#27287=CARTESIAN_POINT ( 'NONE',  ( 1.655278471874998436, 14.63297358603755249, -140.4307724695661364 ) ) ;
#27288=CARTESIAN_POINT ( 'NONE',  ( 0.9378221735089300459, 21.00000000000002132, -109.9493890021159359 ) ) ;
#27291=CARTESIAN_POINT ( 'NONE',  ( 3.310556943750001313, 19.41135094264166838, -129.2682724695661420 ) ) ;
#27292=CARTESIAN_POINT ( 'NONE',  ( -1.655278471874999990, 20.36702641396248836, -55.01827246956612782 ) ) ;
#27295=CARTESIAN_POINT ( 'NONE',  ( -1.750000000000002220, 14.46891108675447768, -44.48806413671076143 ) ) ;
#27296=CARTESIAN_POINT ( 'NONE',  ( 4.648177544792955347E-16, 21.00000000000001066, -42.90473080337742573 ) ) ;
#27298=CARTESIAN_POINT ( 'NONE',  ( -1.750000000000002220, 14.46891108675448834, -132.7943141357548598 ) ) ;
#27299=CARTESIAN_POINT ( 'NONE',  ( 3.310556943750001313, 17.50000000000002132, -112.2641058028994792 ) ) ;
#27300=EDGE_CURVE ( 'NONE', #18588, #3414, #27231, .T. ) ;
#27303=CARTESIAN_POINT ( 'NONE',  ( -7.424026671074350129E-16, 13.45854811567263631, -87.71098080242151696 ) ) ;
#27305=CARTESIAN_POINT ( 'NONE',  ( -3.310556943750000425, 19.41135094264166128, -49.84743913623281486 ) ) ;
#27306=CARTESIAN_POINT ( 'NONE',  ( -1.655278471874999990, 20.36702641396249547, -106.0182724695661278 ) ) ;
#27307=CARTESIAN_POINT ( 'NONE',  ( 0.9378221735089281585, 14.00000000000000888, -38.66632260368299256 ) ) ;
#27309=CARTESIAN_POINT ( 'NONE',  ( -1.394453263437886604E-15, 14.00000000000001776, -88.71098080242148853 ) ) ;
#27310=CARTESIAN_POINT ( 'NONE',  ( 1.655278471875001101, 20.36702641396249547, -127.1849391362327992 ) ) ;
#27313=CARTESIAN_POINT ( 'NONE',  ( -1.750000000000002220, 14.46891108675448656, -116.7943141357548313 ) ) ;
#27315=CARTESIAN_POINT ( 'NONE',  ( 1.655278471874998436, 14.63297358603754184, -57.51827246956612782 ) ) ;
#27318=ORIENTED_EDGE ( 'NONE', *, *, #2782, .F. ) ;
#27319=CARTESIAN_POINT ( 'NONE',  ( -1.655278471874999990, 20.36702641396249192, -80.01827246956614204 ) ) ;
#27324=CARTESIAN_POINT ( 'NONE',  ( -3.310556943750001313, 17.50000000000001066, -38.76410580289947916 ) ) ;
#27325=CARTESIAN_POINT ( 'NONE',  ( 1.655278471875001101, 20.36702641396249192, -100.0974391362328078 ) ) ;
#27329=VECTOR ( 'NONE', #11059, 1000.000000000000000 ) ;
#27330=CARTESIAN_POINT ( 'NONE',  ( 3.310556943750001313, 17.50000000000001421, -53.26410580289947205 ) ) ;
#27331=ORIENTED_EDGE ( 'NONE', *, *, #6454, .T. ) ;
#27332=ORIENTED_EDGE ( 'NONE', *, *, #36552, .F. ) ;
#27333=CARTESIAN_POINT ( 'NONE',  ( -0.9378221735089291577, 21.00000000000001776, -98.86007260463890134 ) ) ;
#27335=CARTESIAN_POINT ( 'NONE',  ( 1.749999999999998224, 14.46891108675448478, -113.6276474690881741 ) ) ;
#27336=ORIENTED_EDGE ( 'NONE', *, *, #28681, .T. ) ;
#27337=CARTESIAN_POINT ( 'NONE',  ( 2.474675557024783212E-16, 21.54145188432739033, -42.21098080242150985 ) ) ;
#27338=LINE ( 'NONE', #7347, #34327 ) ;
#27341=CARTESIAN_POINT ( 'NONE',  ( 3.310556943750001313, 17.50000000000001066, -29.35160580289947063 ) ) ;
#27342=CARTESIAN_POINT ( 'NONE',  ( 0.000000000000000000, 17.50000000000002487, -149.5231586289125687 ) ) ;
#27343=CARTESIAN_POINT ( 'NONE',  ( -3.310556943750001313, 17.50000000000002487, -131.7641058028994507 ) ) ;
#27344=EDGE_CURVE ( 'NONE', #40555, #26058, #9589, .T. ) ;
#27347=CARTESIAN_POINT ( 'NONE',  ( -3.500000000000001332, 17.50000000000001066, -38.65473080337743284 ) ) ;
#27348=CARTESIAN_POINT ( 'NONE',  ( -3.310556943750001313, 17.50000000000002132, -124.8516058028994564 ) ) ;
#27350=CARTESIAN_POINT ( 'NONE',  ( -1.655278471875002211, 14.63297358603754716, -86.59743913623280775 ) ) ;
#27352=CARTESIAN_POINT ( 'NONE',  ( -1.749999999999999778, 20.53108891324555074, -49.82139747004410424 ) ) ;
#27353=CARTESIAN_POINT ( 'NONE',  ( 0.9378221735089281585, 14.00000000000001243, -65.36007260463891555 ) ) ;
#27354=CARTESIAN_POINT ( 'NONE',  ( 1.749999999999998224, 14.46891108675448123, -89.32139747004410424 ) ) ;
#27355=CARTESIAN_POINT ( 'NONE',  ( 1.750000000000001110, 20.53108891324555074, -70.98806413671076143 ) ) ;
#27357=CARTESIAN_POINT ( 'NONE',  ( 3.310556943749999981, 15.58864905735836182, -52.43493913623280633 ) ) ;
#27362=CARTESIAN_POINT ( 'NONE',  ( -7.022189441860112050E-16, 13.67729811471672186, -78.60160580289944221 ) ) ;
#27363=CARTESIAN_POINT ( 'NONE',  ( -1.655278471874999990, 20.36702641396249902, -140.0182724695661420 ) ) ;
#27365=CARTESIAN_POINT ( 'NONE',  ( -1.655278471875002211, 14.63297358603754894, -104.5974391362328078 ) ) ;
#27366=CARTESIAN_POINT ( 'NONE',  ( 1.655278471875001101, 20.36702641396248836, -74.09743913623280775 ) ) ;
#27367=VERTEX_POINT ( 'NONE', #34991 ) ;
#27368=CARTESIAN_POINT ( 'NONE',  ( -3.310556943750002201, 15.58864905735837425, -95.76827246956612782 ) ) ;
#27370=CARTESIAN_POINT ( 'NONE',  ( 3.500000000000001332, 19.52072594216371115, -91.37764746908817415 ) ) ;
#27371=FACE_OUTER_BOUND ( 'NONE', #24101, .T. ) ;
#27373=CARTESIAN_POINT ( 'NONE',  ( 3.310556943750001313, 19.41135094264166483, -55.18077246956612925 ) ) ;
#27375=CARTESIAN_POINT ( 'NONE',  ( -3.310556943750001313, 17.50000000000002132, -116.7641058028994792 ) ) ;
#27376=CARTESIAN_POINT ( 'NONE',  ( 4.648177544792955347E-16, 21.00000000000002132, -115.9047308033774328 ) ) ;
#27378=ORIENTED_EDGE ( 'NONE', *, *, #32132, .F. ) ;
#27381=CARTESIAN_POINT ( 'NONE',  ( 4.286263797015737581E-16, 14.00000000000002487, -149.5231586289125687 ) ) ;
#27382=CARTESIAN_POINT ( 'NONE',  ( -1.655278471874999990, 20.36702641396248836, -69.93077246956613635 ) ) ;
#27395=CARTESIAN_POINT ( 'NONE',  ( 3.310556943750001313, 17.50000000000002487, -137.2641058028994792 ) ) ;
#27397=CARTESIAN_POINT ( 'NONE',  ( 1.655278471875001101, 20.36702641396248836, -47.18493913623279923 ) ) ;
#27399=CARTESIAN_POINT ( 'NONE',  ( 1.655278471874998436, 14.63297358603753828, -33.51827246956613493 ) ) ;
#27400=CARTESIAN_POINT ( 'NONE',  ( -7.022189441860112050E-16, 13.67729811471672541, -99.60160580289947063 ) ) ;
#27402=( BOUNDED_CURVE ( )  B_SPLINE_CURVE ( 2, ( #8028, #7829, #30780, #40359, #13998, #14624, #36969, #37373, #16973 ),
 .UNSPECIFIED., .F., .T. ) 
 B_SPLINE_CURVE_WITH_KNOTS ( ( 3, 2, 2, 2, 3 ),
 ( 0.2562499999999999778, 0.2569444444444444198, 0.2583333333333333592, 0.2597222222222222432, 0.2604166666666666852 ),
 .UNSPECIFIED. ) 
 CURVE ( )  GEOMETRIC_REPRESENTATION_ITEM ( )  RATIONAL_B_SPLINE_CURVE ( ( 0.9330127018922194093, 0.9330127018922194093, 1.000000000000000000, 0.8660254037844387076, 1.000000000000000000, 0.8660254037844387076, 1.000000000000000000, 0.9330127018922194093, 0.9330127018922194093 ) ) 
 REPRESENTATION_ITEM ( '' )  );
#27403=CARTESIAN_POINT ( 'NONE',  ( 1.655278471874998436, 14.63297358603755249, -139.5182724695661420 ) ) ;
#27405=CARTESIAN_POINT ( 'NONE',  ( -1.749999999999999778, 20.53108891324555429, -97.12764746908817415 ) ) ;
#27406=CARTESIAN_POINT ( 'NONE',  ( 4.648177544792955347E-16, 21.00000000000001776, -99.90473080337743284 ) ) ;
#27407=CARTESIAN_POINT ( 'NONE',  ( 3.500000000000001332, 17.50000000000001421, -64.46098080242150274 ) ) ;
#27408=CARTESIAN_POINT ( 'NONE',  ( -3.500000000000002220, 15.47927405783632793, -85.57139747004409003 ) ) ;
#27409=CARTESIAN_POINT ( 'NONE',  ( -1.655278471874999990, 20.36702641396248836, -69.01827246956612782 ) ) ;
#27412=ADVANCED_FACE ( 'NONE', ( #25844 ), #12864, .T. ) ;
#27414=CARTESIAN_POINT ( 'NONE',  ( 0.000000000000000000, 17.50000000000002487, -149.5231586289125687 ) ) ;
#27415=CARTESIAN_POINT ( 'NONE',  ( -3.500000000000000888, 19.52072594216370760, -48.04431413575484555 ) ) ;
#27416=CARTESIAN_POINT ( 'NONE',  ( -1.655278471875002211, 14.63297358603755072, -117.5974391362328078 ) ) ;
#27421=CARTESIAN_POINT ( 'NONE',  ( -3.500000000000001332, 17.50000000000002132, -114.6547308033774328 ) ) ;
#27422=DIRECTION ( 'NONE',  ( -0.000000000000000000, 1.259100132267607459E-16, -1.000000000000000000 ) ) ;
#27427=CARTESIAN_POINT ( 'NONE',  ( 3.310556943749999981, 15.58864905735836714, -79.34743913623280775 ) ) ;
#27429=CARTESIAN_POINT ( 'NONE',  ( 4.648177544792955347E-16, 21.00000000000001776, -89.90473080337741862 ) ) ;
#27431=CARTESIAN_POINT ( 'NONE',  ( 0.9378221735088952959, 21.00000000000003908, -88.25563900116003424 ) ) ;
#27432=CARTESIAN_POINT ( 'NONE',  ( -7.022189441860112050E-16, 13.67729811471672363, -85.51410580289946495 ) ) ;
#27433=ORIENTED_EDGE ( 'NONE', *, *, #22507, .T. ) ;
#27434=ORIENTED_EDGE ( 'NONE', *, *, #22978, .F. ) ;
#27436=EDGE_CURVE ( 'NONE', #11709, #9764, #9464, .T. ) ;
#27441=VECTOR ( 'NONE', #2082, 1000.000000000000000 ) ;
#27442=CARTESIAN_POINT ( 'NONE',  ( 4.648177544792955347E-16, 21.00000000000002132, -117.9047308033774328 ) ) ;
#27443=CARTESIAN_POINT ( 'NONE',  ( -1.655278471875002211, 14.63297358603754184, -50.68493913623279923 ) ) ;
#27444=CARTESIAN_POINT ( 'NONE',  ( 1.655278471874998436, 14.63297358603754894, -114.5182724695661278 ) ) ;
#27445=VERTEX_POINT ( 'NONE', #26053 ) ;
#27446=CARTESIAN_POINT ( 'NONE',  ( 3.500000000000001332, 17.50000000000002132, -127.1547308033774186 ) ) ;
#27447=CARTESIAN_POINT ( 'NONE',  ( -3.310556943750000425, 19.41135094264165772, -41.84743913623280775 ) ) ;
#27449=CARTESIAN_POINT ( 'NONE',  ( 3.310556943750001313, 19.41135094264166128, -64.26827246956614204 ) ) ;
#27450=CARTESIAN_POINT ( 'NONE',  ( -3.500000000000000888, 19.52072594216371826, -113.0443141357548456 ) ) ;
#27452=CARTESIAN_POINT ( 'NONE',  ( -3.310556943750000425, 19.41135094264166483, -95.84743913623282197 ) ) ;
#27455=CARTESIAN_POINT ( 'NONE',  ( -1.750000000000002220, 14.46891108675448123, -70.48806413671076143 ) ) ;
#27457=CARTESIAN_POINT ( 'NONE',  ( -3.500000000000002220, 15.47927405783632437, -65.87764746908815994 ) ) ;
#27459=CARTESIAN_POINT ( 'NONE',  ( -3.310556943750001313, 17.50000000000001066, -29.76410580289948271 ) ) ;
#27460=CARTESIAN_POINT ( 'NONE',  ( -3.310556943750000425, 19.41135094264166483, -90.93493913623279923 ) ) ;
#27461=CARTESIAN_POINT ( 'NONE',  ( 3.500000000000001332, 17.50000000000001421, -54.15473080337743284 ) ) ;
#27462=DIRECTION ( 'NONE',  ( -0.000000000000000000, 1.259100132267607459E-16, -1.000000000000000000 ) ) ;
#27463=CARTESIAN_POINT ( 'NONE',  ( 2.340729813953370519E-16, 21.32270188528331900, -113.1016058028994706 ) ) ;
#27464=CARTESIAN_POINT ( 'NONE',  ( -3.310556943750002201, 15.58864905735836537, -38.76827246956612782 ) ) ;
#27470=CARTESIAN_POINT ( 'NONE',  ( -1.394453263437886604E-15, 14.00000000000000711, -23.40473080337742928 ) ) ;
#27471=CARTESIAN_POINT ( 'NONE',  ( -7.022189441860112050E-16, 13.67729811471672363, -94.51410580289945074 ) ) ;
#27479=ORIENTED_EDGE ( 'NONE', *, *, #10684, .F. ) ;
#27483=( BOUNDED_CURVE ( )  B_SPLINE_CURVE ( 2, ( #611, #12964, #26788, #13586, #4014, #16583, #23600, #16998, #36560 ),
 .UNSPECIFIED., .F., .T. ) 
 B_SPLINE_CURVE_WITH_KNOTS ( ( 3, 2, 2, 2, 3 ),
 ( 0.06875000000000000555, 0.06944444444444444753, 0.07083333333333333148, 0.07222222222222221544, 0.07291666666666667129 ),
 .UNSPECIFIED. ) 
 CURVE ( )  GEOMETRIC_REPRESENTATION_ITEM ( )  RATIONAL_B_SPLINE_CURVE ( ( 0.9330127018922194093, 0.9330127018922200755, 1.000000000000000000, 0.8660254037844387076, 1.000000000000000000, 0.8660254037844387076, 1.000000000000000000, 0.9330127018922187432, 0.9330127018922194093 ) ) 
 REPRESENTATION_ITEM ( '' )  );
#27485=CARTESIAN_POINT ( 'NONE',  ( 3.500000000000001332, 17.50000000000001776, -82.15473080337743284 ) ) ;
#27486=VECTOR ( 'NONE', #28779, 1000.000000000000000 ) ;
#27492=ORIENTED_EDGE ( 'NONE', *, *, #34755, .F. ) ;
#27493=CARTESIAN_POINT ( 'NONE',  ( -1.394453263437886604E-15, 14.00000000000001421, -70.71098080242150274 ) ) ;
#27494=DIRECTION ( 'NONE',  ( 0.000000000000000000, 1.000000000000000000, 0.000000000000000000 ) ) ;
#27496=CARTESIAN_POINT ( 'NONE',  ( 3.310556943749999981, 15.58864905735837780, -142.3474391362327935 ) ) ;
#27497=CARTESIAN_POINT ( 'NONE',  ( -1.394453263437886604E-15, 14.00000000000001776, -104.4047308033774186 ) ) ;
#27498=CARTESIAN_POINT ( 'NONE',  ( 0.9378221735088952959, 21.00000000000003908, -101.2556390011600342 ) ) ;
#27499=CARTESIAN_POINT ( 'NONE',  ( -3.310556943750001313, 17.50000000000002487, -131.8516058028994564 ) ) ;
#27500=CARTESIAN_POINT ( 'NONE',  ( 2.340729813953370519E-16, 21.32270188528330834, -54.10160580289947063 ) ) ;
#27503=CARTESIAN_POINT ( 'NONE',  ( 2.474675557024783212E-16, 21.54145188432740810, -139.9047308033774186 ) ) ;
#27506=CARTESIAN_POINT ( 'NONE',  ( -3.500000000000000888, 19.52072594216371826, -128.0443141357548313 ) ) ;
#27507=CARTESIAN_POINT ( 'NONE',  ( 3.310556943750001313, 17.50000000000002132, -114.2641058028994792 ) ) ;
#27510=CARTESIAN_POINT ( 'NONE',  ( 3.500000000000001776, 19.52072594216371115, -81.37764746908817415 ) ) ;
#27513=CARTESIAN_POINT ( 'NONE',  ( -1.655278471874999990, 20.36702641396248836, -46.93077246956614346 ) ) ;
#27514=CARTESIAN_POINT ( 'NONE',  ( 3.310556943750001313, 19.41135094264166838, -108.2682724695661278 ) ) ;
#27515=CARTESIAN_POINT ( 'NONE',  ( -3.500000000000000000, 19.52072594216371115, -83.04431413575484555 ) ) ;
#27516=CARTESIAN_POINT ( 'NONE',  ( -1.394453263437886604E-15, 14.00000000000001776, -99.40473080337743284 ) ) ;
#27519=CARTESIAN_POINT ( 'NONE',  ( -1.655278471874999990, 20.36702641396249902, -131.0182724695661136 ) ) ;
#27523=DIRECTION ( 'NONE',  ( -0.000000000000000000, 1.259100132267607459E-16, -1.000000000000000000 ) ) ;
#27524=CARTESIAN_POINT ( 'NONE',  ( 1.655278471875001101, 20.36702641396248836, -61.18493913623279923 ) ) ;
#27526=CARTESIAN_POINT ( 'NONE',  ( -1.655278471875002211, 14.63297358603754539, -79.68493913623279923 ) ) ;
#27534=CARTESIAN_POINT ( 'NONE',  ( -1.655278471874999990, 20.36702641396248481, -38.93077246956613635 ) ) ;
#27535=CARTESIAN_POINT ( 'NONE',  ( -1.655278471875002211, 14.63297358603754716, -92.59743913623280775 ) ) ;
#27537=( BOUNDED_CURVE ( )  B_SPLINE_CURVE ( 2, ( #35598, #22406, #38157, #6248, #9233, #18804, #19012, #31979, #19224 ),
 .UNSPECIFIED., .F., .T. ) 
 B_SPLINE_CURVE_WITH_KNOTS ( ( 3, 2, 2, 2, 3 ),
 ( 0.8979166666666666963, 0.8986111111111111382, 0.9000000000000000222, 0.9013888888888889062, 0.9020833333333333481 ),
 .UNSPECIFIED. ) 
 CURVE ( )  GEOMETRIC_REPRESENTATION_ITEM ( )  RATIONAL_B_SPLINE_CURVE ( ( 0.9330127018922194093, 0.9330127018922194093, 1.000000000000000000, 0.8660254037844387076, 1.000000000000000000, 0.8660254037844387076, 1.000000000000000000, 0.9330127018922194093, 0.9330127018922194093 ) ) 
 REPRESENTATION_ITEM ( '' )  );
#27543=CARTESIAN_POINT ( 'NONE',  ( 2.340729813953370519E-16, 21.32270188528330834, -53.01410580289947916 ) ) ;
#27546=CARTESIAN_POINT ( 'NONE',  ( -0.9378221735089310451, 14.00000000000001066, -43.44938900211593591 ) ) ;
#27548=CARTESIAN_POINT ( 'NONE',  ( 4.648177544792955347E-16, 21.00000000000001776, -82.90473080337743284 ) ) ;
#27549=VECTOR ( 'NONE', #21231, 1000.000000000000000 ) ;
#27550=ORIENTED_EDGE ( 'NONE', *, *, #38867, .T. ) ;
#27551=CARTESIAN_POINT ( 'NONE',  ( 3.500000000000001332, 17.50000000000001776, -89.46098080242151696 ) ) ;
#27552=CARTESIAN_POINT ( 'NONE',  ( -3.500000000000002220, 15.47927405783632082, -37.87764746908816704 ) ) ;
#27556=CARTESIAN_POINT ( 'NONE',  ( -7.022189441860112050E-16, 13.67729811471671297, -25.60160580289946708 ) ) ;
#27557=CARTESIAN_POINT ( 'NONE',  ( 3.310556943750001313, 19.41135094264166838, -129.1807724695661364 ) ) ;
#27560=CARTESIAN_POINT ( 'NONE',  ( -1.394453263437886604E-15, 14.00000000000002132, -127.4047308033774186 ) ) ;
#27561=CARTESIAN_POINT ( 'NONE',  ( 3.310556943750001313, 17.50000000000002132, -125.3516058028994706 ) ) ;
#27563=CARTESIAN_POINT ( 'NONE',  ( -3.500000000000000888, 19.52072594216370405, -39.73806413671076854 ) ) ;
#27564=CARTESIAN_POINT ( 'NONE',  ( -3.500000000000001332, 17.50000000000001421, -49.65473080337742573 ) ) ;
#27566=CARTESIAN_POINT ( 'NONE',  ( 3.310556943750001313, 19.41135094264167549, -142.2682724695661420 ) ) ;
#27568=CARTESIAN_POINT ( 'NONE',  ( 1.749999999999998224, 14.46891108675447946, -68.32139747004409003 ) ) ;
#27569=CARTESIAN_POINT ( 'NONE',  ( -7.022189441860112050E-16, 13.67729811471671830, -53.60160580289946353 ) ) ;
#27572=CARTESIAN_POINT ( 'NONE',  ( 1.655278471874998436, 14.63297358603754361, -75.51827246956612782 ) ) ;
#27574=CARTESIAN_POINT ( 'NONE',  ( 2.340729813953370519E-16, 21.32270188528331900, -106.0141058028994792 ) ) ;
#27575=CARTESIAN_POINT ( 'NONE',  ( 3.310556943750001313, 19.41135094264166483, -75.18077246956613635 ) ) ;
#27576=ORIENTED_EDGE ( 'NONE', *, *, #5390, .T. ) ;
#27577=CARTESIAN_POINT ( 'NONE',  ( 1.655278471875001101, 20.36702641396249192, -94.18493913623279923 ) ) ;
#27579=CARTESIAN_POINT ( 'NONE',  ( -1.394453263437886604E-15, 14.00000000000001776, -85.40473080337743284 ) ) ;
#27580=CARTESIAN_POINT ( 'NONE',  ( -3.500000000000001332, 17.50000000000001421, -51.96098080242150985 ) ) ;
#27582=CARTESIAN_POINT ( 'NONE',  ( -3.310556943750001313, 17.50000000000001421, -56.76410580289947916 ) ) ;
#27584=CARTESIAN_POINT ( 'NONE',  ( -7.022189441860112050E-16, 13.67729811471672718, -110.5141058028994792 ) ) ;
#27585=ORIENTED_EDGE ( 'NONE', *, *, #40479, .T. ) ;
#27586=ORIENTED_EDGE ( 'NONE', *, *, #19381, .T. ) ;
#27588=ORIENTED_EDGE ( 'NONE', *, *, #19854, .F. ) ;
#27590=ADVANCED_FACE ( 'NONE', ( #13280 ), #3910, .T. ) ;
#27591=CARTESIAN_POINT ( 'NONE',  ( -3.310556943750000425, 19.41135094264166128, -68.84743913623280775 ) ) ;
#27593=ORIENTED_EDGE ( 'NONE', *, *, #1229, .T. ) ;
#27594=CARTESIAN_POINT ( 'NONE',  ( -3.500000000000001332, 17.50000000000002487, -130.9609808024214885 ) ) ;
#27598=ORIENTED_EDGE ( 'NONE', *, *, #18840, .T. ) ;
#27600=CARTESIAN_POINT ( 'NONE',  ( -3.310556943750000425, 19.41135094264166838, -128.8474391362328220 ) ) ;
#27602=CARTESIAN_POINT ( 'NONE',  ( -1.655278471874999990, 20.36702641396248481, -45.01827246956613493 ) ) ;
#27603=CARTESIAN_POINT ( 'NONE',  ( 3.310556943750001313, 17.50000000000001066, -35.35160580289946353 ) ) ;
#27604=CARTESIAN_POINT ( 'NONE',  ( -3.310556943750002645, 15.58864905735837425, -95.76827246956612782 ) ) ;
#27605=CARTESIAN_POINT ( 'NONE',  ( -7.424026671074350129E-16, 13.45854811567263098, -24.40473080337743639 ) ) ;
#27607=CARTESIAN_POINT ( 'NONE',  ( -3.310556943750001313, 17.50000000000002487, -138.8516058028994564 ) ) ;
#27608=CARTESIAN_POINT ( 'NONE',  ( -3.500000000000001332, 17.50000000000001776, -95.96098080242150274 ) ) ;
#27609=CARTESIAN_POINT ( 'NONE',  ( -3.695301148110399846E-14, 21.00000000000002132, -124.2109808024214885 ) ) ;
#27611=CARTESIAN_POINT ( 'NONE',  ( 2.474675557024783212E-16, 21.54145188432739744, -86.90473080337744705 ) ) ;
#27612=CARTESIAN_POINT ( 'NONE',  ( -3.310556943750002201, 15.58864905735837070, -70.76827246956612782 ) ) ;
#27614=CARTESIAN_POINT ( 'NONE',  ( -1.750000000000002220, 14.46891108675448656, -111.4880641367107614 ) ) ;
#27616=CARTESIAN_POINT ( 'NONE',  ( 1.750000000000001110, 20.53108891324555785, -110.2943141357548456 ) ) ;
#27617=CARTESIAN_POINT ( 'NONE',  ( -1.750000000000002220, 14.46891108675447768, -48.79431413575484555 ) ) ;
#27618=CARTESIAN_POINT ( 'NONE',  ( 3.310556943750001313, 19.41135094264166838, -119.1807724695661364 ) ) ;
#27619=CARTESIAN_POINT ( 'NONE',  ( -0.9378221735089291577, 21.00000000000001776, -79.86007260463892976 ) ) ;
#27621=CARTESIAN_POINT ( 'NONE',  ( 2.474675557024783212E-16, 21.54145188432740099, -112.9047308033774470 ) ) ;
#27623=CARTESIAN_POINT ( 'NONE',  ( 0.000000000000000000, 17.50000000000002487, -149.5231586289125687 ) ) ;
#27627=CARTESIAN_POINT ( 'NONE',  ( -3.310556943750002201, 15.58864905735837070, -70.68077246956613635 ) ) ;
#27628=ORIENTED_EDGE ( 'NONE', *, *, #18453, .T. ) ;
#27629=CARTESIAN_POINT ( 'NONE',  ( -3.310556943750000425, 19.41135094264166128, -23.84743913623281486 ) ) ;
#27630=CARTESIAN_POINT ( 'NONE',  ( 0.9378221735089281585, 14.00000000000000711, -25.66632260368299256 ) ) ;
#27631=CARTESIAN_POINT ( 'NONE',  ( -1.655278471874999990, 20.36702641396249192, -83.93077246956615056 ) ) ;
#27638=( BOUNDED_CURVE ( )  B_SPLINE_CURVE ( 2, ( #20276, #37088, #928, #1558, #17721, #33684, #710, #24117, #36219 ),
 .UNSPECIFIED., .F., .F. ) 
 B_SPLINE_CURVE_WITH_KNOTS ( ( 3, 2, 2, 2, 3 ),
 ( 0.1229166666666666741, 0.1236111111111111160, 0.1250000000000000000, 0.1263888888888888840, 0.1270833333333333259 ),
 .UNSPECIFIED. ) 
 CURVE ( )  GEOMETRIC_REPRESENTATION_ITEM ( )  RATIONAL_B_SPLINE_CURVE ( ( 0.9330127018922194093, 0.9330127018922200755, 1.000000000000000000, 0.8660254037844387076, 1.000000000000000000, 0.8660254037844387076, 1.000000000000000000, 0.9330127018922194093, 0.9330127018922194093 ) ) 
 REPRESENTATION_ITEM ( '' )  );
#27639=( BOUNDED_CURVE ( )  B_SPLINE_CURVE ( 2, ( #37914, #40893, #4953, #37498, #2395, #27919, #21124, #8353, #37710 ),
 .UNSPECIFIED., .F., .T. ) 
 B_SPLINE_CURVE_WITH_KNOTS ( ( 3, 2, 2, 2, 3 ),
 ( 0.1020833333333333315, 0.1027777777777777735, 0.1041666666666666713, 0.1055555555555555552, 0.1062499999999999972 ),
 .UNSPECIFIED. ) 
 CURVE ( )  GEOMETRIC_REPRESENTATION_ITEM ( )  RATIONAL_B_SPLINE_CURVE ( ( 0.9330127018922194093, 0.9330127018922194093, 1.000000000000000000, 0.8660254037844387076, 1.000000000000000000, 0.8660254037844387076, 1.000000000000000000, 0.9330127018922194093, 0.9330127018922194093 ) ) 
 REPRESENTATION_ITEM ( '' )  );
#27640=CARTESIAN_POINT ( 'NONE',  ( -1.975475456537005874E-15, 21.00000000000002487, -141.9047308033773902 ) ) ;
#27641=CARTESIAN_POINT ( 'NONE',  ( 3.310556943750001313, 17.50000000000001066, -46.35160580289945642 ) ) ;
#27642=CARTESIAN_POINT ( 'NONE',  ( 3.310556943749999981, 15.58864905735837247, -116.4349391362327850 ) ) ;
#27643=ORIENTED_EDGE ( 'NONE', *, *, #3416, .F. ) ;
#27644=CARTESIAN_POINT ( 'NONE',  ( 1.655278471875001101, 20.36702641396248481, -37.09743913623281486 ) ) ;
#27645=CARTESIAN_POINT ( 'NONE',  ( 1.655278471875001101, 20.36702641396248836, -67.18493913623279923 ) ) ;
#27646=CARTESIAN_POINT ( 'NONE',  ( -3.500000000000001332, 17.50000000000002132, -113.9609808024215027 ) ) ;
#27648=CARTESIAN_POINT ( 'NONE',  ( -1.655278471875002211, 14.63297358603754894, -96.59743913623280775 ) ) ;
#27650=CARTESIAN_POINT ( 'NONE',  ( -3.500000000000000000, 19.52072594216371826, -124.7380641367107756 ) ) ;
#27653=CARTESIAN_POINT ( 'NONE',  ( 3.500000000000001776, 19.52072594216370760, -64.37764746908817415 ) ) ;
#27655=CARTESIAN_POINT ( 'NONE',  ( -3.310556943750001313, 17.50000000000001066, -31.76410580289946850 ) ) ;
#27656=CARTESIAN_POINT ( 'NONE',  ( -1.655278471874999990, 20.36702641396249192, -89.01827246956612782 ) ) ;
#27657=CARTESIAN_POINT ( 'NONE',  ( 1.749999999999998224, 14.46891108675447590, -52.32139747004409003 ) ) ;
#27658=CARTESIAN_POINT ( 'NONE',  ( 0.000000000000000000, 17.50000000000002487, -149.5231586289125687 ) ) ;
#27659=CARTESIAN_POINT ( 'NONE',  ( -3.310556943750000425, 19.41135094264166838, -106.9349391362327992 ) ) ;
#27660=CARTESIAN_POINT ( 'NONE',  ( 1.655278471874998436, 14.63297358603754006, -40.51827246956612782 ) ) ;
#27662=CARTESIAN_POINT ( 'NONE',  ( 3.500000000000001332, 17.50000000000001421, -66.15473080337743284 ) ) ;
#27667=EDGE_CURVE ( 'NONE', #36901, #25503, #12944, .T. ) ;
#27669=CARTESIAN_POINT ( 'NONE',  ( 2.340729813953370519E-16, 21.32270188528331190, -89.01410580289947916 ) ) ;
#27670=CARTESIAN_POINT ( 'NONE',  ( -1.749999999999999778, 20.53108891324556140, -135.8213974700441042 ) ) ;
#27672=VERTEX_POINT ( 'NONE', #19247 ) ;
#27675=CARTESIAN_POINT ( 'NONE',  ( -1.749999999999999778, 20.53108891324555074, -65.12764746908818836 ) ) ;
#27681=CARTESIAN_POINT ( 'NONE',  ( 4.286263797015737581E-16, 14.00000000000002487, -149.5231586289125687 ) ) ;
#27687=EDGE_CURVE ( 'NONE', #12520, #29090, #23917, .T. ) ;
#27688=CARTESIAN_POINT ( 'NONE',  ( 3.500000000000000000, 15.47927405783632793, -91.23806413671076143 ) ) ;
#27691=CARTESIAN_POINT ( 'NONE',  ( -3.310556943750000425, 19.41135094264167549, -137.8474391362328220 ) ) ;
#27694=CARTESIAN_POINT ( 'NONE',  ( -1.655278471875002211, 14.63297358603755249, -129.6849391362327992 ) ) ;
#27695=CARTESIAN_POINT ( 'NONE',  ( 3.310556943750001313, 17.50000000000001421, -58.35160580289947063 ) ) ;
#27696=ORIENTED_EDGE ( 'NONE', *, *, #34176, .F. ) ;
#27698=CARTESIAN_POINT ( 'NONE',  ( -7.424026671074350129E-16, 13.45854811567264164, -136.4047308033774186 ) ) ;
#27700=CARTESIAN_POINT ( 'NONE',  ( 3.500000000000001332, 17.50000000000002132, -129.4609808024214885 ) ) ;
#27701=CARTESIAN_POINT ( 'NONE',  ( -7.022189441860112050E-16, 13.67729811471672718, -114.5141058028994792 ) ) ;
#27705=CARTESIAN_POINT ( 'NONE',  ( -3.500000000000002220, 15.47927405783632615, -78.87764746908817415 ) ) ;
#27706=CARTESIAN_POINT ( 'NONE',  ( 4.648177544792955347E-16, 21.00000000000001421, -51.21098080242150274 ) ) ;
#27707=CARTESIAN_POINT ( 'NONE',  ( -3.310556943750002645, 15.58864905735836714, -48.68077246956615056 ) ) ;
#27708=CARTESIAN_POINT ( 'NONE',  ( -3.310556943750000425, 19.41135094264166838, -108.9349391362327992 ) ) ;
#27709=CARTESIAN_POINT ( 'NONE',  ( 4.648177544792955347E-16, 21.00000000000002132, -127.9047308033774186 ) ) ;
#27710=CARTESIAN_POINT ( 'NONE',  ( -1.749999999999999778, 20.53108891324554719, -42.82139747004409713 ) ) ;
#27713=CARTESIAN_POINT ( 'NONE',  ( 1.655278471875001101, 20.36702641396249547, -122.1849391362327992 ) ) ;
#27716=CARTESIAN_POINT ( 'NONE',  ( 3.500000000000001332, 19.52072594216370405, -27.37764746908817770 ) ) ;
#27717=DIRECTION ( 'NONE',  ( 0.000000000000000000, -1.000000000000000000, -3.845925372767130591E-16 ) ) ;
#27718=EDGE_CURVE ( 'NONE', #37225, #34104, #13929, .T. ) ;
#27719=( BOUNDED_CURVE ( )  B_SPLINE_CURVE ( 2, ( #14990, #35172, #5834, #18805, #25197, #25404, #2432, #21994, #31148 ),
 .UNSPECIFIED., .F., .T. ) 
 B_SPLINE_CURVE_WITH_KNOTS ( ( 3, 2, 2, 2, 3 ),
 ( 0.5062499999999999778, 0.5069444444444444198, 0.5083333333333333037, 0.5097222222222221877, 0.5104166666666666297 ),
 .UNSPECIFIED. ) 
 CURVE ( )  GEOMETRIC_REPRESENTATION_ITEM ( )  RATIONAL_B_SPLINE_CURVE ( ( 0.9330127018922194093, 0.9330127018922194093, 1.000000000000000000, 0.8660254037844387076, 1.000000000000000000, 0.8660254037844387076, 1.000000000000000000, 0.9330127018922194093, 0.9330127018922194093 ) ) 
 REPRESENTATION_ITEM ( '' )  );
#27720=CARTESIAN_POINT ( 'NONE',  ( 3.310556943750001313, 19.41135094264166128, -58.26827246956613493 ) ) ;
#27722=ORIENTED_EDGE ( 'NONE', *, *, #10100, .T. ) ;
#27723=CARTESIAN_POINT ( 'NONE',  ( 2.340729813953370519E-16, 21.32270188528331190, -79.10160580289945642 ) ) ;
#27726=CARTESIAN_POINT ( 'NONE',  ( 4.286263797015737581E-16, 14.00000000000002487, -149.5231586289125687 ) ) ;
#27730=CARTESIAN_POINT ( 'NONE',  ( 3.310556943750001313, 17.50000000000001066, -42.26410580289947916 ) ) ;
#27736=CARTESIAN_POINT ( 'NONE',  ( -1.655278471874999990, 20.36702641396248836, -48.93077246956615056 ) ) ;
#27738=ORIENTED_EDGE ( 'NONE', *, *, #4867, .F. ) ;
#27740=CARTESIAN_POINT ( 'NONE',  ( -3.500000000000000888, 19.52072594216370405, -24.04431413575484555 ) ) ;
#27743=CARTESIAN_POINT ( 'NONE',  ( 0.9378221735089300459, 21.00000000000002132, -112.2556390011600342 ) ) ;
#27744=CARTESIAN_POINT ( 'NONE',  ( -3.500000000000000888, 19.52072594216370405, -40.04431413575484555 ) ) ;
#27746=CARTESIAN_POINT ( 'NONE',  ( -0.9378221735089291577, 21.00000000000001776, -77.16632260368298546 ) ) ;
#27747=VECTOR ( 'NONE', #6753, 1000.000000000000000 ) ;
#27748=EDGE_CURVE ( 'NONE', #34171, #31096, #16910, .T. ) ;
#27750=CARTESIAN_POINT ( 'NONE',  ( 3.500000000000000000, 15.47927405783633503, -142.5443141357548313 ) ) ;
#27753=CARTESIAN_POINT ( 'NONE',  ( -3.310556943750000425, 19.41135094264167549, -130.8474391362328220 ) ) ;
#27756=CARTESIAN_POINT ( 'NONE',  ( 1.750000000000001110, 20.53108891324554719, -28.98806413671076143 ) ) ;
#27757=CARTESIAN_POINT ( 'NONE',  ( -7.022189441860112050E-16, 13.67729811471672718, -121.6016058028994706 ) ) ;
#27758=CARTESIAN_POINT ( 'NONE',  ( 0.9378221735089367073, 14.00000000000002487, -134.3600726046389013 ) ) ;
#27759=CARTESIAN_POINT ( 'NONE',  ( 3.500000000000001332, 17.50000000000001066, -39.15473080337743284 ) ) ;
#27762=CARTESIAN_POINT ( 'NONE',  ( 3.500000000000000000, 15.47927405783631727, -25.23806413671075788 ) ) ;
#27763=CARTESIAN_POINT ( 'NONE',  ( 3.500000000000000000, 15.47927405783632437, -68.23806413671076143 ) ) ;
#27764=EDGE_CURVE ( 'NONE', #11372, #13493, #30705, .T. ) ;
#27766=CARTESIAN_POINT ( 'NONE',  ( -3.310556943750002201, 15.58864905735836892, -54.76827246956613493 ) ) ;
#27769=CARTESIAN_POINT ( 'NONE',  ( -7.022189441860112050E-16, 13.67729811471672186, -73.60160580289945642 ) ) ;
#27771=CARTESIAN_POINT ( 'NONE',  ( -1.655278471874999990, 20.36702641396249547, -105.9307724695661364 ) ) ;
#27772=CARTESIAN_POINT ( 'NONE',  ( 3.310556943749999981, 15.58864905735836714, -74.34743913623279354 ) ) ;
#27774=( BOUNDED_CURVE ( )  B_SPLINE_CURVE ( 2, ( #9347, #6152, #8707, #35289, #19131, #5522, #31465, #15954, #2333 ),
 .UNSPECIFIED., .F., .T. ) 
 B_SPLINE_CURVE_WITH_KNOTS ( ( 3, 2, 2, 2, 3 ),
 ( 0.6645833333333333037, 0.6652777777777777457, 0.6666666666666666297, 0.6680555555555555136, 0.6687499999999999556 ),
 .UNSPECIFIED. ) 
 CURVE ( )  GEOMETRIC_REPRESENTATION_ITEM ( )  RATIONAL_B_SPLINE_CURVE ( ( 0.9330127018922194093, 0.9330127018922194093, 1.000000000000000000, 0.8660254037844387076, 1.000000000000000000, 0.8660254037844387076, 1.000000000000000000, 0.9330127018922194093, 0.9330127018922194093 ) ) 
 REPRESENTATION_ITEM ( '' )  );
#27775=CARTESIAN_POINT ( 'NONE',  ( -1.655278471875002211, 14.63297358603754894, -98.68493913623279923 ) ) ;
#27776=EDGE_CURVE ( 'NONE', #8868, #3345, #1573, .T. ) ;
#27778=CARTESIAN_POINT ( 'NONE',  ( -1.750000000000002220, 14.46891108675448301, -85.48806413671076143 ) ) ;
#27780=CYLINDRICAL_SURFACE ( 'NONE', #25277, 3.499999999999999556 ) ;
#27781=CARTESIAN_POINT ( 'NONE',  ( -1.655278471875002211, 14.63297358603754361, -56.59743913623280065 ) ) ;
#27783=CARTESIAN_POINT ( 'NONE',  ( -3.310556943750000425, 19.41135094264166838, -112.8474391362328078 ) ) ;
#27788=VERTEX_POINT ( 'NONE', #7957 ) ;
#27789=LINE ( 'NONE', #27381, #32080 ) ;
#27790=CARTESIAN_POINT ( 'NONE',  ( -1.655278471874999990, 20.36702641396248836, -60.93077246956614346 ) ) ;
#27791=ORIENTED_EDGE ( 'NONE', *, *, #30117, .F. ) ;
#27793=CARTESIAN_POINT ( 'NONE',  ( -3.500000000000000000, 19.52072594216371115, -87.04431413575484555 ) ) ;
#27794=AXIS2_PLACEMENT_3D ( 'NONE', #13789, #26768, #10603 ) ;
#27795=CARTESIAN_POINT ( 'NONE',  ( -2.324088772396477673E-16, 14.00000000000002309, -142.4047308033774186 ) ) ;
#27801=CARTESIAN_POINT ( 'NONE',  ( -7.022189441860112050E-16, 13.67729811471672896, -132.5141058028994507 ) ) ;
#27802=CARTESIAN_POINT ( 'NONE',  ( 0.9378221735089300459, 21.00000000000002132, -119.2556390011600200 ) ) ;
#27803=CARTESIAN_POINT ( 'NONE',  ( 1.655278471875001101, 20.36702641396248481, -38.18493913623280633 ) ) ;
#27804=CARTESIAN_POINT ( 'NONE',  ( 2.340729813953370519E-16, 21.32270188528330479, -31.10160580289945642 ) ) ;
#27805=CARTESIAN_POINT ( 'NONE',  ( -1.655278471875002211, 14.63297358603754716, -90.68493913623279923 ) ) ;
#27806=CARTESIAN_POINT ( 'NONE',  ( 3.500000000000000000, 15.47927405783631727, -24.23806413671077209 ) ) ;
#27807=EDGE_LOOP ( 'NONE', ( #20524, #22035, #1757, #33102 ) ) ;
#27810=CARTESIAN_POINT ( 'NONE',  ( -1.655278471874999990, 20.36702641396249902, -139.0182724695661420 ) ) ;
#27812=CARTESIAN_POINT ( 'NONE',  ( 3.500000000000001776, 19.52072594216371115, -98.37764746908817415 ) ) ;
#27813=CARTESIAN_POINT ( 'NONE',  ( 3.310556943749999981, 15.58864905735836537, -58.34743913623280775 ) ) ;
#27815=CARTESIAN_POINT ( 'NONE',  ( 2.474675557024783212E-16, 21.54145188432739744, -83.90473080337743284 ) ) ;
#27816=EDGE_CURVE ( 'NONE', #8481, #16409, #1155, .T. ) ;
#27817=CARTESIAN_POINT ( 'NONE',  ( 3.310556943749999981, 15.58864905735836714, -69.43493913623279923 ) ) ;
#27819=CARTESIAN_POINT ( 'NONE',  ( 3.500000000000001332, 19.52072594216371115, -84.07139747004411845 ) ) ;
#27820=DIRECTION ( 'NONE',  ( -0.000000000000000000, 1.259100132267607459E-16, -1.000000000000000000 ) ) ;
#27821=CARTESIAN_POINT ( 'NONE',  ( 3.500000000000001332, 17.50000000000001421, -50.46098080242150985 ) ) ;
#27822=CARTESIAN_POINT ( 'NONE',  ( -3.310556943750002201, 15.58864905735837780, -120.6807724695661506 ) ) ;
#27823=FACE_OUTER_BOUND ( 'NONE', #40240, .T. ) ;
#27826=CARTESIAN_POINT ( 'NONE',  ( -3.500000000000002220, 15.47927405783633503, -114.5713974700440900 ) ) ;
#27827=LINE ( 'NONE', #1471, #12440 ) ;
#27828=CARTESIAN_POINT ( 'NONE',  ( -1.394453263437886604E-15, 14.00000000000001066, -39.40473080337742573 ) ) ;
#27832=CARTESIAN_POINT ( 'NONE',  ( 1.655278471875001101, 20.36702641396248836, -73.09743913623280775 ) ) ;
#27833=CARTESIAN_POINT ( 'NONE',  ( -0.9378221735089291577, 21.00000000000002487, -134.1663226036829712 ) ) ;
#27834=CARTESIAN_POINT ( 'NONE',  ( 3.500000000000001332, 19.52072594216370760, -72.37764746908817415 ) ) ;
#27835=ORIENTED_EDGE ( 'NONE', *, *, #37565, .T. ) ;
#27836=CARTESIAN_POINT ( 'NONE',  ( -3.500000000000002220, 15.47927405783633503, -132.8776474690881741 ) ) ;
#27837=CARTESIAN_POINT ( 'NONE',  ( 4.648177544792955347E-16, 21.00000000000001066, -25.21098080242150985 ) ) ;
#27838=CARTESIAN_POINT ( 'NONE',  ( -3.310556943750002645, 15.58864905735837070, -77.68077246956615056 ) ) ;
#27840=ORIENTED_EDGE ( 'NONE', *, *, #30117, .T. ) ;
#27844=CARTESIAN_POINT ( 'NONE',  ( 0.9378221735089367073, 14.00000000000002487, -129.3600726046389013 ) ) ;
#27846=LINE ( 'NONE', #4882, #33616 ) ;
#27847=CARTESIAN_POINT ( 'NONE',  ( 3.310556943750001313, 17.50000000000001421, -48.35160580289946353 ) ) ;
#27848=CARTESIAN_POINT ( 'NONE',  ( 3.310556943750001313, 19.41135094264166838, -111.2682724695661278 ) ) ;
#27849=ORIENTED_EDGE ( 'NONE', *, *, #41506, .T. ) ;
#27850=CARTESIAN_POINT ( 'NONE',  ( -3.310556943750000425, 19.41135094264165772, -33.84743913623280775 ) ) ;
#27851=CARTESIAN_POINT ( 'NONE',  ( -3.310556943750000425, 19.41135094264166128, -58.93493913623279212 ) ) ;
#27852=CARTESIAN_POINT ( 'NONE',  ( 3.500000000000001332, 17.50000000000002132, -113.4609808024215027 ) ) ;
#27854=CARTESIAN_POINT ( 'NONE',  ( -1.655278471875002211, 14.63297358603754894, -97.59743913623280775 ) ) ;
#27855=EDGE_CURVE ( 'NONE', #21422, #33769, #37301, .T. ) ;
#27858=CARTESIAN_POINT ( 'NONE',  ( -3.500000000000000888, 19.52072594216370760, -66.04431413575484555 ) ) ;
#27861=CARTESIAN_POINT ( 'NONE',  ( 1.655278471874998436, 14.63297358603753828, -34.43077246956615056 ) ) ;
#27862=CARTESIAN_POINT ( 'NONE',  ( -3.500000000000001332, 17.50000000000001421, -56.65473080337743284 ) ) ;
#27863=CARTESIAN_POINT ( 'NONE',  ( -3.500000000000002220, 15.47927405783633503, -137.8776474690881741 ) ) ;
#27864=CARTESIAN_POINT ( 'NONE',  ( -3.310556943750001313, 17.50000000000002132, -107.8516058028994564 ) ) ;
#27865=CARTESIAN_POINT ( 'NONE',  ( -3.310556943750001313, 17.50000000000001066, -36.85160580289946353 ) ) ;
#27871=DIRECTION ( 'NONE',  ( -0.000000000000000000, 1.259100132267607459E-16, -1.000000000000000000 ) ) ;
#27873=CARTESIAN_POINT ( 'NONE',  ( 3.310556943750001313, 19.41135094264166838, -85.18077246956613635 ) ) ;
#27876=ORIENTED_EDGE ( 'NONE', *, *, #21699, .F. ) ;
#27878=CARTESIAN_POINT ( 'NONE',  ( 4.648177544792955347E-16, 21.00000000000001421, -50.90473080337743284 ) ) ;
#27879=ORIENTED_EDGE ( 'NONE', *, *, #26395, .T. ) ;
#27881=CARTESIAN_POINT ( 'NONE',  ( -0.9378221735089310451, 14.00000000000001066, -30.75563900116002358 ) ) ;
#27884=VERTEX_POINT ( 'NONE', #17321 ) ;
#27885=CARTESIAN_POINT ( 'NONE',  ( 1.750000000000001110, 20.53108891324555785, -117.9880641367107614 ) ) ;
#27886=ORIENTED_EDGE ( 'NONE', *, *, #40135, .T. ) ;
#27887=( BOUNDED_CURVE ( )  B_SPLINE_CURVE ( 2, ( #24373, #41163, #40731, #33939, #21169, #21378, #31371, #27967, #24582 ),
 .UNSPECIFIED., .F., .T. ) 
 B_SPLINE_CURVE_WITH_KNOTS ( ( 3, 2, 2, 2, 3 ),
 ( 0.2312500000000000111, 0.2319444444444444531, 0.2333333333333333370, 0.2347222222222222210, 0.2354166666666666630 ),
 .UNSPECIFIED. ) 
 CURVE ( )  GEOMETRIC_REPRESENTATION_ITEM ( )  RATIONAL_B_SPLINE_CURVE ( ( 0.9330127018922194093, 0.9330127018922194093, 1.000000000000000000, 0.8660254037844387076, 1.000000000000000000, 0.8660254037844387076, 1.000000000000000000, 0.9330127018922194093, 0.9330127018922194093 ) ) 
 REPRESENTATION_ITEM ( '' )  );
#27888=( BOUNDED_CURVE ( )  B_SPLINE_CURVE ( 2, ( #19446, #28797, #22422, #16266, #6880, #38590, #31776, #29420, #39007 ),
 .UNSPECIFIED., .F., .F. ) 
 B_SPLINE_CURVE_WITH_KNOTS ( ( 3, 2, 2, 2, 3 ),
 ( 0.1770833333333333426, 0.1777777777777777846, 0.1791666666666666685, 0.1805555555555555525, 0.1812499999999999944 ),
 .UNSPECIFIED. ) 
 CURVE ( )  GEOMETRIC_REPRESENTATION_ITEM ( )  RATIONAL_B_SPLINE_CURVE ( ( 0.9330127018922194093, 0.9330127018922194093, 1.000000000000000000, 0.8660254037844387076, 1.000000000000000000, 0.8660254037844387076, 1.000000000000000000, 0.9330127018922194093, 0.9330127018922194093 ) ) 
 REPRESENTATION_ITEM ( '' )  );
#27893=ORIENTED_EDGE ( 'NONE', *, *, #41506, .F. ) ;
#27897=CARTESIAN_POINT ( 'NONE',  ( 2.340729813953370519E-16, 21.32270188528332255, -139.0141058028994792 ) ) ;
#27898=CARTESIAN_POINT ( 'NONE',  ( 0.000000000000000000, 17.50000000000002487, -149.5231586289125687 ) ) ;
#27900=CARTESIAN_POINT ( 'NONE',  ( -3.500000000000001332, 17.50000000000001066, -26.65473080337743639 ) ) ;
#27901=CARTESIAN_POINT ( 'NONE',  ( 1.655278471874998436, 14.63297358603755072, -127.5182724695661278 ) ) ;
#27902=CARTESIAN_POINT ( 'NONE',  ( 3.310556943750001313, 19.41135094264166128, -53.26827246956612072 ) ) ;
#27903=ORIENTED_EDGE ( 'NONE', *, *, #7441, .T. ) ;
#27904=ADVANCED_FACE ( 'NONE', ( #10716 ), #21130, .T. ) ;
#27906=CARTESIAN_POINT ( 'NONE',  ( 3.500000000000001776, 19.52072594216372181, -135.0713974700441042 ) ) ;
#27909=CARTESIAN_POINT ( 'NONE',  ( 1.655278471874998436, 14.63297358603754539, -83.51827246956614204 ) ) ;
#27910=CARTESIAN_POINT ( 'NONE',  ( -1.749999999999999778, 20.53108891324555785, -127.1276474690881741 ) ) ;
#27911=CARTESIAN_POINT ( 'NONE',  ( 2.340729813953370519E-16, 21.32270188528331900, -115.0141058028994934 ) ) ;
#27915=CARTESIAN_POINT ( 'NONE',  ( -7.424026671074350129E-16, 13.45854811567263454, -78.71098080242150274 ) ) ;
#27917=CARTESIAN_POINT ( 'NONE',  ( 1.655278471875001101, 20.36702641396248836, -48.09743913623280775 ) ) ;
#27918=CARTESIAN_POINT ( 'NONE',  ( -3.310556943750002645, 15.58864905735837425, -106.7682724695661278 ) ) ;
#27919=CARTESIAN_POINT ( 'NONE',  ( -3.500000000000002220, 15.47927405783633503, -130.5713974700441042 ) ) ;
#27921=LINE ( 'NONE', #40895, #14834 ) ;
#27922=CARTESIAN_POINT ( 'NONE',  ( 3.310556943749999981, 15.58864905735837425, -125.4349391362327992 ) ) ;
#27926=CARTESIAN_POINT ( 'NONE',  ( 0.9378221735089281585, 14.00000000000001243, -60.66632260368298546 ) ) ;
#27927=CARTESIAN_POINT ( 'NONE',  ( -1.394453263437886604E-15, 14.00000000000002132, -115.4047308033774186 ) ) ;
#27928=CARTESIAN_POINT ( 'NONE',  ( -3.310556943750000425, 19.41135094264166128, -60.93493913623279923 ) ) ;
#27930=ORIENTED_EDGE ( 'NONE', *, *, #32501, .T. ) ;
#27931=CARTESIAN_POINT ( 'NONE',  ( -1.655278471874999990, 20.36702641396249192, -75.01827246956612782 ) ) ;
#27933=DIRECTION ( 'NONE',  ( -0.000000000000000000, 1.259100132267607459E-16, -1.000000000000000000 ) ) ;
#27934=CARTESIAN_POINT ( 'NONE',  ( 0.9378221735089300459, 21.00000000000001776, -76.94938900211595012 ) ) ;
#27935=CARTESIAN_POINT ( 'NONE',  ( 0.9378221735089300459, 21.00000000000001776, -98.94938900211596433 ) ) ;
#27937=CARTESIAN_POINT ( 'NONE',  ( -3.310556943750001313, 17.50000000000001066, -37.76410580289947205 ) ) ;
#27938=CARTESIAN_POINT ( 'NONE',  ( -3.500000000000001332, 17.50000000000001776, -93.65473080337743284 ) ) ;
#27939=ORIENTED_EDGE ( 'NONE', *, *, #33630, .F. ) ;
#27944=CARTESIAN_POINT ( 'NONE',  ( -3.310556943750000425, 19.41135094264165772, -44.84743913623280775 ) ) ;
#27945=EDGE_CURVE ( 'NONE', #8739, #35536, #3866, .T. ) ;
#27948=CARTESIAN_POINT ( 'NONE',  ( 0.9378221735089281585, 14.00000000000001243, -56.36007260463890844 ) ) ;
#27950=CARTESIAN_POINT ( 'NONE',  ( -1.394453263437886604E-15, 14.00000000000002132, -113.4047308033774186 ) ) ;
#27951=CARTESIAN_POINT ( 'NONE',  ( 0.9378221735089281585, 14.00000000000002132, -112.6663226036829712 ) ) ;
#27952=CARTESIAN_POINT ( 'NONE',  ( -1.749999999999999778, 20.53108891324554719, -38.12764746908817415 ) ) ;
#27953=DIRECTION ( 'NONE',  ( 0.000000000000000000, 1.000000000000000000, 0.000000000000000000 ) ) ;
#27954=CARTESIAN_POINT ( 'NONE',  ( -3.500000000000002220, 15.47927405783632793, -76.87764746908817415 ) ) ;
#27955=ADVANCED_FACE ( 'NONE', ( #41121 ), #37413, .T. ) ;
#27957=CARTESIAN_POINT ( 'NONE',  ( 1.655278471874998436, 14.63297358603753651, -23.51827246956612782 ) ) ;
#27958=CARTESIAN_POINT ( 'NONE',  ( -1.394453263437886604E-15, 14.00000000000001776, -94.71098080242150274 ) ) ;
#27959=CARTESIAN_POINT ( 'NONE',  ( 3.310556943750001313, 17.50000000000002132, -127.2641058028994792 ) ) ;
#27962=( BOUNDED_CURVE ( )  B_SPLINE_CURVE ( 2, ( #35667, #134, #13116, #26099, #25682, #39254, #19915, #26308, #28852 ),
 .UNSPECIFIED., .F., .F. ) 
 B_SPLINE_CURVE_WITH_KNOTS ( ( 3, 2, 2, 2, 3 ),
 ( 0.4187500000000000111, 0.4194444444444444531, 0.4208333333333333370, 0.4222222222222222210, 0.4229166666666666630 ),
 .UNSPECIFIED. ) 
 CURVE ( )  GEOMETRIC_REPRESENTATION_ITEM ( )  RATIONAL_B_SPLINE_CURVE ( ( 0.9330127018922194093, 0.9330127018922194093, 1.000000000000000000, 0.8660254037844387076, 1.000000000000000000, 0.8660254037844387076, 1.000000000000000000, 0.9330127018922194093, 0.9330127018922194093 ) ) 
 REPRESENTATION_ITEM ( '' )  );
#27963=CARTESIAN_POINT ( 'NONE',  ( -1.394453263437886604E-15, 14.00000000000000711, -25.40473080337742928 ) ) ;
#27965=CARTESIAN_POINT ( 'NONE',  ( -1.655278471875002211, 14.63297358603755072, -120.6849391362327992 ) ) ;
#27966=CARTESIAN_POINT ( 'NONE',  ( -3.500000000000000888, 19.52072594216370405, -36.73806413671076854 ) ) ;
#27967=CARTESIAN_POINT ( 'NONE',  ( 0.9378221735089300459, 21.00000000000002132, -114.9493890021159359 ) ) ;
#27969=CARTESIAN_POINT ( 'NONE',  ( -7.022189441860112050E-16, 13.67729811471673074, -139.6016058028994564 ) ) ;
#27971=CARTESIAN_POINT ( 'NONE',  ( 3.310556943750001313, 17.50000000000001421, -48.35160580289946353 ) ) ;
#27974=CARTESIAN_POINT ( 'NONE',  ( -3.310556943750000425, 19.41135094264166128, -72.93493913623278502 ) ) ;
#27976=CARTESIAN_POINT ( 'NONE',  ( 3.310556943750001313, 17.50000000000002132, -105.2641058028994649 ) ) ;
#27977=CARTESIAN_POINT ( 'NONE',  ( -3.310556943750002645, 15.58864905735837070, -71.68077246956613635 ) ) ;
#27979=CARTESIAN_POINT ( 'NONE',  ( -3.310556943750002201, 15.58864905735837247, -88.76827246956612782 ) ) ;
#27984=CARTESIAN_POINT ( 'NONE',  ( 4.648177544792955347E-16, 21.00000000000001776, -94.90473080337743284 ) ) ;
#27985=CARTESIAN_POINT ( 'NONE',  ( -3.310556943750001313, 17.50000000000001421, -54.76410580289947916 ) ) ;
#27987=CARTESIAN_POINT ( 'NONE',  ( -0.9378221735089291577, 21.00000000000001066, -24.86007260463890844 ) ) ;
#27988=CARTESIAN_POINT ( 'NONE',  ( 3.310556943750001313, 17.50000000000002132, -112.2641058028994792 ) ) ;
#27991=EDGE_CURVE ( 'NONE', #23881, #34688, #28326, .T. ) ;
#27993=ORIENTED_EDGE ( 'NONE', *, *, #5845, .F. ) ;
#27995=CARTESIAN_POINT ( 'NONE',  ( 1.655278471875001101, 20.36702641396248836, -65.09743913623280775 ) ) ;
#27997=VERTEX_POINT ( 'NONE', #1974 ) ;
#27999=DIRECTION ( 'NONE',  ( -0.000000000000000000, 1.259100132267607459E-16, -1.000000000000000000 ) ) ;
#28002=ORIENTED_EDGE ( 'NONE', *, *, #30240, .F. ) ;
#28004=CARTESIAN_POINT ( 'NONE',  ( 4.648177544792955347E-16, 21.00000000000002487, -134.2109808024215170 ) ) ;
#28005=CARTESIAN_POINT ( 'NONE',  ( -3.310556943750002201, 15.58864905735837780, -131.6807724695661364 ) ) ;
#28007=EDGE_CURVE ( 'NONE', #16704, #18479, #11210, .T. ) ;
#28009=CARTESIAN_POINT ( 'NONE',  ( -1.655278471874999990, 20.36702641396248481, -41.01827246956612782 ) ) ;
#28010=CARTESIAN_POINT ( 'NONE',  ( 3.310556943750001313, 19.41135094264165772, -35.26827246956613493 ) ) ;
#28012=CARTESIAN_POINT ( 'NONE',  ( -1.655278471874999990, 20.36702641396249192, -93.01827246956612782 ) ) ;
#28013=CARTESIAN_POINT ( 'NONE',  ( -1.750000000000002220, 14.46891108675447413, -24.48806413671077209 ) ) ;
#28014=ORIENTED_EDGE ( 'NONE', *, *, #38419, .T. ) ;
#28015=VECTOR ( 'NONE', #2051, 1000.000000000000000 ) ;
#28017=CARTESIAN_POINT ( 'NONE',  ( -3.310556943750001313, 17.50000000000002487, -136.8516058028994564 ) ) ;
#28018=CARTESIAN_POINT ( 'NONE',  ( 4.648177544792955347E-16, 21.00000000000001066, -40.21098080242150274 ) ) ;
#28020=CARTESIAN_POINT ( 'NONE',  ( -1.655278471874999990, 20.36702641396248836, -57.93077246956614346 ) ) ;
#28021=CARTESIAN_POINT ( 'NONE',  ( 1.750000000000001110, 20.53108891324555429, -94.98806413671076143 ) ) ;
#28022=CARTESIAN_POINT ( 'NONE',  ( -1.750000000000002220, 14.46891108675448301, -87.48806413671076143 ) ) ;
#28023=CARTESIAN_POINT ( 'NONE',  ( -3.310556943750001313, 17.50000000000001421, -65.85160580289945642 ) ) ;
#28026=CARTESIAN_POINT ( 'NONE',  ( -3.500000000000001332, 17.50000000000001421, -58.65473080337743284 ) ) ;
#28027=CARTESIAN_POINT ( 'NONE',  ( -7.424026671074350129E-16, 13.45854811567263276, -49.71098080242150274 ) ) ;
#28028=CARTESIAN_POINT ( 'NONE',  ( -3.310556943750000425, 19.41135094264166838, -118.8474391362327935 ) ) ;
#28032=CARTESIAN_POINT ( 'NONE',  ( -7.424026671074350129E-16, 13.45854811567263987, -111.4047308033774328 ) ) ;
#28037=CARTESIAN_POINT ( 'NONE',  ( -1.655278471875002211, 14.63297358603754539, -71.59743913623280775 ) ) ;
#28038=FACE_OUTER_BOUND ( 'NONE', #14919, .T. ) ;
#28039=DIRECTION ( 'NONE',  ( 0.000000000000000000, 1.000000000000000000, 0.000000000000000000 ) ) ;
#28042=CARTESIAN_POINT ( 'NONE',  ( 1.655278471875001101, 20.36702641396248481, -26.09743913623280420 ) ) ;
#28043=VECTOR ( 'NONE', #27422, 1000.000000000000000 ) ;
#28045=CARTESIAN_POINT ( 'NONE',  ( 2.340729813953370519E-16, 21.32270188528331190, -79.01410580289947916 ) ) ;
#28048=ORIENTED_EDGE ( 'NONE', *, *, #42080, .F. ) ;
#28049=EDGE_CURVE ( 'NONE', #18643, #5754, #5234, .T. ) ;
#28051=DIRECTION ( 'NONE',  ( -0.000000000000000000, 1.259100132267607459E-16, -1.000000000000000000 ) ) ;
#28052=ORIENTED_EDGE ( 'NONE', *, *, #23847, .F. ) ;
#28053=CARTESIAN_POINT ( 'NONE',  ( -8.715332896486792803E-15, 21.00000000000002842, -138.2109808024214885 ) ) ;
#28054=CARTESIAN_POINT ( 'NONE',  ( -7.022189441860112050E-16, 13.67729811471671653, -49.60160580289946353 ) ) ;
#28055=CARTESIAN_POINT ( 'NONE',  ( 2.340729813953370519E-16, 21.32270188528331900, -108.1016058028994706 ) ) ;
#28056=ORIENTED_EDGE ( 'NONE', *, *, #2372, .T. ) ;
#28057=CARTESIAN_POINT ( 'NONE',  ( 3.310556943749999981, 15.58864905735836182, -32.34743913623280775 ) ) ;
#28058=AXIS2_PLACEMENT_3D ( 'NONE', #21497, #34468, #5328 ) ;
#28059=CARTESIAN_POINT ( 'NONE',  ( 1.655278471875001101, 20.36702641396248836, -62.18493913623279923 ) ) ;
#28060=CARTESIAN_POINT ( 'NONE',  ( 3.500000000000000000, 15.47927405783632970, -110.5443141357548456 ) ) ;
#28062=CARTESIAN_POINT ( 'NONE',  ( 3.310556943750001313, 17.50000000000001776, -96.26410580289946495 ) ) ;
#28064=CARTESIAN_POINT ( 'NONE',  ( -3.500000000000000000, 19.52072594216370405, -26.04431413575483845 ) ) ;
#28068=CARTESIAN_POINT ( 'NONE',  ( -3.500000000000002220, 15.47927405783632437, -66.87764746908817415 ) ) ;
#28070=CARTESIAN_POINT ( 'NONE',  ( -1.655278471875002211, 14.63297358603753828, -24.59743913623281486 ) ) ;
#28071=CARTESIAN_POINT ( 'NONE',  ( -3.500000000000002220, 15.47927405783632260, -52.57139747004409713 ) ) ;
#28073=CARTESIAN_POINT ( 'NONE',  ( -3.310556943750002201, 15.58864905735837425, -106.7682724695661278 ) ) ;
#28075=CARTESIAN_POINT ( 'NONE',  ( 2.340729813953370519E-16, 21.32270188528330834, -38.10160580289946353 ) ) ;
#28079=CARTESIAN_POINT ( 'NONE',  ( -7.460324959392693302E-14, 21.00000000000001776, -88.21098080242150274 ) ) ;
#28081=CARTESIAN_POINT ( 'NONE',  ( 1.655278471874998436, 14.63297358603754539, -86.43077246956613635 ) ) ;
#28082=( BOUNDED_CURVE ( )  B_SPLINE_CURVE ( 2, ( #13658, #22817, #32792, #16442, #23228, #13245, #35987, #10058, #26855 ),
 .UNSPECIFIED., .F., .T. ) 
 B_SPLINE_CURVE_WITH_KNOTS ( ( 3, 2, 2, 2, 3 ),
 ( 0.1604166666666666796, 0.1611111111111111216, 0.1625000000000000056, 0.1638888888888888895, 0.1645833333333333315 ),
 .UNSPECIFIED. ) 
 CURVE ( )  GEOMETRIC_REPRESENTATION_ITEM ( )  RATIONAL_B_SPLINE_CURVE ( ( 0.9330127018922194093, 0.9330127018922207416, 1.000000000000000000, 0.8660254037844387076, 1.000000000000000000, 0.8660254037844387076, 1.000000000000000000, 0.9330127018922194093, 0.9330127018922194093 ) ) 
 REPRESENTATION_ITEM ( '' )  );
#28087=CARTESIAN_POINT ( 'NONE',  ( -3.500000000000000000, 19.52072594216371115, -102.0443141357548456 ) ) ;
#28088=CARTESIAN_POINT ( 'NONE',  ( -3.500000000000001332, 17.50000000000001421, -50.65473080337742573 ) ) ;
#28094=CARTESIAN_POINT ( 'NONE',  ( -3.500000000000001332, 17.50000000000001776, -78.65473080337743284 ) ) ;
#28102=ORIENTED_EDGE ( 'NONE', *, *, #22775, .T. ) ;
#28103=CARTESIAN_POINT ( 'NONE',  ( 4.648177544792955347E-16, 21.00000000000001776, -90.90473080337741862 ) ) ;
#28104=DIRECTION ( 'NONE',  ( -0.000000000000000000, 1.259100132267607459E-16, -1.000000000000000000 ) ) ;
#28105=CARTESIAN_POINT ( 'NONE',  ( -7.022189441860112050E-16, 13.67729811471672896, -137.5141058028994507 ) ) ;
#28107=ORIENTED_EDGE ( 'NONE', *, *, #30881, .T. ) ;
#28108=CARTESIAN_POINT ( 'NONE',  ( 1.750000000000001110, 20.53108891324555429, -101.2943141357548456 ) ) ;
#28109=CARTESIAN_POINT ( 'NONE',  ( -7.022189441860112050E-16, 13.67729811471672718, -125.6016058028994706 ) ) ;
#28110=CARTESIAN_POINT ( 'NONE',  ( 3.310556943750001313, 19.41135094264166128, -55.26827246956612782 ) ) ;
#28111=ORIENTED_EDGE ( 'NONE', *, *, #7073, .T. ) ;
#28113=CARTESIAN_POINT ( 'NONE',  ( -7.424026671074350129E-16, 13.45854811567264164, -138.4047308033774186 ) ) ;
#28116=CARTESIAN_POINT ( 'NONE',  ( -3.310556943750000425, 19.41135094264166483, -74.93493913623279923 ) ) ;
#28117=CARTESIAN_POINT ( 'NONE',  ( 3.500000000000000000, 15.47927405783633503, -128.5443141357548313 ) ) ;
#28118=CARTESIAN_POINT ( 'NONE',  ( 3.310556943750001313, 19.41135094264166838, -115.1807724695661364 ) ) ;
#28122=CARTESIAN_POINT ( 'NONE',  ( 3.500000000000001332, 17.50000000000001776, -79.46098080242150274 ) ) ;
#28124=CARTESIAN_POINT ( 'NONE',  ( -7.022189441860112050E-16, 13.67729811471671653, -45.51410580289947205 ) ) ;
#28125=CARTESIAN_POINT ( 'NONE',  ( -1.655278471875002211, 14.63297358603754894, -99.68493913623279923 ) ) ;
#28126=CARTESIAN_POINT ( 'NONE',  ( -0.9378221735089291577, 21.00000000000002487, -130.1663226036829712 ) ) ;
#28128=CARTESIAN_POINT ( 'NONE',  ( -3.500000000000001332, 17.50000000000001776, -99.65473080337743284 ) ) ;
#28129=CARTESIAN_POINT ( 'NONE',  ( -3.500000000000002220, 15.47927405783632793, -72.57139747004409003 ) ) ;
#28130=CARTESIAN_POINT ( 'NONE',  ( -3.310556943750000425, 19.41135094264166838, -122.9349391362327992 ) ) ;
#28134=CARTESIAN_POINT ( 'NONE',  ( 4.648177544792955347E-16, 21.00000000000001421, -50.21098080242150985 ) ) ;
#28138=( BOUNDED_CURVE ( )  B_SPLINE_CURVE ( 2, ( #29642, #26052, #41802, #26262, #29015, #9461, #19245, #3082, #13478 ),
 .UNSPECIFIED., .F., .F. ) 
 B_SPLINE_CURVE_WITH_KNOTS ( ( 3, 2, 2, 2, 3 ),
 ( 0.6354166666666666297, 0.6361111111111110716, 0.6374999999999999556, 0.6388888888888888395, 0.6395833333333332815 ),
 .UNSPECIFIED. ) 
 CURVE ( )  GEOMETRIC_REPRESENTATION_ITEM ( )  RATIONAL_B_SPLINE_CURVE ( ( 0.9330127018922194093, 0.9330127018922194093, 1.000000000000000000, 0.8660254037844387076, 1.000000000000000000, 0.8660254037844387076, 1.000000000000000000, 0.9330127018922194093, 0.9330127018922194093 ) ) 
 REPRESENTATION_ITEM ( '' )  );
#28139=CARTESIAN_POINT ( 'NONE',  ( 2.340729813953370519E-16, 21.32270188528331190, -74.10160580289947063 ) ) ;
#28141=CARTESIAN_POINT ( 'NONE',  ( 0.9378221735089300459, 21.00000000000001776, -79.94938900211593591 ) ) ;
#28145=CARTESIAN_POINT ( 'NONE',  ( -3.310556943750001313, 17.50000000000001066, -39.76410580289947916 ) ) ;
#28146=CARTESIAN_POINT ( 'NONE',  ( 3.310556943750001313, 17.50000000000001066, -23.30785580289947134 ) ) ;
#28148=ORIENTED_EDGE ( 'NONE', *, *, #23796, .T. ) ;
#28150=CARTESIAN_POINT ( 'NONE',  ( -1.655278471874999990, 20.36702641396248481, -45.93077246956614346 ) ) ;
#28154=DIRECTION ( 'NONE',  ( 0.000000000000000000, 1.000000000000000000, 0.000000000000000000 ) ) ;
#28157=CARTESIAN_POINT ( 'NONE',  ( 1.749999999999998224, 14.46891108675448301, -97.62764746908817415 ) ) ;
#28158=FACE_OUTER_BOUND ( 'NONE', #9271, .T. ) ;
#28159=CARTESIAN_POINT ( 'NONE',  ( -3.500000000000000888, 19.52072594216370405, -39.04431413575484555 ) ) ;
#28160=CARTESIAN_POINT ( 'NONE',  ( 0.000000000000000000, 17.50000000000002487, -149.5231586289125687 ) ) ;
#28162=CARTESIAN_POINT ( 'NONE',  ( -1.394453263437886604E-15, 14.00000000000001421, -64.40473080337743284 ) ) ;
#28164=EDGE_CURVE ( 'NONE', #40609, #29973, #9844, .T. ) ;
#28168=CARTESIAN_POINT ( 'NONE',  ( -1.655278471874999990, 20.36702641396248481, -25.01827246956613138 ) ) ;
#28170=CARTESIAN_POINT ( 'NONE',  ( 2.340729813953370519E-16, 21.32270188528331900, -128.0141058028994792 ) ) ;
#28174=CARTESIAN_POINT ( 'NONE',  ( 1.655278471875001101, 20.36702641396249547, -121.1849391362327992 ) ) ;
#28176=CARTESIAN_POINT ( 'NONE',  ( -7.424026671074350129E-16, 13.45854811567263098, -37.40473080337743284 ) ) ;
#28179=CARTESIAN_POINT ( 'NONE',  ( 3.310556943749999981, 15.58864905735837780, -139.4349391362327708 ) ) ;
#28180=DIRECTION ( 'NONE',  ( 0.000000000000000000, 1.000000000000000000, 0.000000000000000000 ) ) ;
#28181=CARTESIAN_POINT ( 'NONE',  ( -3.310556943750002201, 15.58864905735836714, -50.76827246956612782 ) ) ;
#28184=CARTESIAN_POINT ( 'NONE',  ( 1.655278471874998436, 14.63297358603754361, -72.51827246956612782 ) ) ;
#28186=CARTESIAN_POINT ( 'NONE',  ( 2.340729813953370519E-16, 21.32270188528331900, -103.0141058028994792 ) ) ;
#28187=CARTESIAN_POINT ( 'NONE',  ( 3.310556943750001313, 19.41135094264166128, -70.18077246956613635 ) ) ;
#28189=CARTESIAN_POINT ( 'NONE',  ( 3.310556943750001313, 19.41135094264166838, -92.26827246956612782 ) ) ;
#28193=CARTESIAN_POINT ( 'NONE',  ( 3.310556943750001313, 19.41135094264166483, -57.18077246956614346 ) ) ;
#28195=CARTESIAN_POINT ( 'NONE',  ( -3.500000000000001332, 17.50000000000002487, -137.6547308033774186 ) ) ;
#28196=CARTESIAN_POINT ( 'NONE',  ( -1.655278471874999990, 20.36702641396249547, -112.9307724695661364 ) ) ;
#28199=VERTEX_POINT ( 'NONE', #26214 ) ;
#28200=ORIENTED_EDGE ( 'NONE', *, *, #34250, .T. ) ;
#28205=CARTESIAN_POINT ( 'NONE',  ( -3.310556943750002645, 15.58864905735836892, -63.68077246956615056 ) ) ;
#28207=VERTEX_POINT ( 'NONE', #23005 ) ;
#28212=ORIENTED_EDGE ( 'NONE', *, *, #40502, .F. ) ;
#28214=CARTESIAN_POINT ( 'NONE',  ( 2.340729813953370519E-16, 21.32270188528332255, -133.0141058028994507 ) ) ;
#28215=EDGE_CURVE ( 'NONE', #39933, #31404, #26982, .T. ) ;
#28216=CARTESIAN_POINT ( 'NONE',  ( -3.500000000000000000, 19.52072594216371826, -128.7380641367107614 ) ) ;
#28218=CARTESIAN_POINT ( 'NONE',  ( -3.310556943750000425, 19.41135094264165772, -38.93493913623280633 ) ) ;
#28219=CARTESIAN_POINT ( 'NONE',  ( 2.340729813953370519E-16, 21.32270188528330479, -34.10160580289946353 ) ) ;
#28220=CARTESIAN_POINT ( 'NONE',  ( 2.340729813953370519E-16, 21.32270188528331190, -91.10160580289947063 ) ) ;
#28221=CARTESIAN_POINT ( 'NONE',  ( -7.424026671074350129E-16, 13.45854811567263098, -26.40473080337743639 ) ) ;
#28225=CARTESIAN_POINT ( 'NONE',  ( -3.310556943750002645, 15.58864905735837958, -139.7682724695661420 ) ) ;
#28226=VECTOR ( 'NONE', #6948, 1000.000000000000000 ) ;
#28228=CARTESIAN_POINT ( 'NONE',  ( 3.500000000000001332, 19.52072594216371826, -136.0713974700441042 ) ) ;
#28230=CARTESIAN_POINT ( 'NONE',  ( 3.500000000000001332, 17.50000000000001776, -83.15473080337743284 ) ) ;
#28231=CARTESIAN_POINT ( 'NONE',  ( -3.310556943750000425, 19.41135094264166483, -64.93493913623279923 ) ) ;
#28234=CARTESIAN_POINT ( 'NONE',  ( -1.750000000000002220, 14.46891108675448301, -90.79431413575484555 ) ) ;
#28235=CARTESIAN_POINT ( 'NONE',  ( -0.9378221735089291577, 21.00000000000001421, -60.16632260368299256 ) ) ;
#28237=CARTESIAN_POINT ( 'NONE',  ( 3.310556943749999981, 15.58864905735837247, -122.3474391362328362 ) ) ;
#28238=CARTESIAN_POINT ( 'NONE',  ( 3.500000000000001332, 19.52072594216370760, -62.07139747004410424 ) ) ;
#28239=ORIENTED_EDGE ( 'NONE', *, *, #7460, .T. ) ;
#28240=CARTESIAN_POINT ( 'NONE',  ( 3.500000000000001332, 17.50000000000002132, -108.1547308033774186 ) ) ;
#28241=CARTESIAN_POINT ( 'NONE',  ( 4.648177544792955347E-16, 21.00000000000001776, -89.90473080337741862 ) ) ;
#28242=CARTESIAN_POINT ( 'NONE',  ( -0.9378221735089310451, 14.00000000000002132, -82.44938900211595012 ) ) ;
#28243=CARTESIAN_POINT ( 'NONE',  ( 3.500000000000001332, 17.50000000000001421, -61.15473080337742573 ) ) ;
#28246=CARTESIAN_POINT ( 'NONE',  ( 2.340729813953370519E-16, 21.32270188528331190, -73.01410580289947916 ) ) ;
#28247=ADVANCED_FACE ( 'NONE', ( #4707 ), #4069, .T. ) ;
#28250=EDGE_CURVE ( 'NONE', #15095, #27788, #21011, .T. ) ;
#28252=ORIENTED_EDGE ( 'NONE', *, *, #33823, .F. ) ;
#28253=DIRECTION ( 'NONE',  ( -0.000000000000000000, 1.259100132267607459E-16, -1.000000000000000000 ) ) ;
#28254=CARTESIAN_POINT ( 'NONE',  ( 0.000000000000000000, 17.50000000000002487, -149.5231586289125687 ) ) ;
#28255=CARTESIAN_POINT ( 'NONE',  ( 3.310556943750001313, 19.41135094264166483, -81.18077246956615056 ) ) ;
#28259=( BOUNDED_CURVE ( )  B_SPLINE_CURVE ( 2, ( #12635, #28995, #16254, #36004, #3468, #32605, #6871, #13261, #25617 ),
 .UNSPECIFIED., .F., .T. ) 
 B_SPLINE_CURVE_WITH_KNOTS ( ( 3, 2, 2, 2, 3 ),
 ( 0.2062499999999999889, 0.2069444444444444309, 0.2083333333333333426, 0.2097222222222222265, 0.2104166666666666685 ),
 .UNSPECIFIED. ) 
 CURVE ( )  GEOMETRIC_REPRESENTATION_ITEM ( )  RATIONAL_B_SPLINE_CURVE ( ( 0.9330127018922194093, 0.9330127018922194093, 1.000000000000000000, 0.8660254037844387076, 1.000000000000000000, 0.8660254037844387076, 1.000000000000000000, 0.9330127018922194093, 0.9330127018922194093 ) ) 
 REPRESENTATION_ITEM ( '' )  );
#28262=DIRECTION ( 'NONE',  ( -0.000000000000000000, 1.259100132267607459E-16, -1.000000000000000000 ) ) ;
#28264=CARTESIAN_POINT ( 'NONE',  ( -3.310556943750002645, 15.58864905735836714, -49.76827246956613493 ) ) ;
#28265=CARTESIAN_POINT ( 'NONE',  ( 1.655278471874998436, 14.63297358603754894, -111.5182724695661420 ) ) ;
#28269=CARTESIAN_POINT ( 'NONE',  ( -1.655278471875002211, 14.63297358603754006, -32.59743913623280775 ) ) ;
#28270=CARTESIAN_POINT ( 'NONE',  ( 1.655278471874998436, 14.63297358603754184, -62.51827246956613493 ) ) ;
#28271=CARTESIAN_POINT ( 'NONE',  ( 3.500000000000001332, 17.50000000000002132, -109.4609808024215027 ) ) ;
#28272=EDGE_CURVE ( 'NONE', #24209, #3824, #14080, .T. ) ;
#28274=CARTESIAN_POINT ( 'NONE',  ( -3.310556943750001313, 17.50000000000001776, -90.76410580289947916 ) ) ;
#28275=CARTESIAN_POINT ( 'NONE',  ( 1.749999999999998224, 14.46891108675448301, -97.32139747004409003 ) ) ;
#28276=CARTESIAN_POINT ( 'NONE',  ( 0.000000000000000000, 17.50000000000002487, -149.5231586289125687 ) ) ;
#28278=CARTESIAN_POINT ( 'NONE',  ( -3.500000000000001332, 17.50000000000001421, -62.96098080242150274 ) ) ;
#28279=CARTESIAN_POINT ( 'NONE',  ( 3.310556943750001313, 19.41135094264165772, -26.18077246956613990 ) ) ;
#28280=CARTESIAN_POINT ( 'NONE',  ( 3.500000000000001776, 19.52072594216370760, -53.07139747004409003 ) ) ;
#28281=CARTESIAN_POINT ( 'NONE',  ( -0.9378221735089310451, 14.00000000000001066, -45.75563900116003424 ) ) ;
#28282=CARTESIAN_POINT ( 'NONE',  ( 1.655278471874998436, 14.63297358603754716, -105.5182724695661278 ) ) ;
#28283=CARTESIAN_POINT ( 'NONE',  ( -3.310556943750002201, 15.58864905735836537, -32.76827246956613493 ) ) ;
#28286=EDGE_CURVE ( 'NONE', #20880, #3199, #21257, .T. ) ;
#28291=CARTESIAN_POINT ( 'NONE',  ( 1.655278471875001101, 20.36702641396249192, -90.09743913623280775 ) ) ;
#28292=CARTESIAN_POINT ( 'NONE',  ( -1.394453263437886604E-15, 14.00000000000000711, -25.40473080337742928 ) ) ;
#28293=VERTEX_POINT ( 'NONE', #40637 ) ;
#28298=CARTESIAN_POINT ( 'NONE',  ( -3.500000000000002220, 15.47927405783632082, -30.87764746908818481 ) ) ;
#28300=CARTESIAN_POINT ( 'NONE',  ( -3.310556943750001313, 17.50000000000001776, -96.76410580289947916 ) ) ;
#28303=DIRECTION ( 'NONE',  ( -0.000000000000000000, 1.259100132267607459E-16, -1.000000000000000000 ) ) ;
#28304=ORIENTED_EDGE ( 'NONE', *, *, #25670, .F. ) ;
#28309=ORIENTED_EDGE ( 'NONE', *, *, #22485, .F. ) ;
#28311=CARTESIAN_POINT ( 'NONE',  ( 0.000000000000000000, 21.00000000000002487, -149.5231586289125687 ) ) ;
#28312=CARTESIAN_POINT ( 'NONE',  ( 1.655278471874998436, 14.63297358603755249, -138.4307724695661364 ) ) ;
#28313=CARTESIAN_POINT ( 'NONE',  ( -3.500000000000000000, 19.52072594216371826, -132.7380641367107614 ) ) ;
#28314=ORIENTED_EDGE ( 'NONE', *, *, #35628, .T. ) ;
#28316=CARTESIAN_POINT ( 'NONE',  ( -3.310556943750002645, 15.58864905735837780, -125.7682724695661278 ) ) ;
#28317=CARTESIAN_POINT ( 'NONE',  ( 1.655278471875001101, 20.36702641396248836, -51.18493913623279923 ) ) ;
#28320=CARTESIAN_POINT ( 'NONE',  ( 1.749999999999998224, 14.46891108675448834, -137.3213974700441042 ) ) ;
#28323=CARTESIAN_POINT ( 'NONE',  ( 2.340729813953370519E-16, 21.32270188528331190, -78.10160580289945642 ) ) ;
#28324=CARTESIAN_POINT ( 'NONE',  ( -7.424026671074350129E-16, 13.45854811567264164, -128.7109808024214885 ) ) ;
#28325=CARTESIAN_POINT ( 'NONE',  ( 3.310556943750001313, 17.50000000000002132, -109.2641058028994649 ) ) ;
#28326=( BOUNDED_CURVE ( )  B_SPLINE_CURVE ( 2, ( #24538, #37718, #37504, #31121, #8360, #2404, #2188, #12176, #8781 ),
 .UNSPECIFIED., .F., .T. ) 
 B_SPLINE_CURVE_WITH_KNOTS ( ( 3, 2, 2, 2, 3 ),
 ( 0.1062499999999999972, 0.1069444444444444392, 0.1083333333333333370, 0.1097222222222222210, 0.1104166666666666630 ),
 .UNSPECIFIED. ) 
 CURVE ( )  GEOMETRIC_REPRESENTATION_ITEM ( )  RATIONAL_B_SPLINE_CURVE ( ( 0.9330127018922194093, 0.9330127018922194093, 1.000000000000000000, 0.8660254037844387076, 1.000000000000000000, 0.8660254037844387076, 1.000000000000000000, 0.9330127018922194093, 0.9330127018922194093 ) ) 
 REPRESENTATION_ITEM ( '' )  );
#28330=CARTESIAN_POINT ( 'NONE',  ( -3.500000000000001332, 17.50000000000001776, -80.96098080242150274 ) ) ;
#28331=CARTESIAN_POINT ( 'NONE',  ( 1.749999999999998224, 14.46891108675448301, -103.3213974700440900 ) ) ;
#28332=CARTESIAN_POINT ( 'NONE',  ( 3.310556943749999981, 15.58864905735836182, -40.34743913623281486 ) ) ;
#28333=CARTESIAN_POINT ( 'NONE',  ( 3.310556943750001313, 19.41135094264166838, -103.2682724695661278 ) ) ;
#28334=CARTESIAN_POINT ( 'NONE',  ( 4.648177544792955347E-16, 21.00000000000002132, -110.9047308033774186 ) ) ;
#28337=CARTESIAN_POINT ( 'NONE',  ( 1.655278471875001101, 20.36702641396249547, -125.1849391362327992 ) ) ;
#28338=CARTESIAN_POINT ( 'NONE',  ( -1.750000000000002220, 14.46891108675448834, -129.4880641367107614 ) ) ;
#28339=ADVANCED_FACE ( 'NONE', ( #41060 ), #18100, .T. ) ;
#28342=CARTESIAN_POINT ( 'NONE',  ( 1.750000000000001110, 20.53108891324555074, -50.29431413575484555 ) ) ;
#28344=CARTESIAN_POINT ( 'NONE',  ( -1.749999999999999778, 20.53108891324555074, -52.82139747004409003 ) ) ;
#28346=ORIENTED_EDGE ( 'NONE', *, *, #24315, .T. ) ;
#28347=CARTESIAN_POINT ( 'NONE',  ( -3.310556943750002201, 15.58864905735837070, -74.76827246956611361 ) ) ;
#28349=CARTESIAN_POINT ( 'NONE',  ( 3.500000000000001332, 19.52072594216370405, -40.07139747004409713 ) ) ;
#28352=CYLINDRICAL_SURFACE ( 'NONE', #2111, 3.499999999999999556 ) ;
#28354=CARTESIAN_POINT ( 'NONE',  ( 3.310556943749999981, 15.58864905735836182, -32.34743913623280775 ) ) ;
#28357=ORIENTED_EDGE ( 'NONE', *, *, #4092, .T. ) ;
#28359=CARTESIAN_POINT ( 'NONE',  ( -1.655278471875002211, 14.63297358603754184, -48.59743913623280775 ) ) ;
#28361=ORIENTED_EDGE ( 'NONE', *, *, #31046, .F. ) ;
#28364=CARTESIAN_POINT ( 'NONE',  ( -1.749999999999999778, 20.53108891324554719, -24.12764746908817415 ) ) ;
#28366=CARTESIAN_POINT ( 'NONE',  ( -1.749999999999999778, 20.53108891324555785, -104.8213974700441042 ) ) ;
#28367=CARTESIAN_POINT ( 'NONE',  ( 1.749999999999998224, 14.46891108675447413, -36.62764746908816704 ) ) ;
#28370=CARTESIAN_POINT ( 'NONE',  ( 4.648177544792955347E-16, 21.00000000000001776, -77.21098080242148853 ) ) ;
#28373=CARTESIAN_POINT ( 'NONE',  ( 1.655278471875001101, 20.36702641396248481, -24.18493913623280633 ) ) ;
#28375=CARTESIAN_POINT ( 'NONE',  ( -3.310556943750001313, 17.50000000000002132, -127.7641058028994792 ) ) ;
#28378=CARTESIAN_POINT ( 'NONE',  ( 4.648177544792955347E-16, 21.00000000000002132, -106.9047308033774328 ) ) ;
#28379=( BOUNDED_CURVE ( )  B_SPLINE_CURVE ( 2, ( #30913, #14754, #27710, #40685, #21334, #34308, #5171, #18144, #37711 ),
 .UNSPECIFIED., .F., .F. ) 
 B_SPLINE_CURVE_WITH_KNOTS ( ( 3, 2, 2, 2, 3 ),
 ( 0.8354166666666666963, 0.8361111111111111382, 0.8375000000000000222, 0.8388888888888889062, 0.8395833333333333481 ),
 .UNSPECIFIED. ) 
 CURVE ( )  GEOMETRIC_REPRESENTATION_ITEM ( )  RATIONAL_B_SPLINE_CURVE ( ( 0.9330127018922194093, 0.9330127018922194093, 1.000000000000000000, 0.8660254037844387076, 1.000000000000000000, 0.8660254037844387076, 1.000000000000000000, 0.9330127018922194093, 0.9330127018922194093 ) ) 
 REPRESENTATION_ITEM ( '' )  );
#28380=CARTESIAN_POINT ( 'NONE',  ( -3.310556943750001313, 17.50000000000002132, -117.8516058028994706 ) ) ;
#28381=CARTESIAN_POINT ( 'NONE',  ( 3.500000000000001332, 19.52072594216371826, -134.0713974700441042 ) ) ;
#28382=CARTESIAN_POINT ( 'NONE',  ( 2.474675557024783212E-16, 21.54145188432739033, -37.90473080337742573 ) ) ;
#28384=CARTESIAN_POINT ( 'NONE',  ( 2.340729813953370519E-16, 21.32270188528332255, -139.1016058028994564 ) ) ;
#28388=FACE_OUTER_BOUND ( 'NONE', #9965, .T. ) ;
#28389=CARTESIAN_POINT ( 'NONE',  ( -3.310556943750002201, 15.58864905735836714, -49.76827246956612782 ) ) ;
#28391=CARTESIAN_POINT ( 'NONE',  ( -3.500000000000002220, 15.47927405783633503, -114.5713974700440900 ) ) ;
#28392=CARTESIAN_POINT ( 'NONE',  ( 3.310556943750001313, 17.50000000000001421, -69.35160580289947063 ) ) ;
#28394=CARTESIAN_POINT ( 'NONE',  ( -1.655278471875002211, 14.63297358603754539, -72.59743913623280775 ) ) ;
#28395=AXIS2_PLACEMENT_3D ( 'NONE', #20399, #7636, #16997 ) ;
#28397=CARTESIAN_POINT ( 'NONE',  ( 1.655278471874998436, 14.63297358603754539, -93.51827246956612782 ) ) ;
#28399=CARTESIAN_POINT ( 'NONE',  ( 0.9378221735089300459, 21.00000000000001421, -67.25563900116002003 ) ) ;
#28400=CARTESIAN_POINT ( 'NONE',  ( -1.749999999999999778, 20.53108891324555785, -106.1276474690881741 ) ) ;
#28401=CARTESIAN_POINT ( 'NONE',  ( -3.500000000000002220, 15.47927405783632793, -69.87764746908817415 ) ) ;
#28402=CARTESIAN_POINT ( 'NONE',  ( 3.310556943749999981, 15.58864905735836182, -50.34743913623280775 ) ) ;
#28403=CARTESIAN_POINT ( 'NONE',  ( -1.394453263437886604E-15, 14.00000000000000711, -24.40473080337742928 ) ) ;
#28404=CARTESIAN_POINT ( 'NONE',  ( -1.655278471875002211, 14.63297358603755072, -112.5974391362328078 ) ) ;
#28406=ORIENTED_EDGE ( 'NONE', *, *, #2898, .T. ) ;
#28411=CARTESIAN_POINT ( 'NONE',  ( -3.310556943750000425, 19.41135094264166128, -65.84743913623280775 ) ) ;
#28414=VECTOR ( 'NONE', #22386, 1000.000000000000000 ) ;
#28415=DIRECTION ( 'NONE',  ( -0.000000000000000000, 1.259100132267607459E-16, -1.000000000000000000 ) ) ;
#28418=DIRECTION ( 'NONE',  ( 0.000000000000000000, 1.000000000000000000, 0.000000000000000000 ) ) ;
#28420=CARTESIAN_POINT ( 'NONE',  ( -0.9378221735089310451, 14.00000000000001599, -54.75563900116004845 ) ) ;
#28421=CARTESIAN_POINT ( 'NONE',  ( 3.310556943750001313, 19.41135094264167549, -131.1807724695661364 ) ) ;
#28422=CARTESIAN_POINT ( 'NONE',  ( -1.836030130193217234E-14, 21.00000000000002132, -128.9047308033774470 ) ) ;
#28423=CARTESIAN_POINT ( 'NONE',  ( -3.310556943750000425, 19.41135094264165772, -37.93493913623280633 ) ) ;
#28424=CARTESIAN_POINT ( 'NONE',  ( 3.310556943749999981, 15.58864905735836182, -30.43493913623279568 ) ) ;
#28425=CARTESIAN_POINT ( 'NONE',  ( -3.310556943750002645, 15.58864905735837247, -90.76827246956614204 ) ) ;
#28426=CARTESIAN_POINT ( 'NONE',  ( 1.655278471875001101, 20.36702641396249902, -143.0974391362327935 ) ) ;
#28427=ORIENTED_EDGE ( 'NONE', *, *, #5726, .F. ) ;
#28430=CARTESIAN_POINT ( 'NONE',  ( -3.310556943750000425, 19.41135094264167549, -132.9349391362327992 ) ) ;
#28432=DIRECTION ( 'NONE',  ( 0.000000000000000000, 1.000000000000000000, 0.000000000000000000 ) ) ;
#28433=CARTESIAN_POINT ( 'NONE',  ( 0.9378221735089281585, 14.00000000000001776, -87.36007260463891555 ) ) ;
#28435=CARTESIAN_POINT ( 'NONE',  ( 3.500000000000001776, 19.52072594216371115, -79.07139747004411845 ) ) ;
#28436=CARTESIAN_POINT ( 'NONE',  ( -1.655278471874999990, 20.36702641396248836, -64.01827246956614204 ) ) ;
#28438=CARTESIAN_POINT ( 'NONE',  ( -0.9378221735089335986, 21.00000000000002842, -137.1663226036829997 ) ) ;
#28439=CARTESIAN_POINT ( 'NONE',  ( 4.648177544792955347E-16, 21.00000000000001421, -58.90473080337742573 ) ) ;
#28440=CARTESIAN_POINT ( 'NONE',  ( 3.310556943750001313, 19.41135094264166483, -88.26827246956612782 ) ) ;
#28442=AXIS2_PLACEMENT_3D ( 'NONE', #17418, #30377, #14014 ) ;
#28443=CARTESIAN_POINT ( 'NONE',  ( 1.655278471874998436, 14.63297358603754894, -112.4307724695661506 ) ) ;
#28446=ORIENTED_EDGE ( 'NONE', *, *, #8430, .T. ) ;
#28447=CARTESIAN_POINT ( 'NONE',  ( -1.749999999999999778, 20.53108891324555785, -110.8213974700441042 ) ) ;
#28449=CARTESIAN_POINT ( 'NONE',  ( 4.286263797015737581E-16, 14.00000000000002487, -149.5231586289125687 ) ) ;
#28453=CARTESIAN_POINT ( 'NONE',  ( 3.310556943749999981, 15.58864905735836714, -70.34743913623280775 ) ) ;
#28454=CARTESIAN_POINT ( 'NONE',  ( 4.286263797015737581E-16, 14.00000000000002487, -149.5231586289125687 ) ) ;
#28455=ADVANCED_FACE ( 'NONE', ( #18298 ), #2348, .T. ) ;
#28459=VERTEX_POINT ( 'NONE', #31481 ) ;
#28460=CARTESIAN_POINT ( 'NONE',  ( -3.310556943750001313, 17.50000000000001066, -25.76410580289947916 ) ) ;
#28461=CARTESIAN_POINT ( 'NONE',  ( -1.749999999999999778, 20.53108891324554719, -32.12764746908818125 ) ) ;
#28462=CARTESIAN_POINT ( 'NONE',  ( -3.310556943750000425, 19.41135094264166483, -81.84743913623279354 ) ) ;
#28463=ORIENTED_EDGE ( 'NONE', *, *, #24293, .T. ) ;
#28465=CARTESIAN_POINT ( 'NONE',  ( -3.500000000000000000, 19.52072594216370760, -48.73806413671076854 ) ) ;
#28468=CARTESIAN_POINT ( 'NONE',  ( -0.9378221735089291577, 21.00000000000001776, -89.86007260463890134 ) ) ;
#28469=CARTESIAN_POINT ( 'NONE',  ( -7.022189441860112050E-16, 13.67729811471671653, -43.60160580289947063 ) ) ;
#28470=CARTESIAN_POINT ( 'NONE',  ( 1.655278471875001101, 20.36702641396249547, -110.1849391362327992 ) ) ;
#28471=VERTEX_POINT ( 'NONE', #28079 ) ;
#28472=VECTOR ( 'NONE', #16715, 1000.000000000000000 ) ;
#28473=EDGE_CURVE ( 'NONE', #13874, #37319, #35905, .T. ) ;
#28474=CARTESIAN_POINT ( 'NONE',  ( 3.310556943750001313, 17.50000000000001066, -32.26410580289947205 ) ) ;
#28475=CARTESIAN_POINT ( 'NONE',  ( -3.310556943750001313, 17.50000000000001421, -63.85160580289946353 ) ) ;
#28476=CARTESIAN_POINT ( 'NONE',  ( 1.750000000000001110, 20.53108891324555785, -105.2943141357548313 ) ) ;
#28478=CARTESIAN_POINT ( 'NONE',  ( -1.655278471875002211, 14.63297358603754716, -92.59743913623280775 ) ) ;
#28479=CARTESIAN_POINT ( 'NONE',  ( 3.500000000000001776, 19.52072594216371115, -98.07139747004409003 ) ) ;
#28480=CARTESIAN_POINT ( 'NONE',  ( 7.367361408496833051E-14, 14.00000000000001776, -108.4047308033774186 ) ) ;
#28481=CARTESIAN_POINT ( 'NONE',  ( -0.9378221735089310451, 14.00000000000001599, -56.44938900211595012 ) ) ;
#28483=CARTESIAN_POINT ( 'NONE',  ( -3.500000000000002220, 15.47927405783632437, -57.87764746908817415 ) ) ;
#28484=CARTESIAN_POINT ( 'NONE',  ( 3.310556943750001313, 19.41135094264165772, -27.18077246956613990 ) ) ;
#28485=CARTESIAN_POINT ( 'NONE',  ( -3.500000000000001332, 17.50000000000001421, -50.65473080337742573 ) ) ;
#28487=CARTESIAN_POINT ( 'NONE',  ( 3.310556943750001313, 17.50000000000002132, -107.3516058028994564 ) ) ;
#28488=CARTESIAN_POINT ( 'NONE',  ( -3.310556943750000425, 19.41135094264166128, -33.93493913623279923 ) ) ;
#28491=CARTESIAN_POINT ( 'NONE',  ( -3.500000000000002220, 15.47927405783633503, -120.8776474690881741 ) ) ;
#28494=CARTESIAN_POINT ( 'NONE',  ( -3.310556943750002201, 15.58864905735837247, -87.68077246956613635 ) ) ;
#28497=AXIS2_PLACEMENT_3D ( 'NONE', #40593, #37408, #8266 ) ;
#28499=CARTESIAN_POINT ( 'NONE',  ( -1.750000000000002220, 14.46891108675448478, -101.7943141357548456 ) ) ;
#28500=CARTESIAN_POINT ( 'NONE',  ( -3.500000000000000000, 19.52072594216370760, -65.04431413575484555 ) ) ;
#28501=( BOUNDED_CURVE ( )  B_SPLINE_CURVE ( 2, ( #24936, #14932, #31299, #34702, #34080, #18540, #4731, #41092, #40663 ),
 .UNSPECIFIED., .F., .F. ) 
 B_SPLINE_CURVE_WITH_KNOTS ( ( 3, 2, 2, 2, 3 ),
 ( 0.7395833333333333703, 0.7402777777777778123, 0.7416666666666666963, 0.7430555555555555802, 0.7437500000000000222 ),
 .UNSPECIFIED. ) 
 CURVE ( )  GEOMETRIC_REPRESENTATION_ITEM ( )  RATIONAL_B_SPLINE_CURVE ( ( 0.9330127018922194093, 0.9330127018922194093, 1.000000000000000000, 0.8660254037844387076, 1.000000000000000000, 0.8660254037844387076, 1.000000000000000000, 0.9330127018922194093, 0.9330127018922194093 ) ) 
 REPRESENTATION_ITEM ( '' )  );
#28502=ORIENTED_EDGE ( 'NONE', *, *, #23180, .T. ) ;
#28505=CARTESIAN_POINT ( 'NONE',  ( 2.340729813953370519E-16, 21.32270188528331190, -97.01410580289947916 ) ) ;
#28507=ORIENTED_EDGE ( 'NONE', *, *, #10341, .F. ) ;
#28508=DIRECTION ( 'NONE',  ( 0.000000000000000000, 1.000000000000000000, 0.000000000000000000 ) ) ;
#28510=EDGE_CURVE ( 'NONE', #2948, #3050, #40847, .T. ) ;
#28511=( BOUNDED_CURVE ( )  B_SPLINE_CURVE ( 2, ( #26416, #10247, #23659, #13862, #20459, #1110, #4071, #36183, #20034 ),
 .UNSPECIFIED., .F., .T. ) 
 B_SPLINE_CURVE_WITH_KNOTS ( ( 3, 2, 2, 2, 3 ),
 ( 0.8645833333333333703, 0.8652777777777778123, 0.8666666666666666963, 0.8680555555555555802, 0.8687500000000000222 ),
 .UNSPECIFIED. ) 
 CURVE ( )  GEOMETRIC_REPRESENTATION_ITEM ( )  RATIONAL_B_SPLINE_CURVE ( ( 0.9330127018922194093, 0.9330127018922194093, 1.000000000000000000, 0.8660254037844387076, 1.000000000000000000, 0.8660254037844387076, 1.000000000000000000, 0.9330127018922194093, 0.9330127018922194093 ) ) 
 REPRESENTATION_ITEM ( '' )  );
#28515=EDGE_CURVE ( 'NONE', #6435, #17696, #8104, .T. ) ;
#28518=ORIENTED_EDGE ( 'NONE', *, *, #36981, .T. ) ;
#28520=CARTESIAN_POINT ( 'NONE',  ( 3.500000000000000000, 15.47927405783633503, -129.5443141357548598 ) ) ;
#28521=CARTESIAN_POINT ( 'NONE',  ( -7.022189441860112050E-16, 13.67729811471672718, -135.5141058028994792 ) ) ;
#28524=EDGE_CURVE ( 'NONE', #4923, #466, #40266, .T. ) ;
#28526=CARTESIAN_POINT ( 'NONE',  ( -1.655278471874999990, 20.36702641396249547, -127.0182724695661278 ) ) ;
#28527=CARTESIAN_POINT ( 'NONE',  ( 3.310556943750001313, 19.41135094264166128, -49.26827246956613493 ) ) ;
#28528=ORIENTED_EDGE ( 'NONE', *, *, #32578, .F. ) ;
#28529=CARTESIAN_POINT ( 'NONE',  ( 1.749999999999998224, 14.46891108675448656, -133.3213974700441042 ) ) ;
#28532=CARTESIAN_POINT ( 'NONE',  ( -3.310556943750002645, 15.58864905735837070, -77.76827246956614204 ) ) ;
#28533=CARTESIAN_POINT ( 'NONE',  ( 3.500000000000000000, 15.47927405783633503, -125.5443141357548456 ) ) ;
#28534=CARTESIAN_POINT ( 'NONE',  ( 1.655278471874998436, 14.63297358603754894, -109.4307724695661506 ) ) ;
#28535=CARTESIAN_POINT ( 'NONE',  ( 1.750000000000001110, 20.53108891324555429, -80.98806413671076143 ) ) ;
#28538=CARTESIAN_POINT ( 'NONE',  ( -7.424026671074350129E-16, 13.45854811567263454, -74.71098080242151696 ) ) ;
#28539=CARTESIAN_POINT ( 'NONE',  ( -1.394453263437886604E-15, 14.00000000000001066, -51.71098080242150274 ) ) ;
#28540=CARTESIAN_POINT ( 'NONE',  ( -7.022189441860112050E-16, 13.67729811471671653, -43.51410580289947916 ) ) ;
#28541=VECTOR ( 'NONE', #8950, 1000.000000000000000 ) ;
#28542=CARTESIAN_POINT ( 'NONE',  ( 2.340729813953370519E-16, 21.32270188528331900, -102.1016058028994564 ) ) ;
#28543=CARTESIAN_POINT ( 'NONE',  ( 0.9378221735089300459, 21.00000000000001421, -73.25563900116003424 ) ) ;
#28544=CARTESIAN_POINT ( 'NONE',  ( 3.500000000000001776, 19.52072594216370760, -63.07139747004410424 ) ) ;
#28546=ORIENTED_EDGE ( 'NONE', *, *, #41073, .T. ) ;
#28547=CARTESIAN_POINT ( 'NONE',  ( -3.310556943750002201, 15.58864905735837780, -123.7682724695661136 ) ) ;
#28548=CARTESIAN_POINT ( 'NONE',  ( -3.500000000000001332, 17.50000000000001776, -91.96098080242151696 ) ) ;
#28551=CARTESIAN_POINT ( 'NONE',  ( 4.648177544792955347E-16, 21.00000000000001066, -31.90473080337742573 ) ) ;
#28555=ORIENTED_EDGE ( 'NONE', *, *, #21977, .F. ) ;
#28556=CARTESIAN_POINT ( 'NONE',  ( -1.655278471875002211, 14.63297358603754539, -75.68493913623279923 ) ) ;
#28557=CARTESIAN_POINT ( 'NONE',  ( 4.286263797015737581E-16, 14.00000000000002487, -149.5231586289125687 ) ) ;
#28562=CARTESIAN_POINT ( 'NONE',  ( -7.022189441860112050E-16, 13.67729811471671653, -33.51410580289947205 ) ) ;
#28563=CARTESIAN_POINT ( 'NONE',  ( 0.9378221735089300459, 21.00000000000002132, -106.9493890021159501 ) ) ;
#28566=ORIENTED_EDGE ( 'NONE', *, *, #39997, .T. ) ;
#28570=ORIENTED_EDGE ( 'NONE', *, *, #13910, .F. ) ;
#28579=CARTESIAN_POINT ( 'NONE',  ( -1.749999999999999778, 20.53108891324554719, -35.12764746908818125 ) ) ;
#28580=( BOUNDED_CURVE ( )  B_SPLINE_CURVE ( 2, ( #31334, #34944, #21760, #28760, #41970, #32174, #15814, #41758, #37928 ),
 .UNSPECIFIED., .F., .T. ) 
 B_SPLINE_CURVE_WITH_KNOTS ( ( 3, 2, 2, 2, 3 ),
 ( 0.3354166666666666963, 0.3361111111111111382, 0.3375000000000000222, 0.3388888888888889062, 0.3395833333333333481 ),
 .UNSPECIFIED. ) 
 CURVE ( )  GEOMETRIC_REPRESENTATION_ITEM ( )  RATIONAL_B_SPLINE_CURVE ( ( 0.9330127018922194093, 0.9330127018922220739, 1.000000000000000000, 0.8660254037844387076, 1.000000000000000000, 0.8660254037844387076, 1.000000000000000000, 0.9330127018922194093, 0.9330127018922194093 ) ) 
 REPRESENTATION_ITEM ( '' )  );
#28582=CARTESIAN_POINT ( 'NONE',  ( 1.750000000000001110, 20.53108891324555429, -96.29431413575484555 ) ) ;
#28584=CARTESIAN_POINT ( 'NONE',  ( -3.500000000000002220, 15.47927405783633503, -139.8776474690881741 ) ) ;
#28586=CARTESIAN_POINT ( 'NONE',  ( 2.340729813953370519E-16, 21.32270188528331900, -123.0141058028994792 ) ) ;
#28591=CARTESIAN_POINT ( 'NONE',  ( -3.500000000000001332, 17.50000000000001776, -98.96098080242150274 ) ) ;
#28592=CARTESIAN_POINT ( 'NONE',  ( -1.655278471874999990, 20.36702641396249547, -116.0182724695661278 ) ) ;
#28594=CARTESIAN_POINT ( 'NONE',  ( 2.474675557024783212E-16, 21.54145188432739033, -33.90473080337743284 ) ) ;
#28595=LINE ( 'NONE', #26046, #17222 ) ;
#28597=CARTESIAN_POINT ( 'NONE',  ( -7.022189441860112050E-16, 13.67729811471673074, -136.6016058028994564 ) ) ;
#28600=CARTESIAN_POINT ( 'NONE',  ( 3.310556943749999981, 15.58864905735836182, -50.43493913623279923 ) ) ;
#28603=CARTESIAN_POINT ( 'NONE',  ( -1.655278471874999990, 20.36702641396248836, -72.01827246956612782 ) ) ;
#28605=CARTESIAN_POINT ( 'NONE',  ( -3.310556943750001313, 17.50000000000001421, -72.76410580289947916 ) ) ;
#28607=VECTOR ( 'NONE', #6670, 1000.000000000000000 ) ;
#28608=CARTESIAN_POINT ( 'NONE',  ( 2.340729813953370519E-16, 21.32270188528331190, -91.10160580289947063 ) ) ;
#28610=CARTESIAN_POINT ( 'NONE',  ( 3.500000000000000000, 15.47927405783632082, -49.54431413575484555 ) ) ;
#28611=CARTESIAN_POINT ( 'NONE',  ( -3.500000000000001332, 17.50000000000002132, -105.9609808024215027 ) ) ;
#28612=CARTESIAN_POINT ( 'NONE',  ( -0.9378221735089291577, 21.00000000000001421, -70.16632260368299967 ) ) ;
#28613=CARTESIAN_POINT ( 'NONE',  ( -1.655278471875002211, 14.63297358603754184, -49.59743913623280775 ) ) ;
#28614=CARTESIAN_POINT ( 'NONE',  ( -0.9378221735089335986, 21.00000000000002842, -137.8600726046389298 ) ) ;
#28615=CARTESIAN_POINT ( 'NONE',  ( 1.655278471875001101, 20.36702641396249547, -107.0974391362328078 ) ) ;
#28617=ORIENTED_EDGE ( 'NONE', *, *, #3416, .T. ) ;
#28622=CARTESIAN_POINT ( 'NONE',  ( 1.655278471874998436, 14.63297358603754184, -62.43077246956614346 ) ) ;
#28625=CYLINDRICAL_SURFACE ( 'NONE', #13081, 3.499999999999999556 ) ;
#28630=ORIENTED_EDGE ( 'NONE', *, *, #27945, .T. ) ;
#28632=CARTESIAN_POINT ( 'NONE',  ( -7.022189441860112050E-16, 13.67729811471672896, -123.5141058028994649 ) ) ;
#28634=( BOUNDED_CURVE ( )  B_SPLINE_CURVE ( 2, ( #10419, #23396, #3398, #29972, #846, #22962, #35523, #16387, #201 ),
 .UNSPECIFIED., .F., .F. ) 
 B_SPLINE_CURVE_WITH_KNOTS ( ( 3, 2, 2, 2, 3 ),
 ( 0.7562499999999999778, 0.7569444444444444198, 0.7583333333333333037, 0.7597222222222221877, 0.7604166666666666297 ),
 .UNSPECIFIED. ) 
 CURVE ( )  GEOMETRIC_REPRESENTATION_ITEM ( )  RATIONAL_B_SPLINE_CURVE ( ( 0.9330127018922194093, 0.9330127018922194093, 1.000000000000000000, 0.8660254037844387076, 1.000000000000000000, 0.8660254037844387076, 1.000000000000000000, 0.9330127018922194093, 0.9330127018922194093 ) ) 
 REPRESENTATION_ITEM ( '' )  );
#28636=CARTESIAN_POINT ( 'NONE',  ( 2.340729813953370519E-16, 21.32270188528330479, -38.10160580289946353 ) ) ;
#28637=CARTESIAN_POINT ( 'NONE',  ( 3.310556943750001313, 17.50000000000001066, -28.35160580289947063 ) ) ;
#28638=CARTESIAN_POINT ( 'NONE',  ( -1.655278471875002211, 14.63297358603754716, -86.68493913623278502 ) ) ;
#28639=CARTESIAN_POINT ( 'NONE',  ( 3.310556943749999981, 15.58864905735837780, -138.3474391362328220 ) ) ;
#28642=CARTESIAN_POINT ( 'NONE',  ( 2.340729813953370519E-16, 21.32270188528332255, -132.1016058028994564 ) ) ;
#28645=CARTESIAN_POINT ( 'NONE',  ( 4.648177544792955347E-16, 21.00000000000002487, -135.9047308033774186 ) ) ;
#28646=CARTESIAN_POINT ( 'NONE',  ( -3.500000000000002220, 15.47927405783633503, -122.5713974700441184 ) ) ;
#28647=CARTESIAN_POINT ( 'NONE',  ( -3.500000000000002220, 15.47927405783632615, -78.57139747004410424 ) ) ;
#28648=CARTESIAN_POINT ( 'NONE',  ( -1.655278471874999990, 20.36702641396248836, -63.01827246956613493 ) ) ;
#28650=CARTESIAN_POINT ( 'NONE',  ( -3.310556943750000425, 19.41135094264166483, -82.93493913623278502 ) ) ;
#28651=CARTESIAN_POINT ( 'NONE',  ( 4.286263797015737581E-16, 14.00000000000002487, -149.5231586289125687 ) ) ;
#28652=CARTESIAN_POINT ( 'NONE',  ( 3.310556943749999981, 15.58864905735837247, -113.3474391362328220 ) ) ;
#28655=VERTEX_POINT ( 'NONE', #32898 ) ;
#28656=CARTESIAN_POINT ( 'NONE',  ( -3.500000000000001332, 17.50000000000002132, -105.6547308033774186 ) ) ;
#28661=CARTESIAN_POINT ( 'NONE',  ( -3.310556943750001313, 17.50000000000001421, -63.76410580289947205 ) ) ;
#28662=DIRECTION ( 'NONE',  ( -0.000000000000000000, 1.259100132267607459E-16, -1.000000000000000000 ) ) ;
#28663=CARTESIAN_POINT ( 'NONE',  ( 0.9378221735089281585, 14.00000000000001599, -71.36007260463891555 ) ) ;
#28665=CARTESIAN_POINT ( 'NONE',  ( -0.9378221735089291577, 21.00000000000002132, -125.8600726046389155 ) ) ;
#28666=EDGE_LOOP ( 'NONE', ( #10057, #22778, #19575, #320 ) ) ;
#28669=CARTESIAN_POINT ( 'NONE',  ( -1.655278471874999990, 20.36702641396249192, -76.93077246956615056 ) ) ;
#28671=ORIENTED_EDGE ( 'NONE', *, *, #31035, .T. ) ;
#28672=CYLINDRICAL_SURFACE ( 'NONE', #31000, 3.499999999999999556 ) ;
#28675=CARTESIAN_POINT ( 'NONE',  ( -3.310556943750000425, 19.41135094264167549, -138.8474391362327935 ) ) ;
#28677=LINE ( 'NONE', #12737, #18004 ) ;
#28678=CARTESIAN_POINT ( 'NONE',  ( 1.655278471874998436, 14.63297358603754006, -43.51827246956613493 ) ) ;
#28679=CARTESIAN_POINT ( 'NONE',  ( 2.340729813953370519E-16, 21.32270188528331900, -109.1016058028994564 ) ) ;
#28681=EDGE_CURVE ( 'NONE', #21198, #15133, #18268, .T. ) ;
#28682=ADVANCED_FACE ( 'NONE', ( #13343 ), #7378, .T. ) ;
#28683=CARTESIAN_POINT ( 'NONE',  ( 3.310556943749999981, 15.58864905735836182, -30.34743913623280775 ) ) ;
#28684=CARTESIAN_POINT ( 'NONE',  ( 1.655278471874998436, 14.63297358603754184, -59.51827246956613493 ) ) ;
#28685=CARTESIAN_POINT ( 'NONE',  ( 1.750000000000001110, 20.53108891324555785, -106.2943141357548456 ) ) ;
#28687=CARTESIAN_POINT ( 'NONE',  ( 3.500000000000000000, 15.47927405783632793, -99.23806413671076143 ) ) ;
#28688=CARTESIAN_POINT ( 'NONE',  ( 0.000000000000000000, 17.50000000000002487, -149.5231586289125687 ) ) ;
#28691=CARTESIAN_POINT ( 'NONE',  ( 3.500000000000001332, 17.50000000000001421, -60.46098080242151696 ) ) ;
#28693=CARTESIAN_POINT ( 'NONE',  ( -7.022189441860112050E-16, 13.67729811471671297, -25.51410580289947916 ) ) ;
#28694=CARTESIAN_POINT ( 'NONE',  ( 1.749999999999998224, 14.46891108675447590, -46.32139747004410424 ) ) ;
#28696=CARTESIAN_POINT ( 'NONE',  ( 2.340729813953370519E-16, 21.32270188528330834, -31.10160580289945997 ) ) ;
#28703=CARTESIAN_POINT ( 'NONE',  ( 3.310556943750001313, 17.50000000000001776, -82.26410580289947916 ) ) ;
#28704=AXIS2_PLACEMENT_3D ( 'NONE', #9707, #26076, #39033 ) ;
#28705=DIRECTION ( 'NONE',  ( 0.000000000000000000, 1.000000000000000000, 0.000000000000000000 ) ) ;
#28708=VERTEX_POINT ( 'NONE', #42072 ) ;
#28711=CARTESIAN_POINT ( 'NONE',  ( 1.655278471875001101, 20.36702641396249192, -94.09743913623280775 ) ) ;
#28714=ORIENTED_EDGE ( 'NONE', *, *, #30771, .T. ) ;
#28716=VERTEX_POINT ( 'NONE', #3349 ) ;
#28719=DIRECTION ( 'NONE',  ( 0.000000000000000000, 1.000000000000000000, 0.000000000000000000 ) ) ;
#28723=CARTESIAN_POINT ( 'NONE',  ( -0.9378221735089291577, 21.00000000000002132, -127.8600726046389155 ) ) ;
#28724=FACE_OUTER_BOUND ( 'NONE', #10008, .T. ) ;
#28725=CARTESIAN_POINT ( 'NONE',  ( 3.310556943749999981, 15.58864905735837425, -133.3474391362328220 ) ) ;
#28726=CARTESIAN_POINT ( 'NONE',  ( 1.749999999999998224, 14.46891108675448834, -141.6276474690881741 ) ) ;
#28728=CARTESIAN_POINT ( 'NONE',  ( -1.655278471874999990, 20.36702641396249547, -125.0182724695661278 ) ) ;
#28729=CARTESIAN_POINT ( 'NONE',  ( 1.655278471874998436, 14.63297358603754006, -48.51827246956613493 ) ) ;
#28730=ORIENTED_EDGE ( 'NONE', *, *, #21469, .F. ) ;
#28731=CARTESIAN_POINT ( 'NONE',  ( 3.500000000000001332, 17.50000000000002132, -128.1547308033774186 ) ) ;
#28734=CARTESIAN_POINT ( 'NONE',  ( -3.310556943750000425, 19.41135094264166483, -75.93493913623279923 ) ) ;
#28735=CARTESIAN_POINT ( 'NONE',  ( -7.424026671074350129E-16, 13.45854811567264164, -124.7109808024215027 ) ) ;
#28736=CARTESIAN_POINT ( 'NONE',  ( -7.022189441860112050E-16, 13.67729811471672541, -105.5141058028994649 ) ) ;
#28737=CARTESIAN_POINT ( 'NONE',  ( 4.286263797015737581E-16, 14.00000000000002487, -149.5231586289125687 ) ) ;
#28740=CARTESIAN_POINT ( 'NONE',  ( -1.750000000000002220, 14.46891108675448123, -75.79431413575484555 ) ) ;
#28741=CARTESIAN_POINT ( 'NONE',  ( -1.394453263437886604E-15, 14.00000000000002132, -133.7109808024214885 ) ) ;
#28742=CARTESIAN_POINT ( 'NONE',  ( -1.655278471874999990, 20.36702641396248481, -40.93077246956614346 ) ) ;
#28743=CARTESIAN_POINT ( 'NONE',  ( 2.340729813953370519E-16, 21.32270188528331190, -101.1016058028994706 ) ) ;
#28744=( BOUNDED_CURVE ( )  B_SPLINE_CURVE ( 2, ( #7592, #5018, #8416, #26956, #17588, #30343, #33756, #17792, #11604 ),
 .UNSPECIFIED., .F., .F. ) 
 B_SPLINE_CURVE_WITH_KNOTS ( ( 3, 2, 2, 2, 3 ),
 ( 0.7645833333333332815, 0.7652777777777777235, 0.7666666666666667185, 0.7680555555555556024, 0.7687500000000000444 ),
 .UNSPECIFIED. ) 
 CURVE ( )  GEOMETRIC_REPRESENTATION_ITEM ( )  RATIONAL_B_SPLINE_CURVE ( ( 0.9330127018922194093, 0.9330127018922194093, 1.000000000000000000, 0.8660254037844387076, 1.000000000000000000, 0.8660254037844387076, 1.000000000000000000, 0.9330127018922194093, 0.9330127018922194093 ) ) 
 REPRESENTATION_ITEM ( '' )  );
#28746=CARTESIAN_POINT ( 'NONE',  ( 2.474675557024783212E-16, 21.54145188432739388, -62.90473080337743284 ) ) ;
#28749=CARTESIAN_POINT ( 'NONE',  ( 1.655278471874998436, 14.63297358603754894, -115.5182724695661278 ) ) ;
#28750=CARTESIAN_POINT ( 'NONE',  ( -1.750000000000002220, 14.46891108675448301, -91.79431413575484555 ) ) ;
#28753=FACE_OUTER_BOUND ( 'NONE', #36425, .T. ) ;
#28758=CARTESIAN_POINT ( 'NONE',  ( -1.655278471874999990, 20.36702641396249192, -77.01827246956612782 ) ) ;
#28759=FACE_OUTER_BOUND ( 'NONE', #34581, .T. ) ;
#28760=CARTESIAN_POINT ( 'NONE',  ( -3.500000000000000000, 19.52072594216371826, -102.7380641367107756 ) ) ;
#28764=CARTESIAN_POINT ( 'NONE',  ( -3.310556943750000425, 19.41135094264166128, -31.84743913623280775 ) ) ;
#28767=EDGE_CURVE ( 'NONE', #5882, #32026, #10364, .T. ) ;
#28772=CARTESIAN_POINT ( 'NONE',  ( -3.500000000000002220, 15.47927405783633503, -138.5713974700441042 ) ) ;
#28778=CARTESIAN_POINT ( 'NONE',  ( 3.500000000000000000, 15.47927405783632970, -120.2380641367107614 ) ) ;
#28779=DIRECTION ( 'NONE',  ( -0.000000000000000000, 1.259100132267607459E-16, -1.000000000000000000 ) ) ;
#28780=CARTESIAN_POINT ( 'NONE',  ( -1.750000000000002220, 14.46891108675447590, -35.79431413575484555 ) ) ;
#28784=CARTESIAN_POINT ( 'NONE',  ( -0.9378221735089310451, 14.00000000000001599, -65.44938900211593591 ) ) ;
#28786=CARTESIAN_POINT ( 'NONE',  ( 1.749999999999998224, 14.46891108675448834, -136.6276474690881741 ) ) ;
#28787=CARTESIAN_POINT ( 'NONE',  ( 1.750000000000001110, 20.53108891324555785, -120.2943141357548313 ) ) ;
#28788=CARTESIAN_POINT ( 'NONE',  ( 3.310556943750001313, 17.50000000000002132, -122.2641058028994792 ) ) ;
#28792=CARTESIAN_POINT ( 'NONE',  ( -3.500000000000002220, 15.47927405783632793, -88.87764746908818836 ) ) ;
#28793=EDGE_CURVE ( 'NONE', #22806, #29352, #35671, .T. ) ;
#28795=CARTESIAN_POINT ( 'NONE',  ( -3.310556943750001313, 17.50000000000001421, -59.76410580289947916 ) ) ;
#28796=CARTESIAN_POINT ( 'NONE',  ( -3.310556943750000425, 19.41135094264166838, -118.9349391362327992 ) ) ;
#28797=CARTESIAN_POINT ( 'NONE',  ( -0.9378221735089291577, 21.00000000000002132, -122.1663226036829997 ) ) ;
#28798=CARTESIAN_POINT ( 'NONE',  ( 1.749999999999998224, 14.46891108675447413, -34.32139747004410424 ) ) ;
#28799=CARTESIAN_POINT ( 'NONE',  ( -3.500000000000001332, 17.50000000000002132, -108.9609808024215027 ) ) ;
#28803=CARTESIAN_POINT ( 'NONE',  ( 1.655278471874998436, 14.63297358603755249, -138.5182724695661420 ) ) ;
#28805=CARTESIAN_POINT ( 'NONE',  ( 3.310556943750001313, 17.50000000000002487, -143.3516058028994564 ) ) ;
#28806=CARTESIAN_POINT ( 'NONE',  ( -3.310556943750001313, 17.50000000000001421, -49.85160580289946353 ) ) ;
#28809=CARTESIAN_POINT ( 'NONE',  ( -3.310556943750000425, 19.41135094264166128, -67.93493913623281344 ) ) ;
#28811=CARTESIAN_POINT ( 'NONE',  ( 2.340729813953370519E-16, 21.32270188528330834, -64.01410580289947916 ) ) ;
#28812=ORIENTED_EDGE ( 'NONE', *, *, #32265, .F. ) ;
#28813=CARTESIAN_POINT ( 'NONE',  ( 1.655278471875001101, 20.36702641396249192, -89.18493913623279923 ) ) ;
#28815=CARTESIAN_POINT ( 'NONE',  ( 4.648177544792955347E-16, 21.00000000000001776, -85.21098080242151696 ) ) ;
#28817=CARTESIAN_POINT ( 'NONE',  ( -3.500000000000001332, 17.50000000000001066, -41.96098080242150985 ) ) ;
#28818=CARTESIAN_POINT ( 'NONE',  ( -3.310556943750000425, 19.41135094264166483, -48.84743913623280775 ) ) ;
#28820=CARTESIAN_POINT ( 'NONE',  ( 2.340729813953370519E-16, 21.32270188528331900, -106.0141058028994792 ) ) ;
#28823=ORIENTED_EDGE ( 'NONE', *, *, #22560, .F. ) ;
#28825=VERTEX_POINT ( 'NONE', #4404 ) ;
#28827=CARTESIAN_POINT ( 'NONE',  ( 3.310556943750001313, 19.41135094264166128, -57.18077246956614346 ) ) ;
#28828=( BOUNDED_CURVE ( )  B_SPLINE_CURVE ( 2, ( #16376, #29318, #26157, #20400, #32941, #6998, #6582, #33364, #42110 ),
 .UNSPECIFIED., .F., .F. ) 
 B_SPLINE_CURVE_WITH_KNOTS ( ( 3, 2, 2, 2, 3 ),
 ( 0.9854166666666667185, 0.9861111111111111605, 0.9875000000000000444, 0.9888888888888889284, 0.9895833333333333703 ),
 .UNSPECIFIED. ) 
 CURVE ( )  GEOMETRIC_REPRESENTATION_ITEM ( )  RATIONAL_B_SPLINE_CURVE ( ( 0.9330127018922194093, 0.9330127018922194093, 1.000000000000000000, 0.8660254037844387076, 1.000000000000000000, 0.8660254037844387076, 1.000000000000000000, 0.9330127018922194093, 0.9330127018922194093 ) ) 
 REPRESENTATION_ITEM ( '' )  );
#28834=AXIS2_PLACEMENT_3D ( 'NONE', #485, #40041, #1338 ) ;
#28837=CARTESIAN_POINT ( 'NONE',  ( 3.310556943750001313, 17.50000000000002132, -125.2641058028994792 ) ) ;
#28840=CARTESIAN_POINT ( 'NONE',  ( 1.655278471875001101, 20.36702641396248481, -34.18493913623279923 ) ) ;
#28841=EDGE_CURVE ( 'NONE', #31096, #21455, #15305, .T. ) ;
#28842=CARTESIAN_POINT ( 'NONE',  ( 2.340729813953370519E-16, 21.32270188528330479, -30.10160580289947418 ) ) ;
#28843=CARTESIAN_POINT ( 'NONE',  ( 3.310556943750001313, 17.50000000000001776, -88.35160580289947063 ) ) ;
#28844=CARTESIAN_POINT ( 'NONE',  ( 3.310556943750001313, 19.41135094264167549, -138.1807724695661648 ) ) ;
#28848=CARTESIAN_POINT ( 'NONE',  ( 3.310556943750001313, 19.41135094264167549, -132.2682724695661420 ) ) ;
#28849=AXIS2_PLACEMENT_3D ( 'NONE', #28949, #41313, #12793 ) ;
#28850=CARTESIAN_POINT ( 'NONE',  ( 1.749999999999998224, 14.46891108675447768, -56.62764746908817415 ) ) ;
#28852=CARTESIAN_POINT ( 'NONE',  ( -1.394453263437886604E-15, 14.00000000000001776, -92.71098080242150274 ) ) ;
#28854=CARTESIAN_POINT ( 'NONE',  ( 1.749999999999998224, 14.46891108675447946, -80.32139747004410424 ) ) ;
#28855=CARTESIAN_POINT ( 'NONE',  ( -1.655278471874999990, 20.36702641396248836, -62.01827246956613493 ) ) ;
#28858=CARTESIAN_POINT ( 'NONE',  ( 0.9378221735089281585, 14.00000000000001066, -47.66632260368298546 ) ) ;
#28859=CARTESIAN_POINT ( 'NONE',  ( 1.655278471875001101, 20.36702641396249192, -85.18493913623278502 ) ) ;
#28860=CARTESIAN_POINT ( 'NONE',  ( -0.9378221735089291577, 21.00000000000001776, -77.86007260463890134 ) ) ;
#28861=CARTESIAN_POINT ( 'NONE',  ( -7.022189441860112050E-16, 13.67729811471672896, -115.5141058028994934 ) ) ;
#28862=CARTESIAN_POINT ( 'NONE',  ( 4.648177544792955347E-16, 21.00000000000001066, -34.21098080242150985 ) ) ;
#28866=CARTESIAN_POINT ( 'NONE',  ( 2.474675557024783212E-16, 21.54145188432740099, -105.9047308033774186 ) ) ;
#28867=CARTESIAN_POINT ( 'NONE',  ( -0.9378221735089313782, 21.00000000000002132, -140.1663226036829997 ) ) ;
#28868=AXIS2_PLACEMENT_3D ( 'NONE', #25000, #5213, #2017 ) ;
#28872=EDGE_CURVE ( 'NONE', #37668, #34171, #7972, .T. ) ;
#28875=CARTESIAN_POINT ( 'NONE',  ( -1.655278471874999990, 20.36702641396248836, -68.93077246956613635 ) ) ;
#28877=CARTESIAN_POINT ( 'NONE',  ( 3.310556943749999981, 15.58864905735837247, -119.3474391362327935 ) ) ;
#28883=CARTESIAN_POINT ( 'NONE',  ( -1.655278471874999990, 20.36702641396249192, -74.93077246956613635 ) ) ;
#28886=( BOUNDED_CURVE ( )  B_SPLINE_CURVE ( 2, ( #1097, #13630, #14068, #3851, #30642, #27041, #40004, #10872, #36823 ),
 .UNSPECIFIED., .F., .T. ) 
 B_SPLINE_CURVE_WITH_KNOTS ( ( 3, 2, 2, 2, 3 ),
 ( 0.3562500000000000111, 0.3569444444444444531, 0.3583333333333333370, 0.3597222222222222210, 0.3604166666666666630 ),
 .UNSPECIFIED. ) 
 CURVE ( )  GEOMETRIC_REPRESENTATION_ITEM ( )  RATIONAL_B_SPLINE_CURVE ( ( 0.9330127018922194093, 0.9330127018922194093, 1.000000000000000000, 0.8660254037844387076, 1.000000000000000000, 0.8660254037844387076, 1.000000000000000000, 0.9330127018922194093, 0.9330127018922194093 ) ) 
 REPRESENTATION_ITEM ( '' )  );
#28888=AXIS2_PLACEMENT_3D ( 'NONE', #24567, #17763, #1803 ) ;
#28889=CARTESIAN_POINT ( 'NONE',  ( 1.655278471875001101, 20.36702641396249902, -143.0974391362327935 ) ) ;
#28894=CARTESIAN_POINT ( 'NONE',  ( 3.310556943749999981, 15.58864905735836182, -43.43493913623279212 ) ) ;
#28895=CARTESIAN_POINT ( 'NONE',  ( 3.310556943750001313, 17.50000000000002132, -102.3516058028994564 ) ) ;
#28896=ORIENTED_EDGE ( 'NONE', *, *, #17312, .F. ) ;
#28897=CARTESIAN_POINT ( 'NONE',  ( -3.310556943750002645, 15.58864905735836537, -28.68077246956614346 ) ) ;
#28898=CARTESIAN_POINT ( 'NONE',  ( 1.749999999999998224, 14.46891108675447946, -69.32139747004409003 ) ) ;
#28899=CARTESIAN_POINT ( 'NONE',  ( 3.500000000000001776, 19.52072594216371826, -107.3776474690881741 ) ) ;
#28902=CARTESIAN_POINT ( 'NONE',  ( 3.500000000000001776, 19.52072594216371115, -99.07139747004409003 ) ) ;
#28906=CARTESIAN_POINT ( 'NONE',  ( 1.749999999999998224, 14.46891108675447768, -57.62764746908817415 ) ) ;
#28908=CARTESIAN_POINT ( 'NONE',  ( -1.655278471874999990, 20.36702641396248481, -24.93077246956613990 ) ) ;
#28909=CARTESIAN_POINT ( 'NONE',  ( 3.500000000000001332, 17.50000000000001421, -50.15473080337742573 ) ) ;
#28910=CARTESIAN_POINT ( 'NONE',  ( -1.749999999999999778, 20.53108891324554719, -46.12764746908818125 ) ) ;
#28911=CARTESIAN_POINT ( 'NONE',  ( -7.022189441860112050E-16, 13.67729811471671653, -33.60160580289946353 ) ) ;
#28914=DIRECTION ( 'NONE',  ( 0.000000000000000000, 1.000000000000000000, 0.000000000000000000 ) ) ;
#28918=CARTESIAN_POINT ( 'NONE',  ( -7.022189441860112050E-16, 13.67729811471672363, -81.51410580289946495 ) ) ;
#28920=ORIENTED_EDGE ( 'NONE', *, *, #18158, .T. ) ;
#28922=CARTESIAN_POINT ( 'NONE',  ( -1.394453263437886604E-15, 14.00000000000001776, -87.71098080242151696 ) ) ;
#28923=ORIENTED_EDGE ( 'NONE', *, *, #21041, .F. ) ;
#28926=CARTESIAN_POINT ( 'NONE',  ( 3.310556943750001313, 19.41135094264166483, -94.18077246956613635 ) ) ;
#28927=ORIENTED_EDGE ( 'NONE', *, *, #8171, .F. ) ;
#28929=ORIENTED_EDGE ( 'NONE', *, *, #24525, .F. ) ;
#28934=DIRECTION ( 'NONE',  ( 0.000000000000000000, 1.000000000000000000, 0.000000000000000000 ) ) ;
#28936=CARTESIAN_POINT ( 'NONE',  ( -7.022189441860112050E-16, 13.67729811471672718, -131.5141058028994507 ) ) ;
#28938=CARTESIAN_POINT ( 'NONE',  ( 4.648177544792955347E-16, 21.00000000000002487, -141.2109808024214601 ) ) ;
#28939=CARTESIAN_POINT ( 'NONE',  ( 3.310556943750001313, 19.41135094264166838, -119.2682724695661278 ) ) ;
#28940=CARTESIAN_POINT ( 'NONE',  ( -1.655278471874999990, 20.36702641396248836, -49.01827246956613493 ) ) ;
#28942=CARTESIAN_POINT ( 'NONE',  ( 1.749999999999998224, 14.46891108675448656, -132.3213974700441042 ) ) ;
#28945=CARTESIAN_POINT ( 'NONE',  ( 3.310556943750001313, 17.50000000000001776, -75.35160580289947063 ) ) ;
#28946=CARTESIAN_POINT ( 'NONE',  ( -7.424026671074350129E-16, 13.45854811567263987, -121.7109808024215312 ) ) ;
#28947=CARTESIAN_POINT ( 'NONE',  ( -3.310556943750002645, 15.58864905735837425, -108.6807724695661364 ) ) ;
#28949=CARTESIAN_POINT ( 'NONE',  ( 0.000000000000000000, 17.50000000000002487, -149.5231586289125687 ) ) ;
#28952=CARTESIAN_POINT ( 'NONE',  ( -7.424026671074350129E-16, 13.45854811567263454, -76.71098080242148853 ) ) ;
#28954=CARTESIAN_POINT ( 'NONE',  ( 3.310556943750001313, 19.41135094264165772, -43.18077246956614346 ) ) ;
#28955=CARTESIAN_POINT ( 'NONE',  ( 3.310556943750001313, 19.41135094264166838, -102.2682724695661278 ) ) ;
#28957=CARTESIAN_POINT ( 'NONE',  ( 1.749999999999998224, 14.46891108675447768, -66.32139747004409003 ) ) ;
#28958=DIRECTION ( 'NONE',  ( -0.000000000000000000, 1.259100132267607459E-16, -1.000000000000000000 ) ) ;
#28960=CARTESIAN_POINT ( 'NONE',  ( -1.655278471875002211, 14.63297358603755072, -118.6849391362327992 ) ) ;
#28964=CARTESIAN_POINT ( 'NONE',  ( 1.749999999999998224, 14.46891108675447413, -32.32139747004410424 ) ) ;
#28966=CARTESIAN_POINT ( 'NONE',  ( -3.310556943750001313, 17.50000000000001776, -97.76410580289947916 ) ) ;
#28967=CARTESIAN_POINT ( 'NONE',  ( 0.000000000000000000, 21.00000000000002487, -149.5231586289125687 ) ) ;
#28970=CARTESIAN_POINT ( 'NONE',  ( -1.394453263437886604E-15, 14.00000000000001776, -87.40473080337743284 ) ) ;
#28975=CARTESIAN_POINT ( 'NONE',  ( -3.310556943750002201, 15.58864905735836537, -33.68077246956615056 ) ) ;
#28976=ADVANCED_FACE ( 'NONE', ( #30552 ), #40126, .T. ) ;
#28978=EDGE_CURVE ( 'NONE', #30090, #37215, #31313, .T. ) ;
#28980=EDGE_LOOP ( 'NONE', ( #18115, #30934, #17398, #15884 ) ) ;
#28982=CYLINDRICAL_SURFACE ( 'NONE', #20423, 3.499999999999999556 ) ;
#28983=EDGE_LOOP ( 'NONE', ( #38719, #9805, #19729, #19148 ) ) ;
#28984=CARTESIAN_POINT ( 'NONE',  ( -0.9378221735089291577, 21.00000000000001066, -37.86007260463890134 ) ) ;
#28985=CYLINDRICAL_SURFACE ( 'NONE', #41177, 3.499999999999999556 ) ;
#28988=CARTESIAN_POINT ( 'NONE',  ( -1.750000000000002220, 14.46891108675448656, -121.4880641367107614 ) ) ;
#28990=CARTESIAN_POINT ( 'NONE',  ( 1.655278471874998436, 14.63297358603755072, -134.5182724695661420 ) ) ;
#28991=CARTESIAN_POINT ( 'NONE',  ( -3.500000000000001332, 17.50000000000001066, -30.96098080242150274 ) ) ;
#28993=( BOUNDED_CURVE ( )  B_SPLINE_CURVE ( 2, ( #30639, #39795, #33408, #1298, #33834, #40212, #27455, #17256, #24067 ),
 .UNSPECIFIED., .F., .T. ) 
 B_SPLINE_CURVE_WITH_KNOTS ( ( 3, 2, 2, 2, 3 ),
 ( 0.6020833333333333037, 0.6027777777777777457, 0.6041666666666666297, 0.6055555555555555136, 0.6062499999999999556 ),
 .UNSPECIFIED. ) 
 CURVE ( )  GEOMETRIC_REPRESENTATION_ITEM ( )  RATIONAL_B_SPLINE_CURVE ( ( 0.9330127018922194093, 0.9330127018922194093, 1.000000000000000000, 0.8660254037844387076, 1.000000000000000000, 0.8660254037844387076, 1.000000000000000000, 0.9330127018922194093, 0.9330127018922194093 ) ) 
 REPRESENTATION_ITEM ( '' )  );
#28995=CARTESIAN_POINT ( 'NONE',  ( 0.9378221735089281585, 14.00000000000002132, -118.6663226036829855 ) ) ;
#28997=CARTESIAN_POINT ( 'NONE',  ( -3.500000000000000888, 19.52072594216372181, -139.0443141357548313 ) ) ;
#28998=CARTESIAN_POINT ( 'NONE',  ( -1.394453263437886604E-15, 14.00000000000001776, -83.40473080337743284 ) ) ;
#28999=CARTESIAN_POINT ( 'NONE',  ( -7.022189441860112050E-16, 13.67729811471672718, -124.5141058028994649 ) ) ;
#29002=EDGE_CURVE ( 'NONE', #23990, #13827, #22361, .T. ) ;
#29005=CARTESIAN_POINT ( 'NONE',  ( 3.500000000000000000, 15.47927405783632615, -93.54431413575484555 ) ) ;
#29006=CARTESIAN_POINT ( 'NONE',  ( 3.500000000000000000, 15.47927405783632082, -33.23806413671076854 ) ) ;
#29007=CARTESIAN_POINT ( 'NONE',  ( 3.310556943749999981, 15.58864905735836537, -57.34743913623279354 ) ) ;
#29008=EDGE_CURVE ( 'NONE', #3989, #38542, #892, .T. ) ;
#29009=CARTESIAN_POINT ( 'NONE',  ( 3.310556943750001313, 19.41135094264166838, -116.2682724695661420 ) ) ;
#29010=CARTESIAN_POINT ( 'NONE',  ( 3.500000000000001776, 19.52072594216370405, -33.07139747004410424 ) ) ;
#29011=CARTESIAN_POINT ( 'NONE',  ( 4.648177544792955347E-16, 21.00000000000001066, -30.90473080337742928 ) ) ;
#29013=CARTESIAN_POINT ( 'NONE',  ( -3.310556943750002201, 15.58864905735837780, -131.7682724695661136 ) ) ;
#29015=CARTESIAN_POINT ( 'NONE',  ( -3.500000000000001332, 17.50000000000001421, -66.65473080337743284 ) ) ;
#29016=CARTESIAN_POINT ( 'NONE',  ( -3.310556943750000425, 19.41135094264166128, -40.93493913623278502 ) ) ;
#29018=CARTESIAN_POINT ( 'NONE',  ( 3.310556943750001313, 19.41135094264166128, -67.26827246956612782 ) ) ;
#29020=CARTESIAN_POINT ( 'NONE',  ( -7.022189441860112050E-16, 13.67729811471672186, -67.51410580289946495 ) ) ;
#29021=ORIENTED_EDGE ( 'NONE', *, *, #12405, .T. ) ;
#29022=EDGE_LOOP ( 'NONE', ( #5350, #14872, #3458, #6687 ) ) ;
#29023=CARTESIAN_POINT ( 'NONE',  ( -7.022189441860112050E-16, 13.67729811471672363, -86.60160580289947063 ) ) ;
#29025=FACE_OUTER_BOUND ( 'NONE', #3418, .T. ) ;
#29026=CARTESIAN_POINT ( 'NONE',  ( -3.500000000000001332, 17.50000000000001066, -39.96098080242150985 ) ) ;
#29028=CARTESIAN_POINT ( 'NONE',  ( -3.310556943750001313, 17.50000000000001421, -52.76410580289947205 ) ) ;
#29030=CARTESIAN_POINT ( 'NONE',  ( -1.655278471874999990, 20.36702641396249547, -104.9307724695661364 ) ) ;
#29031=ORIENTED_EDGE ( 'NONE', *, *, #14974, .T. ) ;
#29036=CARTESIAN_POINT ( 'NONE',  ( -1.655278471874999990, 20.36702641396248836, -58.93077246956614346 ) ) ;
#29038=VERTEX_POINT ( 'NONE', #9263 ) ;
#29040=EDGE_CURVE ( 'NONE', #466, #18214, #8214, .T. ) ;
#29043=CYLINDRICAL_SURFACE ( 'NONE', #34679, 3.499999999999999556 ) ;
#29046=CARTESIAN_POINT ( 'NONE',  ( -0.9378221735089310451, 14.00000000000001066, -38.75563900116003424 ) ) ;
#29047=CARTESIAN_POINT ( 'NONE',  ( -3.310556943750002201, 15.58864905735837780, -127.6807724695661364 ) ) ;
#29048=DIRECTION ( 'NONE',  ( -0.000000000000000000, 1.259100132267607459E-16, -1.000000000000000000 ) ) ;
#29050=CARTESIAN_POINT ( 'NONE',  ( 2.340729813953370519E-16, 21.32270188528330479, -36.10160580289946353 ) ) ;
#29051=CARTESIAN_POINT ( 'NONE',  ( 1.655278471875001101, 20.36702641396248481, -30.18493913623279568 ) ) ;
#29053=CARTESIAN_POINT ( 'NONE',  ( -1.655278471875002211, 14.63297358603754716, -89.68493913623279923 ) ) ;
#29054=CARTESIAN_POINT ( 'NONE',  ( -1.655278471874999990, 20.36702641396249902, -139.9307724695661364 ) ) ;
#29058=CARTESIAN_POINT ( 'NONE',  ( 2.340729813953370519E-16, 21.32270188528332255, -135.1016058028994564 ) ) ;
#29059=CARTESIAN_POINT ( 'NONE',  ( 0.9378221735089300459, 21.00000000000001421, -69.94938900211596433 ) ) ;
#29061=CARTESIAN_POINT ( 'NONE',  ( 0.000000000000000000, 17.50000000000002487, -149.5231586289125687 ) ) ;
#29063=CARTESIAN_POINT ( 'NONE',  ( 3.500000000000000000, 15.47927405783632437, -78.23806413671076143 ) ) ;
#29064=CARTESIAN_POINT ( 'NONE',  ( -3.310556943750000425, 19.41135094264166483, -56.93493913623279212 ) ) ;
#29067=CARTESIAN_POINT ( 'NONE',  ( -3.500000000000001332, 17.50000000000002487, -129.6547308033774186 ) ) ;
#29068=CARTESIAN_POINT ( 'NONE',  ( 3.310556943750001313, 19.41135094264166483, -84.26827246956612782 ) ) ;
#29069=CARTESIAN_POINT ( 'NONE',  ( 3.310556943750001313, 17.50000000000002487, -143.3516058028994564 ) ) ;
#29070=CARTESIAN_POINT ( 'NONE',  ( -3.310556943750001313, 17.50000000000002132, -114.7641058028994792 ) ) ;
#29071=CARTESIAN_POINT ( 'NONE',  ( -1.655278471874999990, 20.36702641396249192, -82.93077246956615056 ) ) ;
#29074=CARTESIAN_POINT ( 'NONE',  ( 3.500000000000000000, 15.47927405783632793, -107.2380641367107614 ) ) ;
#29076=DIRECTION ( 'NONE',  ( 0.000000000000000000, 1.000000000000000000, 0.000000000000000000 ) ) ;
#29077=CARTESIAN_POINT ( 'NONE',  ( -1.394453263437886604E-15, 14.00000000000001776, -84.71098080242150274 ) ) ;
#29079=CARTESIAN_POINT ( 'NONE',  ( -1.655278471874999990, 20.36702641396248836, -64.93077246956615056 ) ) ;
#29080=( BOUNDED_CURVE ( )  B_SPLINE_CURVE ( 2, ( #19684, #32655, #16511, #29461, #17135, #14785, #23525, #11376, #4784 ),
 .UNSPECIFIED., .F., .T. ) 
 B_SPLINE_CURVE_WITH_KNOTS ( ( 3, 2, 2, 2, 3 ),
 ( 0.1479166666666666685, 0.1486111111111111105, 0.1499999999999999944, 0.1513888888888888784, 0.1520833333333333481 ),
 .UNSPECIFIED. ) 
 CURVE ( )  GEOMETRIC_REPRESENTATION_ITEM ( )  RATIONAL_B_SPLINE_CURVE ( ( 0.9330127018922194093, 0.9330127018922194093, 1.000000000000000000, 0.8660254037844387076, 1.000000000000000000, 0.8660254037844387076, 1.000000000000000000, 0.9330127018922180770, 0.9330127018922194093 ) ) 
 REPRESENTATION_ITEM ( '' )  );
#29082=CARTESIAN_POINT ( 'NONE',  ( -3.310556943750001313, 17.50000000000002132, -123.7641058028994649 ) ) ;
#29083=CARTESIAN_POINT ( 'NONE',  ( 4.286263797015737581E-16, 14.00000000000002487, -149.5231586289125687 ) ) ;
#29085=VERTEX_POINT ( 'NONE', #41179 ) ;
#29087=CARTESIAN_POINT ( 'NONE',  ( 0.000000000000000000, 21.00000000000002487, -149.5231586289125687 ) ) ;
#29088=CARTESIAN_POINT ( 'NONE',  ( 3.310556943750001313, 17.50000000000001776, -76.26410580289946495 ) ) ;
#29089=ORIENTED_EDGE ( 'NONE', *, *, #6979, .F. ) ;
#29090=VERTEX_POINT ( 'NONE', #2665 ) ;
#29092=CARTESIAN_POINT ( 'NONE',  ( 2.340729813953370519E-16, 21.32270188528332255, -143.0141058028994792 ) ) ;
#29094=CARTESIAN_POINT ( 'NONE',  ( -3.500000000000001332, 17.50000000000001421, -51.65473080337743284 ) ) ;
#29096=CARTESIAN_POINT ( 'NONE',  ( -3.310556943750000425, 19.41135094264165772, -40.93493913623278502 ) ) ;
#29097=EDGE_CURVE ( 'NONE', #11709, #39933, #40018, .T. ) ;
#29098=CARTESIAN_POINT ( 'NONE',  ( 3.310556943749999981, 15.58864905735837070, -105.4349391362327850 ) ) ;
#29099=AXIS2_PLACEMENT_3D ( 'NONE', #10586, #3979, #19940 ) ;
#29100=CARTESIAN_POINT ( 'NONE',  ( -3.310556943750001313, 17.50000000000001066, -29.76410580289948271 ) ) ;
#29101=CARTESIAN_POINT ( 'NONE',  ( -1.750000000000002220, 14.46891108675448656, -111.7943141357548456 ) ) ;
#29102=CARTESIAN_POINT ( 'NONE',  ( -1.750000000000002220, 14.46891108675448478, -106.7943141357548456 ) ) ;
#29105=CARTESIAN_POINT ( 'NONE',  ( -1.750000000000002220, 14.46891108675448478, -97.48806413671076143 ) ) ;
#29106=CYLINDRICAL_SURFACE ( 'NONE', #41098, 3.499999999999999556 ) ;
#29109=CARTESIAN_POINT ( 'NONE',  ( 2.474675557024783212E-16, 21.54145188432739388, -61.21098080242150274 ) ) ;
#29111=CARTESIAN_POINT ( 'NONE',  ( 3.310556943749999981, 15.58864905735836004, -23.34743913623281486 ) ) ;
#29112=CARTESIAN_POINT ( 'NONE',  ( 3.500000000000000000, 15.47927405783632082, -50.23806413671076854 ) ) ;
#29113=CARTESIAN_POINT ( 'NONE',  ( -3.500000000000001332, 17.50000000000002487, -131.9609808024214885 ) ) ;
#29114=CARTESIAN_POINT ( 'NONE',  ( 3.310556943749999981, 15.58864905735836182, -30.43493913623279568 ) ) ;
#29116=CARTESIAN_POINT ( 'NONE',  ( -1.975475456537005874E-15, 21.00000000000002487, -142.2109808024214885 ) ) ;
#29120=CARTESIAN_POINT ( 'NONE',  ( -1.655278471875002211, 14.63297358603754539, -80.59743913623280775 ) ) ;
#29121=ORIENTED_EDGE ( 'NONE', *, *, #9221, .T. ) ;
#29122=CARTESIAN_POINT ( 'NONE',  ( 0.000000000000000000, 17.50000000000002487, -149.5231586289125687 ) ) ;
#29123=( BOUNDED_CURVE ( )  B_SPLINE_CURVE ( 2, ( #22831, #35171, #9439, #41990, #41567, #6036, #22202, #38993, #32195 ),
 .UNSPECIFIED., .F., .F. ) 
 B_SPLINE_CURVE_WITH_KNOTS ( ( 3, 2, 2, 2, 3 ),
 ( 0.6437500000000000444, 0.6444444444444444864, 0.6458333333333333703, 0.6472222222222222543, 0.6479166666666666963 ),
 .UNSPECIFIED. ) 
 CURVE ( )  GEOMETRIC_REPRESENTATION_ITEM ( )  RATIONAL_B_SPLINE_CURVE ( ( 0.9330127018922194093, 0.9330127018922194093, 1.000000000000000000, 0.8660254037844387076, 1.000000000000000000, 0.8660254037844387076, 1.000000000000000000, 0.9330127018922194093, 0.9330127018922194093 ) ) 
 REPRESENTATION_ITEM ( '' )  );
#29124=CARTESIAN_POINT ( 'NONE',  ( 3.500000000000000000, 15.47927405783632970, -108.2380641367107614 ) ) ;
#29128=CARTESIAN_POINT ( 'NONE',  ( -3.310556943750000425, 19.41135094264166483, -90.84743913623279354 ) ) ;
#29130=CARTESIAN_POINT ( 'NONE',  ( 0.000000000000000000, 17.50000000000002487, -149.5231586289125687 ) ) ;
#29131=ORIENTED_EDGE ( 'NONE', *, *, #21707, .T. ) ;
#29132=VECTOR ( 'NONE', #16858, 1000.000000000000000 ) ;
#29136=CARTESIAN_POINT ( 'NONE',  ( 0.9378221735089367073, 14.00000000000002487, -129.6663226036829712 ) ) ;
#29137=VECTOR ( 'NONE', #29732, 1000.000000000000000 ) ;
#29138=CARTESIAN_POINT ( 'NONE',  ( -3.310556943750000425, 19.41135094264167549, -132.8474391362328220 ) ) ;
#29140=CARTESIAN_POINT ( 'NONE',  ( 3.369928719974892676E-15, 14.00000000000002309, -140.7109808024215170 ) ) ;
#29142=CARTESIAN_POINT ( 'NONE',  ( 1.655278471875001101, 20.36702641396249547, -118.1849391362327850 ) ) ;
#29143=CARTESIAN_POINT ( 'NONE',  ( -3.310556943750002645, 15.58864905735836714, -51.76827246956612072 ) ) ;
#29145=CARTESIAN_POINT ( 'NONE',  ( 3.500000000000001332, 17.50000000000002487, -132.1547308033774186 ) ) ;
#29146=CARTESIAN_POINT ( 'NONE',  ( -1.655278471874999990, 20.36702641396248836, -72.01827246956612782 ) ) ;
#29147=CARTESIAN_POINT ( 'NONE',  ( 1.750000000000001110, 20.53108891324555785, -122.2943141357548456 ) ) ;
#29148=CARTESIAN_POINT ( 'NONE',  ( -3.310556943750001313, 17.50000000000002132, -106.7641058028994649 ) ) ;
#29150=CYLINDRICAL_SURFACE ( 'NONE', #29975, 3.499999999999999556 ) ;
#29152=CARTESIAN_POINT ( 'NONE',  ( 2.474675557024783212E-16, 21.54145188432739744, -76.21098080242148853 ) ) ;
#29153=CARTESIAN_POINT ( 'NONE',  ( 3.500000000000001332, 17.50000000000002132, -126.1547308033774470 ) ) ;
#29154=CARTESIAN_POINT ( 'NONE',  ( 3.310556943749999981, 15.58864905735836182, -45.34743913623280775 ) ) ;
#29155=CARTESIAN_POINT ( 'NONE',  ( 2.340729813953370519E-16, 21.32270188528331190, -96.10160580289945642 ) ) ;
#29157=CARTESIAN_POINT ( 'NONE',  ( -7.424026671074350129E-16, 13.45854811567263454, -62.40473080337742573 ) ) ;
#29159=ORIENTED_EDGE ( 'NONE', *, *, #2554, .T. ) ;
#29160=CARTESIAN_POINT ( 'NONE',  ( -7.022189441860112050E-16, 13.67729811471672896, -119.6016058028994706 ) ) ;
#29161=CARTESIAN_POINT ( 'NONE',  ( 0.000000000000000000, 17.50000000000002487, -149.5231586289125687 ) ) ;
#29166=CARTESIAN_POINT ( 'NONE',  ( 1.655278471874998436, 14.63297358603754716, -99.43077246956613635 ) ) ;
#29167=CARTESIAN_POINT ( 'NONE',  ( -0.9378221735089291577, 21.00000000000001421, -52.86007260463890844 ) ) ;
#29171=VECTOR ( 'NONE', #34003, 1000.000000000000000 ) ;
#29172=CARTESIAN_POINT ( 'NONE',  ( -3.500000000000000000, 19.52072594216371826, -127.0443141357548456 ) ) ;
#29176=CARTESIAN_POINT ( 'NONE',  ( 3.310556943750001313, 17.50000000000001066, -33.26410580289947205 ) ) ;
#29185=DIRECTION ( 'NONE',  ( -0.000000000000000000, 1.259100132267607459E-16, -1.000000000000000000 ) ) ;
#29187=CARTESIAN_POINT ( 'NONE',  ( 3.500000000000001332, 17.50000000000002132, -118.1547308033774328 ) ) ;
#29189=CARTESIAN_POINT ( 'NONE',  ( -3.310556943750002645, 15.58864905735837780, -134.7682724695661420 ) ) ;
#29190=CARTESIAN_POINT ( 'NONE',  ( 1.750000000000001110, 20.53108891324554719, -34.29431413575484555 ) ) ;
#29191=CARTESIAN_POINT ( 'NONE',  ( -1.394453263437886604E-15, 14.00000000000001776, -106.7109808024215027 ) ) ;
#29192=CARTESIAN_POINT ( 'NONE',  ( 4.286263797015737581E-16, 14.00000000000002487, -149.5231586289125687 ) ) ;
#29193=AXIS2_PLACEMENT_3D ( 'NONE', #24717, #5769, #11931 ) ;
#29195=CARTESIAN_POINT ( 'NONE',  ( -1.749999999999999778, 20.53108891324556140, -137.1276474690881741 ) ) ;
#29196=CARTESIAN_POINT ( 'NONE',  ( -3.310556943750001313, 17.50000000000002132, -124.7641058028994649 ) ) ;
#29200=ADVANCED_FACE ( 'NONE', ( #29025 ), #42022, .T. ) ;
#29201=DIRECTION ( 'NONE',  ( -0.000000000000000000, 1.259100132267607459E-16, -1.000000000000000000 ) ) ;
#29202=CARTESIAN_POINT ( 'NONE',  ( 3.500000000000001332, 17.50000000000001776, -93.46098080242151696 ) ) ;
#29203=CARTESIAN_POINT ( 'NONE',  ( -0.9378221735089291577, 21.00000000000001066, -45.86007260463890844 ) ) ;
#29204=CARTESIAN_POINT ( 'NONE',  ( -3.310556943750000425, 19.41135094264166128, -58.84743913623280065 ) ) ;
#29205=CARTESIAN_POINT ( 'NONE',  ( -1.655278471874999990, 20.36702641396249547, -115.0182724695661278 ) ) ;
#29206=EDGE_CURVE ( 'NONE', #3989, #4551, #6278, .T. ) ;
#29207=CARTESIAN_POINT ( 'NONE',  ( 4.286263797015737581E-16, 14.00000000000002487, -149.5231586289125687 ) ) ;
#29208=CARTESIAN_POINT ( 'NONE',  ( -3.500000000000002220, 15.47927405783632082, -33.57139747004410424 ) ) ;
#29209=CYLINDRICAL_SURFACE ( 'NONE', #18578, 3.499999999999999556 ) ;
#29211=CARTESIAN_POINT ( 'NONE',  ( -3.310556943750001313, 17.50000000000002487, -133.8516058028994564 ) ) ;
#29215=CARTESIAN_POINT ( 'NONE',  ( 1.655278471874998436, 14.63297358603754184, -67.51827246956612782 ) ) ;
#29218=CARTESIAN_POINT ( 'NONE',  ( -1.655278471875002211, 14.63297358603754361, -66.59743913623280775 ) ) ;
#29219=VERTEX_POINT ( 'NONE', #38816 ) ;
#29220=CARTESIAN_POINT ( 'NONE',  ( 2.340729813953370519E-16, 21.32270188528331190, -85.10160580289947063 ) ) ;
#29223=CARTESIAN_POINT ( 'NONE',  ( 0.9378221735089300459, 21.00000000000002487, -131.2556390011600342 ) ) ;
#29224=CARTESIAN_POINT ( 'NONE',  ( -7.022189441860112050E-16, 13.67729811471671830, -48.51410580289947205 ) ) ;
#29226=CARTESIAN_POINT ( 'NONE',  ( 3.310556943750001313, 17.50000000000002132, -108.2641058028994649 ) ) ;
#29233=CARTESIAN_POINT ( 'NONE',  ( 3.310556943750001313, 19.41135094264166128, -59.18077246956614346 ) ) ;
#29234=ORIENTED_EDGE ( 'NONE', *, *, #8792, .F. ) ;
#29236=( BOUNDED_CURVE ( )  B_SPLINE_CURVE ( 2, ( #7753, #20728, #33703, #11156, #24138, #7962, #26682, #40496, #4761 ),
 .UNSPECIFIED., .F., .T. ) 
 B_SPLINE_CURVE_WITH_KNOTS ( ( 3, 2, 2, 2, 3 ),
 ( 0.8229166666666666297, 0.8236111111111110716, 0.8249999999999999556, 0.8263888888888888395, 0.8270833333333332815 ),
 .UNSPECIFIED. ) 
 CURVE ( )  GEOMETRIC_REPRESENTATION_ITEM ( )  RATIONAL_B_SPLINE_CURVE ( ( 0.9330127018922194093, 0.9330127018922194093, 1.000000000000000000, 0.8660254037844387076, 1.000000000000000000, 0.8660254037844387076, 1.000000000000000000, 0.9330127018922194093, 0.9330127018922194093 ) ) 
 REPRESENTATION_ITEM ( '' )  );
#29239=EDGE_CURVE ( 'NONE', #31100, #15353, #18526, .T. ) ;
#29244=CARTESIAN_POINT ( 'NONE',  ( -3.500000000000001332, 17.50000000000002487, -138.9609808024214885 ) ) ;
#29245=CARTESIAN_POINT ( 'NONE',  ( 3.310556943749999981, 15.58864905735837425, -125.3474391362328078 ) ) ;
#29247=CARTESIAN_POINT ( 'NONE',  ( -0.9378221735089136146, 14.00000000000001066, -117.4493890021159501 ) ) ;
#29249=CARTESIAN_POINT ( 'NONE',  ( 3.310556943750001313, 17.50000000000001066, -34.35160580289946353 ) ) ;
#29250=CARTESIAN_POINT ( 'NONE',  ( -1.655278471874999990, 20.36702641396248481, -27.01827246956613138 ) ) ;
#29251=CARTESIAN_POINT ( 'NONE',  ( 3.310556943750001313, 17.50000000000001776, -85.35160580289947063 ) ) ;
#29252=CARTESIAN_POINT ( 'NONE',  ( -7.022189441860112050E-16, 13.67729811471672896, -140.5141058028994792 ) ) ;
#29254=LINE ( 'NONE', #128, #15942 ) ;
#29255=CARTESIAN_POINT ( 'NONE',  ( -3.500000000000001332, 17.50000000000001421, -66.96098080242150274 ) ) ;
#29258=CARTESIAN_POINT ( 'NONE',  ( 3.310556943749999981, 15.58864905735837425, -131.4349391362327992 ) ) ;
#29260=CARTESIAN_POINT ( 'NONE',  ( -3.310556943750002645, 15.58864905735837247, -90.68077246956613635 ) ) ;
#29261=CARTESIAN_POINT ( 'NONE',  ( 1.750000000000001110, 20.53108891324554719, -27.98806413671076143 ) ) ;
#29262=FACE_OUTER_BOUND ( 'NONE', #39232, .T. ) ;
#29263=CARTESIAN_POINT ( 'NONE',  ( 3.500000000000000000, 15.47927405783633326, -111.5443141357548456 ) ) ;
#29264=CARTESIAN_POINT ( 'NONE',  ( -1.749999999999999778, 20.53108891324555074, -72.82139747004409003 ) ) ;
#29265=CARTESIAN_POINT ( 'NONE',  ( 3.310556943750001313, 19.41135094264166483, -59.26827246956613493 ) ) ;
#29269=CARTESIAN_POINT ( 'NONE',  ( -7.022189441860112050E-16, 13.67729811471672363, -85.60160580289947063 ) ) ;
#29271=CARTESIAN_POINT ( 'NONE',  ( -7.022189441860112050E-16, 13.67729811471672896, -116.5141058028994792 ) ) ;
#29272=CARTESIAN_POINT ( 'NONE',  ( -3.310556943750002645, 15.58864905735837070, -80.68077246956613635 ) ) ;
#29273=CARTESIAN_POINT ( 'NONE',  ( -3.500000000000002220, 15.47927405783633326, -96.57139747004409003 ) ) ;
#29274=ORIENTED_EDGE ( 'NONE', *, *, #35988, .T. ) ;
#29275=CARTESIAN_POINT ( 'NONE',  ( 1.655278471874998436, 14.63297358603754716, -99.51827246956612782 ) ) ;
#29276=CARTESIAN_POINT ( 'NONE',  ( 3.500000000000000000, 15.47927405783632793, -105.2380641367107614 ) ) ;
#29280=CARTESIAN_POINT ( 'NONE',  ( 3.500000000000001332, 19.52072594216371115, -88.07139747004409003 ) ) ;
#29284=CARTESIAN_POINT ( 'NONE',  ( 3.310556943749999981, 15.58864905735836537, -67.34743913623280775 ) ) ;
#29286=CARTESIAN_POINT ( 'NONE',  ( -7.022189441860112050E-16, 13.67729811471672718, -122.5141058028994934 ) ) ;
#29288=CYLINDRICAL_SURFACE ( 'NONE', #3980, 3.499999999999999556 ) ;
#29290=ORIENTED_EDGE ( 'NONE', *, *, #34527, .F. ) ;
#29292=CARTESIAN_POINT ( 'NONE',  ( 3.500000000000001332, 17.50000000000002132, -128.1547308033774186 ) ) ;
#29293=CARTESIAN_POINT ( 'NONE',  ( 1.655278471874998436, 14.63297358603754361, -74.43077246956613635 ) ) ;
#29303=CARTESIAN_POINT ( 'NONE',  ( -3.500000000000002220, 15.47927405783632970, -89.57139747004409003 ) ) ;
#29304=CARTESIAN_POINT ( 'NONE',  ( 3.310556943750001313, 19.41135094264165772, -42.26827246956612782 ) ) ;
#29305=CARTESIAN_POINT ( 'NONE',  ( 3.310556943750001313, 19.41135094264166838, -106.2682724695661278 ) ) ;
#29306=CARTESIAN_POINT ( 'NONE',  ( -3.310556943750002645, 15.58864905735836537, -27.68077246956613990 ) ) ;
#29308=CARTESIAN_POINT ( 'NONE',  ( 2.474675557024783212E-16, 21.54145188432740099, -103.2109808024214885 ) ) ;
#29311=CARTESIAN_POINT ( 'NONE',  ( 2.474675557024783212E-16, 21.54145188432739744, -92.90473080337743284 ) ) ;
#29313=( BOUNDED_CURVE ( )  B_SPLINE_CURVE ( 2, ( #12456, #2461, #25648, #9694, #28817, #19046, #19256, #26063, #22233 ),
 .UNSPECIFIED., .F., .T. ) 
 B_SPLINE_CURVE_WITH_KNOTS ( ( 3, 2, 2, 2, 3 ),
 ( 0.8437500000000000000, 0.8444444444444444420, 0.8458333333333333259, 0.8472222222222222099, 0.8479166666666666519 ),
 .UNSPECIFIED. ) 
 CURVE ( )  GEOMETRIC_REPRESENTATION_ITEM ( )  RATIONAL_B_SPLINE_CURVE ( ( 0.9330127018922194093, 0.9330127018922194093, 1.000000000000000000, 0.8660254037844387076, 1.000000000000000000, 0.8660254037844387076, 1.000000000000000000, 0.9330127018922194093, 0.9330127018922194093 ) ) 
 REPRESENTATION_ITEM ( '' )  );
#29316=CARTESIAN_POINT ( 'NONE',  ( 3.500000000000001332, 17.50000000000001421, -58.46098080242151696 ) ) ;
#29318=CARTESIAN_POINT ( 'NONE',  ( -0.9378221735089291577, 21.00000000000001066, -25.16632260368298546 ) ) ;
#29320=CARTESIAN_POINT ( 'NONE',  ( -1.749999999999999778, 20.53108891324555074, -46.82139747004410424 ) ) ;
#29321=CARTESIAN_POINT ( 'NONE',  ( -1.394453263437886604E-15, 14.00000000000002132, -131.7109808024214885 ) ) ;
#29322=EDGE_CURVE ( 'NONE', #20461, #32026, #25361, .T. ) ;
#29323=CARTESIAN_POINT ( 'NONE',  ( 1.655278471874998436, 14.63297358603753828, -26.51827246956613138 ) ) ;
#29326=FACE_OUTER_BOUND ( 'NONE', #5934, .T. ) ;
#29330=CARTESIAN_POINT ( 'NONE',  ( -1.655278471875002211, 14.63297358603754716, -84.59743913623279354 ) ) ;
#29332=ORIENTED_EDGE ( 'NONE', *, *, #23772, .F. ) ;
#29333=LINE ( 'NONE', #19773, #36649 ) ;
#29334=EDGE_LOOP ( 'NONE', ( #3088, #6904, #5503, #17662 ) ) ;
#29335=EDGE_CURVE ( 'NONE', #10439, #15570, #33705, .T. ) ;
#29336=VECTOR ( 'NONE', #10998, 1000.000000000000000 ) ;
#29337=DIRECTION ( 'NONE',  ( -0.000000000000000000, 1.259100132267607459E-16, -1.000000000000000000 ) ) ;
#29338=CARTESIAN_POINT ( 'NONE',  ( -3.310556943750001313, 17.50000000000001776, -90.76410580289947916 ) ) ;
#29343=CARTESIAN_POINT ( 'NONE',  ( 0.9378221735089281585, 14.00000000000001243, -66.66632260368298546 ) ) ;
#29346=CARTESIAN_POINT ( 'NONE',  ( -1.836030130193217234E-14, 21.00000000000002132, -129.2109808024214601 ) ) ;
#29347=CARTESIAN_POINT ( 'NONE',  ( -3.310556943750002645, 15.58864905735837780, -131.6807724695661364 ) ) ;
#29348=ORIENTED_EDGE ( 'NONE', *, *, #15304, .F. ) ;
#29350=CARTESIAN_POINT ( 'NONE',  ( 3.500000000000001332, 17.50000000000001421, -73.15473080337743284 ) ) ;
#29351=CARTESIAN_POINT ( 'NONE',  ( -3.310556943750000425, 19.41135094264166838, -119.9349391362327850 ) ) ;
#29352=VERTEX_POINT ( 'NONE', #7755 ) ;
#29354=CARTESIAN_POINT ( 'NONE',  ( 3.500000000000001776, 19.52072594216372181, -133.0713974700441042 ) ) ;
#29357=CARTESIAN_POINT ( 'NONE',  ( 3.310556943750001313, 17.50000000000001421, -73.35160580289947063 ) ) ;
#29358=CARTESIAN_POINT ( 'NONE',  ( -1.750000000000002220, 14.46891108675448656, -120.7943141357548313 ) ) ;
#29360=CARTESIAN_POINT ( 'NONE',  ( 3.310556943749999981, 15.58864905735837070, -100.3474391362328220 ) ) ;
#29361=AXIS2_PLACEMENT_3D ( 'NONE', #17521, #1566, #33890 ) ;
#29365=CARTESIAN_POINT ( 'NONE',  ( 3.500000000000001776, 19.52072594216370760, -73.37764746908817415 ) ) ;
#29367=CARTESIAN_POINT ( 'NONE',  ( -7.022189441860112050E-16, 13.67729811471671475, -39.51410580289947916 ) ) ;
#29368=( BOUNDED_CURVE ( )  B_SPLINE_CURVE ( 2, ( #10978, #30962, #30115, #24375, #36931, #23964, #13960, #30536, #24584 ),
 .UNSPECIFIED., .F., .T. ) 
 B_SPLINE_CURVE_WITH_KNOTS ( ( 3, 2, 2, 2, 3 ),
 ( 0.6312499999999999778, 0.6319444444444444198, 0.6333333333333333037, 0.6347222222222221877, 0.6354166666666666297 ),
 .UNSPECIFIED. ) 
 CURVE ( )  GEOMETRIC_REPRESENTATION_ITEM ( )  RATIONAL_B_SPLINE_CURVE ( ( 0.9330127018922194093, 0.9330127018922194093, 1.000000000000000000, 0.8660254037844387076, 1.000000000000000000, 0.8660254037844387076, 1.000000000000000000, 0.9330127018922194093, 0.9330127018922194093 ) ) 
 REPRESENTATION_ITEM ( '' )  );
#29369=CARTESIAN_POINT ( 'NONE',  ( -3.310556943750002645, 15.58864905735837425, -95.76827246956612782 ) ) ;
#29370=CARTESIAN_POINT ( 'NONE',  ( 2.474675557024783212E-16, 21.54145188432739388, -66.90473080337743284 ) ) ;
#29372=CARTESIAN_POINT ( 'NONE',  ( -1.655278471874999990, 20.36702641396249547, -117.0182724695661278 ) ) ;
#29373=CARTESIAN_POINT ( 'NONE',  ( -1.394453263437886604E-15, 14.00000000000001066, -27.71098080242150985 ) ) ;
#29378=CARTESIAN_POINT ( 'NONE',  ( -3.310556943750001313, 17.50000000000001776, -96.76410580289947916 ) ) ;
#29379=CARTESIAN_POINT ( 'NONE',  ( 4.648177544792955347E-16, 21.00000000000001776, -96.90473080337741862 ) ) ;
#29385=ORIENTED_EDGE ( 'NONE', *, *, #22007, .T. ) ;
#29388=ADVANCED_FACE ( 'NONE', ( #4347 ), #28352, .T. ) ;
#29390=CARTESIAN_POINT ( 'NONE',  ( -1.655278471875002211, 14.63297358603754006, -26.59743913623280420 ) ) ;
#29396=CARTESIAN_POINT ( 'NONE',  ( -1.749999999999999778, 20.53108891324555074, -58.12764746908817415 ) ) ;
#29397=VECTOR ( 'NONE', #28262, 1000.000000000000000 ) ;
#29401=LINE ( 'NONE', #10269, #39436 ) ;
#29402=CARTESIAN_POINT ( 'NONE',  ( 1.750000000000001110, 20.53108891324555785, -120.9880641367107614 ) ) ;
#29404=CARTESIAN_POINT ( 'NONE',  ( -1.655278471874999990, 20.36702641396249902, -136.0182724695661420 ) ) ;
#29405=CARTESIAN_POINT ( 'NONE',  ( -7.424026671074350129E-16, 13.45854811567263098, -27.71098080242151340 ) ) ;
#29409=CARTESIAN_POINT ( 'NONE',  ( -1.975475456537005874E-15, 21.00000000000002487, -142.2109808024214885 ) ) ;
#29411=CARTESIAN_POINT ( 'NONE',  ( -1.750000000000002220, 14.46891108675449011, -136.7943141357548598 ) ) ;
#29412=CARTESIAN_POINT ( 'NONE',  ( -3.310556943750001313, 17.50000000000002132, -120.7641058028994792 ) ) ;
#29416=CARTESIAN_POINT ( 'NONE',  ( -3.500000000000001332, 17.50000000000001776, -91.96098080242151696 ) ) ;
#29417=CARTESIAN_POINT ( 'NONE',  ( -0.9378221735089310451, 14.00000000000001066, -36.75563900116003424 ) ) ;
#29418=CARTESIAN_POINT ( 'NONE',  ( 1.655278471875001101, 20.36702641396248836, -56.09743913623280065 ) ) ;
#29419=CARTESIAN_POINT ( 'NONE',  ( 3.310556943750001313, 17.50000000000002132, -114.3516058028994706 ) ) ;
#29420=CARTESIAN_POINT ( 'NONE',  ( -0.9378221735089310451, 14.00000000000002309, -121.7556390011600485 ) ) ;
#29421=CARTESIAN_POINT ( 'NONE',  ( -1.750000000000002220, 14.46891108675447590, -32.48806413671076143 ) ) ;
#29424=CARTESIAN_POINT ( 'NONE',  ( 2.340729813953370519E-16, 21.32270188528332255, -132.1016058028994564 ) ) ;
#29425=VECTOR ( 'NONE', #35304, 1000.000000000000000 ) ;
#29430=CARTESIAN_POINT ( 'NONE',  ( 1.655278471874998436, 14.63297358603754184, -62.51827246956613493 ) ) ;
#29432=CARTESIAN_POINT ( 'NONE',  ( 3.310556943750001313, 19.41135094264166128, -65.18077246956615056 ) ) ;
#29433=ORIENTED_EDGE ( 'NONE', *, *, #23272, .T. ) ;
#29434=CARTESIAN_POINT ( 'NONE',  ( -3.310556943750002201, 15.58864905735837247, -84.76827246956612782 ) ) ;
#29437=CARTESIAN_POINT ( 'NONE',  ( -0.9378221735089291577, 21.00000000000001066, -40.16632260368298546 ) ) ;
#29439=CARTESIAN_POINT ( 'NONE',  ( -1.655278471875002211, 14.63297358603754184, -45.59743913623280775 ) ) ;
#29441=CARTESIAN_POINT ( 'NONE',  ( -3.310556943750002645, 15.58864905735837425, -104.6807724695661364 ) ) ;
#29443=VERTEX_POINT ( 'NONE', #25179 ) ;
#29448=CARTESIAN_POINT ( 'NONE',  ( 1.655278471874998436, 14.63297358603754184, -57.43077246956614346 ) ) ;
#29449=ORIENTED_EDGE ( 'NONE', *, *, #40047, .T. ) ;
#29450=ORIENTED_EDGE ( 'NONE', *, *, #29335, .T. ) ;
#29452=CARTESIAN_POINT ( 'NONE',  ( 0.000000000000000000, 17.50000000000002487, -149.5231586289125687 ) ) ;
#29457=CARTESIAN_POINT ( 'NONE',  ( 1.750000000000001110, 20.53108891324555074, -46.98806413671076143 ) ) ;
#29460=CARTESIAN_POINT ( 'NONE',  ( 1.655278471875001101, 20.36702641396249547, -127.0974391362328078 ) ) ;
#29461=CARTESIAN_POINT ( 'NONE',  ( 3.500000000000000000, 15.47927405783633503, -125.5443141357548456 ) ) ;
#29464=CARTESIAN_POINT ( 'NONE',  ( 3.310556943749999981, 15.58864905735836182, -36.43493913623279923 ) ) ;
#29465=CARTESIAN_POINT ( 'NONE',  ( 1.655278471875001101, 20.36702641396248481, -24.18493913623280633 ) ) ;
#29466=CARTESIAN_POINT ( 'NONE',  ( 3.310556943750001313, 19.41135094264166483, -87.26827246956612782 ) ) ;
#29467=CARTESIAN_POINT ( 'NONE',  ( -7.022189441860112050E-16, 13.67729811471672896, -139.5141058028994507 ) ) ;
#29471=CARTESIAN_POINT ( 'NONE',  ( -0.9378221735089310451, 14.00000000000002132, -100.4493890021159643 ) ) ;
#29472=CARTESIAN_POINT ( 'NONE',  ( 3.310556943750001313, 17.50000000000002132, -126.3516058028994706 ) ) ;
#29474=CARTESIAN_POINT ( 'NONE',  ( -3.310556943750000425, 19.41135094264166483, -90.84743913623279354 ) ) ;
#29477=CARTESIAN_POINT ( 'NONE',  ( -1.394453263437886604E-15, 14.00000000000000711, -23.40473080337742928 ) ) ;
#29478=CARTESIAN_POINT ( 'NONE',  ( 1.750000000000001110, 20.53108891324555429, -75.98806413671076143 ) ) ;
#29479=ADVANCED_FACE ( 'NONE', ( #24546 ), #5387, .T. ) ;
#29480=CARTESIAN_POINT ( 'NONE',  ( 1.655278471874998436, 14.63297358603754184, -58.51827246956613493 ) ) ;
#29484=CARTESIAN_POINT ( 'NONE',  ( -7.022189441860112050E-16, 13.67729811471672363, -86.60160580289945642 ) ) ;
#29485=DIRECTION ( 'NONE',  ( -0.000000000000000000, 1.259100132267607459E-16, -1.000000000000000000 ) ) ;
#29487=CARTESIAN_POINT ( 'NONE',  ( 2.340729813953370519E-16, 21.32270188528331900, -111.0141058028994649 ) ) ;
#29488=CARTESIAN_POINT ( 'NONE',  ( 3.310556943749999981, 15.58864905735836714, -80.34743913623279354 ) ) ;
#29489=DIRECTION ( 'NONE',  ( 0.000000000000000000, 1.000000000000000000, 0.000000000000000000 ) ) ;
#29491=CARTESIAN_POINT ( 'NONE',  ( -3.310556943750000425, 19.41135094264166838, -103.9349391362328134 ) ) ;
#29493=CARTESIAN_POINT ( 'NONE',  ( 3.500000000000000000, 15.47927405783632793, -103.2380641367107756 ) ) ;
#29496=CARTESIAN_POINT ( 'NONE',  ( 1.750000000000001110, 20.53108891324555429, -87.98806413671076143 ) ) ;
#29499=CARTESIAN_POINT ( 'NONE',  ( 2.340729813953370519E-16, 21.32270188528331190, -64.01410580289946495 ) ) ;
#29500=CARTESIAN_POINT ( 'NONE',  ( -0.9378221735089310451, 14.00000000000001066, -29.75563900116003069 ) ) ;
#29501=CARTESIAN_POINT ( 'NONE',  ( -1.655278471875002211, 14.63297358603755249, -123.5974391362328078 ) ) ;
#29503=( BOUNDED_CURVE ( )  B_SPLINE_CURVE ( 2, ( #42007, #41582, #6478, #6266, #28799, #12858, #22639, #22218, #25838 ),
 .UNSPECIFIED., .F., .T. ) 
 B_SPLINE_CURVE_WITH_KNOTS ( ( 3, 2, 2, 2, 3 ),
 ( 0.2854166666666666519, 0.2861111111111110938, 0.2874999999999999778, 0.2888888888888888618, 0.2895833333333333592 ),
 .UNSPECIFIED. ) 
 CURVE ( )  GEOMETRIC_REPRESENTATION_ITEM ( )  RATIONAL_B_SPLINE_CURVE ( ( 0.9330127018922194093, 0.9330127018922194093, 1.000000000000000000, 0.8660254037844387076, 1.000000000000000000, 0.8660254037844387076, 1.000000000000000000, 0.9330127018922167448, 0.9330127018922194093 ) ) 
 REPRESENTATION_ITEM ( '' )  );
#29505=ORIENTED_EDGE ( 'NONE', *, *, #12685, .F. ) ;
#29506=AXIS2_PLACEMENT_3D ( 'NONE', #21852, #9516, #31216 ) ;
#29510=CARTESIAN_POINT ( 'NONE',  ( 3.310556943750001313, 19.41135094264166128, -74.18077246956613635 ) ) ;
#29511=VERTEX_POINT ( 'NONE', #8368 ) ;
#29512=EDGE_LOOP ( 'NONE', ( #26638, #30778, #23620, #7248 ) ) ;
#29514=CARTESIAN_POINT ( 'NONE',  ( -1.394453263437886604E-15, 14.00000000000001066, -53.40473080337743284 ) ) ;
#29515=EDGE_CURVE ( 'NONE', #3516, #19149, #29947, .T. ) ;
#29517=CARTESIAN_POINT ( 'NONE',  ( 3.310556943750001313, 19.41135094264167549, -140.1807724695661364 ) ) ;
#29518=CARTESIAN_POINT ( 'NONE',  ( -3.500000000000000000, 19.52072594216371826, -129.0443141357548313 ) ) ;
#29522=CARTESIAN_POINT ( 'NONE',  ( 1.655278471874998436, 14.63297358603753828, -36.51827246956612782 ) ) ;
#29523=CARTESIAN_POINT ( 'NONE',  ( 3.310556943749999981, 15.58864905735837070, -106.4349391362327992 ) ) ;
#29524=CARTESIAN_POINT ( 'NONE',  ( -3.310556943750000425, 19.41135094264165772, -29.84743913623280420 ) ) ;
#29527=CARTESIAN_POINT ( 'NONE',  ( 1.749999999999998224, 14.46891108675448301, -99.62764746908817415 ) ) ;
#29529=DIRECTION ( 'NONE',  ( -0.000000000000000000, 1.259100132267607459E-16, -1.000000000000000000 ) ) ;
#29530=CARTESIAN_POINT ( 'NONE',  ( -3.500000000000002220, 15.47927405783632793, -93.57139747004409003 ) ) ;
#29536=CARTESIAN_POINT ( 'NONE',  ( 1.750000000000001110, 20.53108891324555074, -52.29431413575484555 ) ) ;
#29540=CARTESIAN_POINT ( 'NONE',  ( 3.500000000000000000, 15.47927405783632082, -41.23806413671076143 ) ) ;
#29542=CARTESIAN_POINT ( 'NONE',  ( 3.310556943750001313, 19.41135094264166128, -26.26827246956613138 ) ) ;
#29544=DIRECTION ( 'NONE',  ( -0.000000000000000000, 1.259100132267607459E-16, -1.000000000000000000 ) ) ;
#29549=CARTESIAN_POINT ( 'NONE',  ( 3.310556943750001313, 19.41135094264166838, -82.18077246956616477 ) ) ;
#29550=CARTESIAN_POINT ( 'NONE',  ( 1.045839947578414805E-15, 14.00000000000002665, -141.4047308033774470 ) ) ;
#29552=CARTESIAN_POINT ( 'NONE',  ( -3.500000000000000000, 19.52072594216370405, -35.73806413671076854 ) ) ;
#29553=CARTESIAN_POINT ( 'NONE',  ( -0.9378221735089310451, 14.00000000000001599, -64.75563900116003424 ) ) ;
#29554=VECTOR ( 'NONE', #14989, 1000.000000000000000 ) ;
#29555=ORIENTED_EDGE ( 'NONE', *, *, #4443, .T. ) ;
#29557=CARTESIAN_POINT ( 'NONE',  ( -1.655278471874999990, 20.36702641396249192, -91.93077246956613635 ) ) ;
#29558=ORIENTED_EDGE ( 'NONE', *, *, #5842, .F. ) ;
#29563=DIRECTION ( 'NONE',  ( -0.000000000000000000, 1.259100132267607459E-16, -1.000000000000000000 ) ) ;
#29564=DIRECTION ( 'NONE',  ( -0.000000000000000000, 1.259100132267607459E-16, -1.000000000000000000 ) ) ;
#29565=EDGE_CURVE ( 'NONE', #13615, #22667, #24248, .T. ) ;
#29566=CARTESIAN_POINT ( 'NONE',  ( 3.310556943750001313, 19.41135094264167549, -130.1807724695661364 ) ) ;
#29567=ORIENTED_EDGE ( 'NONE', *, *, #30308, .F. ) ;
#29571=CARTESIAN_POINT ( 'NONE',  ( 1.655278471875001101, 20.36702641396249547, -120.1849391362327992 ) ) ;
#29574=CARTESIAN_POINT ( 'NONE',  ( -1.749999999999999778, 20.53108891324556140, -132.8213974700441042 ) ) ;
#29575=CARTESIAN_POINT ( 'NONE',  ( 1.655278471874998436, 14.63297358603754361, -70.51827246956612782 ) ) ;
#29576=CARTESIAN_POINT ( 'NONE',  ( 3.500000000000001776, 19.52072594216371826, -116.3776474690881741 ) ) ;
#29577=CARTESIAN_POINT ( 'NONE',  ( -3.310556943750002645, 15.58864905735837425, -100.6807724695661364 ) ) ;
#29580=CARTESIAN_POINT ( 'NONE',  ( 0.9378221735089300459, 21.00000000000002132, -105.2556390011600342 ) ) ;
#29582=CARTESIAN_POINT ( 'NONE',  ( 3.500000000000000000, 15.47927405783632437, -71.54431413575483134 ) ) ;
#29583=CARTESIAN_POINT ( 'NONE',  ( 4.648177544792955347E-16, 21.00000000000001421, -51.21098080242150274 ) ) ;
#29584=CARTESIAN_POINT ( 'NONE',  ( 1.655278471874998436, 14.63297358603753828, -38.43077246956613635 ) ) ;
#29585=CARTESIAN_POINT ( 'NONE',  ( -7.022189441860112050E-16, 13.67729811471672541, -95.60160580289945642 ) ) ;
#29586=CARTESIAN_POINT ( 'NONE',  ( 3.500000000000001332, 17.50000000000001421, -57.15473080337743284 ) ) ;
#29587=VECTOR ( 'NONE', #15363, 1000.000000000000000 ) ;
#29588=CARTESIAN_POINT ( 'NONE',  ( -3.310556943750002201, 15.58864905735837780, -117.7682724695661420 ) ) ;
#29595=CARTESIAN_POINT ( 'NONE',  ( -3.310556943750000425, 19.41135094264166838, -95.84743913623280775 ) ) ;
#29596=CARTESIAN_POINT ( 'NONE',  ( 1.749999999999998224, 14.46891108675447768, -62.62764746908818125 ) ) ;
#29599=CARTESIAN_POINT ( 'NONE',  ( 7.785697387528201340E-15, 14.00000000000002487, -136.7109808024214885 ) ) ;
#29600=CARTESIAN_POINT ( 'NONE',  ( 3.500000000000001332, 17.50000000000001776, -81.46098080242150274 ) ) ;
#29601=DIRECTION ( 'NONE',  ( 0.000000000000000000, 1.000000000000000000, 0.000000000000000000 ) ) ;
#29602=ORIENTED_EDGE ( 'NONE', *, *, #22052, .F. ) ;
#29606=CARTESIAN_POINT ( 'NONE',  ( 1.655278471875001101, 20.36702641396248481, -29.09743913623280420 ) ) ;
#29607=VERTEX_POINT ( 'NONE', #24503 ) ;
#29608=FACE_OUTER_BOUND ( 'NONE', #23631, .T. ) ;
#29615=CARTESIAN_POINT ( 'NONE',  ( 3.500000000000000000, 15.47927405783632082, -31.23806413671076498 ) ) ;
#29617=CARTESIAN_POINT ( 'NONE',  ( -1.750000000000002220, 14.46891108675448656, -120.4880641367107614 ) ) ;
#29618=CARTESIAN_POINT ( 'NONE',  ( -3.500000000000002220, 15.47927405783633503, -135.8776474690881741 ) ) ;
#29619=CARTESIAN_POINT ( 'NONE',  ( 2.340729813953370519E-16, 21.32270188528332255, -138.1016058028994564 ) ) ;
#29620=CARTESIAN_POINT ( 'NONE',  ( 2.474675557024783212E-16, 21.54145188432739033, -30.21098080242151696 ) ) ;
#29622=DIRECTION ( 'NONE',  ( -0.000000000000000000, 1.259100132267607459E-16, -1.000000000000000000 ) ) ;
#29623=( BOUNDED_CURVE ( )  B_SPLINE_CURVE ( 2, ( #48, #13434, #3651, #7057, #33002, #19816, #12816, #26419, #28970 ),
 .UNSPECIFIED., .F., .T. ) 
 B_SPLINE_CURVE_WITH_KNOTS ( ( 3, 2, 2, 2, 3 ),
 ( 0.4604166666666666963, 0.4611111111111111382, 0.4625000000000000222, 0.4638888888888889062, 0.4645833333333333481 ),
 .UNSPECIFIED. ) 
 CURVE ( )  GEOMETRIC_REPRESENTATION_ITEM ( )  RATIONAL_B_SPLINE_CURVE ( ( 0.9330127018922194093, 0.9330127018922220739, 1.000000000000000000, 0.8660254037844387076, 1.000000000000000000, 0.8660254037844387076, 1.000000000000000000, 0.9330127018922194093, 0.9330127018922194093 ) ) 
 REPRESENTATION_ITEM ( '' )  );
#29624=CARTESIAN_POINT ( 'NONE',  ( 3.500000000000000000, 15.47927405783632082, -37.23806413671076143 ) ) ;
#29626=CARTESIAN_POINT ( 'NONE',  ( 3.500000000000001332, 17.50000000000002487, -134.4609808024214885 ) ) ;
#29627=CARTESIAN_POINT ( 'NONE',  ( -7.022189441860112050E-16, 13.67729811471672718, -118.5141058028994792 ) ) ;
#29631=CARTESIAN_POINT ( 'NONE',  ( 4.648177544792955347E-16, 21.00000000000001776, -82.21098080242150274 ) ) ;
#29632=CARTESIAN_POINT ( 'NONE',  ( -1.750000000000002220, 14.46891108675448301, -88.79431413575483134 ) ) ;
#29634=CARTESIAN_POINT ( 'NONE',  ( 1.655278471874998436, 14.63297358603754006, -51.43077246956613635 ) ) ;
#29635=CARTESIAN_POINT ( 'NONE',  ( -3.310556943750002645, 15.58864905735837780, -111.7682724695661420 ) ) ;
#29636=CARTESIAN_POINT ( 'NONE',  ( 3.500000000000001332, 17.50000000000001066, -38.46098080242150985 ) ) ;
#29637=CARTESIAN_POINT ( 'NONE',  ( -3.500000000000002220, 15.47927405783632082, -27.57139747004409713 ) ) ;
#29638=CARTESIAN_POINT ( 'NONE',  ( 1.749999999999998224, 14.46891108675448478, -116.6276474690881741 ) ) ;
#29640=CARTESIAN_POINT ( 'NONE',  ( 3.310556943750001313, 19.41135094264167549, -131.2682724695661136 ) ) ;
#29642=CARTESIAN_POINT ( 'NONE',  ( 4.648177544792955347E-16, 21.00000000000001421, -66.90473080337743284 ) ) ;
#29643=DIRECTION ( 'NONE',  ( 0.000000000000000000, 1.000000000000000000, 0.000000000000000000 ) ) ;
#29644=CARTESIAN_POINT ( 'NONE',  ( -3.310556943750002645, 15.58864905735836892, -62.76827246956612782 ) ) ;
#29646=CARTESIAN_POINT ( 'NONE',  ( -1.655278471875002211, 14.63297358603754361, -64.59743913623280775 ) ) ;
#29648=CARTESIAN_POINT ( 'NONE',  ( -3.310556943750000425, 19.41135094264166838, -83.93493913623278502 ) ) ;
#29650=CARTESIAN_POINT ( 'NONE',  ( -1.394453263437886604E-15, 14.00000000000001066, -39.71098080242150985 ) ) ;
#29652=CARTESIAN_POINT ( 'NONE',  ( -3.310556943750002201, 15.58864905735836714, -44.68077246956615056 ) ) ;
#29654=CARTESIAN_POINT ( 'NONE',  ( 1.655278471874998436, 14.63297358603754716, -98.43077246956613635 ) ) ;
#29655=CARTESIAN_POINT ( 'NONE',  ( 0.000000000000000000, 17.50000000000002487, -149.5231586289125687 ) ) ;
#29658=ORIENTED_EDGE ( 'NONE', *, *, #6449, .T. ) ;
#29660=AXIS2_PLACEMENT_3D ( 'NONE', #12551, #38501, #28705 ) ;
#29661=CARTESIAN_POINT ( 'NONE',  ( 3.310556943750001313, 17.50000000000001421, -60.26410580289947916 ) ) ;
#29665=CARTESIAN_POINT ( 'NONE',  ( 4.648177544792955347E-16, 21.00000000000001066, -24.21098080242150985 ) ) ;
#29666=CARTESIAN_POINT ( 'NONE',  ( 1.749999999999998224, 14.46891108675447413, -31.62764746908818125 ) ) ;
#29669=CARTESIAN_POINT ( 'NONE',  ( -3.500000000000000000, 19.52072594216371826, -140.7380641367107614 ) ) ;
#29670=ORIENTED_EDGE ( 'NONE', *, *, #14798, .F. ) ;
#29672=CARTESIAN_POINT ( 'NONE',  ( 3.500000000000000000, 15.47927405783632082, -43.54431413575483845 ) ) ;
#29673=CARTESIAN_POINT ( 'NONE',  ( 3.310556943750001313, 19.41135094264165772, -44.18077246956614346 ) ) ;
#29674=CARTESIAN_POINT ( 'NONE',  ( 3.500000000000001332, 19.52072594216370405, -35.07139747004410424 ) ) ;
#29676=CARTESIAN_POINT ( 'NONE',  ( -1.394453263437886604E-15, 14.00000000000001776, -104.4047308033774186 ) ) ;
#29678=CARTESIAN_POINT ( 'NONE',  ( 3.310556943749999981, 15.58864905735836182, -32.43493913623279923 ) ) ;
#29680=CARTESIAN_POINT ( 'NONE',  ( 3.310556943750001313, 17.50000000000001776, -80.35160580289945642 ) ) ;
#29681=CARTESIAN_POINT ( 'NONE',  ( -3.310556943750001313, 17.50000000000002487, -135.7641058028994792 ) ) ;
#29685=CARTESIAN_POINT ( 'NONE',  ( -1.750000000000002220, 14.46891108675448478, -100.4880641367107756 ) ) ;
#29687=UNCERTAINTY_MEASURE_WITH_UNIT (LENGTH_MEASURE( 1.000000000000000082E-05 ), #14938, 'distance_accuracy_value', 'NONE');
#29688=CARTESIAN_POINT ( 'NONE',  ( 1.655278471875001101, 20.36702641396249902, -130.1849391362327992 ) ) ;
#29690=CARTESIAN_POINT ( 'NONE',  ( 2.340729813953370519E-16, 21.32270188528331190, -89.01410580289947916 ) ) ;
#29692=CARTESIAN_POINT ( 'NONE',  ( 4.648177544792955347E-16, 21.00000000000001776, -76.21098080242148853 ) ) ;
#29693=CARTESIAN_POINT ( 'NONE',  ( 3.500000000000000000, 15.47927405783633503, -126.5443141357548456 ) ) ;
#29694=CARTESIAN_POINT ( 'NONE',  ( 2.474675557024783212E-16, 21.54145188432739744, -75.90473080337741862 ) ) ;
#29695=CARTESIAN_POINT ( 'NONE',  ( 1.655278471874998436, 14.63297358603754184, -61.51827246956613493 ) ) ;
#29696=( BOUNDED_CURVE ( )  B_SPLINE_CURVE ( 2, ( #26849, #10254, #22599, #10468, #16643, #19409, #35576, #13437, #23221 ),
 .UNSPECIFIED., .F., .F. ) 
 B_SPLINE_CURVE_WITH_KNOTS ( ( 3, 2, 2, 2, 3 ),
 ( 0.2520833333333333259, 0.2527777777777777679, 0.2541666666666666519, 0.2555555555555555358, 0.2562499999999999778 ),
 .UNSPECIFIED. ) 
 CURVE ( )  GEOMETRIC_REPRESENTATION_ITEM ( )  RATIONAL_B_SPLINE_CURVE ( ( 0.9330127018922194093, 0.9330127018922194093, 1.000000000000000000, 0.8660254037844387076, 1.000000000000000000, 0.8660254037844387076, 1.000000000000000000, 0.9330127018922194093, 0.9330127018922194093 ) ) 
 REPRESENTATION_ITEM ( '' )  );
#29700=CARTESIAN_POINT ( 'NONE',  ( -7.022189441860112050E-16, 13.67729811471672363, -81.60160580289947063 ) ) ;
#29701=CARTESIAN_POINT ( 'NONE',  ( -3.500000000000000000, 19.52072594216371115, -77.73806413671076143 ) ) ;
#29703=CARTESIAN_POINT ( 'NONE',  ( 3.310556943749999981, 15.58864905735837247, -110.3474391362328220 ) ) ;
#29704=CARTESIAN_POINT ( 'NONE',  ( 3.310556943750001313, 19.41135094264166483, -83.18077246956613635 ) ) ;
#29706=EDGE_LOOP ( 'NONE', ( #16705, #17125, #40666, #23666 ) ) ;
#29707=CARTESIAN_POINT ( 'NONE',  ( -3.310556943750001313, 17.50000000000001776, -99.85160580289947063 ) ) ;
#29708=CARTESIAN_POINT ( 'NONE',  ( 2.474675557024783212E-16, 21.54145188432740099, -102.9047308033774186 ) ) ;
#29710=CARTESIAN_POINT ( 'NONE',  ( 4.648177544792955347E-16, 21.00000000000001421, -71.21098080242150274 ) ) ;
#29711=CARTESIAN_POINT ( 'NONE',  ( 4.648177544792955347E-16, 21.00000000000001066, -38.21098080242150985 ) ) ;
#29714=CARTESIAN_POINT ( 'NONE',  ( -3.310556943750002201, 15.58864905735836892, -60.68077246956614346 ) ) ;
#29716=CARTESIAN_POINT ( 'NONE',  ( -3.310556943750002645, 15.58864905735837780, -122.6807724695661506 ) ) ;
#29717=CARTESIAN_POINT ( 'NONE',  ( -1.749999999999999778, 20.53108891324555785, -118.1276474690881741 ) ) ;
#29719=VERTEX_POINT ( 'NONE', #5971 ) ;
#29723=DIRECTION ( 'NONE',  ( -0.000000000000000000, 1.259100132267607459E-16, -1.000000000000000000 ) ) ;
#29724=CARTESIAN_POINT ( 'NONE',  ( -3.310556943750000425, 19.41135094264166128, -73.84743913623280775 ) ) ;
#29730=EDGE_CURVE ( 'NONE', #1891, #20433, #2253, .T. ) ;
#29731=CARTESIAN_POINT ( 'NONE',  ( 1.655278471874998436, 14.63297358603755249, -137.4307724695661364 ) ) ;
#29732=DIRECTION ( 'NONE',  ( -0.000000000000000000, 1.259100132267607459E-16, -1.000000000000000000 ) ) ;
#29733=CARTESIAN_POINT ( 'NONE',  ( -3.310556943750002645, 15.58864905735836537, -35.76827246956612782 ) ) ;
#29734=CARTESIAN_POINT ( 'NONE',  ( 3.310556943749999981, 15.58864905735837070, -97.43493913623279923 ) ) ;
#29736=CARTESIAN_POINT ( 'NONE',  ( -3.310556943750000425, 19.41135094264165772, -24.84743913623281841 ) ) ;
#29737=CARTESIAN_POINT ( 'NONE',  ( -0.9378221735089291577, 21.00000000000002132, -112.1663226036829712 ) ) ;
#29738=CARTESIAN_POINT ( 'NONE',  ( -3.500000000000000888, 19.52072594216371115, -102.0443141357548456 ) ) ;
#29741=CARTESIAN_POINT ( 'NONE',  ( -1.750000000000002220, 14.46891108675448301, -90.48806413671076143 ) ) ;
#29742=CARTESIAN_POINT ( 'NONE',  ( 4.648177544792955347E-16, 21.00000000000001776, -78.21098080242148853 ) ) ;
#29744=EDGE_CURVE ( 'NONE', #26790, #41382, #22874, .T. ) ;
#29746=CARTESIAN_POINT ( 'NONE',  ( 3.500000000000001776, 19.52072594216370760, -54.37764746908817415 ) ) ;
#29748=CYLINDRICAL_SURFACE ( 'NONE', #16984, 3.499999999999999556 ) ;
#29749=( BOUNDED_CURVE ( )  B_SPLINE_CURVE ( 2, ( #3667, #19214, #13248, #25603, #41979, #28772, #26019, #23023, #32185 ),
 .UNSPECIFIED., .F., .T. ) 
 B_SPLINE_CURVE_WITH_KNOTS ( ( 3, 2, 2, 2, 3 ),
 ( 0.03541666666666666574, 0.03611111111111110772, 0.03749999999999999861, 0.03888888888888888951, 0.03958333333333333842 ),
 .UNSPECIFIED. ) 
 CURVE ( )  GEOMETRIC_REPRESENTATION_ITEM ( )  RATIONAL_B_SPLINE_CURVE ( ( 0.9330127018922194093, 0.9330127018922194093, 1.000000000000000000, 0.8660254037844387076, 1.000000000000000000, 0.8660254037844387076, 1.000000000000000000, 0.9330127018922189652, 0.9330127018922192983 ) ) 
 REPRESENTATION_ITEM ( '' )  );
#29751=CARTESIAN_POINT ( 'NONE',  ( 1.749999999999998224, 14.46891108675447590, -44.32139747004409713 ) ) ;
#29753=CARTESIAN_POINT ( 'NONE',  ( 2.340729813953370519E-16, 21.32270188528330834, -27.10160580289947063 ) ) ;
#29755=CARTESIAN_POINT ( 'NONE',  ( -3.500000000000002220, 15.47927405783632082, -39.57139747004409713 ) ) ;
#29756=CARTESIAN_POINT ( 'NONE',  ( -0.9378221735089310451, 14.00000000000001599, -56.75563900116002714 ) ) ;
#29758=CARTESIAN_POINT ( 'NONE',  ( 3.500000000000000000, 15.47927405783633326, -120.2380641367107614 ) ) ;
#29760=CARTESIAN_POINT ( 'NONE',  ( -3.310556943750002201, 15.58864905735837070, -75.68077246956613635 ) ) ;
#29761=DIRECTION ( 'NONE',  ( -0.000000000000000000, 1.259100132267607459E-16, -1.000000000000000000 ) ) ;
#29765=CARTESIAN_POINT ( 'NONE',  ( 3.500000000000000000, 15.47927405783632082, -27.23806413671076143 ) ) ;
#29768=CARTESIAN_POINT ( 'NONE',  ( -1.655278471874999990, 20.36702641396249192, -88.93077246956613635 ) ) ;
#29770=VERTEX_POINT ( 'NONE', #11309 ) ;
#29776=ADVANCED_FACE ( 'NONE', ( #14918 ), #4514, .T. ) ;
#29777=CARTESIAN_POINT ( 'NONE',  ( -1.655278471874999990, 20.36702641396249547, -125.9307724695661364 ) ) ;
#29778=ORIENTED_EDGE ( 'NONE', *, *, #386, .T. ) ;
#29779=CARTESIAN_POINT ( 'NONE',  ( -1.750000000000002220, 14.46891108675448301, -94.79431413575484555 ) ) ;
#29780=CARTESIAN_POINT ( 'NONE',  ( 2.340729813953370519E-16, 21.32270188528330834, -56.10160580289946353 ) ) ;
#29781=CARTESIAN_POINT ( 'NONE',  ( 3.310556943750001313, 19.41135094264166838, -121.2682724695661420 ) ) ;
#29782=ORIENTED_EDGE ( 'NONE', *, *, #10436, .F. ) ;
#29784=CARTESIAN_POINT ( 'NONE',  ( 2.474675557024783212E-16, 21.54145188432740099, -125.9047308033774470 ) ) ;
#29785=CARTESIAN_POINT ( 'NONE',  ( -1.655278471875002211, 14.63297358603754184, -41.59743913623280065 ) ) ;
#29786=CARTESIAN_POINT ( 'NONE',  ( 2.340729813953370519E-16, 21.32270188528330834, -72.10160580289947063 ) ) ;
#29787=CARTESIAN_POINT ( 'NONE',  ( -7.424026671074350129E-16, 13.45854811567263987, -116.7109808024215027 ) ) ;
#29788=CARTESIAN_POINT ( 'NONE',  ( -3.310556943750001313, 17.50000000000001776, -101.7641058028994792 ) ) ;
#29792=CARTESIAN_POINT ( 'NONE',  ( -7.424026671074350129E-16, 13.45854811567263454, -71.71098080242151696 ) ) ;
#29794=CARTESIAN_POINT ( 'NONE',  ( 3.310556943750001313, 17.50000000000001066, -36.26410580289947205 ) ) ;
#29795=CARTESIAN_POINT ( 'NONE',  ( 2.340729813953370519E-16, 21.32270188528331190, -94.10160580289948484 ) ) ;
#29796=CARTESIAN_POINT ( 'NONE',  ( 3.500000000000001332, 17.50000000000001421, -59.15473080337743994 ) ) ;
#29798=CARTESIAN_POINT ( 'NONE',  ( 1.655278471875001101, 20.36702641396249547, -114.1849391362327850 ) ) ;
#29799=CARTESIAN_POINT ( 'NONE',  ( 3.310556943750001313, 17.50000000000001066, -45.35160580289947063 ) ) ;
#29801=CARTESIAN_POINT ( 'NONE',  ( 4.648177544792955347E-16, 21.00000000000002132, -127.2109808024214885 ) ) ;
#29806=CARTESIAN_POINT ( 'NONE',  ( 3.310556943750001313, 19.41135094264166838, -93.18077246956613635 ) ) ;
#29807=CARTESIAN_POINT ( 'NONE',  ( 3.500000000000001332, 17.50000000000001066, -23.30785580289947134 ) ) ;
#29810=VERTEX_POINT ( 'NONE', #17496 ) ;
#29814=CARTESIAN_POINT ( 'NONE',  ( 3.500000000000000000, 15.47927405783633503, -123.2380641367107614 ) ) ;
#29815=VERTEX_POINT ( 'NONE', #20684 ) ;
#29817=EDGE_CURVE ( 'NONE', #23461, #745, #22619, .T. ) ;
#29820=CARTESIAN_POINT ( 'NONE',  ( -1.655278471874999990, 20.36702641396248481, -27.93077246956614346 ) ) ;
#29821=ORIENTED_EDGE ( 'NONE', *, *, #8800, .F. ) ;
#29826=ORIENTED_EDGE ( 'NONE', *, *, #31399, .T. ) ;
#29830=CARTESIAN_POINT ( 'NONE',  ( 2.340729813953370519E-16, 21.32270188528332255, -140.0141058028994792 ) ) ;
#29831=CARTESIAN_POINT ( 'NONE',  ( -1.394453263437886604E-15, 14.00000000000001421, -68.71098080242148853 ) ) ;
#29833=CARTESIAN_POINT ( 'NONE',  ( -3.310556943750000425, 19.41135094264167549, -137.9349391362327708 ) ) ;
#29834=CARTESIAN_POINT ( 'NONE',  ( 1.749999999999998224, 14.46891108675447413, -28.62764746908817770 ) ) ;
#29836=CARTESIAN_POINT ( 'NONE',  ( -0.9378221735089310451, 14.00000000000001066, -44.44938900211595012 ) ) ;
#29837=VECTOR ( 'NONE', #23615, 1000.000000000000000 ) ;
#29839=CARTESIAN_POINT ( 'NONE',  ( 3.500000000000000000, 15.47927405783633503, -133.5443141357548598 ) ) ;
#29840=CARTESIAN_POINT ( 'NONE',  ( -1.655278471874999990, 20.36702641396249547, -116.9307724695661364 ) ) ;
#29844=CARTESIAN_POINT ( 'NONE',  ( 3.500000000000001776, 19.52072594216371115, -86.37764746908817415 ) ) ;
#29845=CARTESIAN_POINT ( 'NONE',  ( -0.9378221735089310451, 14.00000000000001599, -69.44938900211597854 ) ) ;
#29846=CARTESIAN_POINT ( 'NONE',  ( -3.310556943750002645, 15.58864905735836714, -52.68077246956613635 ) ) ;
#29848=CARTESIAN_POINT ( 'NONE',  ( -3.310556943750001313, 17.50000000000002132, -113.8516058028994706 ) ) ;
#29849=DIRECTION ( 'NONE',  ( -0.000000000000000000, 1.259100132267607459E-16, -1.000000000000000000 ) ) ;
#29850=CARTESIAN_POINT ( 'NONE',  ( 3.500000000000001332, 17.50000000000001066, -28.15473080337743639 ) ) ;
#29854=CARTESIAN_POINT ( 'NONE',  ( -1.655278471875002211, 14.63297358603755249, -135.6849391362327992 ) ) ;
#29858=CARTESIAN_POINT ( 'NONE',  ( 1.655278471875001101, 20.36702641396248836, -66.18493913623279923 ) ) ;
#29860=CARTESIAN_POINT ( 'NONE',  ( 1.655278471874998436, 14.63297358603754184, -61.43077246956614346 ) ) ;
#29861=ORIENTED_EDGE ( 'NONE', *, *, #5095, .T. ) ;
#29862=CARTESIAN_POINT ( 'NONE',  ( 2.340729813953370519E-16, 21.32270188528331190, -86.10160580289948484 ) ) ;
#29867=CARTESIAN_POINT ( 'NONE',  ( 3.310556943750001313, 19.41135094264166128, -45.18077246956614346 ) ) ;
#29869=CARTESIAN_POINT ( 'NONE',  ( 3.310556943750001313, 17.50000000000001776, -98.26410580289947916 ) ) ;
#29872=EDGE_LOOP ( 'NONE', ( #14672, #28107, #2989, #38205 ) ) ;
#29876=ADVANCED_FACE ( 'NONE', ( #40029 ), #30249, .T. ) ;
#29877=CARTESIAN_POINT ( 'NONE',  ( 1.655278471875001101, 20.36702641396248836, -50.09743913623280775 ) ) ;
#29878=ORIENTED_EDGE ( 'NONE', *, *, #13695, .F. ) ;
#29879=ORIENTED_EDGE ( 'NONE', *, *, #24994, .F. ) ;
#29882=CARTESIAN_POINT ( 'NONE',  ( -3.500000000000002220, 15.47927405783633326, -95.87764746908817415 ) ) ;
#29886=CARTESIAN_POINT ( 'NONE',  ( -7.424026671074350129E-16, 13.45854811567263276, -46.71098080242150274 ) ) ;
#29887=CARTESIAN_POINT ( 'NONE',  ( 2.340729813953370519E-16, 21.32270188528330479, -43.01410580289948626 ) ) ;
#29888=CARTESIAN_POINT ( 'NONE',  ( -1.749999999999999778, 20.53108891324554719, -39.12764746908817415 ) ) ;
#29891=CARTESIAN_POINT ( 'NONE',  ( 3.310556943750001313, 17.50000000000001066, -31.35160580289945997 ) ) ;
#29893=CARTESIAN_POINT ( 'NONE',  ( -3.310556943750000425, 19.41135094264166483, -79.93493913623281344 ) ) ;
#29894=CARTESIAN_POINT ( 'NONE',  ( -1.655278471875002211, 14.63297358603755249, -132.5974391362328220 ) ) ;
#29897=CARTESIAN_POINT ( 'NONE',  ( -0.9378221735089291577, 21.00000000000001776, -75.86007260463890134 ) ) ;
#29899=CARTESIAN_POINT ( 'NONE',  ( 0.9378221735089281585, 14.00000000000001776, -85.66632260368298546 ) ) ;
#29900=CARTESIAN_POINT ( 'NONE',  ( -3.310556943750001313, 17.50000000000002487, -129.8516058028994564 ) ) ;
#29901=CARTESIAN_POINT ( 'NONE',  ( -0.9378221735089291577, 21.00000000000001421, -69.16632260368298546 ) ) ;
#29902=CARTESIAN_POINT ( 'NONE',  ( -1.655278471875002211, 14.63297358603754716, -83.59743913623279354 ) ) ;
#29903=DIRECTION ( 'NONE',  ( 0.000000000000000000, 1.000000000000000000, 0.000000000000000000 ) ) ;
#29904=CARTESIAN_POINT ( 'NONE',  ( 3.500000000000001332, 17.50000000000001776, -75.46098080242151696 ) ) ;
#29906=CARTESIAN_POINT ( 'NONE',  ( 3.500000000000000000, 15.47927405783632437, -75.23806413671076143 ) ) ;
#29907=CARTESIAN_POINT ( 'NONE',  ( -3.310556943750002201, 15.58864905735836892, -60.76827246956613493 ) ) ;
#29910=CARTESIAN_POINT ( 'NONE',  ( -1.749999999999999778, 20.53108891324556140, -129.8213974700441042 ) ) ;
#29911=CARTESIAN_POINT ( 'NONE',  ( 3.310556943750001313, 17.50000000000001776, -78.35160580289945642 ) ) ;
#29912=CARTESIAN_POINT ( 'NONE',  ( 1.655278471874998436, 14.63297358603755249, -138.5182724695661420 ) ) ;
#29914=CARTESIAN_POINT ( 'NONE',  ( 3.310556943750001313, 19.41135094264166838, -109.1807724695661506 ) ) ;
#29915=CARTESIAN_POINT ( 'NONE',  ( 2.340729813953370519E-16, 21.32270188528331190, -81.01410580289947916 ) ) ;
#29917=ORIENTED_EDGE ( 'NONE', *, *, #33165, .F. ) ;
#29918=CARTESIAN_POINT ( 'NONE',  ( 3.310556943750001313, 19.41135094264166838, -103.2682724695661278 ) ) ;
#29919=CARTESIAN_POINT ( 'NONE',  ( 3.500000000000001776, 19.52072594216371826, -102.0713974700440900 ) ) ;
#29922=CARTESIAN_POINT ( 'NONE',  ( 3.500000000000000000, 15.47927405783632793, -88.23806413671076143 ) ) ;
#29924=CARTESIAN_POINT ( 'NONE',  ( 4.648177544792955347E-16, 21.00000000000002132, -119.2109808024215170 ) ) ;
#29925=CARTESIAN_POINT ( 'NONE',  ( 3.310556943749999981, 15.58864905735836537, -62.34743913623280775 ) ) ;
#29926=CARTESIAN_POINT ( 'NONE',  ( 4.648177544792955347E-16, 21.00000000000001421, -68.90473080337741862 ) ) ;
#29927=CARTESIAN_POINT ( 'NONE',  ( -3.310556943750002645, 15.58864905735837780, -118.6807724695661364 ) ) ;
#29928=CARTESIAN_POINT ( 'NONE',  ( 4.648177544792955347E-16, 21.00000000000001421, -67.90473080337741862 ) ) ;
#29930=ORIENTED_EDGE ( 'NONE', *, *, #41054, .T. ) ;
#29935=EDGE_CURVE ( 'NONE', #41828, #26191, #18114, .T. ) ;
#29936=CARTESIAN_POINT ( 'NONE',  ( -3.310556943750002645, 15.58864905735836892, -66.68077246956613635 ) ) ;
#29941=CARTESIAN_POINT ( 'NONE',  ( -3.310556943750000425, 19.41135094264167549, -135.8474391362328220 ) ) ;
#29942=FACE_OUTER_BOUND ( 'NONE', #36799, .T. ) ;
#29943=CARTESIAN_POINT ( 'NONE',  ( -1.655278471874999990, 20.36702641396248836, -47.01827246956613493 ) ) ;
#29944=CARTESIAN_POINT ( 'NONE',  ( -0.9378221735089291577, 21.00000000000002132, -111.1663226036829712 ) ) ;
#29945=CARTESIAN_POINT ( 'NONE',  ( -1.655278471875002211, 14.63297358603754006, -38.68493913623280633 ) ) ;
#29946=CARTESIAN_POINT ( 'NONE',  ( -1.655278471875002211, 14.63297358603754894, -96.68493913623279923 ) ) ;
#29947=( BOUNDED_CURVE ( )  B_SPLINE_CURVE ( 2, ( #37311, #30928, #2198, #21350, #8582, #9857, #36846, #27062, #7064 ),
 .UNSPECIFIED., .F., .T. ) 
 B_SPLINE_CURVE_WITH_KNOTS ( ( 3, 2, 2, 2, 3 ),
 ( 0.5729166666666666297, 0.5736111111111110716, 0.5749999999999999556, 0.5763888888888888395, 0.5770833333333332815 ),
 .UNSPECIFIED. ) 
 CURVE ( )  GEOMETRIC_REPRESENTATION_ITEM ( )  RATIONAL_B_SPLINE_CURVE ( ( 0.9330127018922194093, 0.9330127018922194093, 1.000000000000000000, 0.8660254037844387076, 1.000000000000000000, 0.8660254037844387076, 1.000000000000000000, 0.9330127018922194093, 0.9330127018922194093 ) ) 
 REPRESENTATION_ITEM ( '' )  );
#29949=CARTESIAN_POINT ( 'NONE',  ( -7.022189441860112050E-16, 13.67729811471671475, -26.51410580289947916 ) ) ;
#29951=CARTESIAN_POINT ( 'NONE',  ( 3.500000000000001776, 19.52072594216371115, -99.37764746908815994 ) ) ;
#29954=CARTESIAN_POINT ( 'NONE',  ( 3.500000000000000000, 15.47927405783632615, -93.23806413671076143 ) ) ;
#29958=CARTESIAN_POINT ( 'NONE',  ( -1.750000000000002220, 14.46891108675447946, -55.79431413575483845 ) ) ;
#29960=LINE ( 'NONE', #20826, #3951 ) ;
#29961=CARTESIAN_POINT ( 'NONE',  ( -3.310556943750000425, 19.41135094264165772, -23.84743913623281486 ) ) ;
#29962=ORIENTED_EDGE ( 'NONE', *, *, #21816, .F. ) ;
#29963=CARTESIAN_POINT ( 'NONE',  ( -7.424026671074350129E-16, 13.45854811567263276, -42.40473080337743284 ) ) ;
#29965=CARTESIAN_POINT ( 'NONE',  ( -3.310556943750001313, 17.50000000000001066, -24.85160580289946708 ) ) ;
#29967=CARTESIAN_POINT ( 'NONE',  ( -3.500000000000002220, 15.47927405783632970, -90.57139747004410424 ) ) ;
#29969=CARTESIAN_POINT ( 'NONE',  ( -1.750000000000002220, 14.46891108675447590, -33.48806413671076854 ) ) ;
#29971=CARTESIAN_POINT ( 'NONE',  ( -1.655278471875002211, 14.63297358603754539, -78.59743913623280775 ) ) ;
#29972=CARTESIAN_POINT ( 'NONE',  ( 3.500000000000000000, 15.47927405783632082, -52.54431413575484555 ) ) ;
#29973=VERTEX_POINT ( 'NONE', #1121 ) ;
#29975=AXIS2_PLACEMENT_3D ( 'NONE', #32764, #13009, #25988 ) ;
#29978=CARTESIAN_POINT ( 'NONE',  ( -1.750000000000002220, 14.46891108675448301, -87.79431413575483134 ) ) ;
#29979=CARTESIAN_POINT ( 'NONE',  ( 1.655278471874998436, 14.63297358603754539, -87.43077246956613635 ) ) ;
#29980=ORIENTED_EDGE ( 'NONE', *, *, #5079, .F. ) ;
#29986=EDGE_CURVE ( 'NONE', #8219, #18739, #6600, .T. ) ;
#29987=CARTESIAN_POINT ( 'NONE',  ( 2.340729813953370519E-16, 21.32270188528331900, -127.0141058028994507 ) ) ;
#29990=CARTESIAN_POINT ( 'NONE',  ( 2.340729813953370519E-16, 21.32270188528330834, -52.10160580289946353 ) ) ;
#29991=CARTESIAN_POINT ( 'NONE',  ( -3.310556943750002645, 15.58864905735837780, -113.7682724695661278 ) ) ;
#29994=CARTESIAN_POINT ( 'NONE',  ( -1.749999999999999778, 20.53108891324555785, -125.8213974700440900 ) ) ;
#29995=( BOUNDED_CURVE ( )  B_SPLINE_CURVE ( 2, ( #39503, #35894, #19731, #32701, #39721, #10377, #10592, #23133, #23573 ),
 .UNSPECIFIED., .F., .T. ) 
 B_SPLINE_CURVE_WITH_KNOTS ( ( 3, 2, 2, 2, 3 ),
 ( 0.4437499999999999778, 0.4444444444444444198, 0.4458333333333333592, 0.4472222222222222432, 0.4479166666666666852 ),
 .UNSPECIFIED. ) 
 CURVE ( )  GEOMETRIC_REPRESENTATION_ITEM ( )  RATIONAL_B_SPLINE_CURVE ( ( 0.9330127018922194093, 0.9330127018922194093, 1.000000000000000000, 0.8660254037844387076, 1.000000000000000000, 0.8660254037844387076, 1.000000000000000000, 0.9330127018922194093, 0.9330127018922194093 ) ) 
 REPRESENTATION_ITEM ( '' )  );
#29996=AXIS2_PLACEMENT_3D ( 'NONE', #10136, #32670, #16730 ) ;
#29997=CARTESIAN_POINT ( 'NONE',  ( -3.310556943750002645, 15.58864905735836537, -39.68077246956613635 ) ) ;
#29998=CARTESIAN_POINT ( 'NONE',  ( 3.310556943750001313, 19.41135094264166128, -70.26827246956612782 ) ) ;
#29999=CARTESIAN_POINT ( 'NONE',  ( 3.500000000000001776, 19.52072594216371826, -115.3776474690881884 ) ) ;
#30000=CARTESIAN_POINT ( 'NONE',  ( 1.655278471875001101, 20.36702641396249547, -104.0974391362328220 ) ) ;
#30001=DIRECTION ( 'NONE',  ( 0.000000000000000000, 1.000000000000000000, 0.000000000000000000 ) ) ;
#30004=CARTESIAN_POINT ( 'NONE',  ( 3.500000000000001776, 19.52072594216370760, -68.37764746908817415 ) ) ;
#30005=CARTESIAN_POINT ( 'NONE',  ( 1.750000000000001110, 20.53108891324555785, -122.2943141357548456 ) ) ;
#30006=CARTESIAN_POINT ( 'NONE',  ( 3.310556943750001313, 19.41135094264165772, -37.18077246956613635 ) ) ;
#30007=CARTESIAN_POINT ( 'NONE',  ( -7.022189441860112050E-16, 13.67729811471672541, -98.60160580289947063 ) ) ;
#30008=CARTESIAN_POINT ( 'NONE',  ( -1.749999999999999778, 20.53108891324555074, -58.82139747004409713 ) ) ;
#30009=CARTESIAN_POINT ( 'NONE',  ( 0.9378221735089300459, 21.00000000000001066, -39.25563900116003424 ) ) ;
#30010=CARTESIAN_POINT ( 'NONE',  ( -3.310556943750000425, 19.41135094264166838, -112.9349391362327992 ) ) ;
#30011=CARTESIAN_POINT ( 'NONE',  ( 3.310556943750001313, 17.50000000000001066, -41.35160580289947063 ) ) ;
#30018=EDGE_CURVE ( 'NONE', #29090, #28655, #34299, .T. ) ;
#30019=CARTESIAN_POINT ( 'NONE',  ( 3.310556943749999981, 15.58864905735836892, -91.34743913623280775 ) ) ;
#30020=CARTESIAN_POINT ( 'NONE',  ( -0.9378221735089310451, 14.00000000000001066, -36.44938900211595723 ) ) ;
#30024=DIRECTION ( 'NONE',  ( 0.000000000000000000, 1.000000000000000000, 0.000000000000000000 ) ) ;
#30027=LINE ( 'NONE', #33213, #9418 ) ;
#30028=ORIENTED_EDGE ( 'NONE', *, *, #39420, .F. ) ;
#30032=CARTESIAN_POINT ( 'NONE',  ( 1.655278471875001101, 20.36702641396248481, -30.09743913623280775 ) ) ;
#30033=ORIENTED_EDGE ( 'NONE', *, *, #25806, .F. ) ;
#30034=CARTESIAN_POINT ( 'NONE',  ( 4.648177544792955347E-16, 21.00000000000001066, -38.90473080337743284 ) ) ;
#30038=VERTEX_POINT ( 'NONE', #2779 ) ;
#30039=LINE ( 'NONE', #10693, #39605 ) ;
#30041=ADVANCED_FACE ( 'NONE', ( #22549 ), #15981, .T. ) ;
#30042=CARTESIAN_POINT ( 'NONE',  ( 3.310556943750001313, 19.41135094264167549, -143.1807724695661364 ) ) ;
#30044=CARTESIAN_POINT ( 'NONE',  ( 3.310556943750001313, 19.41135094264167549, -131.2682724695661136 ) ) ;
#30045=CARTESIAN_POINT ( 'NONE',  ( 2.474675557024783212E-16, 21.54145188432739033, -28.21098080242151340 ) ) ;
#30046=VERTEX_POINT ( 'NONE', #18943 ) ;
#30049=CARTESIAN_POINT ( 'NONE',  ( -7.424026671074350129E-16, 13.45854811567264164, -140.4047308033774186 ) ) ;
#30051=CARTESIAN_POINT ( 'NONE',  ( -7.424026671074350129E-16, 13.45854811567264164, -135.7109808024214885 ) ) ;
#30052=CARTESIAN_POINT ( 'NONE',  ( 3.310556943749999981, 15.58864905735837247, -119.3474391362327935 ) ) ;
#30055=CARTESIAN_POINT ( 'NONE',  ( -1.750000000000002220, 14.46891108675448301, -83.79431413575483134 ) ) ;
#30056=CARTESIAN_POINT ( 'NONE',  ( -0.9378221735089291577, 21.00000000000001776, -92.86007260463891555 ) ) ;
#30057=CARTESIAN_POINT ( 'NONE',  ( -3.310556943750001313, 17.50000000000001421, -53.76410580289947916 ) ) ;
#30058=CARTESIAN_POINT ( 'NONE',  ( -3.310556943750000425, 19.41135094264166838, -113.9349391362327850 ) ) ;
#30059=CARTESIAN_POINT ( 'NONE',  ( -3.500000000000000000, 19.52072594216371115, -94.04431413575484555 ) ) ;
#30060=CARTESIAN_POINT ( 'NONE',  ( -3.500000000000001332, 17.50000000000001066, -28.65473080337743639 ) ) ;
#30061=CARTESIAN_POINT ( 'NONE',  ( 3.500000000000000000, 15.47927405783633326, -116.5443141357548313 ) ) ;
#30063=CARTESIAN_POINT ( 'NONE',  ( 3.310556943750001313, 17.50000000000002132, -126.3516058028994706 ) ) ;
#30066=CARTESIAN_POINT ( 'NONE',  ( 0.000000000000000000, 21.00000000000002487, -149.5231586289125687 ) ) ;
#30068=CARTESIAN_POINT ( 'NONE',  ( 1.655278471875001101, 20.36702641396248836, -65.18493913623279923 ) ) ;
#30070=ORIENTED_EDGE ( 'NONE', *, *, #30018, .T. ) ;
#30071=CARTESIAN_POINT ( 'NONE',  ( -3.310556943750002201, 15.58864905735837247, -82.76827246956615625 ) ) ;
#30072=ADVANCED_FACE ( 'NONE', ( #25754 ), #5553, .T. ) ;
#30074=CARTESIAN_POINT ( 'NONE',  ( -1.394453263437886604E-15, 14.00000000000001066, -52.40473080337743284 ) ) ;
#30079=CARTESIAN_POINT ( 'NONE',  ( 3.310556943750001313, 17.50000000000001421, -47.26410580289947205 ) ) ;
#30082=CARTESIAN_POINT ( 'NONE',  ( -3.310556943750000425, 19.41135094264166483, -98.84743913623280775 ) ) ;
#30083=CARTESIAN_POINT ( 'NONE',  ( 3.500000000000001332, 17.50000000000001066, -42.15473080337743284 ) ) ;
#30088=CARTESIAN_POINT ( 'NONE',  ( -1.655278471874999990, 20.36702641396248836, -51.93077246956613635 ) ) ;
#30090=VERTEX_POINT ( 'NONE', #2145 ) ;
#30093=ORIENTED_EDGE ( 'NONE', *, *, #39865, .F. ) ;
#30094=CARTESIAN_POINT ( 'NONE',  ( 1.750000000000001110, 20.53108891324554719, -44.29431413575483845 ) ) ;
#30095=FACE_OUTER_BOUND ( 'NONE', #1290, .T. ) ;
#30096=DIRECTION ( 'NONE',  ( -0.000000000000000000, 1.259100132267607459E-16, -1.000000000000000000 ) ) ;
#30099=CARTESIAN_POINT ( 'NONE',  ( 1.655278471874998436, 14.63297358603753828, -31.51827246956613493 ) ) ;
#30100=ADVANCED_FACE ( 'NONE', ( #31285 ), #9159, .T. ) ;
#30101=CARTESIAN_POINT ( 'NONE',  ( -1.394453263437886604E-15, 14.00000000000001066, -51.40473080337743284 ) ) ;
#30103=CARTESIAN_POINT ( 'NONE',  ( -3.310556943750000425, 19.41135094264166483, -81.93493913623278502 ) ) ;
#30104=CARTESIAN_POINT ( 'NONE',  ( -1.655278471875002211, 14.63297358603755249, -134.5974391362328220 ) ) ;
#30108=CARTESIAN_POINT ( 'NONE',  ( -1.394453263437886604E-15, 14.00000000000001776, -103.4047308033774186 ) ) ;
#30109=CARTESIAN_POINT ( 'NONE',  ( 3.369928719974892676E-15, 14.00000000000002309, -140.4047308033774186 ) ) ;
#30110=CARTESIAN_POINT ( 'NONE',  ( -7.022189441860112050E-16, 13.67729811471672718, -125.6016058028994706 ) ) ;
#30111=CYLINDRICAL_SURFACE ( 'NONE', #37021, 3.499999999999999556 ) ;
#30112=CARTESIAN_POINT ( 'NONE',  ( 1.655278471874998436, 14.63297358603754539, -87.43077246956613635 ) ) ;
#30113=CARTESIAN_POINT ( 'NONE',  ( -1.394453263437886604E-15, 14.00000000000001421, -68.71098080242148853 ) ) ;
#30114=DIRECTION ( 'NONE',  ( 0.000000000000000000, -1.259100132267607459E-16, 1.000000000000000000 ) ) ;
#30115=CARTESIAN_POINT ( 'NONE',  ( 1.749999999999998224, 14.46891108675447768, -67.32139747004409003 ) ) ;
#30116=CARTESIAN_POINT ( 'NONE',  ( -3.500000000000002220, 15.47927405783632615, -74.57139747004410424 ) ) ;
#30117=EDGE_CURVE ( 'NONE', #10678, #18307, #15762, .T. ) ;
#30118=CARTESIAN_POINT ( 'NONE',  ( -7.022189441860112050E-16, 13.67729811471671830, -52.60160580289946353 ) ) ;
#30120=CARTESIAN_POINT ( 'NONE',  ( 1.750000000000001110, 20.53108891324556140, -137.2943141357548598 ) ) ;
#30122=CARTESIAN_POINT ( 'NONE',  ( 3.310556943750001313, 19.41135094264166483, -82.26827246956614204 ) ) ;
#30123=CARTESIAN_POINT ( 'NONE',  ( -3.310556943750000425, 19.41135094264167549, -138.9349391362327708 ) ) ;
#30125=CARTESIAN_POINT ( 'NONE',  ( 1.655278471875001101, 20.36702641396249547, -110.0974391362328078 ) ) ;
#30126=CARTESIAN_POINT ( 'NONE',  ( 2.340729813953370519E-16, 21.32270188528331190, -76.01410580289947916 ) ) ;
#30127=ORIENTED_EDGE ( 'NONE', *, *, #20466, .F. ) ;
#30128=CARTESIAN_POINT ( 'NONE',  ( 1.655278471875001101, 20.36702641396249192, -101.1849391362327992 ) ) ;
#30129=CARTESIAN_POINT ( 'NONE',  ( 3.500000000000001332, 17.50000000000002132, -105.1547308033774186 ) ) ;
#30130=( BOUNDED_CURVE ( )  B_SPLINE_CURVE ( 2, ( #9661, #22623, #32198, #15840, #35173, #35386, #490, #2850, #19226 ),
 .UNSPECIFIED., .F., .T. ) 
 B_SPLINE_CURVE_WITH_KNOTS ( ( 3, 2, 2, 2, 3 ),
 ( 0.3062500000000000222, 0.3069444444444444642, 0.3083333333333333481, 0.3097222222222222321, 0.3104166666666666741 ),
 .UNSPECIFIED. ) 
 CURVE ( )  GEOMETRIC_REPRESENTATION_ITEM ( )  RATIONAL_B_SPLINE_CURVE ( ( 0.9330127018922194093, 0.9330127018922194093, 1.000000000000000000, 0.8660254037844387076, 1.000000000000000000, 0.8660254037844387076, 1.000000000000000000, 0.9330127018922194093, 0.9330127018922194093 ) ) 
 REPRESENTATION_ITEM ( '' )  );
#30133=CARTESIAN_POINT ( 'NONE',  ( -3.500000000000001332, 17.50000000000001776, -95.65473080337743284 ) ) ;
#30135=CARTESIAN_POINT ( 'NONE',  ( 1.655278471875001101, 20.36702641396248836, -63.09743913623280775 ) ) ;
#30137=CARTESIAN_POINT ( 'NONE',  ( -1.655278471875002211, 14.63297358603755072, -118.5974391362328078 ) ) ;
#30138=CARTESIAN_POINT ( 'NONE',  ( 3.602337597214540226E-14, 14.00000000000002132, -117.7109808024215027 ) ) ;
#30145=CARTESIAN_POINT ( 'NONE',  ( -7.022189441860112050E-16, 13.67729811471672186, -68.51410580289947916 ) ) ;
#30148=DIRECTION ( 'NONE',  ( -0.000000000000000000, 1.259100132267607459E-16, -1.000000000000000000 ) ) ;
#30154=ORIENTED_EDGE ( 'NONE', *, *, #30679, .F. ) ;
#30155=CARTESIAN_POINT ( 'NONE',  ( -1.655278471874999990, 20.36702641396249902, -133.9307724695661364 ) ) ;
#30156=CARTESIAN_POINT ( 'NONE',  ( -3.500000000000002220, 15.47927405783633503, -131.5713974700441042 ) ) ;
#30157=CARTESIAN_POINT ( 'NONE',  ( -3.310556943750000425, 19.41135094264165772, -42.93493913623279923 ) ) ;
#30158=CARTESIAN_POINT ( 'NONE',  ( 7.367361408496833051E-14, 14.00000000000002132, -110.7109808024214743 ) ) ;
#30159=CARTESIAN_POINT ( 'NONE',  ( 3.310556943750001313, 17.50000000000001066, -39.35160580289946353 ) ) ;
#30160=CARTESIAN_POINT ( 'NONE',  ( -1.655278471874999990, 20.36702641396249192, -100.0182724695661278 ) ) ;
#30162=CARTESIAN_POINT ( 'NONE',  ( 3.310556943750001313, 19.41135094264167549, -143.2682724695661420 ) ) ;
#30163=AXIS2_PLACEMENT_3D ( 'NONE', #29122, #32330, #6383 ) ;
#30164=LINE ( 'NONE', #21015, #24394 ) ;
#30165=CARTESIAN_POINT ( 'NONE',  ( 1.750000000000001110, 20.53108891324555785, -102.2943141357548456 ) ) ;
#30166=CARTESIAN_POINT ( 'NONE',  ( 3.500000000000001332, 17.50000000000001776, -100.1547308033774328 ) ) ;
#30168=CARTESIAN_POINT ( 'NONE',  ( -3.500000000000002220, 15.47927405783632793, -89.57139747004409003 ) ) ;
#30174=FACE_OUTER_BOUND ( 'NONE', #1276, .T. ) ;
#30175=CARTESIAN_POINT ( 'NONE',  ( -3.500000000000002220, 15.47927405783632260, -53.87764746908817415 ) ) ;
#30178=CARTESIAN_POINT ( 'NONE',  ( 3.500000000000001332, 17.50000000000002132, -103.4609808024215027 ) ) ;
#30180=CARTESIAN_POINT ( 'NONE',  ( -1.749999999999999778, 20.53108891324554719, -41.82139747004409713 ) ) ;
#30182=AXIS2_PLACEMENT_3D ( 'NONE', #20088, #36032, #42023 ) ;
#30183=CARTESIAN_POINT ( 'NONE',  ( 1.655278471875001101, 20.36702641396248481, -28.18493913623279568 ) ) ;
#30184=CARTESIAN_POINT ( 'NONE',  ( -1.750000000000002220, 14.46891108675448123, -80.48806413671076143 ) ) ;
#30187=DIRECTION ( 'NONE',  ( 0.000000000000000000, 1.000000000000000000, 0.000000000000000000 ) ) ;
#30188=CARTESIAN_POINT ( 'NONE',  ( -3.310556943750001313, 17.50000000000001776, -77.76410580289946495 ) ) ;
#30190=ORIENTED_EDGE ( 'NONE', *, *, #27300, .F. ) ;
#30191=CARTESIAN_POINT ( 'NONE',  ( 4.648177544792955347E-16, 21.00000000000001776, -98.21098080242148853 ) ) ;
#30192=CARTESIAN_POINT ( 'NONE',  ( -3.500000000000000000, 19.52072594216370405, -45.04431413575484555 ) ) ;
#30193=VERTEX_POINT ( 'NONE', #5337 ) ;
#30194=LINE ( 'NONE', #24042, #27329 ) ;
#30195=CARTESIAN_POINT ( 'NONE',  ( -7.022189441860112050E-16, 13.67729811471672363, -82.51410580289946495 ) ) ;
#30197=EDGE_LOOP ( 'NONE', ( #15980, #36039, #2627, #17166 ) ) ;
#30199=( BOUNDED_CURVE ( )  B_SPLINE_CURVE ( 2, ( #37872, #24913, #11502, #5756, #2563, #12341, #25328, #38286, #1734 ),
 .UNSPECIFIED., .F., .T. ) 
 B_SPLINE_CURVE_WITH_KNOTS ( ( 3, 2, 2, 2, 3 ),
 ( 0.2812500000000000000, 0.2819444444444444420, 0.2833333333333333259, 0.2847222222222222099, 0.2854166666666666519 ),
 .UNSPECIFIED. ) 
 CURVE ( )  GEOMETRIC_REPRESENTATION_ITEM ( )  RATIONAL_B_SPLINE_CURVE ( ( 0.9330127018922194093, 0.9330127018922194093, 1.000000000000000000, 0.8660254037844387076, 1.000000000000000000, 0.8660254037844387076, 1.000000000000000000, 0.9330127018922194093, 0.9330127018922194093 ) ) 
 REPRESENTATION_ITEM ( '' )  );
#30201=LINE ( 'NONE', #17023, #7682 ) ;
#30202=CARTESIAN_POINT ( 'NONE',  ( -3.310556943750002645, 15.58864905735837780, -127.6807724695661364 ) ) ;
#30203=VECTOR ( 'NONE', #10696, 1000.000000000000000 ) ;
#30206=CARTESIAN_POINT ( 'NONE',  ( -3.310556943750000425, 19.41135094264166128, -53.93493913623280633 ) ) ;
#30207=CARTESIAN_POINT ( 'NONE',  ( -3.310556943750002645, 15.58864905735837780, -115.7682724695661278 ) ) ;
#30210=CARTESIAN_POINT ( 'NONE',  ( 3.500000000000001776, 19.52072594216371826, -126.0713974700440900 ) ) ;
#30211=CARTESIAN_POINT ( 'NONE',  ( 2.340729813953370519E-16, 21.32270188528330479, -41.01410580289947916 ) ) ;
#30212=CARTESIAN_POINT ( 'NONE',  ( -1.655278471875002211, 14.63297358603754361, -66.68493913623279923 ) ) ;
#30213=CARTESIAN_POINT ( 'NONE',  ( -3.500000000000001332, 17.50000000000002132, -116.9609808024215170 ) ) ;
#30214=CARTESIAN_POINT ( 'NONE',  ( -3.310556943750002645, 15.58864905735837425, -102.6807724695661364 ) ) ;
#30216=CARTESIAN_POINT ( 'NONE',  ( 0.000000000000000000, 21.00000000000002487, -149.5231586289125687 ) ) ;
#30217=DIRECTION ( 'NONE',  ( -0.000000000000000000, 1.259100132267607459E-16, -1.000000000000000000 ) ) ;
#30219=CARTESIAN_POINT ( 'NONE',  ( 3.500000000000001332, 17.50000000000001421, -69.46098080242150274 ) ) ;
#30220=DIRECTION ( 'NONE',  ( -0.000000000000000000, 1.259100132267607459E-16, -1.000000000000000000 ) ) ;
#30221=CARTESIAN_POINT ( 'NONE',  ( -3.310556943750000425, 19.41135094264165772, -34.84743913623281486 ) ) ;
#30222=CARTESIAN_POINT ( 'NONE',  ( 1.655278471874998436, 14.63297358603754539, -90.51827246956612782 ) ) ;
#30224=CARTESIAN_POINT ( 'NONE',  ( -3.500000000000002220, 15.47927405783632437, -59.57139747004409713 ) ) ;
#30225=CARTESIAN_POINT ( 'NONE',  ( 0.000000000000000000, 17.50000000000002487, -149.5231586289125687 ) ) ;
#30226=CARTESIAN_POINT ( 'NONE',  ( -1.655278471874999990, 20.36702641396249547, -111.0182724695661420 ) ) ;
#30227=CARTESIAN_POINT ( 'NONE',  ( -3.310556943750002201, 15.58864905735836714, -44.76827246956613493 ) ) ;
#30234=CARTESIAN_POINT ( 'NONE',  ( -1.655278471874999990, 20.36702641396249192, -94.93077246956613635 ) ) ;
#30235=CARTESIAN_POINT ( 'NONE',  ( 4.648177544792955347E-16, 21.00000000000001421, -62.21098080242150274 ) ) ;
#30237=ORIENTED_EDGE ( 'NONE', *, *, #37903, .T. ) ;
#30240=EDGE_CURVE ( 'NONE', #27884, #29719, #15354, .T. ) ;
#30243=CARTESIAN_POINT ( 'NONE',  ( 1.750000000000001110, 20.53108891324554719, -46.29431413575483845 ) ) ;
#30244=EDGE_LOOP ( 'NONE', ( #23512, #30873, #17545, #41920 ) ) ;
#30247=CARTESIAN_POINT ( 'NONE',  ( 3.310556943750001313, 17.50000000000001066, -29.26410580289948271 ) ) ;
#30249=CYLINDRICAL_SURFACE ( 'NONE', #6854, 3.499999999999999556 ) ;
#30253=ORIENTED_EDGE ( 'NONE', *, *, #11524, .T. ) ;
#30255=( BOUNDED_CURVE ( )  B_SPLINE_CURVE ( 2, ( #40390, #23815, #30393, #17435, #34210, #14446, #21032, #11448, #11046 ),
 .UNSPECIFIED., .F., .T. ) 
 B_SPLINE_CURVE_WITH_KNOTS ( ( 3, 2, 2, 2, 3 ),
 ( 0.7312499999999999556, 0.7319444444444443976, 0.7333333333333332815, 0.7347222222222222765, 0.7354166666666667185 ),
 .UNSPECIFIED. ) 
 CURVE ( )  GEOMETRIC_REPRESENTATION_ITEM ( )  RATIONAL_B_SPLINE_CURVE ( ( 0.9330127018922194093, 0.9330127018922194093, 1.000000000000000000, 0.8660254037844387076, 1.000000000000000000, 0.8660254037844387076, 1.000000000000000000, 0.9330127018922194093, 0.9330127018922194093 ) ) 
 REPRESENTATION_ITEM ( '' )  );
#30257=CARTESIAN_POINT ( 'NONE',  ( 1.655278471875001101, 20.36702641396249902, -141.0974391362327935 ) ) ;
#30259=LINE ( 'NONE', #35998, #15948 ) ;
#30260=CARTESIAN_POINT ( 'NONE',  ( 1.655278471874998436, 14.63297358603755072, -128.5182724695661136 ) ) ;
#30261=CARTESIAN_POINT ( 'NONE',  ( -7.424026671074350129E-16, 13.45854811567263098, -28.71098080242151340 ) ) ;
#30264=CARTESIAN_POINT ( 'NONE',  ( -7.424026671074350129E-16, 13.45854811567264164, -142.4047308033774186 ) ) ;
#30267=CARTESIAN_POINT ( 'NONE',  ( 2.474675557024783212E-16, 21.54145188432740810, -131.2109808024214885 ) ) ;
#30268=CARTESIAN_POINT ( 'NONE',  ( -1.655278471874999990, 20.36702641396249547, -118.9307724695661364 ) ) ;
#30271=CARTESIAN_POINT ( 'NONE',  ( -1.750000000000002220, 14.46891108675448301, -86.79431413575483134 ) ) ;
#30272=CARTESIAN_POINT ( 'NONE',  ( -3.500000000000000000, 19.52072594216370760, -69.73806413671077564 ) ) ;
#30273=CARTESIAN_POINT ( 'NONE',  ( -3.310556943750002645, 15.58864905735836892, -55.68077246956614346 ) ) ;
#30274=CARTESIAN_POINT ( 'NONE',  ( -1.655278471875002211, 14.63297358603755072, -110.6849391362327992 ) ) ;
#30278=CARTESIAN_POINT ( 'NONE',  ( -7.022189441860112050E-16, 13.67729811471672896, -126.6016058028994564 ) ) ;
#30281=FACE_OUTER_BOUND ( 'NONE', #19210, .T. ) ;
#30282=DIRECTION ( 'NONE',  ( 0.000000000000000000, 1.000000000000000000, 0.000000000000000000 ) ) ;
#30283=CARTESIAN_POINT ( 'NONE',  ( 3.310556943750001313, 17.50000000000001421, -66.35160580289945642 ) ) ;
#30285=ORIENTED_EDGE ( 'NONE', *, *, #32747, .T. ) ;
#30286=CARTESIAN_POINT ( 'NONE',  ( 2.340729813953370519E-16, 21.32270188528331190, -82.10160580289945642 ) ) ;
#30287=ADVANCED_FACE ( 'NONE', ( #25968 ), #38930, .T. ) ;
#30292=CARTESIAN_POINT ( 'NONE',  ( -3.310556943750002201, 15.58864905735836714, -45.68077246956614346 ) ) ;
#30293=CARTESIAN_POINT ( 'NONE',  ( 4.648177544792955347E-16, 21.00000000000001066, -28.21098080242150985 ) ) ;
#30294=ORIENTED_EDGE ( 'NONE', *, *, #24762, .F. ) ;
#30297=ORIENTED_EDGE ( 'NONE', *, *, #19032, .T. ) ;
#30299=CARTESIAN_POINT ( 'NONE',  ( 1.655278471874998436, 14.63297358603754006, -51.43077246956613635 ) ) ;
#30301=ORIENTED_EDGE ( 'NONE', *, *, #34349, .T. ) ;
#30302=CARTESIAN_POINT ( 'NONE',  ( 0.000000000000000000, 17.50000000000002487, -149.5231586289125687 ) ) ;
#30303=CARTESIAN_POINT ( 'NONE',  ( -1.749999999999999778, 20.53108891324555429, -91.82139747004409003 ) ) ;
#30305=CARTESIAN_POINT ( 'NONE',  ( -1.394453263437886604E-15, 14.00000000000002132, -113.7109808024214743 ) ) ;
#30306=ORIENTED_EDGE ( 'NONE', *, *, #36552, .T. ) ;
#30307=CARTESIAN_POINT ( 'NONE',  ( 1.749999999999998224, 14.46891108675447590, -44.62764746908817415 ) ) ;
#30308=EDGE_CURVE ( 'NONE', #20737, #29719, #26731, .T. ) ;
#30311=CARTESIAN_POINT ( 'NONE',  ( -1.749999999999999778, 20.53108891324555785, -110.8213974700441042 ) ) ;
#30314=CARTESIAN_POINT ( 'NONE',  ( -1.655278471874999990, 20.36702641396248481, -27.01827246956613138 ) ) ;
#30315=CARTESIAN_POINT ( 'NONE',  ( -3.310556943750002645, 15.58864905735836182, -23.76827246956612782 ) ) ;
#30316=CARTESIAN_POINT ( 'NONE',  ( -1.655278471875002211, 14.63297358603754539, -80.68493913623279923 ) ) ;
#30317=CARTESIAN_POINT ( 'NONE',  ( 2.340729813953370519E-16, 21.32270188528332255, -134.0141058028994792 ) ) ;
#30321=CARTESIAN_POINT ( 'NONE',  ( -1.394453263437886604E-15, 14.00000000000001776, -85.71098080242151696 ) ) ;
#30322=CARTESIAN_POINT ( 'NONE',  ( 3.310556943750001313, 19.41135094264166838, -128.2682724695661136 ) ) ;
#30323=CARTESIAN_POINT ( 'NONE',  ( 3.500000000000000000, 15.47927405783632082, -42.54431413575483845 ) ) ;
#30324=CARTESIAN_POINT ( 'NONE',  ( 3.310556943749999981, 15.58864905735836892, -87.34743913623280775 ) ) ;
#30325=CARTESIAN_POINT ( 'NONE',  ( 1.749999999999998224, 14.46891108675447235, -24.62764746908817415 ) ) ;
#30328=CARTESIAN_POINT ( 'NONE',  ( 1.750000000000001110, 20.53108891324555074, -71.98806413671076143 ) ) ;
#30329=CARTESIAN_POINT ( 'NONE',  ( 3.310556943750001313, 17.50000000000001421, -51.35160580289946353 ) ) ;
#30332=CARTESIAN_POINT ( 'NONE',  ( -1.655278471874999990, 20.36702641396249192, -79.01827246956614204 ) ) ;
#30333=CARTESIAN_POINT ( 'NONE',  ( -3.310556943750002645, 15.58864905735837958, -140.7682724695661136 ) ) ;
#30335=CARTESIAN_POINT ( 'NONE',  ( -3.310556943750000425, 19.41135094264166838, -106.8474391362328078 ) ) ;
#30336=CARTESIAN_POINT ( 'NONE',  ( 3.310556943750001313, 17.50000000000001776, -75.26410580289947916 ) ) ;
#30338=ORIENTED_EDGE ( 'NONE', *, *, #2010, .F. ) ;
#30339=CARTESIAN_POINT ( 'NONE',  ( 3.310556943750001313, 19.41135094264166838, -94.26827246956612782 ) ) ;
#30340=CARTESIAN_POINT ( 'NONE',  ( -1.749999999999999778, 20.53108891324555429, -99.82139747004409003 ) ) ;
#30342=CARTESIAN_POINT ( 'NONE',  ( -3.500000000000001332, 17.50000000000001776, -86.65473080337743284 ) ) ;
#30343=CARTESIAN_POINT ( 'NONE',  ( 3.500000000000001332, 19.52072594216370760, -51.07139747004409003 ) ) ;
#30345=CARTESIAN_POINT ( 'NONE',  ( 1.655278471874998436, 14.63297358603754184, -59.43077246956614346 ) ) ;
#30346=CARTESIAN_POINT ( 'NONE',  ( -1.749999999999999778, 20.53108891324555785, -113.1276474690881741 ) ) ;
#30347=CARTESIAN_POINT ( 'NONE',  ( -7.022189441860112050E-16, 13.67729811471672718, -118.5141058028994792 ) ) ;
#30348=CARTESIAN_POINT ( 'NONE',  ( -3.500000000000002220, 15.47927405783633503, -117.8776474690881741 ) ) ;
#30349=EDGE_CURVE ( 'NONE', #10255, #40976, #10950, .T. ) ;
#30351=ORIENTED_EDGE ( 'NONE', *, *, #5608, .F. ) ;
#30356=CARTESIAN_POINT ( 'NONE',  ( 0.000000000000000000, 21.00000000000002487, -149.5231586289125687 ) ) ;
#30357=CARTESIAN_POINT ( 'NONE',  ( 3.310556943749999981, 15.58864905735836537, -66.34743913623280775 ) ) ;
#30358=ORIENTED_EDGE ( 'NONE', *, *, #18687, .T. ) ;
#30361=CARTESIAN_POINT ( 'NONE',  ( -1.394453263437886604E-15, 14.00000000000001776, -83.71098080242150274 ) ) ;
#30365=ORIENTED_EDGE ( 'NONE', *, *, #20226, .T. ) ;
#30366=DIRECTION ( 'NONE',  ( -0.000000000000000000, 1.259100132267607459E-16, -1.000000000000000000 ) ) ;
#30367=CARTESIAN_POINT ( 'NONE',  ( -1.655278471875002211, 14.63297358603755427, -137.5974391362328220 ) ) ;
#30370=CARTESIAN_POINT ( 'NONE',  ( 3.310556943749999981, 15.58864905735836182, -43.43493913623279212 ) ) ;
#30372=CARTESIAN_POINT ( 'NONE',  ( 3.310556943750001313, 17.50000000000001066, -40.35160580289947063 ) ) ;
#30373=CARTESIAN_POINT ( 'NONE',  ( -3.310556943750000425, 19.41135094264166483, -96.93493913623281344 ) ) ;
#30376=CARTESIAN_POINT ( 'NONE',  ( -1.655278471874999990, 20.36702641396248481, -23.93077246956613990 ) ) ;
#30377=DIRECTION ( 'NONE',  ( -0.000000000000000000, 1.259100132267607459E-16, -1.000000000000000000 ) ) ;
#30378=CARTESIAN_POINT ( 'NONE',  ( -3.500000000000002220, 15.47927405783632970, -98.87764746908815994 ) ) ;
#30379=DIRECTION ( 'NONE',  ( -0.000000000000000000, 1.259100132267607459E-16, -1.000000000000000000 ) ) ;
#30381=CARTESIAN_POINT ( 'NONE',  ( -1.750000000000002220, 14.46891108675448301, -88.48806413671076143 ) ) ;
#30382=CARTESIAN_POINT ( 'NONE',  ( -1.655278471874999990, 20.36702641396248836, -70.01827246956612782 ) ) ;
#30386=LINE ( 'NONE', #1256, #3102 ) ;
#30387=CARTESIAN_POINT ( 'NONE',  ( -3.500000000000002220, 15.47927405783632260, -51.87764746908817415 ) ) ;
#30388=CARTESIAN_POINT ( 'NONE',  ( -1.749999999999999778, 20.53108891324555074, -74.12764746908817415 ) ) ;
#30390=CARTESIAN_POINT ( 'NONE',  ( 3.500000000000000000, 15.47927405783632970, -103.5443141357548456 ) ) ;
#30391=EDGE_LOOP ( 'NONE', ( #10952, #22130, #12021, #21822 ) ) ;
#30392=CARTESIAN_POINT ( 'NONE',  ( -1.750000000000002220, 14.46891108675447768, -41.48806413671076143 ) ) ;
#30393=CARTESIAN_POINT ( 'NONE',  ( 1.749999999999998224, 14.46891108675447768, -55.32139747004409713 ) ) ;
#30394=CARTESIAN_POINT ( 'NONE',  ( 1.655278471874998436, 14.63297358603753651, -24.51827246956613138 ) ) ;
#30395=CARTESIAN_POINT ( 'NONE',  ( 3.500000000000001332, 19.52072594216371115, -76.07139747004410424 ) ) ;
#30396=CARTESIAN_POINT ( 'NONE',  ( 4.648177544792955347E-16, 21.00000000000001776, -90.90473080337741862 ) ) ;
#30398=CARTESIAN_POINT ( 'NONE',  ( 1.749999999999998224, 14.46891108675447413, -36.32139747004409003 ) ) ;
#30400=CARTESIAN_POINT ( 'NONE',  ( 3.310556943750001313, 19.41135094264166838, -77.18077246956613635 ) ) ;
#30401=CARTESIAN_POINT ( 'NONE',  ( 3.500000000000000000, 15.47927405783632970, -98.54431413575484555 ) ) ;
#30403=DIRECTION ( 'NONE',  ( -0.000000000000000000, 1.259100132267607459E-16, -1.000000000000000000 ) ) ;
#30406=EDGE_CURVE ( 'NONE', #5345, #31245, #40071, .T. ) ;
#30408=CARTESIAN_POINT ( 'NONE',  ( -3.310556943750001313, 17.50000000000001776, -84.76410580289947916 ) ) ;
#30409=VERTEX_POINT ( 'NONE', #8161 ) ;
#30410=ORIENTED_EDGE ( 'NONE', *, *, #41548, .F. ) ;
#30414=CARTESIAN_POINT ( 'NONE',  ( 0.000000000000000000, 17.50000000000002487, -149.5231586289125687 ) ) ;
#30415=CARTESIAN_POINT ( 'NONE',  ( -1.655278471875002211, 14.63297358603755249, -127.5974391362328078 ) ) ;
#30416=ORIENTED_EDGE ( 'NONE', *, *, #22858, .F. ) ;
#30417=CARTESIAN_POINT ( 'NONE',  ( 0.000000000000000000, 17.50000000000002487, -149.5231586289125687 ) ) ;
#30418=CARTESIAN_POINT ( 'NONE',  ( -7.022189441860112050E-16, 13.67729811471671830, -56.60160580289947063 ) ) ;
#30419=CARTESIAN_POINT ( 'NONE',  ( 1.655278471875001101, 20.36702641396249547, -112.1849391362327992 ) ) ;
#30421=CARTESIAN_POINT ( 'NONE',  ( 3.500000000000001332, 17.50000000000002132, -123.1547308033774186 ) ) ;
#30422=CARTESIAN_POINT ( 'NONE',  ( -1.655278471875002211, 14.63297358603754006, -37.59743913623281486 ) ) ;
#30423=CARTESIAN_POINT ( 'NONE',  ( -1.655278471874999990, 20.36702641396248836, -69.01827246956612782 ) ) ;
#30424=CARTESIAN_POINT ( 'NONE',  ( -3.500000000000002220, 15.47927405783633503, -119.8776474690881741 ) ) ;
#30425=CARTESIAN_POINT ( 'NONE',  ( 3.310556943749999981, 15.58864905735836892, -94.34743913623280775 ) ) ;
#30426=CARTESIAN_POINT ( 'NONE',  ( 3.500000000000001332, 17.50000000000001776, -98.15473080337743284 ) ) ;
#30427=CARTESIAN_POINT ( 'NONE',  ( 3.500000000000000000, 15.47927405783632082, -52.23806413671078275 ) ) ;
#30430=CARTESIAN_POINT ( 'NONE',  ( 1.749999999999998224, 14.46891108675447946, -69.62764746908817415 ) ) ;
#30432=CARTESIAN_POINT ( 'NONE',  ( -1.749999999999999778, 20.53108891324554719, -44.12764746908817415 ) ) ;
#30433=CARTESIAN_POINT ( 'NONE',  ( 2.340729813953370519E-16, 21.32270188528330479, -31.01410580289947205 ) ) ;
#30434=CARTESIAN_POINT ( 'NONE',  ( 1.655278471874998436, 14.63297358603754539, -91.51827246956612782 ) ) ;
#30435=CARTESIAN_POINT ( 'NONE',  ( 3.500000000000001776, 19.52072594216370760, -60.07139747004409713 ) ) ;
#30436=DIRECTION ( 'NONE',  ( 0.000000000000000000, 1.000000000000000000, 0.000000000000000000 ) ) ;
#30437=CARTESIAN_POINT ( 'NONE',  ( -3.310556943750002201, 15.58864905735837780, -110.7682724695661420 ) ) ;
#30438=CARTESIAN_POINT ( 'NONE',  ( -3.310556943750000425, 19.41135094264166128, -41.93493913623279212 ) ) ;
#30440=CARTESIAN_POINT ( 'NONE',  ( 4.648177544792955347E-16, 21.00000000000001066, -38.21098080242150985 ) ) ;
#30445=CARTESIAN_POINT ( 'NONE',  ( 3.310556943750001313, 19.41135094264166838, -92.18077246956613635 ) ) ;
#30446=CARTESIAN_POINT ( 'NONE',  ( -0.9378221735089221633, 14.00000000000001599, -135.4493890021159359 ) ) ;
#30453=ORIENTED_EDGE ( 'NONE', *, *, #29008, .T. ) ;
#30456=( BOUNDED_CURVE ( )  B_SPLINE_CURVE ( 2, ( #13185, #15974, #35934, #29124, #26172, #25541, #25748, #25960, #35101 ),
 .UNSPECIFIED., .F., .T. ) 
 B_SPLINE_CURVE_WITH_KNOTS ( ( 3, 2, 2, 2, 3 ),
 ( 0.2895833333333333592, 0.2902777777777778012, 0.2916666666666666852, 0.2930555555555555691, 0.2937500000000000111 ),
 .UNSPECIFIED. ) 
 CURVE ( )  GEOMETRIC_REPRESENTATION_ITEM ( )  RATIONAL_B_SPLINE_CURVE ( ( 0.9330127018922194093, 0.9330127018922220739, 1.000000000000000000, 0.8660254037844387076, 1.000000000000000000, 0.8660254037844387076, 1.000000000000000000, 0.9330127018922194093, 0.9330127018922194093 ) ) 
 REPRESENTATION_ITEM ( '' )  );
#30462=EDGE_CURVE ( 'NONE', #10316, #15387, #1783, .T. ) ;
#30464=CARTESIAN_POINT ( 'NONE',  ( -1.394453263437886604E-15, 14.00000000000001066, -27.40473080337743284 ) ) ;
#30466=CARTESIAN_POINT ( 'NONE',  ( -3.310556943750001313, 17.50000000000002487, -140.7641058028994792 ) ) ;
#30469=CARTESIAN_POINT ( 'NONE',  ( -7.022189441860112050E-16, 13.67729811471672718, -131.6016058028994564 ) ) ;
#30470=CARTESIAN_POINT ( 'NONE',  ( -3.310556943750000425, 19.41135094264166128, -57.93493913623279923 ) ) ;
#30473=CARTESIAN_POINT ( 'NONE',  ( 1.750000000000001110, 20.53108891324556140, -139.9880641367107614 ) ) ;
#30474=CARTESIAN_POINT ( 'NONE',  ( 0.9378221735089300459, 21.00000000000001066, -36.94938900211595723 ) ) ;
#30476=CARTESIAN_POINT ( 'NONE',  ( -3.500000000000002220, 15.47927405783633503, -132.8776474690881741 ) ) ;
#30477=CARTESIAN_POINT ( 'NONE',  ( -1.655278471874999990, 20.36702641396249547, -110.9307724695661506 ) ) ;
#30480=CARTESIAN_POINT ( 'NONE',  ( -3.500000000000001332, 17.50000000000001776, -87.96098080242151696 ) ) ;
#30483=CARTESIAN_POINT ( 'NONE',  ( 3.310556943750001313, 17.50000000000001421, -49.26410580289947205 ) ) ;
#30484=CARTESIAN_POINT ( 'NONE',  ( -1.655278471875002211, 14.63297358603754894, -106.6849391362327992 ) ) ;
#30485=CARTESIAN_POINT ( 'NONE',  ( -3.500000000000002220, 15.47927405783632970, -93.87764746908815994 ) ) ;
#30486=CARTESIAN_POINT ( 'NONE',  ( -1.749999999999999778, 20.53108891324555429, -99.82139747004409003 ) ) ;
#30488=CARTESIAN_POINT ( 'NONE',  ( -1.655278471874999990, 20.36702641396249547, -128.0182724695661136 ) ) ;
#30491=DIRECTION ( 'NONE',  ( -0.000000000000000000, 1.259100132267607459E-16, -1.000000000000000000 ) ) ;
#30492=DIRECTION ( 'NONE',  ( -0.000000000000000000, 1.259100132267607459E-16, -1.000000000000000000 ) ) ;
#30493=CARTESIAN_POINT ( 'NONE',  ( 1.655278471875001101, 20.36702641396248836, -60.18493913623279923 ) ) ;
#30494=ORIENTED_EDGE ( 'NONE', *, *, #27855, .F. ) ;
#30495=CARTESIAN_POINT ( 'NONE',  ( 3.310556943750001313, 19.41135094264166838, -80.26827246956614204 ) ) ;
#30500=CARTESIAN_POINT ( 'NONE',  ( 2.340729813953370519E-16, 21.32270188528330834, -39.01410580289948626 ) ) ;
#30502=CARTESIAN_POINT ( 'NONE',  ( -3.310556943750001313, 17.50000000000001776, -100.7641058028994792 ) ) ;
#30504=( BOUNDED_CURVE ( )  B_SPLINE_CURVE ( 2, ( #12963, #38907, #403, #11040, #13378, #32940, #7856, #24022, #39959 ),
 .UNSPECIFIED., .F., .F. ) 
 B_SPLINE_CURVE_WITH_KNOTS ( ( 3, 2, 2, 2, 3 ),
 ( 0.9354166666666666741, 0.9361111111111111160, 0.9375000000000000000, 0.9388888888888888840, 0.9395833333333333259 ),
 .UNSPECIFIED. ) 
 CURVE ( )  GEOMETRIC_REPRESENTATION_ITEM ( )  RATIONAL_B_SPLINE_CURVE ( ( 0.9330127018922194093, 0.9330127018922194093, 1.000000000000000000, 0.8660254037844387076, 1.000000000000000000, 0.8660254037844387076, 1.000000000000000000, 0.9330127018922194093, 0.9330127018922194093 ) ) 
 REPRESENTATION_ITEM ( '' )  );
#30508=CARTESIAN_POINT ( 'NONE',  ( -3.310556943750000425, 19.41135094264166128, -50.84743913623280775 ) ) ;
#30511=AXIS2_PLACEMENT_3D ( 'NONE', #34217, #8065, #18260 ) ;
#30516=ORIENTED_EDGE ( 'NONE', *, *, #39950, .F. ) ;
#30518=CARTESIAN_POINT ( 'NONE',  ( 3.500000000000001776, 19.52072594216370405, -43.37764746908818125 ) ) ;
#30524=CARTESIAN_POINT ( 'NONE',  ( 2.340729813953370519E-16, 21.32270188528330479, -28.10160580289947418 ) ) ;
#30525=CARTESIAN_POINT ( 'NONE',  ( 4.648177544792955347E-16, 21.00000000000001421, -59.90473080337743284 ) ) ;
#30526=CARTESIAN_POINT ( 'NONE',  ( 1.655278471874998436, 14.63297358603754539, -81.51827246956614204 ) ) ;
#30527=CARTESIAN_POINT ( 'NONE',  ( 3.310556943749999981, 15.58864905735837425, -131.3474391362327935 ) ) ;
#30531=CARTESIAN_POINT ( 'NONE',  ( -3.310556943750002645, 15.58864905735837780, -121.7682724695661278 ) ) ;
#30533=CARTESIAN_POINT ( 'NONE',  ( -3.310556943750002645, 15.58864905735837247, -86.68077246956615056 ) ) ;
#30535=CARTESIAN_POINT ( 'NONE',  ( 4.648177544792955347E-16, 21.00000000000001421, -61.90473080337742573 ) ) ;
#30536=CARTESIAN_POINT ( 'NONE',  ( 0.9378221735089300459, 21.00000000000001421, -66.94938900211595012 ) ) ;
#30537=CARTESIAN_POINT ( 'NONE',  ( 1.749999999999998224, 14.46891108675447946, -70.32139747004409003 ) ) ;
#30538=CARTESIAN_POINT ( 'NONE',  ( -1.655278471875002211, 14.63297358603754361, -54.68493913623280633 ) ) ;
#30542=CARTESIAN_POINT ( 'NONE',  ( 2.340729813953370519E-16, 21.32270188528331190, -81.10160580289945642 ) ) ;
#30543=CARTESIAN_POINT ( 'NONE',  ( -1.655278471875002211, 14.63297358603755427, -140.6849391362327708 ) ) ;
#30546=CARTESIAN_POINT ( 'NONE',  ( -3.310556943750001313, 17.50000000000001776, -101.7641058028994792 ) ) ;
#30547=CARTESIAN_POINT ( 'NONE',  ( -3.310556943750001313, 17.50000000000001421, -73.76410580289947916 ) ) ;
#30548=DIRECTION ( 'NONE',  ( -0.000000000000000000, 1.259100132267607459E-16, -1.000000000000000000 ) ) ;
#30550=CARTESIAN_POINT ( 'NONE',  ( -3.310556943750001313, 17.50000000000001776, -96.85160580289945642 ) ) ;
#30552=FACE_OUTER_BOUND ( 'NONE', #31708, .T. ) ;
#30553=EDGE_CURVE ( 'NONE', #30683, #12051, #7961, .T. ) ;
#30554=CARTESIAN_POINT ( 'NONE',  ( -0.9378221735089310451, 14.00000000000001066, -37.75563900116004135 ) ) ;
#30556=CARTESIAN_POINT ( 'NONE',  ( -3.310556943750000425, 19.41135094264166483, -55.84743913623280065 ) ) ;
#30557=EDGE_CURVE ( 'NONE', #42029, #4518, #38646, .T. ) ;
#30558=CARTESIAN_POINT ( 'NONE',  ( -3.310556943750001313, 17.50000000000002132, -118.7641058028994792 ) ) ;
#30563=ORIENTED_EDGE ( 'NONE', *, *, #1981, .F. ) ;
#30567=CARTESIAN_POINT ( 'NONE',  ( 1.655278471875001101, 20.36702641396248836, -67.09743913623280775 ) ) ;
#30568=ORIENTED_EDGE ( 'NONE', *, *, #904, .T. ) ;
#30571=CARTESIAN_POINT ( 'NONE',  ( 0.9378221735089300459, 21.00000000000001776, -83.25563900116002003 ) ) ;
#30576=CARTESIAN_POINT ( 'NONE',  ( 2.340729813953370519E-16, 21.32270188528332255, -135.0141058028994507 ) ) ;
#30579=CARTESIAN_POINT ( 'NONE',  ( -1.655278471875002211, 14.63297358603754184, -43.68493913623279212 ) ) ;
#30581=CARTESIAN_POINT ( 'NONE',  ( -1.655278471874999990, 20.36702641396248481, -31.01827246956613493 ) ) ;
#30582=CARTESIAN_POINT ( 'NONE',  ( -7.022189441860112050E-16, 13.67729811471672541, -96.60160580289947063 ) ) ;
#30585=CARTESIAN_POINT ( 'NONE',  ( 1.655278471874998436, 14.63297358603755249, -141.5182724695661420 ) ) ;
#30586=DIRECTION ( 'NONE',  ( -0.000000000000000000, 1.259100132267607459E-16, -1.000000000000000000 ) ) ;
#30587=CARTESIAN_POINT ( 'NONE',  ( -3.500000000000001332, 17.50000000000001776, -93.96098080242151696 ) ) ;
#30588=CARTESIAN_POINT ( 'NONE',  ( -1.394453263437886604E-15, 14.00000000000001776, -100.4047308033774328 ) ) ;
#30589=EDGE_CURVE ( 'NONE', #36671, #17447, #28580, .T. ) ;
#30590=CYLINDRICAL_SURFACE ( 'NONE', #36300, 3.499999999999999556 ) ;
#30591=CARTESIAN_POINT ( 'NONE',  ( -3.500000000000000888, 19.52072594216371115, -85.73806413671076143 ) ) ;
#30592=CARTESIAN_POINT ( 'NONE',  ( -7.022189441860112050E-16, 13.67729811471672186, -71.60160580289947063 ) ) ;
#30597=CARTESIAN_POINT ( 'NONE',  ( -3.500000000000000888, 19.52072594216370760, -47.04431413575484555 ) ) ;
#30598=CARTESIAN_POINT ( 'NONE',  ( -3.310556943750000425, 19.41135094264166838, -117.8474391362328078 ) ) ;
#30599=LINE ( 'NONE', #14442, #29171 ) ;
#30601=ORIENTED_EDGE ( 'NONE', *, *, #5439, .T. ) ;
#30602=CARTESIAN_POINT ( 'NONE',  ( -3.500000000000001332, 17.50000000000002132, -115.6547308033774328 ) ) ;
#30604=CARTESIAN_POINT ( 'NONE',  ( 3.500000000000000000, 15.47927405783632615, -76.23806413671076143 ) ) ;
#30605=CARTESIAN_POINT ( 'NONE',  ( 4.648177544792955347E-16, 21.00000000000001066, -37.90473080337743284 ) ) ;
#30608=CARTESIAN_POINT ( 'NONE',  ( 1.655278471874998436, 14.63297358603754361, -78.43077246956615056 ) ) ;
#30610=CARTESIAN_POINT ( 'NONE',  ( 1.749999999999998224, 14.46891108675448478, -116.3213974700440900 ) ) ;
#30611=EDGE_CURVE ( 'NONE', #36360, #13587, #31073, .T. ) ;
#30612=CARTESIAN_POINT ( 'NONE',  ( 0.9378221735089300459, 21.00000000000001066, -26.94938900211595012 ) ) ;
#30613=ORIENTED_EDGE ( 'NONE', *, *, #33888, .F. ) ;
#30614=CARTESIAN_POINT ( 'NONE',  ( -3.500000000000001332, 17.50000000000001421, -63.96098080242150274 ) ) ;
#30615=CARTESIAN_POINT ( 'NONE',  ( -3.310556943750000425, 19.41135094264166483, -86.84743913623280775 ) ) ;
#30617=ORIENTED_EDGE ( 'NONE', *, *, #19645, .F. ) ;
#30622=( BOUNDED_CURVE ( )  B_SPLINE_CURVE ( 2, ( #9226, #8807, #28157, #34960, #8384, #21364, #14986, #12417, #5829 ),
 .UNSPECIFIED., .F., .F. ) 
 B_SPLINE_CURVE_WITH_KNOTS ( ( 3, 2, 2, 2, 3 ),
 ( 0.3812499999999999778, 0.3819444444444444198, 0.3833333333333333592, 0.3847222222222222432, 0.3854166666666666852 ),
 .UNSPECIFIED. ) 
 CURVE ( )  GEOMETRIC_REPRESENTATION_ITEM ( )  RATIONAL_B_SPLINE_CURVE ( ( 0.9330127018922194093, 0.9330127018922194093, 1.000000000000000000, 0.8660254037844387076, 1.000000000000000000, 0.8660254037844387076, 1.000000000000000000, 0.9330127018922194093, 0.9330127018922194093 ) ) 
 REPRESENTATION_ITEM ( '' )  );
#30624=DIRECTION ( 'NONE',  ( -0.000000000000000000, 1.259100132267607459E-16, -1.000000000000000000 ) ) ;
#30625=CARTESIAN_POINT ( 'NONE',  ( 1.655278471874998436, 14.63297358603754006, -46.51827246956613493 ) ) ;
#30626=CARTESIAN_POINT ( 'NONE',  ( 3.310556943750001313, 17.50000000000002132, -115.3516058028994706 ) ) ;
#30627=ORIENTED_EDGE ( 'NONE', *, *, #5673, .T. ) ;
#30628=CARTESIAN_POINT ( 'NONE',  ( -1.749999999999999778, 20.53108891324555785, -122.8213974700441042 ) ) ;
#30629=VECTOR ( 'NONE', #36241, 1000.000000000000000 ) ;
#30631=CARTESIAN_POINT ( 'NONE',  ( -3.310556943750000425, 19.41135094264165772, -39.84743913623280775 ) ) ;
#30632=CARTESIAN_POINT ( 'NONE',  ( -7.022189441860112050E-16, 13.67729811471671830, -66.60160580289947063 ) ) ;
#30633=CARTESIAN_POINT ( 'NONE',  ( 2.474675557024783212E-16, 21.54145188432740099, -113.2109808024215170 ) ) ;
#30636=CARTESIAN_POINT ( 'NONE',  ( 3.310556943750001313, 19.41135094264166483, -98.18077246956613635 ) ) ;
#30638=CARTESIAN_POINT ( 'NONE',  ( -0.9378221735089310451, 14.00000000000000888, -25.75563900116002714 ) ) ;
#30639=CARTESIAN_POINT ( 'NONE',  ( 4.648177544792955347E-16, 21.00000000000001421, -70.90473080337743284 ) ) ;
#30641=CARTESIAN_POINT ( 'NONE',  ( 2.474675557024783212E-16, 21.54145188432739388, -66.21098080242150274 ) ) ;
#30642=CARTESIAN_POINT ( 'NONE',  ( 3.500000000000001332, 17.50000000000001776, -100.4609808024215027 ) ) ;
#30643=CARTESIAN_POINT ( 'NONE',  ( 1.655278471875001101, 20.36702641396248481, -32.09743913623280775 ) ) ;
#30644=AXIS2_PLACEMENT_3D ( 'NONE', #26251, #29201, #39199 ) ;
#30645=CARTESIAN_POINT ( 'NONE',  ( 2.340729813953370519E-16, 21.32270188528331190, -93.10160580289947063 ) ) ;
#30646=CARTESIAN_POINT ( 'NONE',  ( -1.750000000000002220, 14.46891108675447768, -53.48806413671076854 ) ) ;
#30648=CARTESIAN_POINT ( 'NONE',  ( 1.655278471875001101, 20.36702641396249547, -112.1849391362327992 ) ) ;
#30649=CARTESIAN_POINT ( 'NONE',  ( -1.655278471875002211, 14.63297358603754006, -35.68493913623279923 ) ) ;
#30656=CARTESIAN_POINT ( 'NONE',  ( -7.022189441860112050E-16, 13.67729811471672363, -93.51410580289950758 ) ) ;
#30659=ORIENTED_EDGE ( 'NONE', *, *, #28215, .F. ) ;
#30662=CARTESIAN_POINT ( 'NONE',  ( 3.500000000000001332, 17.50000000000001066, -46.46098080242150274 ) ) ;
#30668=VERTEX_POINT ( 'NONE', #38346 ) ;
#30673=ORIENTED_EDGE ( 'NONE', *, *, #19328, .F. ) ;
#30674=CARTESIAN_POINT ( 'NONE',  ( -3.500000000000001332, 17.50000000000001421, -53.96098080242150985 ) ) ;
#30676=CARTESIAN_POINT ( 'NONE',  ( 3.500000000000001332, 17.50000000000002487, -140.1547308033774186 ) ) ;
#30678=DIRECTION ( 'NONE',  ( -0.000000000000000000, 1.259100132267607459E-16, -1.000000000000000000 ) ) ;
#30679=EDGE_CURVE ( 'NONE', #18829, #3618, #19627, .T. ) ;
#30680=CARTESIAN_POINT ( 'NONE',  ( -3.500000000000000000, 19.52072594216370405, -26.73806413671076143 ) ) ;
#30681=CARTESIAN_POINT ( 'NONE',  ( -3.310556943750002645, 15.58864905735837780, -130.7682724695661420 ) ) ;
#30682=CARTESIAN_POINT ( 'NONE',  ( 3.310556943750001313, 19.41135094264166128, -54.26827246956613493 ) ) ;
#30683=VERTEX_POINT ( 'NONE', #39169 ) ;
#30685=CARTESIAN_POINT ( 'NONE',  ( -3.500000000000001332, 17.50000000000002487, -139.6547308033774186 ) ) ;
#30688=CARTESIAN_POINT ( 'NONE',  ( -3.500000000000001332, 17.50000000000002132, -127.9609808024215170 ) ) ;
#30689=CARTESIAN_POINT ( 'NONE',  ( -3.310556943750001313, 17.50000000000002132, -113.7641058028994792 ) ) ;
#30692=CARTESIAN_POINT ( 'NONE',  ( -1.749999999999999778, 20.53108891324555429, -86.12764746908817415 ) ) ;
#30694=CARTESIAN_POINT ( 'NONE',  ( 1.655278471874998436, 14.63297358603754006, -47.43077246956614346 ) ) ;
#30695=CARTESIAN_POINT ( 'NONE',  ( 2.340729813953370519E-16, 21.32270188528331900, -108.1016058028994706 ) ) ;
#30697=CARTESIAN_POINT ( 'NONE',  ( -3.500000000000002220, 15.47927405783633326, -99.57139747004409003 ) ) ;
#30700=CARTESIAN_POINT ( 'NONE',  ( 1.655278471875001101, 20.36702641396249547, -126.1849391362327992 ) ) ;
#30701=EDGE_CURVE ( 'NONE', #29352, #14873, #24011, .T. ) ;
#30704=CARTESIAN_POINT ( 'NONE',  ( 4.648177544792955347E-16, 21.00000000000001066, -27.21098080242150985 ) ) ;
#30705=LINE ( 'NONE', #36885, #35993 ) ;
#30706=( BOUNDED_CURVE ( )  B_SPLINE_CURVE ( 2, ( #20204, #16802, #7871, #29765, #10207, #19991, #4666, #30612, #14454 ),
 .UNSPECIFIED., .F., .T. ) 
 B_SPLINE_CURVE_WITH_KNOTS ( ( 3, 2, 2, 2, 3 ),
 ( 0.9645833333333333481, 0.9652777777777777901, 0.9666666666666666741, 0.9680555555555555580, 0.9687500000000000000 ),
 .UNSPECIFIED. ) 
 CURVE ( )  GEOMETRIC_REPRESENTATION_ITEM ( )  RATIONAL_B_SPLINE_CURVE ( ( 0.9330127018922194093, 0.9330127018922194093, 1.000000000000000000, 0.8660254037844387076, 1.000000000000000000, 0.8660254037844387076, 1.000000000000000000, 0.9330127018922194093, 0.9330127018922194093 ) ) 
 REPRESENTATION_ITEM ( '' )  );
#30707=CARTESIAN_POINT ( 'NONE',  ( -3.310556943750000425, 19.41135094264166128, -58.93493913623279212 ) ) ;
#30708=EDGE_CURVE ( 'NONE', #13493, #39088, #29696, .T. ) ;
#30711=CARTESIAN_POINT ( 'NONE',  ( 3.310556943750001313, 19.41135094264166838, -78.26827246956615625 ) ) ;
#30712=CARTESIAN_POINT ( 'NONE',  ( 3.500000000000000000, 15.47927405783632437, -58.23806413671076143 ) ) ;
#30713=CARTESIAN_POINT ( 'NONE',  ( 1.750000000000001110, 20.53108891324554719, -29.98806413671076143 ) ) ;
#30717=CARTESIAN_POINT ( 'NONE',  ( 1.655278471875001101, 20.36702641396248481, -39.09743913623281486 ) ) ;
#30718=CARTESIAN_POINT ( 'NONE',  ( -3.310556943750001313, 17.50000000000001776, -94.76410580289946495 ) ) ;
#30719=DIRECTION ( 'NONE',  ( -0.000000000000000000, 1.259100132267607459E-16, -1.000000000000000000 ) ) ;
#30724=CARTESIAN_POINT ( 'NONE',  ( 3.310556943750001313, 19.41135094264166128, -54.18077246956613635 ) ) ;
#30725=ORIENTED_EDGE ( 'NONE', *, *, #7847, .F. ) ;
#30726=ORIENTED_EDGE ( 'NONE', *, *, #28250, .F. ) ;
#30727=CARTESIAN_POINT ( 'NONE',  ( -0.9378221735089291577, 21.00000000000001066, -43.86007260463891555 ) ) ;
#30732=CARTESIAN_POINT ( 'NONE',  ( 3.500000000000001332, 17.50000000000002132, -112.4609808024215027 ) ) ;
#30733=CARTESIAN_POINT ( 'NONE',  ( 3.500000000000000000, 15.47927405783632082, -38.54431413575484555 ) ) ;
#30738=CARTESIAN_POINT ( 'NONE',  ( -1.750000000000002220, 14.46891108675449011, -141.7943141357548313 ) ) ;
#30739=CARTESIAN_POINT ( 'NONE',  ( 3.500000000000000000, 15.47927405783633326, -122.2380641367107614 ) ) ;
#30740=CARTESIAN_POINT ( 'NONE',  ( -3.310556943750002645, 15.58864905735837780, -128.6807724695661364 ) ) ;
#30744=CARTESIAN_POINT ( 'NONE',  ( -1.655278471874999990, 20.36702641396249547, -125.0182724695661278 ) ) ;
#30745=CARTESIAN_POINT ( 'NONE',  ( 0.9378221735089300459, 21.00000000000001066, -42.25563900116002714 ) ) ;
#30746=CARTESIAN_POINT ( 'NONE',  ( -3.310556943750001313, 17.50000000000001776, -88.76410580289947916 ) ) ;
#30749=CARTESIAN_POINT ( 'NONE',  ( 4.648177544792955347E-16, 21.00000000000002487, -130.2109808024214885 ) ) ;
#30750=CARTESIAN_POINT ( 'NONE',  ( 0.9378221735089300459, 21.00000000000001776, -88.94938900211595012 ) ) ;
#30751=CARTESIAN_POINT ( 'NONE',  ( -3.500000000000000888, 19.52072594216370760, -68.73806413671077564 ) ) ;
#30752=CARTESIAN_POINT ( 'NONE',  ( 3.310556943749999981, 15.58864905735836537, -54.43493913623280633 ) ) ;
#30756=CARTESIAN_POINT ( 'NONE',  ( -3.310556943750001313, 17.50000000000001776, -76.85160580289945642 ) ) ;
#30758=CARTESIAN_POINT ( 'NONE',  ( 3.310556943750001313, 17.50000000000001776, -101.2641058028994792 ) ) ;
#30759=CARTESIAN_POINT ( 'NONE',  ( 2.340729813953370519E-16, 21.32270188528331190, -75.01410580289947916 ) ) ;
#30761=( BOUNDED_CURVE ( )  B_SPLINE_CURVE ( 2, ( #12911, #557, #25889, #29693, #13527, #26515, #23324, #22691, #35668 ),
 .UNSPECIFIED., .F., .F. ) 
 B_SPLINE_CURVE_WITH_KNOTS ( ( 3, 2, 2, 2, 3 ),
 ( 0.1395833333333333370, 0.1402777777777777790, 0.1416666666666666630, 0.1430555555555555469, 0.1437499999999999889 ),
 .UNSPECIFIED. ) 
 CURVE ( )  GEOMETRIC_REPRESENTATION_ITEM ( )  RATIONAL_B_SPLINE_CURVE ( ( 0.9330127018922194093, 0.9330127018922194093, 1.000000000000000000, 0.8660254037844387076, 1.000000000000000000, 0.8660254037844387076, 1.000000000000000000, 0.9330127018922194093, 0.9330127018922194093 ) ) 
 REPRESENTATION_ITEM ( '' )  );
#30762=CARTESIAN_POINT ( 'NONE',  ( 1.655278471875001101, 20.36702641396249192, -97.18493913623279923 ) ) ;
#30765=DIRECTION ( 'NONE',  ( -0.000000000000000000, 1.259100132267607459E-16, -1.000000000000000000 ) ) ;
#30766=CARTESIAN_POINT ( 'NONE',  ( 0.000000000000000000, 21.00000000000002487, -149.5231586289125687 ) ) ;
#30767=CARTESIAN_POINT ( 'NONE',  ( -1.655278471874999990, 20.36702641396248836, -57.93077246956614346 ) ) ;
#30768=CARTESIAN_POINT ( 'NONE',  ( -0.9378221735089310451, 14.00000000000002309, -124.7556390011600342 ) ) ;
#30769=CARTESIAN_POINT ( 'NONE',  ( -3.310556943750000425, 19.41135094264166838, -114.8474391362327935 ) ) ;
#30771=EDGE_CURVE ( 'NONE', #22966, #12728, #33004, .T. ) ;
#30772=ORIENTED_EDGE ( 'NONE', *, *, #5095, .F. ) ;
#30776=CARTESIAN_POINT ( 'NONE',  ( 2.340729813953370519E-16, 21.32270188528330834, -70.01410580289947916 ) ) ;
#30778=ORIENTED_EDGE ( 'NONE', *, *, #3328, .T. ) ;
#30780=CARTESIAN_POINT ( 'NONE',  ( 1.749999999999998224, 14.46891108675448478, -112.3213974700441042 ) ) ;
#30783=AXIS2_PLACEMENT_3D ( 'NONE', #17467, #17670, #5102 ) ;
#30784=ORIENTED_EDGE ( 'NONE', *, *, #20402, .F. ) ;
#30787=CARTESIAN_POINT ( 'NONE',  ( -3.310556943750001313, 17.50000000000002487, -132.7641058028994507 ) ) ;
#30788=CARTESIAN_POINT ( 'NONE',  ( 1.749999999999998224, 14.46891108675448478, -119.6276474690881741 ) ) ;
#30789=CARTESIAN_POINT ( 'NONE',  ( -1.655278471874999990, 20.36702641396248481, -46.01827246956613493 ) ) ;
#30790=CARTESIAN_POINT ( 'NONE',  ( 1.655278471875001101, 20.36702641396248481, -35.18493913623279923 ) ) ;
#30791=CARTESIAN_POINT ( 'NONE',  ( -3.310556943750001313, 17.50000000000001776, -94.85160580289945642 ) ) ;
#30792=CARTESIAN_POINT ( 'NONE',  ( 3.500000000000000000, 15.47927405783631727, -23.23806413671076854 ) ) ;
#30793=EDGE_CURVE ( 'NONE', #37404, #6853, #37051, .T. ) ;
#30795=ADVANCED_FACE ( 'NONE', ( #32580 ), #3872, .T. ) ;
#30796=CARTESIAN_POINT ( 'NONE',  ( 3.310556943750001313, 17.50000000000002487, -141.3516058028994564 ) ) ;
#30797=CARTESIAN_POINT ( 'NONE',  ( 4.286263797015737581E-16, 14.00000000000002487, -149.5231586289125687 ) ) ;
#30798=CARTESIAN_POINT ( 'NONE',  ( 1.749999999999998224, 14.46891108675448301, -95.62764746908817415 ) ) ;
#30800=CARTESIAN_POINT ( 'NONE',  ( 4.648177544792955347E-16, 21.00000000000001421, -64.21098080242150274 ) ) ;
#30801=CARTESIAN_POINT ( 'NONE',  ( -3.500000000000001332, 17.50000000000001776, -84.65473080337743284 ) ) ;
#30802=CARTESIAN_POINT ( 'NONE',  ( 3.310556943750001313, 19.41135094264166483, -72.26827246956612782 ) ) ;
#30806=CYLINDRICAL_SURFACE ( 'NONE', #9910, 3.499999999999999556 ) ;
#30807=CARTESIAN_POINT ( 'NONE',  ( 2.474675557024783212E-16, 21.54145188432739388, -49.21098080242150274 ) ) ;
#30808=CARTESIAN_POINT ( 'NONE',  ( 3.310556943749999981, 15.58864905735837247, -117.3474391362327935 ) ) ;
#30812=CARTESIAN_POINT ( 'NONE',  ( 3.500000000000000000, 15.47927405783632970, -113.2380641367107614 ) ) ;
#30815=FACE_OUTER_BOUND ( 'NONE', #36474, .T. ) ;
#30819=CARTESIAN_POINT ( 'NONE',  ( -7.022189441860112050E-16, 13.67729811471672186, -73.51410580289947916 ) ) ;
#30820=CARTESIAN_POINT ( 'NONE',  ( 3.500000000000001332, 19.52072594216371115, -98.37764746908817415 ) ) ;
#30825=CARTESIAN_POINT ( 'NONE',  ( 3.500000000000001332, 19.52072594216371115, -88.37764746908817415 ) ) ;
#30826=CARTESIAN_POINT ( 'NONE',  ( -1.655278471874999990, 20.36702641396249192, -86.93077246956613635 ) ) ;
#30831=FACE_OUTER_BOUND ( 'NONE', #32389, .T. ) ;
#30832=AXIS2_PLACEMENT_3D ( 'NONE', #22483, #13539, #29489 ) ;
#30834=CARTESIAN_POINT ( 'NONE',  ( -3.500000000000002220, 15.47927405783633503, -126.5713974700440900 ) ) ;
#30835=CARTESIAN_POINT ( 'NONE',  ( -1.655278471875002211, 14.63297358603754184, -48.68493913623279923 ) ) ;
#30836=CARTESIAN_POINT ( 'NONE',  ( -1.655278471875002211, 14.63297358603755072, -114.6849391362327850 ) ) ;
#30838=EDGE_CURVE ( 'NONE', #4203, #524, #30027, .T. ) ;
#30839=EDGE_CURVE ( 'NONE', #12339, #39978, #34057, .T. ) ;
#30840=CARTESIAN_POINT ( 'NONE',  ( 1.750000000000001110, 20.53108891324555785, -121.9880641367107614 ) ) ;
#30841=EDGE_CURVE ( 'NONE', #24347, #37404, #7490, .T. ) ;
#30842=CARTESIAN_POINT ( 'NONE',  ( 1.655278471875001101, 20.36702641396248481, -32.09743913623280775 ) ) ;
#30844=CARTESIAN_POINT ( 'NONE',  ( 2.340729813953370519E-16, 21.32270188528330834, -69.10160580289947063 ) ) ;
#30845=CARTESIAN_POINT ( 'NONE',  ( -7.424026671074350129E-16, 13.45854811567263987, -111.7109808024215027 ) ) ;
#30847=CARTESIAN_POINT ( 'NONE',  ( -3.310556943750000425, 19.41135094264166483, -98.84743913623280775 ) ) ;
#30848=CARTESIAN_POINT ( 'NONE',  ( 4.648177544792955347E-16, 21.00000000000001421, -59.90473080337743284 ) ) ;
#30849=CARTESIAN_POINT ( 'NONE',  ( -1.749999999999999778, 20.53108891324555785, -124.8213974700440900 ) ) ;
#30850=CARTESIAN_POINT ( 'NONE',  ( -1.394453263437886604E-15, 14.00000000000002132, -124.7109808024214885 ) ) ;
#30852=CARTESIAN_POINT ( 'NONE',  ( 3.500000000000000000, 15.47927405783632260, -62.54431413575483845 ) ) ;
#30854=CARTESIAN_POINT ( 'NONE',  ( -3.310556943750002645, 15.58864905735836537, -29.68077246956614701 ) ) ;
#30855=CARTESIAN_POINT ( 'NONE',  ( -3.310556943750001313, 17.50000000000001776, -90.85160580289947063 ) ) ;
#30856=CARTESIAN_POINT ( 'NONE',  ( 1.749999999999998224, 14.46891108675447590, -53.32139747004409003 ) ) ;
#30857=LINE ( 'NONE', #4699, #26685 ) ;
#30858=CARTESIAN_POINT ( 'NONE',  ( 1.655278471875001101, 20.36702641396249547, -108.1849391362327992 ) ) ;
#30859=CARTESIAN_POINT ( 'NONE',  ( -7.022189441860112050E-16, 13.67729811471671830, -40.60160580289947063 ) ) ;
#30867=CARTESIAN_POINT ( 'NONE',  ( -7.022189441860112050E-16, 13.67729811471672363, -86.51410580289947916 ) ) ;
#30872=CARTESIAN_POINT ( 'NONE',  ( 4.648177544792955347E-16, 21.00000000000001421, -65.21098080242150274 ) ) ;
#30873=ORIENTED_EDGE ( 'NONE', *, *, #39972, .F. ) ;
#30879=CARTESIAN_POINT ( 'NONE',  ( 0.9378221735089300459, 21.00000000000001776, -81.94938900211595012 ) ) ;
#30880=( BOUNDED_CURVE ( )  B_SPLINE_CURVE ( 2, ( #10738, #27333, #20311, #37322, #20527, #30939, #17546, #7769, #11169 ),
 .UNSPECIFIED., .F., .T. ) 
 B_SPLINE_CURVE_WITH_KNOTS ( ( 3, 2, 2, 2, 3 ),
 ( 0.3687500000000000222, 0.3694444444444444642, 0.3708333333333333481, 0.3722222222222222321, 0.3729166666666666741 ),
 .UNSPECIFIED. ) 
 CURVE ( )  GEOMETRIC_REPRESENTATION_ITEM ( )  RATIONAL_B_SPLINE_CURVE ( ( 0.9330127018922194093, 0.9330127018922194093, 1.000000000000000000, 0.8660254037844387076, 1.000000000000000000, 0.8660254037844387076, 1.000000000000000000, 0.9330127018922194093, 0.9330127018922194093 ) ) 
 REPRESENTATION_ITEM ( '' )  );
#30881=EDGE_CURVE ( 'NONE', #16691, #5302, #40024, .T. ) ;
#30885=EDGE_CURVE ( 'NONE', #38542, #31391, #14506, .T. ) ;
#30889=CARTESIAN_POINT ( 'NONE',  ( -1.394453263437886604E-15, 14.00000000000002132, -132.4047308033774186 ) ) ;
#30890=LINE ( 'NONE', #31093, #5158 ) ;
#30891=CARTESIAN_POINT ( 'NONE',  ( 3.310556943750001313, 17.50000000000002487, -134.2641058028994507 ) ) ;
#30892=CARTESIAN_POINT ( 'NONE',  ( 3.500000000000001332, 19.52072594216371115, -78.37764746908817415 ) ) ;
#30894=CARTESIAN_POINT ( 'NONE',  ( -0.9378221735089310451, 14.00000000000001599, -63.44938900211594301 ) ) ;
#30895=CARTESIAN_POINT ( 'NONE',  ( -7.022189441860112050E-16, 13.67729811471672718, -128.6016058028994848 ) ) ;
#30896=CARTESIAN_POINT ( 'NONE',  ( -3.310556943750002645, 15.58864905735836714, -53.76827246956612782 ) ) ;
#30899=CARTESIAN_POINT ( 'NONE',  ( -7.424026671074350129E-16, 13.45854811567264164, -135.4047308033774186 ) ) ;
#30900=ADVANCED_FACE ( 'NONE', ( #31438 ), #17695, .T. ) ;
#30902=CARTESIAN_POINT ( 'NONE',  ( 2.474675557024783212E-16, 21.54145188432740099, -126.2109808024215312 ) ) ;
#30903=CARTESIAN_POINT ( 'NONE',  ( -3.310556943750001313, 17.50000000000002132, -114.7641058028994792 ) ) ;
#30907=CARTESIAN_POINT ( 'NONE',  ( -1.749999999999999778, 20.53108891324555429, -79.12764746908817415 ) ) ;
#30910=CARTESIAN_POINT ( 'NONE',  ( -3.310556943750002645, 15.58864905735836714, -47.68077246956615056 ) ) ;
#30911=CARTESIAN_POINT ( 'NONE',  ( 1.655278471874998436, 14.63297358603754716, -106.5182724695661278 ) ) ;
#30913=CARTESIAN_POINT ( 'NONE',  ( 4.648177544792955347E-16, 21.00000000000001066, -42.90473080337742573 ) ) ;
#30916=CARTESIAN_POINT ( 'NONE',  ( -3.310556943750001313, 17.50000000000002132, -128.8516058028994564 ) ) ;
#30919=CARTESIAN_POINT ( 'NONE',  ( 3.602337597214540226E-14, 14.00000000000002132, -116.7109808024215170 ) ) ;
#30921=CARTESIAN_POINT ( 'NONE',  ( -1.655278471875002211, 14.63297358603754361, -58.68493913623279212 ) ) ;
#30922=ORIENTED_EDGE ( 'NONE', *, *, #39614, .F. ) ;
#30923=CARTESIAN_POINT ( 'NONE',  ( 3.310556943750001313, 19.41135094264166838, -82.26827246956614204 ) ) ;
#30924=CARTESIAN_POINT ( 'NONE',  ( 4.648177544792955347E-16, 21.00000000000001776, -101.9047308033774186 ) ) ;
#30926=CARTESIAN_POINT ( 'NONE',  ( -0.9378221735089288247, 14.00000000000002309, -139.4493890021159359 ) ) ;
#30927=CYLINDRICAL_SURFACE ( 'NONE', #17395, 3.499999999999999556 ) ;
#30928=CARTESIAN_POINT ( 'NONE',  ( 0.9378221735089281585, 14.00000000000001599, -74.36007260463891555 ) ) ;
#30930=CARTESIAN_POINT ( 'NONE',  ( -3.310556943750000425, 19.41135094264166128, -38.84743913623281486 ) ) ;
#30934=ORIENTED_EDGE ( 'NONE', *, *, #386, .F. ) ;
#30936=CARTESIAN_POINT ( 'NONE',  ( -3.310556943750002645, 15.58864905735836714, -49.68077246956614346 ) ) ;
#30939=CARTESIAN_POINT ( 'NONE',  ( -3.500000000000002220, 15.47927405783633326, -98.57139747004409003 ) ) ;
#30945=CARTESIAN_POINT ( 'NONE',  ( -1.394453263437886604E-15, 14.00000000000002132, -112.7109808024214885 ) ) ;
#30946=CARTESIAN_POINT ( 'NONE',  ( -1.749999999999999778, 20.53108891324554719, -36.12764746908816704 ) ) ;
#30948=CARTESIAN_POINT ( 'NONE',  ( 3.500000000000000000, 15.47927405783633326, -119.2380641367107614 ) ) ;
#30950=CARTESIAN_POINT ( 'NONE',  ( -7.022189441860112050E-16, 13.67729811471671297, -24.60160580289946708 ) ) ;
#30951=CARTESIAN_POINT ( 'NONE',  ( 0.000000000000000000, 17.50000000000002487, -149.5231586289125687 ) ) ;
#30952=CARTESIAN_POINT ( 'NONE',  ( -7.022189441860112050E-16, 13.67729811471672718, -130.5141058028994507 ) ) ;
#30955=( BOUNDED_CURVE ( )  B_SPLINE_CURVE ( 2, ( #34980, #37960, #34764, #12430, #12006, #2229, #15209, #2441, #5632 ),
 .UNSPECIFIED., .F., .T. ) 
 B_SPLINE_CURVE_WITH_KNOTS ( ( 3, 2, 2, 2, 3 ),
 ( 0.5520833333333333703, 0.5527777777777778123, 0.5541666666666666963, 0.5555555555555555802, 0.5562500000000000222 ),
 .UNSPECIFIED. ) 
 CURVE ( )  GEOMETRIC_REPRESENTATION_ITEM ( )  RATIONAL_B_SPLINE_CURVE ( ( 0.9330127018922194093, 0.9330127018922194093, 1.000000000000000000, 0.8660254037844387076, 1.000000000000000000, 0.8660254037844387076, 1.000000000000000000, 0.9330127018922194093, 0.9330127018922194093 ) ) 
 REPRESENTATION_ITEM ( '' )  );
#30956=CARTESIAN_POINT ( 'NONE',  ( 3.500000000000001332, 17.50000000000001066, -29.15473080337743639 ) ) ;
#30957=CARTESIAN_POINT ( 'NONE',  ( 2.340729813953370519E-16, 21.32270188528331900, -124.1016058028994706 ) ) ;
#30959=CARTESIAN_POINT ( 'NONE',  ( -3.500000000000002220, 15.47927405783632260, -40.57139747004409713 ) ) ;
#30961=CARTESIAN_POINT ( 'NONE',  ( 3.500000000000000000, 15.47927405783633503, -130.5443141357548598 ) ) ;
#30962=CARTESIAN_POINT ( 'NONE',  ( 0.9378221735089281585, 14.00000000000001599, -67.36007260463890134 ) ) ;
#30963=CARTESIAN_POINT ( 'NONE',  ( -1.750000000000002220, 14.46891108675448123, -69.48806413671077564 ) ) ;
#30964=DIRECTION ( 'NONE',  ( -0.000000000000000000, 1.259100132267607459E-16, -1.000000000000000000 ) ) ;
#30965=CARTESIAN_POINT ( 'NONE',  ( -1.655278471875002211, 14.63297358603754184, -52.68493913623280633 ) ) ;
#30967=CARTESIAN_POINT ( 'NONE',  ( 4.648177544792955347E-16, 21.00000000000001421, -66.21098080242148853 ) ) ;
#30968=CARTESIAN_POINT ( 'NONE',  ( -3.310556943750001313, 17.50000000000001421, -73.85160580289947063 ) ) ;
#30970=CARTESIAN_POINT ( 'NONE',  ( -3.310556943750002201, 15.58864905735837425, -105.6807724695661364 ) ) ;
#30971=CARTESIAN_POINT ( 'NONE',  ( -3.310556943750001313, 17.50000000000001776, -75.76410580289946495 ) ) ;
#30972=ORIENTED_EDGE ( 'NONE', *, *, #14331, .T. ) ;
#30973=CARTESIAN_POINT ( 'NONE',  ( -7.022189441860112050E-16, 13.67729811471672363, -94.60160580289945642 ) ) ;
#30976=CARTESIAN_POINT ( 'NONE',  ( -3.500000000000002220, 15.47927405783632082, -32.87764746908818125 ) ) ;
#30977=CARTESIAN_POINT ( 'NONE',  ( -3.500000000000001332, 17.50000000000001776, -81.65473080337743284 ) ) ;
#30979=CARTESIAN_POINT ( 'NONE',  ( -3.310556943750002201, 15.58864905735836892, -57.68077246956615056 ) ) ;
#30981=CARTESIAN_POINT ( 'NONE',  ( -7.022189441860112050E-16, 13.67729811471672718, -112.5141058028994649 ) ) ;
#30986=CARTESIAN_POINT ( 'NONE',  ( -1.394453263437886604E-15, 14.00000000000001421, -76.40473080337740441 ) ) ;
#30987=CARTESIAN_POINT ( 'NONE',  ( -3.310556943750002645, 15.58864905735836892, -65.68077246956613635 ) ) ;
#30990=CARTESIAN_POINT ( 'NONE',  ( -0.9378221735089291577, 21.00000000000002487, -131.1663226036829712 ) ) ;
#30997=CARTESIAN_POINT ( 'NONE',  ( 3.310556943750001313, 17.50000000000002132, -128.2641058028994792 ) ) ;
#30998=CARTESIAN_POINT ( 'NONE',  ( 3.500000000000001332, 19.52072594216371826, -119.3776474690881741 ) ) ;
#30999=EDGE_CURVE ( 'NONE', #41828, #29511, #38402, .T. ) ;
#31000=AXIS2_PLACEMENT_3D ( 'NONE', #41030, #11881, #35273 ) ;
#31001=CARTESIAN_POINT ( 'NONE',  ( 3.310556943749999981, 15.58864905735836182, -39.43493913623280633 ) ) ;
#31002=CARTESIAN_POINT ( 'NONE',  ( -1.655278471875002211, 14.63297358603754006, -31.68493913623279923 ) ) ;
#31003=CARTESIAN_POINT ( 'NONE',  ( -3.310556943750001313, 17.50000000000001776, -90.85160580289947063 ) ) ;
#31004=CARTESIAN_POINT ( 'NONE',  ( 1.655278471874998436, 14.63297358603755249, -142.4307724695661364 ) ) ;
#31007=CARTESIAN_POINT ( 'NONE',  ( -1.655278471874999990, 20.36702641396249902, -140.0182724695661420 ) ) ;
#31008=CARTESIAN_POINT ( 'NONE',  ( -1.749999999999999778, 20.53108891324555429, -84.12764746908818836 ) ) ;
#31009=CARTESIAN_POINT ( 'NONE',  ( 2.474675557024783212E-16, 21.54145188432739744, -97.21098080242150274 ) ) ;
#31011=DIRECTION ( 'NONE',  ( -0.000000000000000000, 1.259100132267607459E-16, -1.000000000000000000 ) ) ;
#31012=CARTESIAN_POINT ( 'NONE',  ( -3.500000000000001332, 17.50000000000001776, -86.65473080337743284 ) ) ;
#31013=CARTESIAN_POINT ( 'NONE',  ( -3.310556943750001313, 17.50000000000001421, -70.85160580289947063 ) ) ;
#31015=CARTESIAN_POINT ( 'NONE',  ( -1.749999999999999778, 20.53108891324555785, -111.8213974700441042 ) ) ;
#31017=CYLINDRICAL_SURFACE ( 'NONE', #17380, 3.499999999999999556 ) ;
#31018=CARTESIAN_POINT ( 'NONE',  ( -3.500000000000001332, 17.50000000000001421, -49.96098080242150274 ) ) ;
#31019=CARTESIAN_POINT ( 'NONE',  ( 1.655278471874998436, 14.63297358603754894, -121.4307724695661364 ) ) ;
#31021=CARTESIAN_POINT ( 'NONE',  ( 3.500000000000000000, 15.47927405783632970, -95.54431413575485976 ) ) ;
#31022=ORIENTED_EDGE ( 'NONE', *, *, #30406, .T. ) ;
#31023=CARTESIAN_POINT ( 'NONE',  ( -1.750000000000002220, 14.46891108675448656, -115.4880641367107614 ) ) ;
#31025=CARTESIAN_POINT ( 'NONE',  ( -1.394453263437886604E-15, 14.00000000000001776, -97.71098080242148853 ) ) ;
#31029=CARTESIAN_POINT ( 'NONE',  ( -1.655278471874999990, 20.36702641396248836, -70.93077246956613635 ) ) ;
#31030=CARTESIAN_POINT ( 'NONE',  ( 0.9378221735089300459, 21.00000000000002132, -115.9493890021159501 ) ) ;
#31031=VERTEX_POINT ( 'NONE', #21868 ) ;
#31033=CARTESIAN_POINT ( 'NONE',  ( 1.750000000000001110, 20.53108891324554719, -25.29431413575484910 ) ) ;
#31034=CARTESIAN_POINT ( 'NONE',  ( -3.310556943750002645, 15.58864905735837247, -83.68077246956615056 ) ) ;
#31035=EDGE_CURVE ( 'NONE', #40713, #10589, #5497, .T. ) ;
#31037=ORIENTED_EDGE ( 'NONE', *, *, #24762, .T. ) ;
#31043=CARTESIAN_POINT ( 'NONE',  ( 3.310556943750001313, 17.50000000000001421, -49.35160580289946353 ) ) ;
#31044=CARTESIAN_POINT ( 'NONE',  ( -1.655278471874999990, 20.36702641396249547, -109.0182724695661420 ) ) ;
#31046=EDGE_CURVE ( 'NONE', #24826, #12468, #19886, .T. ) ;
#31047=ADVANCED_FACE ( 'NONE', ( #12078 ), #7703, .T. ) ;
#31048=CARTESIAN_POINT ( 'NONE',  ( -1.655278471874999990, 20.36702641396248481, -32.93077246956614346 ) ) ;
#31049=CARTESIAN_POINT ( 'NONE',  ( -3.310556943750000425, 19.41135094264166128, -60.93493913623279923 ) ) ;
#31050=CARTESIAN_POINT ( 'NONE',  ( -1.750000000000002220, 14.46891108675448656, -111.7943141357548456 ) ) ;
#31052=CARTESIAN_POINT ( 'NONE',  ( -7.022189441860112050E-16, 13.67729811471672541, -95.51410580289947916 ) ) ;
#31053=CARTESIAN_POINT ( 'NONE',  ( 1.749999999999998224, 14.46891108675448301, -98.32139747004409003 ) ) ;
#31054=CARTESIAN_POINT ( 'NONE',  ( -3.695301148110399846E-14, 21.00000000000002132, -124.9047308033774186 ) ) ;
#31057=CARTESIAN_POINT ( 'NONE',  ( -7.424026671074350129E-16, 13.45854811567263454, -62.71098080242150274 ) ) ;
#31059=CARTESIAN_POINT ( 'NONE',  ( 1.655278471874998436, 14.63297358603753828, -30.43077246956614346 ) ) ;
#31060=CARTESIAN_POINT ( 'NONE',  ( 1.655278471875001101, 20.36702641396249192, -89.18493913623279923 ) ) ;
#31061=CARTESIAN_POINT ( 'NONE',  ( 3.500000000000001776, 19.52072594216370760, -55.07139747004409713 ) ) ;
#31063=CARTESIAN_POINT ( 'NONE',  ( -3.310556943750000425, 19.41135094264166838, -105.9349391362328277 ) ) ;
#31064=CARTESIAN_POINT ( 'NONE',  ( 3.310556943750001313, 17.50000000000001066, -40.35160580289947063 ) ) ;
#31072=CARTESIAN_POINT ( 'NONE',  ( -1.655278471875002211, 14.63297358603754716, -85.59743913623279354 ) ) ;
#31073=( BOUNDED_CURVE ( )  B_SPLINE_CURVE ( 2, ( #35364, #18993, #31542, #25801, #5384, #18363, #2195, #28141, #31958 ),
 .UNSPECIFIED., .F., .T. ) 
 B_SPLINE_CURVE_WITH_KNOTS ( ( 3, 2, 2, 2, 3 ),
 ( 0.5229166666666666963, 0.5236111111111111382, 0.5250000000000000222, 0.5263888888888889062, 0.5270833333333333481 ),
 .UNSPECIFIED. ) 
 CURVE ( )  GEOMETRIC_REPRESENTATION_ITEM ( )  RATIONAL_B_SPLINE_CURVE ( ( 0.9330127018922194093, 0.9330127018922194093, 1.000000000000000000, 0.8660254037844387076, 1.000000000000000000, 0.8660254037844387076, 1.000000000000000000, 0.9330127018922194093, 0.9330127018922194093 ) ) 
 REPRESENTATION_ITEM ( '' )  );
#31080=CARTESIAN_POINT ( 'NONE',  ( -3.500000000000000000, 19.52072594216370405, -31.04431413575484200 ) ) ;
#31084=CARTESIAN_POINT ( 'NONE',  ( 0.9378221735089281585, 14.00000000000002132, -118.3600726046389013 ) ) ;
#31086=ADVANCED_FACE ( 'NONE', ( #20679 ), #33656, .T. ) ;
#31088=DIRECTION ( 'NONE',  ( -0.000000000000000000, 1.259100132267607459E-16, -1.000000000000000000 ) ) ;
#31092=DIRECTION ( 'NONE',  ( -0.000000000000000000, 1.259100132267607459E-16, -1.000000000000000000 ) ) ;
#31093=CARTESIAN_POINT ( 'NONE',  ( 0.000000000000000000, 21.00000000000002487, -149.5231586289125687 ) ) ;
#31094=CARTESIAN_POINT ( 'NONE',  ( -1.655278471875002211, 14.63297358603755427, -136.5974391362328220 ) ) ;
#31095=CARTESIAN_POINT ( 'NONE',  ( 0.9378221735089281585, 14.00000000000002132, -104.3600726046389155 ) ) ;
#31096=VERTEX_POINT ( 'NONE', #24090 ) ;
#31097=CARTESIAN_POINT ( 'NONE',  ( -7.460324959392693302E-14, 21.00000000000001776, -101.2109808024215170 ) ) ;
#31098=CARTESIAN_POINT ( 'NONE',  ( -3.310556943750001313, 17.50000000000002132, -124.8516058028994564 ) ) ;
#31099=CARTESIAN_POINT ( 'NONE',  ( 3.310556943750001313, 17.50000000000001421, -53.35160580289946353 ) ) ;
#31100=VERTEX_POINT ( 'NONE', #41443 ) ;
#31102=CARTESIAN_POINT ( 'NONE',  ( 3.500000000000001332, 17.50000000000002487, -137.1547308033774186 ) ) ;
#31104=CARTESIAN_POINT ( 'NONE',  ( -3.500000000000001332, 17.50000000000002487, -130.9609808024214885 ) ) ;
#31105=CARTESIAN_POINT ( 'NONE',  ( 1.655278471875001101, 20.36702641396249547, -113.0974391362328078 ) ) ;
#31109=CARTESIAN_POINT ( 'NONE',  ( -7.424026671074350129E-16, 13.45854811567263631, -82.71098080242151696 ) ) ;
#31111=CARTESIAN_POINT ( 'NONE',  ( 3.310556943750001313, 19.41135094264166128, -48.18077246956614346 ) ) ;
#31112=CARTESIAN_POINT ( 'NONE',  ( 3.310556943750001313, 17.50000000000002132, -108.3516058028994564 ) ) ;
#31113=CARTESIAN_POINT ( 'NONE',  ( -1.750000000000002220, 14.46891108675448834, -129.7943141357548598 ) ) ;
#31117=CARTESIAN_POINT ( 'NONE',  ( -1.655278471874999990, 20.36702641396249547, -124.0182724695661278 ) ) ;
#31121=CARTESIAN_POINT ( 'NONE',  ( 3.500000000000000000, 15.47927405783633503, -130.2380641367107614 ) ) ;
#31122=CARTESIAN_POINT ( 'NONE',  ( 2.340729813953370519E-16, 21.32270188528330834, -61.10160580289946353 ) ) ;
#31123=ORIENTED_EDGE ( 'NONE', *, *, #16510, .F. ) ;
#31125=CARTESIAN_POINT ( 'NONE',  ( -3.310556943750002201, 15.58864905735837070, -73.76827246956612782 ) ) ;
#31129=CARTESIAN_POINT ( 'NONE',  ( 0.000000000000000000, 17.50000000000002487, -149.5231586289125687 ) ) ;
#31131=CARTESIAN_POINT ( 'NONE',  ( -7.022189441860112050E-16, 13.67729811471671830, -40.51410580289947916 ) ) ;
#31132=CARTESIAN_POINT ( 'NONE',  ( 7.367361408496833051E-14, 14.00000000000001776, -93.40473080337741862 ) ) ;
#31134=ADVANCED_FACE ( 'NONE', ( #35479 ), #29288, .T. ) ;
#31136=ORIENTED_EDGE ( 'NONE', *, *, #17160, .T. ) ;
#31138=CARTESIAN_POINT ( 'NONE',  ( 1.655278471875001101, 20.36702641396248481, -45.09743913623280775 ) ) ;
#31139=ORIENTED_EDGE ( 'NONE', *, *, #33630, .T. ) ;
#31145=CARTESIAN_POINT ( 'NONE',  ( 3.500000000000001332, 19.52072594216371115, -89.37764746908817415 ) ) ;
#31146=CARTESIAN_POINT ( 'NONE',  ( 1.749999999999998224, 14.46891108675447413, -38.62764746908817415 ) ) ;
#31147=LINE ( 'NONE', #2005, #29554 ) ;
#31148=CARTESIAN_POINT ( 'NONE',  ( 4.648177544792955347E-16, 21.00000000000001776, -82.21098080242150274 ) ) ;
#31150=CARTESIAN_POINT ( 'NONE',  ( -3.310556943750002645, 15.58864905735836182, -23.76827246956612782 ) ) ;
#31151=CARTESIAN_POINT ( 'NONE',  ( -1.394453263437886604E-15, 14.00000000000001421, -59.40473080337742573 ) ) ;
#31152=CARTESIAN_POINT ( 'NONE',  ( -3.310556943750002645, 15.58864905735837780, -130.6807724695661364 ) ) ;
#31155=DIRECTION ( 'NONE',  ( 0.000000000000000000, 1.000000000000000000, 0.000000000000000000 ) ) ;
#31156=CARTESIAN_POINT ( 'NONE',  ( 2.340729813953370519E-16, 21.32270188528331900, -123.1016058028994564 ) ) ;
#31157=CARTESIAN_POINT ( 'NONE',  ( 0.9378221735089300459, 21.00000000000002487, -140.9493890021159359 ) ) ;
#31158=CARTESIAN_POINT ( 'NONE',  ( 3.500000000000001776, 19.52072594216370405, -38.07139747004409713 ) ) ;
#31160=EDGE_CURVE ( 'NONE', #14868, #19157, #15929, .T. ) ;
#31161=CARTESIAN_POINT ( 'NONE',  ( -3.310556943750002201, 15.58864905735837958, -136.7682724695661420 ) ) ;
#31162=CARTESIAN_POINT ( 'NONE',  ( 3.500000000000000000, 15.47927405783632260, -63.23806413671076854 ) ) ;
#31163=CARTESIAN_POINT ( 'NONE',  ( 3.500000000000000000, 15.47927405783632082, -29.54431413575483134 ) ) ;
#31164=CARTESIAN_POINT ( 'NONE',  ( -3.310556943750000425, 19.41135094264166483, -48.93493913623281344 ) ) ;
#31166=CARTESIAN_POINT ( 'NONE',  ( -3.500000000000002220, 15.47927405783632793, -72.87764746908815994 ) ) ;
#31167=CARTESIAN_POINT ( 'NONE',  ( 1.655278471875001101, 20.36702641396248836, -74.18493913623279923 ) ) ;
#31169=CARTESIAN_POINT ( 'NONE',  ( 1.655278471874998436, 14.63297358603754716, -102.4307724695661364 ) ) ;
#31170=CARTESIAN_POINT ( 'NONE',  ( -1.655278471874999990, 20.36702641396248836, -68.93077246956613635 ) ) ;
#31171=ORIENTED_EDGE ( 'NONE', *, *, #23847, .T. ) ;
#31172=CARTESIAN_POINT ( 'NONE',  ( 1.655278471875001101, 20.36702641396249192, -95.18493913623279923 ) ) ;
#31175=FACE_OUTER_BOUND ( 'NONE', #9917, .T. ) ;
#31176=EDGE_CURVE ( 'NONE', #35536, #15700, #630, .T. ) ;
#31178=CARTESIAN_POINT ( 'NONE',  ( 3.310556943749999981, 15.58864905735836537, -56.34743913623280065 ) ) ;
#31179=CYLINDRICAL_SURFACE ( 'NONE', #136, 3.499999999999999556 ) ;
#31180=CARTESIAN_POINT ( 'NONE',  ( -3.310556943750002645, 15.58864905735837780, -110.6807724695661506 ) ) ;
#31181=AXIS2_PLACEMENT_3D ( 'NONE', #29655, #3710, #20516 ) ;
#31182=ORIENTED_EDGE ( 'NONE', *, *, #22007, .F. ) ;
#31187=CARTESIAN_POINT ( 'NONE',  ( -3.310556943750002645, 15.58864905735836892, -60.68077246956614346 ) ) ;
#31190=CARTESIAN_POINT ( 'NONE',  ( 3.500000000000000000, 15.47927405783632082, -30.54431413575483845 ) ) ;
#31192=CARTESIAN_POINT ( 'NONE',  ( -0.9378221735089303790, 14.00000000000002487, -142.4493890021159643 ) ) ;
#31194=LINE ( 'NONE', #11623, #2738 ) ;
#31197=CARTESIAN_POINT ( 'NONE',  ( 1.655278471875001101, 20.36702641396249902, -132.0974391362328220 ) ) ;
#31199=CARTESIAN_POINT ( 'NONE',  ( -7.022189441860112050E-16, 13.67729811471671653, -42.60160580289946353 ) ) ;
#31200=EDGE_CURVE ( 'NONE', #21407, #28825, #9964, .T. ) ;
#31201=CARTESIAN_POINT ( 'NONE',  ( 1.655278471874998436, 14.63297358603753828, -30.51827246956613493 ) ) ;
#31202=CARTESIAN_POINT ( 'NONE',  ( 3.310556943749999981, 15.58864905735836892, -93.43493913623281344 ) ) ;
#31203=CARTESIAN_POINT ( 'NONE',  ( -3.500000000000001332, 17.50000000000001066, -24.65473080337743284 ) ) ;
#31204=EDGE_LOOP ( 'NONE', ( #34681, #33977, #24055, #34235 ) ) ;
#31207=CARTESIAN_POINT ( 'NONE',  ( 3.310556943750001313, 19.41135094264167549, -137.2682724695661420 ) ) ;
#31208=CARTESIAN_POINT ( 'NONE',  ( 4.648177544792955347E-16, 21.00000000000001776, -84.21098080242150274 ) ) ;
#31209=CARTESIAN_POINT ( 'NONE',  ( -1.394453263437886604E-15, 14.00000000000001421, -73.40473080337743284 ) ) ;
#31210=CARTESIAN_POINT ( 'NONE',  ( -1.655278471875002211, 14.63297358603754361, -58.59743913623280065 ) ) ;
#31212=CARTESIAN_POINT ( 'NONE',  ( 3.500000000000001776, 19.52072594216371115, -85.07139747004407582 ) ) ;
#31213=CARTESIAN_POINT ( 'NONE',  ( -1.655278471875002211, 14.63297358603754539, -68.68493913623279923 ) ) ;
#31215=CARTESIAN_POINT ( 'NONE',  ( 0.000000000000000000, 21.00000000000002487, -149.5231586289125687 ) ) ;
#31216=DIRECTION ( 'NONE',  ( 0.000000000000000000, 1.000000000000000000, 0.000000000000000000 ) ) ;
#31218=CARTESIAN_POINT ( 'NONE',  ( -3.500000000000000888, 19.52072594216370760, -51.04431413575484555 ) ) ;
#31219=CARTESIAN_POINT ( 'NONE',  ( -1.655278471874999990, 20.36702641396249547, -118.9307724695661364 ) ) ;
#31220=ORIENTED_EDGE ( 'NONE', *, *, #7083, .T. ) ;
#31222=CARTESIAN_POINT ( 'NONE',  ( -1.750000000000002220, 14.46891108675448656, -111.4880641367107614 ) ) ;
#31226=EDGE_CURVE ( 'NONE', #39031, #18739, #42079, .T. ) ;
#31229=CARTESIAN_POINT ( 'NONE',  ( -3.310556943750000425, 19.41135094264166483, -69.84743913623280775 ) ) ;
#31233=CARTESIAN_POINT ( 'NONE',  ( -1.655278471875002211, 14.63297358603753828, -24.59743913623281486 ) ) ;
#31234=CARTESIAN_POINT ( 'NONE',  ( -0.9378221735089291577, 21.00000000000001066, -32.16632260368299256 ) ) ;
#31235=CARTESIAN_POINT ( 'NONE',  ( -3.310556943750002645, 15.58864905735837070, -79.68077246956613635 ) ) ;
#31236=ORIENTED_EDGE ( 'NONE', *, *, #33918, .F. ) ;
#31238=VECTOR ( 'NONE', #3351, 1000.000000000000000 ) ;
#31240=( BOUNDED_CURVE ( )  B_SPLINE_CURVE ( 2, ( #38732, #6613, #19576, #16407, #29350, #12148, #25140, #38105, #34911 ),
 .UNSPECIFIED., .F., .T. ) 
 B_SPLINE_CURVE_WITH_KNOTS ( ( 3, 2, 2, 2, 3 ),
 ( 0.5812500000000000444, 0.5819444444444444864, 0.5833333333333333703, 0.5847222222222222543, 0.5854166666666666963 ),
 .UNSPECIFIED. ) 
 CURVE ( )  GEOMETRIC_REPRESENTATION_ITEM ( )  RATIONAL_B_SPLINE_CURVE ( ( 0.9330127018922194093, 0.9330127018922194093, 1.000000000000000000, 0.8660254037844387076, 1.000000000000000000, 0.8660254037844387076, 1.000000000000000000, 0.9330127018922194093, 0.9330127018922194093 ) ) 
 REPRESENTATION_ITEM ( '' )  );
#31243=( BOUNDED_CURVE ( )  B_SPLINE_CURVE ( 2, ( #39813, #40019, #13646, #39588, #7054, #26842, #4291, #30020, #20672 ),
 .UNSPECIFIED., .F., .T. ) 
 B_SPLINE_CURVE_WITH_KNOTS ( ( 3, 2, 2, 2, 3 ),
 ( 0.8854166666666666297, 0.8861111111111110716, 0.8874999999999999556, 0.8888888888888888395, 0.8895833333333332815 ),
 .UNSPECIFIED. ) 
 CURVE ( )  GEOMETRIC_REPRESENTATION_ITEM ( )  RATIONAL_B_SPLINE_CURVE ( ( 0.9330127018922194093, 0.9330127018922194093, 1.000000000000000000, 0.8660254037844387076, 1.000000000000000000, 0.8660254037844387076, 1.000000000000000000, 0.9330127018922194093, 0.9330127018922194093 ) ) 
 REPRESENTATION_ITEM ( '' )  );
#31245=VERTEX_POINT ( 'NONE', #3557 ) ;
#31246=CYLINDRICAL_SURFACE ( 'NONE', #21399, 3.499999999999999556 ) ;
#31247=CARTESIAN_POINT ( 'NONE',  ( 2.340729813953370519E-16, 21.32270188528330834, -49.10160580289945642 ) ) ;
#31248=CARTESIAN_POINT ( 'NONE',  ( 3.310556943749999981, 15.58864905735837247, -109.4349391362327992 ) ) ;
#31249=VERTEX_POINT ( 'NONE', #19522 ) ;
#31250=CARTESIAN_POINT ( 'NONE',  ( -3.310556943750002645, 15.58864905735836537, -36.68077246956612925 ) ) ;
#31251=CARTESIAN_POINT ( 'NONE',  ( 1.655278471875001101, 20.36702641396248836, -61.18493913623279923 ) ) ;
#31252=CARTESIAN_POINT ( 'NONE',  ( -3.500000000000002220, 15.47927405783633503, -110.8776474690881884 ) ) ;
#31254=CARTESIAN_POINT ( 'NONE',  ( 3.310556943749999981, 15.58864905735837070, -96.34743913623280775 ) ) ;
#31255=CARTESIAN_POINT ( 'NONE',  ( 3.500000000000001332, 17.50000000000001421, -52.15473080337743284 ) ) ;
#31256=CARTESIAN_POINT ( 'NONE',  ( 0.9378221735089281585, 14.00000000000001776, -85.36007260463890134 ) ) ;
#31258=CARTESIAN_POINT ( 'NONE',  ( -7.424026671074350129E-16, 13.45854811567263454, -63.71098080242150985 ) ) ;
#31261=CARTESIAN_POINT ( 'NONE',  ( 2.340729813953370519E-16, 21.32270188528330479, -34.01410580289947205 ) ) ;
#31262=CARTESIAN_POINT ( 'NONE',  ( -3.500000000000001332, 17.50000000000001421, -55.65473080337743284 ) ) ;
#31264=CARTESIAN_POINT ( 'NONE',  ( -1.655278471874999990, 20.36702641396249547, -109.0182724695661420 ) ) ;
#31265=CARTESIAN_POINT ( 'NONE',  ( 2.340729813953370519E-16, 21.32270188528330834, -36.10160580289946353 ) ) ;
#31267=CARTESIAN_POINT ( 'NONE',  ( 3.500000000000001332, 17.50000000000002487, -143.4609808024215170 ) ) ;
#31271=DIRECTION ( 'NONE',  ( -0.000000000000000000, 1.259100132267607459E-16, -1.000000000000000000 ) ) ;
#31273=CARTESIAN_POINT ( 'NONE',  ( -7.022189441860112050E-16, 13.67729811471672363, -85.51410580289946495 ) ) ;
#31275=CARTESIAN_POINT ( 'NONE',  ( -0.9378221735089310451, 14.00000000000000888, -23.75563900116002714 ) ) ;
#31276=ORIENTED_EDGE ( 'NONE', *, *, #27257, .F. ) ;
#31279=CARTESIAN_POINT ( 'NONE',  ( 3.500000000000001332, 17.50000000000001421, -74.46098080242151696 ) ) ;
#31280=ORIENTED_EDGE ( 'NONE', *, *, #21041, .T. ) ;
#31284=ORIENTED_EDGE ( 'NONE', *, *, #22281, .T. ) ;
#31285=FACE_OUTER_BOUND ( 'NONE', #23875, .T. ) ;
#31294=CARTESIAN_POINT ( 'NONE',  ( 3.500000000000001332, 19.52072594216371826, -109.0713974700440900 ) ) ;
#31295=CYLINDRICAL_SURFACE ( 'NONE', #2457, 3.499999999999999556 ) ;
#31296=CARTESIAN_POINT ( 'NONE',  ( -7.022189441860112050E-16, 13.67729811471672896, -138.5141058028994792 ) ) ;
#31298=ORIENTED_EDGE ( 'NONE', *, *, #22281, .F. ) ;
#31299=CARTESIAN_POINT ( 'NONE',  ( 1.749999999999998224, 14.46891108675447768, -54.62764746908817415 ) ) ;
#31300=CARTESIAN_POINT ( 'NONE',  ( -3.310556943750000425, 19.41135094264166838, -126.9349391362328134 ) ) ;
#31301=CARTESIAN_POINT ( 'NONE',  ( -3.310556943750002645, 15.58864905735836892, -54.76827246956612072 ) ) ;
#31304=CARTESIAN_POINT ( 'NONE',  ( -7.424026671074350129E-16, 13.45854811567264164, -137.4047308033774186 ) ) ;
#31308=CARTESIAN_POINT ( 'NONE',  ( 2.340729813953370519E-16, 21.32270188528331190, -75.10160580289947063 ) ) ;
#31309=CARTESIAN_POINT ( 'NONE',  ( -3.500000000000002220, 15.47927405783633503, -125.8776474690881599 ) ) ;
#31310=CARTESIAN_POINT ( 'NONE',  ( 3.310556943749999981, 15.58864905735837247, -111.3474391362328078 ) ) ;
#31313=( BOUNDED_CURVE ( )  B_SPLINE_CURVE ( 2, ( #39917, #20785, #8010, #1421, #33542, #27370, #14394, #40343, #17791 ),
 .UNSPECIFIED., .F., .T. ) 
 B_SPLINE_CURVE_WITH_KNOTS ( ( 3, 2, 2, 2, 3 ),
 ( 0.4312500000000000222, 0.4319444444444444642, 0.4333333333333333481, 0.4347222222222222321, 0.4354166666666666741 ),
 .UNSPECIFIED. ) 
 CURVE ( )  GEOMETRIC_REPRESENTATION_ITEM ( )  RATIONAL_B_SPLINE_CURVE ( ( 0.9330127018922194093, 0.9330127018922194093, 1.000000000000000000, 0.8660254037844387076, 1.000000000000000000, 0.8660254037844387076, 1.000000000000000000, 0.9330127018922194093, 0.9330127018922194093 ) ) 
 REPRESENTATION_ITEM ( '' )  );
#31316=CARTESIAN_POINT ( 'NONE',  ( -3.500000000000000888, 19.52072594216371115, -78.04431413575485976 ) ) ;
#31317=LINE ( 'NONE', #2595, #6300 ) ;
#31318=CARTESIAN_POINT ( 'NONE',  ( 3.310556943749999981, 15.58864905735836182, -48.34743913623281486 ) ) ;
#31319=ADVANCED_FACE ( 'NONE', ( #16755 ), #13551, .T. ) ;
#31320=CARTESIAN_POINT ( 'NONE',  ( -3.310556943750000425, 19.41135094264166838, -104.9349391362327992 ) ) ;
#31323=CARTESIAN_POINT ( 'NONE',  ( 4.648177544792955347E-16, 21.00000000000001421, -72.90473080337743284 ) ) ;
#31324=CARTESIAN_POINT ( 'NONE',  ( -3.310556943750002201, 15.58864905735837780, -124.7682724695661278 ) ) ;
#31328=CARTESIAN_POINT ( 'NONE',  ( 1.750000000000001110, 20.53108891324554719, -31.98806413671076498 ) ) ;
#31329=CARTESIAN_POINT ( 'NONE',  ( 1.749999999999998224, 14.46891108675447768, -60.62764746908818125 ) ) ;
#31331=ORIENTED_EDGE ( 'NONE', *, *, #4668, .F. ) ;
#31332=CARTESIAN_POINT ( 'NONE',  ( 3.310556943750001313, 19.41135094264166838, -77.26827246956614204 ) ) ;
#31333=DIRECTION ( 'NONE',  ( -0.000000000000000000, 1.259100132267607459E-16, -1.000000000000000000 ) ) ;
#31334=CARTESIAN_POINT ( 'NONE',  ( -7.460324959392693302E-14, 21.00000000000002132, -102.9047308033774044 ) ) ;
#31335=CARTESIAN_POINT ( 'NONE',  ( -0.9378221735089310451, 14.00000000000001599, -55.75563900116002714 ) ) ;
#31338=CARTESIAN_POINT ( 'NONE',  ( 3.310556943750001313, 17.50000000000001066, -37.26410580289947205 ) ) ;
#31340=VECTOR ( 'NONE', #36873, 1000.000000000000000 ) ;
#31343=EDGE_LOOP ( 'NONE', ( #9818, #23135, #1846, #18706 ) ) ;
#31345=CARTESIAN_POINT ( 'NONE',  ( -1.655278471875002211, 14.63297358603754184, -47.59743913623280775 ) ) ;
#31346=VERTEX_POINT ( 'NONE', #16961 ) ;
#31347=ORIENTED_EDGE ( 'NONE', *, *, #40681, .T. ) ;
#31351=CARTESIAN_POINT ( 'NONE',  ( 3.500000000000001332, 17.50000000000001421, -63.15473080337742573 ) ) ;
#31352=DIRECTION ( 'NONE',  ( -0.000000000000000000, 1.259100132267607459E-16, -1.000000000000000000 ) ) ;
#31353=CARTESIAN_POINT ( 'NONE',  ( 1.749999999999998224, 14.46891108675447413, -39.62764746908817415 ) ) ;
#31358=CARTESIAN_POINT ( 'NONE',  ( 1.655278471874998436, 14.63297358603753651, -25.51827246956613138 ) ) ;
#31359=CARTESIAN_POINT ( 'NONE',  ( -0.9378221735089640188, 20.99999999999999645, -100.8600726046388871 ) ) ;
#31360=CARTESIAN_POINT ( 'NONE',  ( -1.655278471875002211, 14.63297358603755249, -129.5974391362328220 ) ) ;
#31363=EDGE_CURVE ( 'NONE', #12038, #22382, #7182, .T. ) ;
#31364=CARTESIAN_POINT ( 'NONE',  ( 0.9378221735089300459, 21.00000000000001066, -23.94938900211595723 ) ) ;
#31365=( BOUNDED_CURVE ( )  B_SPLINE_CURVE ( 2, ( #33167, #26376, #10424, #852, #17015, #10639, #29978, #13825, #16392 ),
 .UNSPECIFIED., .F., .T. ) 
 B_SPLINE_CURVE_WITH_KNOTS ( ( 3, 2, 2, 2, 3 ),
 ( 0.4604166666666666963, 0.4611111111111111382, 0.4625000000000000222, 0.4638888888888889062, 0.4645833333333333481 ),
 .UNSPECIFIED. ) 
 CURVE ( )  GEOMETRIC_REPRESENTATION_ITEM ( )  RATIONAL_B_SPLINE_CURVE ( ( 0.9330127018922194093, 0.9330127018922220739, 1.000000000000000000, 0.8660254037844387076, 1.000000000000000000, 0.8660254037844387076, 1.000000000000000000, 0.9330127018922194093, 0.9330127018922194093 ) ) 
 REPRESENTATION_ITEM ( '' )  );
#31368=CARTESIAN_POINT ( 'NONE',  ( -3.310556943750002645, 15.58864905735837780, -123.7682724695661420 ) ) ;
#31370=CARTESIAN_POINT ( 'NONE',  ( -3.500000000000000888, 19.52072594216370405, -37.73806413671076854 ) ) ;
#31371=CARTESIAN_POINT ( 'NONE',  ( 1.750000000000001110, 20.53108891324555785, -114.9880641367107614 ) ) ;
#31372=CARTESIAN_POINT ( 'NONE',  ( -1.655278471875002211, 14.63297358603755427, -138.6849391362327992 ) ) ;
#31374=CARTESIAN_POINT ( 'NONE',  ( 3.310556943749999981, 15.58864905735836182, -49.43493913623280633 ) ) ;
#31377=CARTESIAN_POINT ( 'NONE',  ( 3.310556943750001313, 19.41135094264166128, -74.26827246956614204 ) ) ;
#31379=CARTESIAN_POINT ( 'NONE',  ( -3.310556943750000425, 19.41135094264166838, -103.8474391362328220 ) ) ;
#31380=CARTESIAN_POINT ( 'NONE',  ( 3.310556943749999981, 15.58864905735836714, -72.34743913623279354 ) ) ;
#31381=ORIENTED_EDGE ( 'NONE', *, *, #20013, .F. ) ;
#31382=CARTESIAN_POINT ( 'NONE',  ( -7.022189441860112050E-16, 13.67729811471672363, -88.60160580289947063 ) ) ;
#31386=CARTESIAN_POINT ( 'NONE',  ( 1.749999999999998224, 14.46891108675448478, -117.6276474690881741 ) ) ;
#31387=CARTESIAN_POINT ( 'NONE',  ( -3.310556943750000425, 19.41135094264166483, -53.84743913623281486 ) ) ;
#31388=CARTESIAN_POINT ( 'NONE',  ( 0.000000000000000000, 17.50000000000002487, -149.5231586289125687 ) ) ;
#31389=CARTESIAN_POINT ( 'NONE',  ( 2.340729813953370519E-16, 21.32270188528331900, -112.0141058028994792 ) ) ;
#31391=VERTEX_POINT ( 'NONE', #29928 ) ;
#31395=CARTESIAN_POINT ( 'NONE',  ( -3.310556943750001313, 17.50000000000001421, -65.76410580289947916 ) ) ;
#31396=ORIENTED_EDGE ( 'NONE', *, *, #13644, .F. ) ;
#31398=CARTESIAN_POINT ( 'NONE',  ( 1.750000000000001110, 20.53108891324554719, -30.29431413575484200 ) ) ;
#31399=EDGE_CURVE ( 'NONE', #14042, #37421, #3770, .T. ) ;
#31403=EDGE_CURVE ( 'NONE', #16391, #21152, #23987, .T. ) ;
#31404=VERTEX_POINT ( 'NONE', #26751 ) ;
#31406=CARTESIAN_POINT ( 'NONE',  ( -3.310556943750000425, 19.41135094264166838, -127.8474391362328078 ) ) ;
#31407=CARTESIAN_POINT ( 'NONE',  ( -0.9378221735089377065, 21.00000000000001421, -128.8600726046389013 ) ) ;
#31408=CARTESIAN_POINT ( 'NONE',  ( 1.655278471875001101, 20.36702641396248481, -40.18493913623280633 ) ) ;
#31409=CARTESIAN_POINT ( 'NONE',  ( 3.310556943750001313, 19.41135094264165772, -32.26827246956613493 ) ) ;
#31412=CARTESIAN_POINT ( 'NONE',  ( -7.022189441860112050E-16, 13.67729811471672363, -91.60160580289947063 ) ) ;
#31413=CARTESIAN_POINT ( 'NONE',  ( -7.424026671074350129E-16, 13.45854811567263098, -23.40473080337742928 ) ) ;
#31415=VECTOR ( 'NONE', #19217, 1000.000000000000000 ) ;
#31417=CARTESIAN_POINT ( 'NONE',  ( -1.655278471875002211, 14.63297358603755427, -136.6849391362327992 ) ) ;
#31421=CARTESIAN_POINT ( 'NONE',  ( 3.500000000000000000, 15.47927405783632615, -83.23806413671074722 ) ) ;
#31422=CARTESIAN_POINT ( 'NONE',  ( -3.310556943750000425, 19.41135094264166483, -66.93493913623279923 ) ) ;
#31424=CARTESIAN_POINT ( 'NONE',  ( -3.500000000000001332, 17.50000000000001776, -90.96098080242151696 ) ) ;
#31425=CARTESIAN_POINT ( 'NONE',  ( -1.394453263437886604E-15, 14.00000000000002132, -119.4047308033774328 ) ) ;
#31426=ORIENTED_EDGE ( 'NONE', *, *, #19645, .T. ) ;
#31427=CARTESIAN_POINT ( 'NONE',  ( -3.310556943750000425, 19.41135094264166838, -120.8474391362328078 ) ) ;
#31429=LINE ( 'NONE', #15280, #27441 ) ;
#31431=CARTESIAN_POINT ( 'NONE',  ( 3.500000000000001332, 17.50000000000002132, -111.1547308033774328 ) ) ;
#31433=CARTESIAN_POINT ( 'NONE',  ( -3.500000000000000000, 19.52072594216371115, -82.73806413671074722 ) ) ;
#31436=CARTESIAN_POINT ( 'NONE',  ( 3.310556943750001313, 19.41135094264166483, -72.18077246956613635 ) ) ;
#31438=FACE_OUTER_BOUND ( 'NONE', #37370, .T. ) ;
#31439=CARTESIAN_POINT ( 'NONE',  ( 4.648177544792955347E-16, 21.00000000000001421, -72.21098080242150274 ) ) ;
#31441=CARTESIAN_POINT ( 'NONE',  ( 4.648177544792955347E-16, 21.00000000000002487, -133.2109808024214885 ) ) ;
#31443=FACE_OUTER_BOUND ( 'NONE', #8846, .T. ) ;
#31444=CARTESIAN_POINT ( 'NONE',  ( 1.655278471875001101, 20.36702641396249192, -81.09743913623280775 ) ) ;
#31448=CARTESIAN_POINT ( 'NONE',  ( -0.9378221735089291577, 21.00000000000001421, -48.86007260463891555 ) ) ;
#31450=EDGE_CURVE ( 'NONE', #18659, #11503, #20155, .T. ) ;
#31452=CYLINDRICAL_SURFACE ( 'NONE', #23316, 3.499999999999999556 ) ;
#31454=CARTESIAN_POINT ( 'NONE',  ( -1.655278471874999990, 20.36702641396248836, -47.01827246956613493 ) ) ;
#31456=CARTESIAN_POINT ( 'NONE',  ( 3.310556943750001313, 19.41135094264166838, -108.2682724695661278 ) ) ;
#31458=CARTESIAN_POINT ( 'NONE',  ( -1.655278471875002211, 14.63297358603754006, -35.59743913623280775 ) ) ;
#31459=CARTESIAN_POINT ( 'NONE',  ( 2.340729813953370519E-16, 21.32270188528330834, -63.10160580289946353 ) ) ;
#31460=CARTESIAN_POINT ( 'NONE',  ( 1.750000000000001110, 20.53108891324555785, -108.2943141357548456 ) ) ;
#31462=CARTESIAN_POINT ( 'NONE',  ( -1.655278471875002211, 14.63297358603754716, -89.59743913623280775 ) ) ;
#31464=CARTESIAN_POINT ( 'NONE',  ( -1.750000000000002220, 14.46891108675448478, -95.48806413671076143 ) ) ;
#31465=CARTESIAN_POINT ( 'NONE',  ( 1.750000000000001110, 20.53108891324555074, -63.29431413575484555 ) ) ;
#31469=CARTESIAN_POINT ( 'NONE',  ( -3.500000000000000888, 19.52072594216370760, -67.04431413575484555 ) ) ;
#31470=CARTESIAN_POINT ( 'NONE',  ( -3.500000000000002220, 15.47927405783632793, -71.87764746908817415 ) ) ;
#31471=CARTESIAN_POINT ( 'NONE',  ( 1.655278471874998436, 14.63297358603753828, -26.43077246956613990 ) ) ;
#31472=CARTESIAN_POINT ( 'NONE',  ( -7.424026671074350129E-16, 13.45854811567263276, -53.40473080337743284 ) ) ;
#31473=DIRECTION ( 'NONE',  ( 0.000000000000000000, 1.000000000000000000, 0.000000000000000000 ) ) ;
#31475=CARTESIAN_POINT ( 'NONE',  ( 3.310556943750001313, 19.41135094264166838, -109.2682724695661278 ) ) ;
#31476=CARTESIAN_POINT ( 'NONE',  ( -7.022189441860112050E-16, 13.67729811471671653, -39.60160580289946353 ) ) ;
#31478=CARTESIAN_POINT ( 'NONE',  ( 3.500000000000001332, 19.52072594216370760, -66.07139747004409003 ) ) ;
#31481=CARTESIAN_POINT ( 'NONE',  ( 4.648177544792955347E-16, 21.00000000000001776, -89.21098080242148853 ) ) ;
#31483=CARTESIAN_POINT ( 'NONE',  ( 3.310556943750001313, 17.50000000000001776, -88.26410580289947916 ) ) ;
#31486=CARTESIAN_POINT ( 'NONE',  ( -0.9378221735089291577, 21.00000000000001421, -65.16632260368298546 ) ) ;
#31487=( BOUNDED_CURVE ( )  B_SPLINE_CURVE ( 2, ( #25480, #28858, #41220, #25055, #19086, #5695, #12063, #6106, #38444 ),
 .UNSPECIFIED., .F., .F. ) 
 B_SPLINE_CURVE_WITH_KNOTS ( ( 3, 2, 2, 2, 3 ),
 ( 0.7979166666666667185, 0.7986111111111111605, 0.8000000000000000444, 0.8013888888888889284, 0.8020833333333333703 ),
 .UNSPECIFIED. ) 
 CURVE ( )  GEOMETRIC_REPRESENTATION_ITEM ( )  RATIONAL_B_SPLINE_CURVE ( ( 0.9330127018922194093, 0.9330127018922194093, 1.000000000000000000, 0.8660254037844387076, 1.000000000000000000, 0.8660254037844387076, 1.000000000000000000, 0.9330127018922194093, 0.9330127018922194093 ) ) 
 REPRESENTATION_ITEM ( '' )  );
#31488=ORIENTED_EDGE ( 'NONE', *, *, #9770, .T. ) ;
#31492=CARTESIAN_POINT ( 'NONE',  ( -1.655278471874999990, 20.36702641396249192, -96.93077246956613635 ) ) ;
#31496=VERTEX_POINT ( 'NONE', #39278 ) ;
#31497=AXIS2_PLACEMENT_3D ( 'NONE', #36840, #34061, #30024 ) ;
#31502=ORIENTED_EDGE ( 'NONE', *, *, #23062, .T. ) ;
#31503=EDGE_CURVE ( 'NONE', #27445, #25967, #4979, .T. ) ;
#31504=CARTESIAN_POINT ( 'NONE',  ( 0.9378221735089281585, 14.00000000000001776, -91.36007260463891555 ) ) ;
#31506=CARTESIAN_POINT ( 'NONE',  ( -1.655278471874999990, 20.36702641396249902, -135.9307724695661364 ) ) ;
#31507=CARTESIAN_POINT ( 'NONE',  ( 3.500000000000000000, 15.47927405783633503, -133.5443141357548598 ) ) ;
#31508=VERTEX_POINT ( 'NONE', #1015 ) ;
#31510=CARTESIAN_POINT ( 'NONE',  ( -3.310556943750001313, 17.50000000000002132, -123.8516058028994564 ) ) ;
#31511=CARTESIAN_POINT ( 'NONE',  ( 3.310556943749999981, 15.58864905735836182, -52.43493913623280633 ) ) ;
#31512=ORIENTED_EDGE ( 'NONE', *, *, #39886, .T. ) ;
#31514=CARTESIAN_POINT ( 'NONE',  ( 2.474675557024783212E-16, 21.54145188432740810, -137.9047308033774186 ) ) ;
#31517=CARTESIAN_POINT ( 'NONE',  ( 3.310556943750001313, 19.41135094264166483, -79.26827246956612782 ) ) ;
#31518=CARTESIAN_POINT ( 'NONE',  ( 3.500000000000000000, 15.47927405783633503, -130.5443141357548313 ) ) ;
#31519=CARTESIAN_POINT ( 'NONE',  ( -3.310556943750001313, 17.50000000000002132, -108.7641058028994649 ) ) ;
#31520=FACE_OUTER_BOUND ( 'NONE', #34060, .T. ) ;
#31523=CARTESIAN_POINT ( 'NONE',  ( -1.750000000000002220, 14.46891108675448123, -79.79431413575484555 ) ) ;
#31524=CARTESIAN_POINT ( 'NONE',  ( 1.750000000000001110, 20.53108891324555785, -102.9880641367107756 ) ) ;
#31525=CARTESIAN_POINT ( 'NONE',  ( 1.655278471875001101, 20.36702641396248481, -44.09743913623280775 ) ) ;
#31526=CARTESIAN_POINT ( 'NONE',  ( -1.655278471874999990, 20.36702641396249192, -99.01827246956612782 ) ) ;
#31527=DIRECTION ( 'NONE',  ( 0.000000000000000000, 1.000000000000000000, 0.000000000000000000 ) ) ;
#31529=CARTESIAN_POINT ( 'NONE',  ( 3.500000000000001332, 19.52072594216370405, -39.37764746908817415 ) ) ;
#31531=CARTESIAN_POINT ( 'NONE',  ( 3.310556943750001313, 19.41135094264166838, -125.2682724695661136 ) ) ;
#31535=CARTESIAN_POINT ( 'NONE',  ( -1.394453263437886604E-15, 14.00000000000001421, -57.40473080337742573 ) ) ;
#31536=CARTESIAN_POINT ( 'NONE',  ( 4.286263797015737581E-16, 14.00000000000002487, -149.5231586289125687 ) ) ;
#31538=ORIENTED_EDGE ( 'NONE', *, *, #23524, .T. ) ;
#31539=CARTESIAN_POINT ( 'NONE',  ( 1.655278471875001101, 20.36702641396249192, -76.18493913623279923 ) ) ;
#31542=CARTESIAN_POINT ( 'NONE',  ( 1.749999999999998224, 14.46891108675447946, -80.32139747004410424 ) ) ;
#31545=CARTESIAN_POINT ( 'NONE',  ( -1.655278471875002211, 14.63297358603754006, -32.59743913623280775 ) ) ;
#31550=CARTESIAN_POINT ( 'NONE',  ( -7.022189441860112050E-16, 13.67729811471671653, -45.51410580289947205 ) ) ;
#31552=ORIENTED_EDGE ( 'NONE', *, *, #10501, .F. ) ;
#31554=CARTESIAN_POINT ( 'NONE',  ( -1.394453263437886604E-15, 14.00000000000001421, -73.71098080242151696 ) ) ;
#31557=CARTESIAN_POINT ( 'NONE',  ( 4.648177544792955347E-16, 21.00000000000002132, -104.9047308033774186 ) ) ;
#31559=CARTESIAN_POINT ( 'NONE',  ( -1.749999999999999778, 20.53108891324554719, -39.12764746908817415 ) ) ;
#31564=VECTOR ( 'NONE', #12701, 1000.000000000000000 ) ;
#31565=FACE_OUTER_BOUND ( 'NONE', #38775, .T. ) ;
#31567=CARTESIAN_POINT ( 'NONE',  ( 3.310556943749999981, 15.58864905735836004, -23.43493913623280633 ) ) ;
#31569=CARTESIAN_POINT ( 'NONE',  ( -7.022189441860112050E-16, 13.67729811471672718, -128.5141058028994792 ) ) ;
#31572=EDGE_CURVE ( 'NONE', #27672, #23444, #9335, .T. ) ;
#31573=DIRECTION ( 'NONE',  ( -0.000000000000000000, 1.259100132267607459E-16, -1.000000000000000000 ) ) ;
#31574=CARTESIAN_POINT ( 'NONE',  ( 1.655278471875001101, 20.36702641396249547, -117.1849391362327850 ) ) ;
#31575=EDGE_CURVE ( 'NONE', #25746, #16808, #13673, .T. ) ;
#31577=CARTESIAN_POINT ( 'NONE',  ( 1.749999999999998224, 14.46891108675447413, -39.32139747004409713 ) ) ;
#31578=CYLINDRICAL_SURFACE ( 'NONE', #21271, 3.499999999999999556 ) ;
#31580=CARTESIAN_POINT ( 'NONE',  ( -3.310556943750001313, 17.50000000000002487, -140.8516058028994564 ) ) ;
#31582=CARTESIAN_POINT ( 'NONE',  ( 3.310556943749999981, 15.58864905735836182, -47.43493913623279923 ) ) ;
#31585=CARTESIAN_POINT ( 'NONE',  ( 3.310556943750001313, 19.41135094264166483, -77.26827246956614204 ) ) ;
#31587=CARTESIAN_POINT ( 'NONE',  ( 3.310556943750001313, 19.41135094264166838, -97.18077246956613635 ) ) ;
#31588=CARTESIAN_POINT ( 'NONE',  ( 3.310556943750001313, 19.41135094264166128, -68.18077246956613635 ) ) ;
#31590=CARTESIAN_POINT ( 'NONE',  ( 2.340729813953370519E-16, 21.32270188528331190, -90.10160580289948484 ) ) ;
#31594=CARTESIAN_POINT ( 'NONE',  ( -1.394453263437886604E-15, 14.00000000000001776, -105.7109808024215027 ) ) ;
#31596=CARTESIAN_POINT ( 'NONE',  ( -1.655278471874999990, 20.36702641396248836, -49.93077246956615056 ) ) ;
#31597=CARTESIAN_POINT ( 'NONE',  ( -1.749999999999999778, 20.53108891324554719, -24.82139747004409713 ) ) ;
#31598=CARTESIAN_POINT ( 'NONE',  ( 3.310556943749999981, 15.58864905735837247, -113.3474391362328220 ) ) ;
#31599=CARTESIAN_POINT ( 'NONE',  ( -1.394453263437886604E-15, 14.00000000000001066, -35.71098080242150985 ) ) ;
#31603=AXIS2_PLACEMENT_3D ( 'NONE', #15192, #24774, #37737 ) ;
#31607=CARTESIAN_POINT ( 'NONE',  ( -3.310556943750002645, 15.58864905735836892, -61.68077246956614346 ) ) ;
#31608=ORIENTED_EDGE ( 'NONE', *, *, #7209, .T. ) ;
#31609=ORIENTED_EDGE ( 'NONE', *, *, #17358, .T. ) ;
#31610=FACE_OUTER_BOUND ( 'NONE', #7285, .T. ) ;
#31612=EDGE_CURVE ( 'NONE', #25980, #5960, #18027, .T. ) ;
#31616=CARTESIAN_POINT ( 'NONE',  ( -3.500000000000001332, 17.50000000000001421, -54.96098080242150985 ) ) ;
#31617=CARTESIAN_POINT ( 'NONE',  ( 3.310556943750001313, 17.50000000000002132, -129.2641058028994507 ) ) ;
#31618=CARTESIAN_POINT ( 'NONE',  ( 7.785697387528201340E-15, 14.00000000000002487, -136.4047308033774186 ) ) ;
#31619=( BOUNDED_CURVE ( )  B_SPLINE_CURVE ( 2, ( #19094, #15285, #15703, #41436, #5911, #18883, #22078, #41013, #24859 ),
 .UNSPECIFIED., .F., .T. ) 
 B_SPLINE_CURVE_WITH_KNOTS ( ( 3, 2, 2, 2, 3 ),
 ( 0.9520833333333332815, 0.9527777777777777235, 0.9541666666666667185, 0.9555555555555556024, 0.9562500000000000444 ),
 .UNSPECIFIED. ) 
 CURVE ( )  GEOMETRIC_REPRESENTATION_ITEM ( )  RATIONAL_B_SPLINE_CURVE ( ( 0.9330127018922194093, 0.9330127018922194093, 1.000000000000000000, 0.8660254037844387076, 1.000000000000000000, 0.8660254037844387076, 1.000000000000000000, 0.9330127018922194093, 0.9330127018922194093 ) ) 
 REPRESENTATION_ITEM ( '' )  );
#31620=CARTESIAN_POINT ( 'NONE',  ( 1.655278471874998436, 14.63297358603754006, -40.51827246956612782 ) ) ;
#31621=CARTESIAN_POINT ( 'NONE',  ( -7.022189441860112050E-16, 13.67729811471671475, -27.60160580289947063 ) ) ;
#31622=CARTESIAN_POINT ( 'NONE',  ( -3.310556943750001313, 17.50000000000001776, -91.85160580289947063 ) ) ;
#31623=CARTESIAN_POINT ( 'NONE',  ( -3.500000000000000888, 19.52072594216370405, -23.73806413671077209 ) ) ;
#31624=ORIENTED_EDGE ( 'NONE', *, *, #20376, .T. ) ;
#31626=CARTESIAN_POINT ( 'NONE',  ( -3.310556943750000425, 19.41135094264167549, -140.9349391362327708 ) ) ;
#31630=CARTESIAN_POINT ( 'NONE',  ( -3.500000000000000888, 19.52072594216371115, -79.73806413671076143 ) ) ;
#31631=CARTESIAN_POINT ( 'NONE',  ( 1.655278471874998436, 14.63297358603754184, -64.51827246956614204 ) ) ;
#31634=CARTESIAN_POINT ( 'NONE',  ( 0.000000000000000000, 17.50000000000002487, -149.5231586289125687 ) ) ;
#31635=CARTESIAN_POINT ( 'NONE',  ( -3.500000000000001332, 17.50000000000001421, -47.96098080242150274 ) ) ;
#31637=CARTESIAN_POINT ( 'NONE',  ( 1.655278471874998436, 14.63297358603754894, -113.4307724695661364 ) ) ;
#31639=EDGE_CURVE ( 'NONE', #23444, #4672, #9846, .T. ) ;
#31640=ORIENTED_EDGE ( 'NONE', *, *, #29097, .F. ) ;
#31641=CARTESIAN_POINT ( 'NONE',  ( -1.749999999999999778, 20.53108891324555785, -108.8213974700441042 ) ) ;
#31642=CARTESIAN_POINT ( 'NONE',  ( -3.500000000000000000, 19.52072594216371826, -140.0443141357548313 ) ) ;
#31643=EDGE_CURVE ( 'NONE', #35484, #41433, #2497, .T. ) ;
#31644=CARTESIAN_POINT ( 'NONE',  ( 4.648177544792955347E-16, 21.00000000000001066, -37.21098080242150985 ) ) ;
#31645=CARTESIAN_POINT ( 'NONE',  ( 3.500000000000001332, 19.52072594216370760, -65.37764746908818836 ) ) ;
#31647=CARTESIAN_POINT ( 'NONE',  ( 3.310556943749999981, 15.58864905735836714, -74.34743913623279354 ) ) ;
#31650=CARTESIAN_POINT ( 'NONE',  ( 0.9378221735089281585, 14.00000000000001599, -69.66632260368298546 ) ) ;
#31652=CARTESIAN_POINT ( 'NONE',  ( -0.9378221735089310451, 14.00000000000002309, -132.7556390011600342 ) ) ;
#31655=CARTESIAN_POINT ( 'NONE',  ( -7.022189441860112050E-16, 13.67729811471672186, -79.51410580289947916 ) ) ;
#31656=ORIENTED_EDGE ( 'NONE', *, *, #9534, .F. ) ;
#31657=ORIENTED_EDGE ( 'NONE', *, *, #3252, .F. ) ;
#31658=FACE_OUTER_BOUND ( 'NONE', #40398, .T. ) ;
#31659=ADVANCED_FACE ( 'NONE', ( #16286 ), #9055, .T. ) ;
#31663=CARTESIAN_POINT ( 'NONE',  ( -3.310556943750001313, 17.50000000000001066, -41.85160580289947063 ) ) ;
#31664=CARTESIAN_POINT ( 'NONE',  ( -1.655278471874999990, 20.36702641396249547, -111.0182724695661420 ) ) ;
#31665=ORIENTED_EDGE ( 'NONE', *, *, #29002, .T. ) ;
#31666=CARTESIAN_POINT ( 'NONE',  ( -1.655278471874999990, 20.36702641396248481, -33.93077246956615056 ) ) ;
#31667=CARTESIAN_POINT ( 'NONE',  ( 2.340729813953370519E-16, 21.32270188528330834, -60.10160580289947063 ) ) ;
#31668=CARTESIAN_POINT ( 'NONE',  ( 1.749999999999998224, 14.46891108675448301, -105.6276474690881741 ) ) ;
#31670=CARTESIAN_POINT ( 'NONE',  ( -3.310556943750000425, 19.41135094264166483, -93.84743913623279354 ) ) ;
#31671=CARTESIAN_POINT ( 'NONE',  ( -1.749999999999999778, 20.53108891324555429, -95.82139747004409003 ) ) ;
#31673=CARTESIAN_POINT ( 'NONE',  ( -1.749999999999999778, 20.53108891324555074, -56.82139747004409713 ) ) ;
#31675=CARTESIAN_POINT ( 'NONE',  ( -3.500000000000001332, 17.50000000000001421, -59.96098080242151696 ) ) ;
#31677=CARTESIAN_POINT ( 'NONE',  ( 1.655278471875001101, 20.36702641396248481, -28.09743913623280420 ) ) ;
#31678=CARTESIAN_POINT ( 'NONE',  ( 2.474675557024783212E-16, 21.54145188432739388, -50.90473080337743284 ) ) ;
#31680=CARTESIAN_POINT ( 'NONE',  ( 1.655278471875001101, 20.36702641396249547, -109.1849391362327992 ) ) ;
#31682=CARTESIAN_POINT ( 'NONE',  ( -1.655278471874999990, 20.36702641396248481, -30.01827246956613493 ) ) ;
#31689=CARTESIAN_POINT ( 'NONE',  ( 2.340729813953370519E-16, 21.32270188528331190, -90.01410580289947916 ) ) ;
#31690=ORIENTED_EDGE ( 'NONE', *, *, #18935, .F. ) ;
#31692=CARTESIAN_POINT ( 'NONE',  ( -3.500000000000002220, 15.47927405783632082, -23.87764746908817415 ) ) ;
#31695=CARTESIAN_POINT ( 'NONE',  ( 4.648177544792955347E-16, 21.00000000000001421, -74.21098080242151696 ) ) ;
#31699=CARTESIAN_POINT ( 'NONE',  ( -7.022189441860112050E-16, 13.67729811471672541, -95.51410580289947916 ) ) ;
#31708=EDGE_LOOP ( 'NONE', ( #41280, #21613, #35938, #7832 ) ) ;
#31709=CARTESIAN_POINT ( 'NONE',  ( 0.9378221735089300459, 21.00000000000002132, -108.9493890021159501 ) ) ;
#31711=CARTESIAN_POINT ( 'NONE',  ( 3.310556943750001313, 19.41135094264167549, -139.1807724695661364 ) ) ;
#31712=CARTESIAN_POINT ( 'NONE',  ( 3.500000000000001332, 17.50000000000001066, -38.15473080337743284 ) ) ;
#31715=CARTESIAN_POINT ( 'NONE',  ( -7.022189441860112050E-16, 13.67729811471672718, -122.6016058028994706 ) ) ;
#31716=CARTESIAN_POINT ( 'NONE',  ( -7.022189441860112050E-16, 13.67729811471671653, -49.60160580289946353 ) ) ;
#31718=CARTESIAN_POINT ( 'NONE',  ( 3.500000000000001776, 19.52072594216372181, -138.0713974700441042 ) ) ;
#31720=CARTESIAN_POINT ( 'NONE',  ( 1.655278471874998436, 14.63297358603754361, -78.51827246956614204 ) ) ;
#31721=CARTESIAN_POINT ( 'NONE',  ( 3.500000000000000000, 15.47927405783632970, -122.5443141357548313 ) ) ;
#31722=CARTESIAN_POINT ( 'NONE',  ( 1.655278471875001101, 20.36702641396249547, -109.0974391362328078 ) ) ;
#31723=CARTESIAN_POINT ( 'NONE',  ( -1.394453263437886604E-15, 14.00000000000001421, -72.71098080242151696 ) ) ;
#31726=CARTESIAN_POINT ( 'NONE',  ( -3.500000000000002220, 15.47927405783632793, -81.87764746908817415 ) ) ;
#31727=CARTESIAN_POINT ( 'NONE',  ( 4.648177544792955347E-16, 21.00000000000001421, -63.21098080242150274 ) ) ;
#31728=CARTESIAN_POINT ( 'NONE',  ( 3.310556943750001313, 17.50000000000001066, -40.26410580289947916 ) ) ;
#31729=CARTESIAN_POINT ( 'NONE',  ( -7.022189441860112050E-16, 13.67729811471672541, -101.6016058028994706 ) ) ;
#31730=( BOUNDED_CURVE ( )  B_SPLINE_CURVE ( 2, ( #7479, #4065, #17050, #26210, #23867, #40011, #39807, #32992, #29801 ),
 .UNSPECIFIED., .F., .F. ) 
 B_SPLINE_CURVE_WITH_KNOTS ( ( 3, 2, 2, 2, 3 ),
 ( 0.1312500000000000056, 0.1319444444444444475, 0.1333333333333333315, 0.1347222222222222154, 0.1354166666666666574 ),
 .UNSPECIFIED. ) 
 CURVE ( )  GEOMETRIC_REPRESENTATION_ITEM ( )  RATIONAL_B_SPLINE_CURVE ( ( 0.9330127018922194093, 0.9330127018922194093, 1.000000000000000000, 0.8660254037844387076, 1.000000000000000000, 0.8660254037844387076, 1.000000000000000000, 0.9330127018922194093, 0.9330127018922194093 ) ) 
 REPRESENTATION_ITEM ( '' )  );
#31734=CARTESIAN_POINT ( 'NONE',  ( -7.022189441860112050E-16, 13.67729811471672896, -121.6016058028994706 ) ) ;
#31735=CARTESIAN_POINT ( 'NONE',  ( -1.749999999999999778, 20.53108891324555429, -92.12764746908815994 ) ) ;
#31739=CARTESIAN_POINT ( 'NONE',  ( -1.394453263437886604E-15, 14.00000000000001421, -62.71098080242150274 ) ) ;
#31742=CARTESIAN_POINT ( 'NONE',  ( 3.310556943749999981, 15.58864905735836714, -75.43493913623278502 ) ) ;
#31744=CARTESIAN_POINT ( 'NONE',  ( 3.500000000000000000, 15.47927405783632082, -45.23806413671076143 ) ) ;
#31745=CARTESIAN_POINT ( 'NONE',  ( -1.749999999999999778, 20.53108891324556140, -139.8213974700441042 ) ) ;
#31747=CARTESIAN_POINT ( 'NONE',  ( 0.000000000000000000, 17.50000000000002487, -149.5231586289125687 ) ) ;
#31750=CARTESIAN_POINT ( 'NONE',  ( -7.022189441860112050E-16, 13.67729811471671653, -35.51410580289947205 ) ) ;
#31753=VERTEX_POINT ( 'NONE', #26690 ) ;
#31755=CARTESIAN_POINT ( 'NONE',  ( -1.655278471874999990, 20.36702641396248836, -49.93077246956615056 ) ) ;
#31756=VERTEX_POINT ( 'NONE', #30293 ) ;
#31761=CARTESIAN_POINT ( 'NONE',  ( -1.394453263437886604E-15, 14.00000000000001776, -104.4047308033774186 ) ) ;
#31763=CARTESIAN_POINT ( 'NONE',  ( 3.500000000000000000, 15.47927405783632082, -31.54431413575484200 ) ) ;
#31765=DIRECTION ( 'NONE',  ( 0.000000000000000000, 1.000000000000000000, 0.000000000000000000 ) ) ;
#31768=CARTESIAN_POINT ( 'NONE',  ( -3.500000000000002220, 15.47927405783633503, -140.8776474690882026 ) ) ;
#31769=CARTESIAN_POINT ( 'NONE',  ( -1.394453263437886604E-15, 14.00000000000001066, -52.71098080242150985 ) ) ;
#31770=CARTESIAN_POINT ( 'NONE',  ( 1.655278471874998436, 14.63297358603755072, -124.4307724695661364 ) ) ;
#31773=CYLINDRICAL_SURFACE ( 'NONE', #13665, 3.499999999999999556 ) ;
#31774=CARTESIAN_POINT ( 'NONE',  ( 3.500000000000000000, 15.47927405783632793, -96.54431413575484555 ) ) ;
#31775=CARTESIAN_POINT ( 'NONE',  ( -1.655278471874999990, 20.36702641396249547, -117.0182724695661278 ) ) ;
#31776=CARTESIAN_POINT ( 'NONE',  ( -1.750000000000002220, 14.46891108675448656, -121.7943141357548456 ) ) ;
#31777=CARTESIAN_POINT ( 'NONE',  ( -7.424026671074350129E-16, 13.45854811567263098, -33.40473080337742573 ) ) ;
#31778=CARTESIAN_POINT ( 'NONE',  ( 0.000000000000000000, 17.50000000000002487, -149.5231586289125687 ) ) ;
#31780=CARTESIAN_POINT ( 'NONE',  ( -3.310556943750001313, 17.50000000000002487, -136.8516058028994564 ) ) ;
#31783=ADVANCED_FACE ( 'NONE', ( #13492 ), #6903, .T. ) ;
#31784=CARTESIAN_POINT ( 'NONE',  ( -3.310556943750002201, 15.58864905735836714, -46.76827246956613493 ) ) ;
#31786=CARTESIAN_POINT ( 'NONE',  ( -0.9378221735089291577, 21.00000000000002132, -114.8600726046389155 ) ) ;
#31787=CARTESIAN_POINT ( 'NONE',  ( -3.310556943750000425, 19.41135094264166128, -71.93493913623279923 ) ) ;
#31789=CARTESIAN_POINT ( 'NONE',  ( -3.310556943750002645, 15.58864905735837070, -70.68077246956615056 ) ) ;
#31790=VERTEX_POINT ( 'NONE', #520 ) ;
#31791=CARTESIAN_POINT ( 'NONE',  ( -7.022189441860112050E-16, 13.67729811471672363, -91.60160580289947063 ) ) ;
#31794=CYLINDRICAL_SURFACE ( 'NONE', #19978, 3.499999999999999556 ) ;
#31796=CARTESIAN_POINT ( 'NONE',  ( 3.310556943750001313, 19.41135094264166483, -52.18077246956612925 ) ) ;
#31798=CARTESIAN_POINT ( 'NONE',  ( 3.310556943749999981, 15.58864905735837247, -109.3474391362328220 ) ) ;
#31803=VERTEX_POINT ( 'NONE', #23715 ) ;
#31805=CARTESIAN_POINT ( 'NONE',  ( -1.655278471875002211, 14.63297358603754361, -63.59743913623280775 ) ) ;
#31806=( BOUNDED_CURVE ( )  B_SPLINE_CURVE ( 2, ( #17195, #23788, #17614, #4838, #7616, #30156, #24413, #24212, #40774 ),
 .UNSPECIFIED., .F., .F. ) 
 B_SPLINE_CURVE_WITH_KNOTS ( ( 3, 2, 2, 2, 3 ),
 ( 0.09375000000000000000, 0.09444444444444444198, 0.09583333333333333981, 0.09722222222222222376, 0.09791666666666666574 ),
 .UNSPECIFIED. ) 
 CURVE ( )  GEOMETRIC_REPRESENTATION_ITEM ( )  RATIONAL_B_SPLINE_CURVE ( ( 0.9330127018922194093, 0.9330127018922194093, 1.000000000000000000, 0.8660254037844387076, 1.000000000000000000, 0.8660254037844387076, 1.000000000000000000, 0.9330127018922194093, 0.9330127018922194093 ) ) 
 REPRESENTATION_ITEM ( '' )  );
#31808=ORIENTED_EDGE ( 'NONE', *, *, #27687, .F. ) ;
#31810=AXIS2_PLACEMENT_3D ( 'NONE', #27273, #40236, #11105 ) ;
#31818=CARTESIAN_POINT ( 'NONE',  ( 1.655278471875001101, 20.36702641396249547, -124.0974391362328078 ) ) ;
#31820=CARTESIAN_POINT ( 'NONE',  ( 3.310556943750001313, 19.41135094264165772, -39.26827246956613493 ) ) ;
#31821=CARTESIAN_POINT ( 'NONE',  ( -3.310556943750001313, 17.50000000000001066, -28.85160580289947063 ) ) ;
#31822=CARTESIAN_POINT ( 'NONE',  ( -3.310556943750001313, 17.50000000000001776, -85.85160580289947063 ) ) ;
#31823=CARTESIAN_POINT ( 'NONE',  ( -7.022189441860112050E-16, 13.67729811471672896, -138.5141058028994792 ) ) ;
#31825=EDGE_CURVE ( 'NONE', #9388, #24979, #36247, .T. ) ;
#31828=CARTESIAN_POINT ( 'NONE',  ( -1.655278471874999990, 20.36702641396249902, -136.0182724695661420 ) ) ;
#31830=CARTESIAN_POINT ( 'NONE',  ( 4.648177544792955347E-16, 21.00000000000001421, -49.90473080337742573 ) ) ;
#31831=CARTESIAN_POINT ( 'NONE',  ( -1.394453263437886604E-15, 14.00000000000002132, -122.7109808024214885 ) ) ;
#31832=CARTESIAN_POINT ( 'NONE',  ( 7.367361408496833051E-14, 14.00000000000001776, -95.40473080337743284 ) ) ;
#31834=CARTESIAN_POINT ( 'NONE',  ( -3.500000000000002220, 15.47927405783632615, -79.57139747004410424 ) ) ;
#31836=EDGE_CURVE ( 'NONE', #15570, #3050, #6840, .T. ) ;
#31837=CARTESIAN_POINT ( 'NONE',  ( 3.310556943750001313, 17.50000000000001421, -65.35160580289945642 ) ) ;
#31839=CARTESIAN_POINT ( 'NONE',  ( -0.9378221735089268263, 14.00000000000002309, -136.7556390011600627 ) ) ;
#31840=CARTESIAN_POINT ( 'NONE',  ( 0.000000000000000000, 21.00000000000002487, -149.5231586289125687 ) ) ;
#31841=CARTESIAN_POINT ( 'NONE',  ( 1.655278471875001101, 20.36702641396249192, -87.18493913623278502 ) ) ;
#31842=CARTESIAN_POINT ( 'NONE',  ( -1.749999999999999778, 20.53108891324555074, -48.12764746908818125 ) ) ;
#31844=CARTESIAN_POINT ( 'NONE',  ( -3.310556943750001313, 17.50000000000002132, -115.7641058028994792 ) ) ;
#31848=EDGE_CURVE ( 'NONE', #3604, #15516, #32925, .T. ) ;
#31849=CARTESIAN_POINT ( 'NONE',  ( -1.750000000000002220, 14.46891108675448656, -109.4880641367107614 ) ) ;
#31851=CARTESIAN_POINT ( 'NONE',  ( -0.9378221735089291577, 21.00000000000001776, -82.86007260463891555 ) ) ;
#31853=CARTESIAN_POINT ( 'NONE',  ( 0.9378221735089281585, 14.00000000000001243, -65.66632260368298546 ) ) ;
#31855=CARTESIAN_POINT ( 'NONE',  ( -1.655278471875002211, 14.63297358603754361, -66.59743913623280775 ) ) ;
#31856=CARTESIAN_POINT ( 'NONE',  ( 1.749999999999998224, 14.46891108675447768, -59.62764746908817415 ) ) ;
#31857=CARTESIAN_POINT ( 'NONE',  ( 0.9378221735089300459, 21.00000000000001421, -70.94938900211595012 ) ) ;
#31859=ORIENTED_EDGE ( 'NONE', *, *, #10501, .T. ) ;
#31862=CARTESIAN_POINT ( 'NONE',  ( 3.310556943749999981, 15.58864905735836892, -81.34743913623280775 ) ) ;
#31863=VERTEX_POINT ( 'NONE', #33488 ) ;
#31865=( BOUNDED_CURVE ( )  B_SPLINE_CURVE ( 2, ( #30321, #29899, #986, #13954, #769, #13742, #20330, #26722, #39684 ),
 .UNSPECIFIED., .F., .T. ) 
 B_SPLINE_CURVE_WITH_KNOTS ( ( 3, 2, 2, 2, 3 ),
 ( 0.4812500000000000111, 0.4819444444444444531, 0.4833333333333333370, 0.4847222222222222210, 0.4854166666666666630 ),
 .UNSPECIFIED. ) 
 CURVE ( )  GEOMETRIC_REPRESENTATION_ITEM ( )  RATIONAL_B_SPLINE_CURVE ( ( 0.9330127018922194093, 0.9330127018922194093, 1.000000000000000000, 0.8660254037844387076, 1.000000000000000000, 0.8660254037844387076, 1.000000000000000000, 0.9330127018922194093, 0.9330127018922194093 ) ) 
 REPRESENTATION_ITEM ( '' )  );
#31866=CARTESIAN_POINT ( 'NONE',  ( 4.648177544792955347E-16, 21.00000000000001421, -53.90473080337743284 ) ) ;
#31871=CARTESIAN_POINT ( 'NONE',  ( 2.340729813953370519E-16, 21.32270188528330479, -46.10160580289946353 ) ) ;
#31872=CARTESIAN_POINT ( 'NONE',  ( -3.310556943750001313, 17.50000000000002132, -106.8516058028994564 ) ) ;
#31874=AXIS2_PLACEMENT_3D ( 'NONE', #38367, #9017, #31765 ) ;
#31875=CARTESIAN_POINT ( 'NONE',  ( -7.022189441860112050E-16, 13.67729811471671475, -27.51410580289948271 ) ) ;
#31876=CARTESIAN_POINT ( 'NONE',  ( -3.310556943750001313, 17.50000000000001421, -60.85160580289945642 ) ) ;
#31877=CARTESIAN_POINT ( 'NONE',  ( -1.750000000000002220, 14.46891108675448478, -105.7943141357548313 ) ) ;
#31879=CARTESIAN_POINT ( 'NONE',  ( 2.474675557024783212E-16, 21.54145188432739744, -97.90473080337743284 ) ) ;
#31881=FACE_OUTER_BOUND ( 'NONE', #38866, .T. ) ;
#31884=CARTESIAN_POINT ( 'NONE',  ( -3.500000000000002220, 15.47927405783632437, -56.87764746908817415 ) ) ;
#31886=CARTESIAN_POINT ( 'NONE',  ( -7.022189441860112050E-16, 13.67729811471671475, -27.51410580289948271 ) ) ;
#31887=EDGE_CURVE ( 'NONE', #25969, #19673, #37287, .T. ) ;
#31888=CARTESIAN_POINT ( 'NONE',  ( -3.500000000000001332, 17.50000000000001421, -48.65473080337742573 ) ) ;
#31889=CARTESIAN_POINT ( 'NONE',  ( 4.648177544792955347E-16, 21.00000000000001421, -56.90473080337742573 ) ) ;
#31890=CARTESIAN_POINT ( 'NONE',  ( -7.022189441860112050E-16, 13.67729811471672541, -99.60160580289947063 ) ) ;
#31891=CARTESIAN_POINT ( 'NONE',  ( 3.310556943750001313, 17.50000000000001066, -31.35160580289945997 ) ) ;
#31893=LINE ( 'NONE', #2761, #40326 ) ;
#31898=CARTESIAN_POINT ( 'NONE',  ( 1.655278471875001101, 20.36702641396249192, -83.09743913623279354 ) ) ;
#31899=CARTESIAN_POINT ( 'NONE',  ( -1.394453263437886604E-15, 14.00000000000000711, -23.40473080337742928 ) ) ;
#31901=VERTEX_POINT ( 'NONE', #37114 ) ;
#31903=CARTESIAN_POINT ( 'NONE',  ( 0.9378221735089300459, 21.00000000000001776, -80.25563900116000582 ) ) ;
#31907=CARTESIAN_POINT ( 'NONE',  ( 1.655278471875001101, 20.36702641396249192, -96.09743913623280775 ) ) ;
#31909=ORIENTED_EDGE ( 'NONE', *, *, #25952, .F. ) ;
#31911=CARTESIAN_POINT ( 'NONE',  ( 0.9378221735089302680, 14.00000000000002132, -139.6663226036829712 ) ) ;
#31917=ORIENTED_EDGE ( 'NONE', *, *, #7183, .F. ) ;
#31919=DIRECTION ( 'NONE',  ( -0.000000000000000000, 1.259100132267607459E-16, -1.000000000000000000 ) ) ;
#31920=EDGE_CURVE ( 'NONE', #18006, #35892, #40292, .T. ) ;
#31921=CARTESIAN_POINT ( 'NONE',  ( 3.310556943750001313, 17.50000000000002487, -132.2641058028994507 ) ) ;
#31924=ORIENTED_EDGE ( 'NONE', *, *, #34536, .F. ) ;
#31925=CARTESIAN_POINT ( 'NONE',  ( -1.749999999999999778, 20.53108891324556140, -141.1276474690881741 ) ) ;
#31926=CARTESIAN_POINT ( 'NONE',  ( 3.310556943750001313, 17.50000000000001421, -50.35160580289946353 ) ) ;
#31928=CARTESIAN_POINT ( 'NONE',  ( -1.750000000000002220, 14.46891108675448834, -130.4880641367107614 ) ) ;
#31931=CARTESIAN_POINT ( 'NONE',  ( -1.655278471874999990, 20.36702641396249192, -79.01827246956614204 ) ) ;
#31932=CARTESIAN_POINT ( 'NONE',  ( 3.500000000000001776, 19.52072594216371826, -124.3776474690881741 ) ) ;
#31933=CARTESIAN_POINT ( 'NONE',  ( -1.655278471875002211, 14.63297358603754894, -105.5974391362328078 ) ) ;
#31935=CARTESIAN_POINT ( 'NONE',  ( 3.500000000000001332, 19.52072594216371115, -93.07139747004409003 ) ) ;
#31938=CARTESIAN_POINT ( 'NONE',  ( -3.500000000000001332, 17.50000000000001776, -75.96098080242150274 ) ) ;
#31940=CARTESIAN_POINT ( 'NONE',  ( 3.310556943750001313, 17.50000000000001066, -43.26410580289947916 ) ) ;
#31942=CARTESIAN_POINT ( 'NONE',  ( 2.340729813953370519E-16, 21.32270188528331190, -100.1016058028994564 ) ) ;
#31943=CYLINDRICAL_SURFACE ( 'NONE', #40447, 3.499999999999999556 ) ;
#31944=CARTESIAN_POINT ( 'NONE',  ( 1.749999999999998224, 14.46891108675447768, -67.32139747004409003 ) ) ;
#31945=CYLINDRICAL_SURFACE ( 'NONE', #11696, 3.499999999999999556 ) ;
#31946=ORIENTED_EDGE ( 'NONE', *, *, #31363, .F. ) ;
#31947=CARTESIAN_POINT ( 'NONE',  ( 1.655278471875001101, 20.36702641396249547, -120.1849391362327992 ) ) ;
#31951=CYLINDRICAL_SURFACE ( 'NONE', #32309, 3.499999999999999556 ) ;
#31956=CARTESIAN_POINT ( 'NONE',  ( -3.310556943750001313, 17.50000000000001776, -77.85160580289945642 ) ) ;
#31958=CARTESIAN_POINT ( 'NONE',  ( 4.648177544792955347E-16, 21.00000000000001776, -79.90473080337741862 ) ) ;
#31962=CARTESIAN_POINT ( 'NONE',  ( 1.655278471875001101, 20.36702641396248481, -32.09743913623280775 ) ) ;
#31963=FACE_OUTER_BOUND ( 'NONE', #3650, .T. ) ;
#31966=ORIENTED_EDGE ( 'NONE', *, *, #31887, .T. ) ;
#31969=CARTESIAN_POINT ( 'NONE',  ( -1.750000000000002220, 14.46891108675447946, -57.79431413575483845 ) ) ;
#31973=CARTESIAN_POINT ( 'NONE',  ( 4.648177544792955347E-16, 21.00000000000001776, -90.21098080242150274 ) ) ;
#31975=CARTESIAN_POINT ( 'NONE',  ( -3.500000000000001332, 17.50000000000002132, -119.6547308033774328 ) ) ;
#31976=CARTESIAN_POINT ( 'NONE',  ( -3.500000000000000888, 19.52072594216371826, -119.7380641367107756 ) ) ;
#31977=CARTESIAN_POINT ( 'NONE',  ( -3.500000000000002220, 15.47927405783632082, -33.87764746908818125 ) ) ;
#31978=CARTESIAN_POINT ( 'NONE',  ( 3.500000000000001776, 19.52072594216370405, -35.37764746908818125 ) ) ;
#31979=CARTESIAN_POINT ( 'NONE',  ( 0.9378221735089300459, 21.00000000000001066, -35.25563900116002714 ) ) ;
#31980=ORIENTED_EDGE ( 'NONE', *, *, #19211, .F. ) ;
#31983=( BOUNDED_CURVE ( )  B_SPLINE_CURVE ( 2, ( #9493, #6711, #42042, #19682, #329 ),
 .UNSPECIFIED., .F., .T. ) 
 B_SPLINE_CURVE_WITH_KNOTS ( ( 3, 2, 3 ),
 ( 0.000000000000000000, 0.001388888888888888942, 0.002083333333333334605 ),
 .UNSPECIFIED. ) 
 CURVE ( )  GEOMETRIC_REPRESENTATION_ITEM ( )  RATIONAL_B_SPLINE_CURVE ( ( 1.000000000000000000, 0.8660254037844387076, 1.000000000000000000, 0.9330127018922191873, 0.9330127018922192983 ) ) 
 REPRESENTATION_ITEM ( '' )  );
#31984=CARTESIAN_POINT ( 'NONE',  ( -3.500000000000000000, 19.52072594216370760, -65.73806413671076143 ) ) ;
#31986=CARTESIAN_POINT ( 'NONE',  ( -7.424026671074350129E-16, 13.45854811567264164, -136.7109808024214885 ) ) ;
#31988=CARTESIAN_POINT ( 'NONE',  ( -1.655278471875002211, 14.63297358603755072, -122.5974391362328078 ) ) ;
#31992=AXIS2_PLACEMENT_3D ( 'NONE', #21918, #22136, #2570 ) ;
#31993=CARTESIAN_POINT ( 'NONE',  ( -1.749999999999999778, 20.53108891324555429, -91.12764746908817415 ) ) ;
#31994=CARTESIAN_POINT ( 'NONE',  ( 1.655278471875001101, 20.36702641396248836, -59.09743913623280775 ) ) ;
#31995=CARTESIAN_POINT ( 'NONE',  ( -3.310556943750002645, 15.58864905735837780, -118.7682724695661278 ) ) ;
#31997=CARTESIAN_POINT ( 'NONE',  ( 1.750000000000001110, 20.53108891324554719, -32.98806413671076854 ) ) ;
#32000=CARTESIAN_POINT ( 'NONE',  ( 3.310556943750001313, 17.50000000000002487, -141.3516058028994564 ) ) ;
#32003=CARTESIAN_POINT ( 'NONE',  ( -1.655278471875002211, 14.63297358603754184, -49.68493913623279923 ) ) ;
#32006=CARTESIAN_POINT ( 'NONE',  ( -1.655278471875002211, 14.63297358603754539, -68.68493913623279923 ) ) ;
#32008=CARTESIAN_POINT ( 'NONE',  ( -7.022189441860112050E-16, 13.67729811471672186, -69.51410580289946495 ) ) ;
#32009=EDGE_LOOP ( 'NONE', ( #4412, #21359, #22434, #40191 ) ) ;
#32010=AXIS2_PLACEMENT_3D ( 'NONE', #41996, #19019, #12211 ) ;
#32011=CARTESIAN_POINT ( 'NONE',  ( -1.655278471874999990, 20.36702641396249192, -91.01827246956612782 ) ) ;
#32013=CARTESIAN_POINT ( 'NONE',  ( 1.750000000000001110, 20.53108891324555074, -67.29431413575484555 ) ) ;
#32014=CARTESIAN_POINT ( 'NONE',  ( 0.000000000000000000, 17.50000000000002487, -149.5231586289125687 ) ) ;
#32016=CARTESIAN_POINT ( 'NONE',  ( 3.310556943750001313, 19.41135094264166483, -49.18077246956615056 ) ) ;
#32018=CARTESIAN_POINT ( 'NONE',  ( 3.310556943750001313, 19.41135094264166838, -106.1807724695661506 ) ) ;
#32020=ORIENTED_EDGE ( 'NONE', *, *, #41785, .T. ) ;
#32023=ORIENTED_EDGE ( 'NONE', *, *, #21601, .T. ) ;
#32025=CARTESIAN_POINT ( 'NONE',  ( -3.310556943750000425, 19.41135094264166128, -56.84743913623280775 ) ) ;
#32026=VERTEX_POINT ( 'NONE', #4974 ) ;
#32028=CARTESIAN_POINT ( 'NONE',  ( 1.749999999999998224, 14.46891108675447413, -30.62764746908817770 ) ) ;
#32029=CARTESIAN_POINT ( 'NONE',  ( -1.394453263437886604E-15, 14.00000000000001066, -40.40473080337743284 ) ) ;
#32031=FACE_OUTER_BOUND ( 'NONE', #35466, .T. ) ;
#32033=CARTESIAN_POINT ( 'NONE',  ( -0.9378221735089291577, 21.00000000000001421, -55.16632260368299256 ) ) ;
#32034=CARTESIAN_POINT ( 'NONE',  ( 2.340729813953370519E-16, 21.32270188528331900, -124.0141058028994792 ) ) ;
#32036=VECTOR ( 'NONE', #6727, 1000.000000000000000 ) ;
#32038=CARTESIAN_POINT ( 'NONE',  ( 1.655278471875001101, 20.36702641396248481, -33.18493913623279923 ) ) ;
#32039=CARTESIAN_POINT ( 'NONE',  ( 1.655278471875001101, 20.36702641396248481, -26.18493913623279212 ) ) ;
#32040=CARTESIAN_POINT ( 'NONE',  ( -7.022189441860112050E-16, 13.67729811471672363, -86.60160580289945642 ) ) ;
#32041=CARTESIAN_POINT ( 'NONE',  ( 3.310556943749999981, 15.58864905735837780, -137.3474391362328220 ) ) ;
#32044=CARTESIAN_POINT ( 'NONE',  ( 3.310556943750001313, 19.41135094264167549, -131.2682724695661136 ) ) ;
#32045=CARTESIAN_POINT ( 'NONE',  ( -1.394453263437886604E-15, 14.00000000000001421, -70.40473080337741862 ) ) ;
#32046=CARTESIAN_POINT ( 'NONE',  ( 4.648177544792955347E-16, 21.00000000000002132, -112.2109808024214885 ) ) ;
#32047=DIRECTION ( 'NONE',  ( 0.000000000000000000, 1.000000000000000000, 0.000000000000000000 ) ) ;
#32049=CARTESIAN_POINT ( 'NONE',  ( -3.500000000000001332, 17.50000000000001776, -81.65473080337743284 ) ) ;
#32050=CARTESIAN_POINT ( 'NONE',  ( 2.340729813953370519E-16, 21.32270188528331190, -64.10160580289945642 ) ) ;
#32052=CARTESIAN_POINT ( 'NONE',  ( -3.500000000000002220, 15.47927405783633503, -136.8776474690881741 ) ) ;
#32055=CARTESIAN_POINT ( 'NONE',  ( -3.310556943750000425, 19.41135094264166483, -86.93493913623278502 ) ) ;
#32056=CARTESIAN_POINT ( 'NONE',  ( -7.022189441860112050E-16, 13.67729811471672896, -114.5141058028994792 ) ) ;
#32059=CARTESIAN_POINT ( 'NONE',  ( -1.749999999999999778, 20.53108891324555785, -106.8213974700441042 ) ) ;
#32063=CARTESIAN_POINT ( 'NONE',  ( -1.750000000000002220, 14.46891108675448301, -82.48806413671074722 ) ) ;
#32067=CARTESIAN_POINT ( 'NONE',  ( -3.310556943750002201, 15.58864905735837070, -67.68077246956613635 ) ) ;
#32068=( BOUNDED_CURVE ( )  B_SPLINE_CURVE ( 2, ( #30396, #10628, #10414, #39967, #33597, #29967, #4457, #1269, #4021 ),
 .UNSPECIFIED., .F., .T. ) 
 B_SPLINE_CURVE_WITH_KNOTS ( ( 3, 2, 2, 2, 3 ),
 ( 0.4354166666666666741, 0.4361111111111111160, 0.4375000000000000000, 0.4388888888888888840, 0.4395833333333333259 ),
 .UNSPECIFIED. ) 
 CURVE ( )  GEOMETRIC_REPRESENTATION_ITEM ( )  RATIONAL_B_SPLINE_CURVE ( ( 0.9330127018922194093, 0.9330127018922194093, 1.000000000000000000, 0.8660254037844387076, 1.000000000000000000, 0.8660254037844387076, 1.000000000000000000, 0.9330127018922194093, 0.9330127018922194093 ) ) 
 REPRESENTATION_ITEM ( '' )  );
#32069=CARTESIAN_POINT ( 'NONE',  ( 4.286263797015737581E-16, 14.00000000000002487, -149.5231586289125687 ) ) ;
#32070=CARTESIAN_POINT ( 'NONE',  ( 3.310556943750001313, 17.50000000000002132, -119.2641058028994792 ) ) ;
#32076=CARTESIAN_POINT ( 'NONE',  ( -1.655278471874999990, 20.36702641396249192, -77.93077246956615056 ) ) ;
#32080=VECTOR ( 'NONE', #11412, 1000.000000000000000 ) ;
#32081=EDGE_CURVE ( 'NONE', #1748, #6275, #37516, .T. ) ;
#32082=AXIS2_PLACEMENT_3D ( 'NONE', #11803, #12442, #28180 ) ;
#32083=CARTESIAN_POINT ( 'NONE',  ( -3.310556943750002201, 15.58864905735837958, -141.6807724695661364 ) ) ;
#32086=DIRECTION ( 'NONE',  ( -0.000000000000000000, 1.259100132267607459E-16, -1.000000000000000000 ) ) ;
#32087=CARTESIAN_POINT ( 'NONE',  ( -3.310556943750000425, 19.41135094264165772, -45.93493913623279923 ) ) ;
#32088=CARTESIAN_POINT ( 'NONE',  ( -1.655278471874999990, 20.36702641396249547, -103.0182724695661278 ) ) ;
#32089=ORIENTED_EDGE ( 'NONE', *, *, #19931, .T. ) ;
#32090=CARTESIAN_POINT ( 'NONE',  ( -3.310556943750002645, 15.58864905735836537, -30.68077246956614346 ) ) ;
#32092=CARTESIAN_POINT ( 'NONE',  ( -3.500000000000002220, 15.47927405783632970, -107.8776474690881741 ) ) ;
#32095=CARTESIAN_POINT ( 'NONE',  ( 2.474675557024783212E-16, 21.54145188432739744, -98.90473080337743284 ) ) ;
#32096=CARTESIAN_POINT ( 'NONE',  ( 4.648177544792955347E-16, 21.00000000000001776, -82.21098080242150274 ) ) ;
#32100=CARTESIAN_POINT ( 'NONE',  ( -3.500000000000000888, 19.52072594216370760, -57.04431413575483845 ) ) ;
#32102=CARTESIAN_POINT ( 'NONE',  ( -1.655278471875002211, 14.63297358603753828, -25.59743913623280065 ) ) ;
#32105=CARTESIAN_POINT ( 'NONE',  ( 1.749999999999998224, 14.46891108675447590, -49.32139747004410424 ) ) ;
#32106=CYLINDRICAL_SURFACE ( 'NONE', #13785, 3.499999999999999556 ) ;
#32107=CARTESIAN_POINT ( 'NONE',  ( -7.022189441860112050E-16, 13.67729811471671653, -34.60160580289946353 ) ) ;
#32110=CARTESIAN_POINT ( 'NONE',  ( 4.648177544792955347E-16, 21.00000000000001421, -49.90473080337742573 ) ) ;
#32114=CARTESIAN_POINT ( 'NONE',  ( 3.310556943749999981, 15.58864905735836892, -83.34743913623279354 ) ) ;
#32115=CARTESIAN_POINT ( 'NONE',  ( -0.9378221735089291577, 21.00000000000001066, -25.86007260463891200 ) ) ;
#32118=( BOUNDED_CURVE ( )  B_SPLINE_CURVE ( 2, ( #17554, #39455, #20319, #33724, #10331, #10745, #4151, #756, #36695 ),
 .UNSPECIFIED., .F., .F. ) 
 B_SPLINE_CURVE_WITH_KNOTS ( ( 3, 2, 2, 2, 3 ),
 ( 0.3812499999999999778, 0.3819444444444444198, 0.3833333333333333592, 0.3847222222222222432, 0.3854166666666666852 ),
 .UNSPECIFIED. ) 
 CURVE ( )  GEOMETRIC_REPRESENTATION_ITEM ( )  RATIONAL_B_SPLINE_CURVE ( ( 0.9330127018922194093, 0.9330127018922194093, 1.000000000000000000, 0.8660254037844387076, 1.000000000000000000, 0.8660254037844387076, 1.000000000000000000, 0.9330127018922194093, 0.9330127018922194093 ) ) 
 REPRESENTATION_ITEM ( '' )  );
#32123=CARTESIAN_POINT ( 'NONE',  ( -3.310556943750000425, 19.41135094264166483, -94.84743913623280775 ) ) ;
#32127=ORIENTED_EDGE ( 'NONE', *, *, #24893, .F. ) ;
#32129=CARTESIAN_POINT ( 'NONE',  ( 3.500000000000001332, 17.50000000000001421, -66.46098080242150274 ) ) ;
#32132=EDGE_CURVE ( 'NONE', #19567, #8739, #6350, .T. ) ;
#32133=ORIENTED_EDGE ( 'NONE', *, *, #15304, .T. ) ;
#32134=DIRECTION ( 'NONE',  ( 0.000000000000000000, 1.000000000000000000, 0.000000000000000000 ) ) ;
#32136=EDGE_CURVE ( 'NONE', #33117, #18958, #41139, .T. ) ;
#32137=CARTESIAN_POINT ( 'NONE',  ( 3.310556943750001313, 19.41135094264167549, -131.1807724695661364 ) ) ;
#32140=VECTOR ( 'NONE', #33301, 1000.000000000000000 ) ;
#32141=CARTESIAN_POINT ( 'NONE',  ( -1.394453263437886604E-15, 14.00000000000001066, -28.71098080242150985 ) ) ;
#32142=CARTESIAN_POINT ( 'NONE',  ( -3.310556943750001313, 17.50000000000002132, -117.8516058028994706 ) ) ;
#32143=CARTESIAN_POINT ( 'NONE',  ( 3.310556943750001313, 19.41135094264166128, -50.26827246956614204 ) ) ;
#32146=CARTESIAN_POINT ( 'NONE',  ( 1.750000000000001110, 20.53108891324555785, -127.9880641367107614 ) ) ;
#32148=CARTESIAN_POINT ( 'NONE',  ( 1.655278471874998436, 14.63297358603754361, -75.51827246956612782 ) ) ;
#32149=CARTESIAN_POINT ( 'NONE',  ( 2.474675557024783212E-16, 21.54145188432740099, -123.2109808024215027 ) ) ;
#32150=CARTESIAN_POINT ( 'NONE',  ( -1.655278471874999990, 20.36702641396249547, -109.9307724695661506 ) ) ;
#32151=CARTESIAN_POINT ( 'NONE',  ( 0.000000000000000000, 17.50000000000002487, -149.5231586289125687 ) ) ;
#32154=CARTESIAN_POINT ( 'NONE',  ( 3.500000000000001332, 17.50000000000001421, -74.46098080242151696 ) ) ;
#32156=CARTESIAN_POINT ( 'NONE',  ( -3.310556943750001313, 17.50000000000001066, -41.76410580289947916 ) ) ;
#32157=CARTESIAN_POINT ( 'NONE',  ( 1.655278471874998436, 14.63297358603754716, -101.5182724695661278 ) ) ;
#32159=CARTESIAN_POINT ( 'NONE',  ( -1.749999999999999778, 20.53108891324555074, -65.82139747004409003 ) ) ;
#32162=CARTESIAN_POINT ( 'NONE',  ( 2.340729813953370519E-16, 21.32270188528331900, -117.1016058028994706 ) ) ;
#32163=CARTESIAN_POINT ( 'NONE',  ( -1.750000000000002220, 14.46891108675447590, -27.79431413575483845 ) ) ;
#32168=CARTESIAN_POINT ( 'NONE',  ( -3.500000000000001332, 17.50000000000001421, -52.65473080337743284 ) ) ;
#32172=ADVANCED_FACE ( 'NONE', ( #31963 ), #18582, .T. ) ;
#32174=CARTESIAN_POINT ( 'NONE',  ( -3.500000000000002220, 15.47927405783633326, -102.5713974700440900 ) ) ;
#32179=CARTESIAN_POINT ( 'NONE',  ( 1.655278471875001101, 20.36702641396248481, -34.09743913623280775 ) ) ;
#32180=CARTESIAN_POINT ( 'NONE',  ( 1.750000000000001110, 20.53108891324555785, -106.9880641367107614 ) ) ;
#32184=EDGE_CURVE ( 'NONE', #3345, #12339, #28082, .T. ) ;
#32185=CARTESIAN_POINT ( 'NONE',  ( 7.785697387528201340E-15, 14.00000000000002487, -138.4047308033774470 ) ) ;
#32187=CARTESIAN_POINT ( 'NONE',  ( -3.500000000000001332, 17.50000000000001066, -37.65473080337743284 ) ) ;
#32188=CARTESIAN_POINT ( 'NONE',  ( -1.749999999999999778, 20.53108891324555785, -115.1276474690881741 ) ) ;
#32191=CARTESIAN_POINT ( 'NONE',  ( 0.9378221735089300459, 21.00000000000001066, -30.94938900211594657 ) ) ;
#32192=CARTESIAN_POINT ( 'NONE',  ( 1.750000000000001110, 20.53108891324555785, -116.9880641367107614 ) ) ;
#32194=CARTESIAN_POINT ( 'NONE',  ( 3.500000000000001776, 19.52072594216370405, -34.37764746908818125 ) ) ;
#32195=CARTESIAN_POINT ( 'NONE',  ( -1.394453263437886604E-15, 14.00000000000001421, -65.71098080242150274 ) ) ;
#32196=CARTESIAN_POINT ( 'NONE',  ( 4.648177544792955347E-16, 21.00000000000001066, -44.90473080337743994 ) ) ;
#32198=CARTESIAN_POINT ( 'NONE',  ( 1.749999999999998224, 14.46891108675448301, -106.3213974700441042 ) ) ;
#32200=CARTESIAN_POINT ( 'NONE',  ( 3.500000000000001332, 17.50000000000002487, -139.4609808024214885 ) ) ;
#32201=CARTESIAN_POINT ( 'NONE',  ( 1.749999999999998224, 14.46891108675448478, -120.6276474690881741 ) ) ;
#32202=CARTESIAN_POINT ( 'NONE',  ( -7.022189441860112050E-16, 13.67729811471672718, -125.5141058028994934 ) ) ;
#32206=CARTESIAN_POINT ( 'NONE',  ( 3.500000000000001776, 19.52072594216371115, -89.37764746908818836 ) ) ;
#32207=CARTESIAN_POINT ( 'NONE',  ( 3.500000000000001332, 17.50000000000001066, -33.15473080337742573 ) ) ;
#32208=CARTESIAN_POINT ( 'NONE',  ( -1.655278471875002211, 14.63297358603754361, -56.59743913623280065 ) ) ;
#32209=CARTESIAN_POINT ( 'NONE',  ( 3.310556943750001313, 17.50000000000002132, -119.3516058028994706 ) ) ;
#32211=CARTESIAN_POINT ( 'NONE',  ( -7.424026671074350129E-16, 13.45854811567263098, -31.40473080337742218 ) ) ;
#32212=CARTESIAN_POINT ( 'NONE',  ( 3.500000000000001332, 19.52072594216371115, -92.07139747004409003 ) ) ;
#32213=VECTOR ( 'NONE', #1010, 1000.000000000000000 ) ;
#32215=CARTESIAN_POINT ( 'NONE',  ( 3.310556943750001313, 17.50000000000002487, -134.3516058028994564 ) ) ;
#32217=CARTESIAN_POINT ( 'NONE',  ( 3.310556943749999981, 15.58864905735836182, -43.43493913623279212 ) ) ;
#32219=CARTESIAN_POINT ( 'NONE',  ( 2.340729813953370519E-16, 21.32270188528330834, -67.10160580289945642 ) ) ;
#32221=CARTESIAN_POINT ( 'NONE',  ( -3.310556943750000425, 19.41135094264166128, -64.84743913623280775 ) ) ;
#32222=ORIENTED_EDGE ( 'NONE', *, *, #6640, .T. ) ;
#32223=CARTESIAN_POINT ( 'NONE',  ( -1.655278471875002211, 14.63297358603754716, -93.68493913623279923 ) ) ;
#32226=CARTESIAN_POINT ( 'NONE',  ( 0.000000000000000000, 17.50000000000002487, -149.5231586289125687 ) ) ;
#32228=CARTESIAN_POINT ( 'NONE',  ( 3.310556943750001313, 17.50000000000001421, -52.26410580289947205 ) ) ;
#32230=CARTESIAN_POINT ( 'NONE',  ( -3.310556943750001313, 17.50000000000002132, -104.7641058028994649 ) ) ;
#32234=ORIENTED_EDGE ( 'NONE', *, *, #14049, .T. ) ;
#32236=ADVANCED_FACE ( 'NONE', ( #29608 ), #26015, .T. ) ;
#32237=CARTESIAN_POINT ( 'NONE',  ( 1.655278471875001101, 20.36702641396248836, -59.09743913623280775 ) ) ;
#32238=ORIENTED_EDGE ( 'NONE', *, *, #20044, .T. ) ;
#32240=( BOUNDED_CURVE ( )  B_SPLINE_CURVE ( 2, ( #16448, #28984, #13450, #23234, #32187, #19832, #3258, #16242, #32393 ),
 .UNSPECIFIED., .F., .T. ) 
 B_SPLINE_CURVE_WITH_KNOTS ( ( 3, 2, 2, 2, 3 ),
 ( 0.8770833333333333259, 0.8777777777777777679, 0.8791666666666666519, 0.8805555555555555358, 0.8812499999999999778 ),
 .UNSPECIFIED. ) 
 CURVE ( )  GEOMETRIC_REPRESENTATION_ITEM ( )  RATIONAL_B_SPLINE_CURVE ( ( 0.9330127018922194093, 0.9330127018922194093, 1.000000000000000000, 0.8660254037844387076, 1.000000000000000000, 0.8660254037844387076, 1.000000000000000000, 0.9330127018922194093, 0.9330127018922194093 ) ) 
 REPRESENTATION_ITEM ( '' )  );
#32242=DIRECTION ( 'NONE',  ( 0.000000000000000000, 1.000000000000000000, 0.000000000000000000 ) ) ;
#32243=( BOUNDED_CURVE ( )  B_SPLINE_CURVE ( 2, ( #26457, #27307, #715, #40058, #29636, #26882, #11141, #10502, #13687 ),
 .UNSPECIFIED., .F., .F. ) 
 B_SPLINE_CURVE_WITH_KNOTS ( ( 3, 2, 2, 2, 3 ),
 ( 0.8729166666666666741, 0.8736111111111111160, 0.8750000000000000000, 0.8763888888888888840, 0.8770833333333333259 ),
 .UNSPECIFIED. ) 
 CURVE ( )  GEOMETRIC_REPRESENTATION_ITEM ( )  RATIONAL_B_SPLINE_CURVE ( ( 0.9330127018922194093, 0.9330127018922194093, 1.000000000000000000, 0.8660254037844387076, 1.000000000000000000, 0.8660254037844387076, 1.000000000000000000, 0.9330127018922194093, 0.9330127018922194093 ) ) 
 REPRESENTATION_ITEM ( '' )  );
#32245=DIRECTION ( 'NONE',  ( -0.000000000000000000, 1.259100132267607459E-16, -1.000000000000000000 ) ) ;
#32249=CARTESIAN_POINT ( 'NONE',  ( 3.310556943750001313, 17.50000000000002132, -127.2641058028994792 ) ) ;
#32250=CARTESIAN_POINT ( 'NONE',  ( -0.9378221735089310451, 14.00000000000002132, -102.7556390011600058 ) ) ;
#32252=CARTESIAN_POINT ( 'NONE',  ( 1.655278471874998436, 14.63297358603753828, -36.51827246956612782 ) ) ;
#32253=CARTESIAN_POINT ( 'NONE',  ( 1.655278471874998436, 14.63297358603753828, -28.51827246956613493 ) ) ;
#32254=CARTESIAN_POINT ( 'NONE',  ( 1.655278471874998436, 14.63297358603754539, -87.51827246956612782 ) ) ;
#32255=CARTESIAN_POINT ( 'NONE',  ( -1.655278471875002211, 14.63297358603755427, -138.5974391362327935 ) ) ;
#32257=CYLINDRICAL_SURFACE ( 'NONE', #14572, 3.499999999999999556 ) ;
#32258=CARTESIAN_POINT ( 'NONE',  ( -0.9378221735089291577, 21.00000000000001066, -34.86007260463891555 ) ) ;
#32259=CARTESIAN_POINT ( 'NONE',  ( 3.310556943750001313, 19.41135094264167549, -134.2682724695661420 ) ) ;
#32260=VECTOR ( 'NONE', #33189, 1000.000000000000000 ) ;
#32265=EDGE_CURVE ( 'NONE', #27367, #15387, #23748, .T. ) ;
#32266=CARTESIAN_POINT ( 'NONE',  ( 3.500000000000000000, 15.47927405783632437, -80.23806413671076143 ) ) ;
#32267=CARTESIAN_POINT ( 'NONE',  ( 1.655278471874998436, 14.63297358603754184, -57.51827246956612782 ) ) ;
#32270=CARTESIAN_POINT ( 'NONE',  ( -1.655278471874999990, 20.36702641396249192, -87.01827246956612782 ) ) ;
#32272=CARTESIAN_POINT ( 'NONE',  ( 2.340729813953370519E-16, 21.32270188528331900, -115.0141058028995076 ) ) ;
#32273=CARTESIAN_POINT ( 'NONE',  ( -3.310556943750000425, 19.41135094264166483, -78.84743913623282197 ) ) ;
#32276=EDGE_LOOP ( 'NONE', ( #1702, #37271, #28314, #3623 ) ) ;
#32277=CARTESIAN_POINT ( 'NONE',  ( 2.474675557024783212E-16, 21.54145188432740099, -106.9047308033774186 ) ) ;
#32282=DIRECTION ( 'NONE',  ( -0.000000000000000000, 1.259100132267607459E-16, -1.000000000000000000 ) ) ;
#32285=CARTESIAN_POINT ( 'NONE',  ( -7.022189441860112050E-16, 13.67729811471672186, -64.51410580289946495 ) ) ;
#32287=CARTESIAN_POINT ( 'NONE',  ( -3.310556943750002645, 15.58864905735837780, -123.6807724695661364 ) ) ;
#32292=CARTESIAN_POINT ( 'NONE',  ( -1.394453263437886604E-15, 14.00000000000001421, -79.40473080337740441 ) ) ;
#32293=EDGE_CURVE ( 'NONE', #24771, #11163, #23020, .T. ) ;
#32294=CARTESIAN_POINT ( 'NONE',  ( 3.310556943750001313, 19.41135094264166483, -75.18077246956613635 ) ) ;
#32296=VERTEX_POINT ( 'NONE', #30034 ) ;
#32298=CARTESIAN_POINT ( 'NONE',  ( -1.655278471874999990, 20.36702641396249902, -142.9307724695661364 ) ) ;
#32300=CARTESIAN_POINT ( 'NONE',  ( -1.750000000000002220, 14.46891108675448656, -113.4880641367107614 ) ) ;
#32301=CARTESIAN_POINT ( 'NONE',  ( -1.655278471875002211, 14.63297358603754184, -45.68493913623279923 ) ) ;
#32302=CARTESIAN_POINT ( 'NONE',  ( -1.655278471874999990, 20.36702641396249547, -106.0182724695661278 ) ) ;
#32303=CARTESIAN_POINT ( 'NONE',  ( -3.310556943750002645, 15.58864905735836537, -29.68077246956614701 ) ) ;
#32305=CARTESIAN_POINT ( 'NONE',  ( -7.424026671074350129E-16, 13.45854811567263809, -107.7109808024215027 ) ) ;
#32308=CARTESIAN_POINT ( 'NONE',  ( -7.424026671074350129E-16, 13.45854811567263631, -94.40473080337743284 ) ) ;
#32309=AXIS2_PLACEMENT_3D ( 'NONE', #18565, #37921, #2607 ) ;
#32311=( BOUNDED_CURVE ( )  B_SPLINE_CURVE ( 2, ( #41159, #34137, #4998, #17979, #30956, #14792, #27756, #22632, #22839 ),
 .UNSPECIFIED., .F., .T. ) 
 B_SPLINE_CURVE_WITH_KNOTS ( ( 3, 2, 2, 2, 3 ),
 ( 0.9479166666666666297, 0.9486111111111110716, 0.9499999999999999556, 0.9513888888888888395, 0.9520833333333332815 ),
 .UNSPECIFIED. ) 
 CURVE ( )  GEOMETRIC_REPRESENTATION_ITEM ( )  RATIONAL_B_SPLINE_CURVE ( ( 0.9330127018922194093, 0.9330127018922194093, 1.000000000000000000, 0.8660254037844387076, 1.000000000000000000, 0.8660254037844387076, 1.000000000000000000, 0.9330127018922194093, 0.9330127018922194093 ) ) 
 REPRESENTATION_ITEM ( '' )  );
#32314=CARTESIAN_POINT ( 'NONE',  ( -3.500000000000000888, 19.52072594216370760, -61.04431413575483845 ) ) ;
#32316=CARTESIAN_POINT ( 'NONE',  ( 2.340729813953370519E-16, 21.32270188528330479, -25.01410580289947561 ) ) ;
#32317=CARTESIAN_POINT ( 'NONE',  ( -7.424026671074350129E-16, 13.45854811567263276, -46.40473080337741862 ) ) ;
#32319=CARTESIAN_POINT ( 'NONE',  ( -1.655278471875002211, 14.63297358603754006, -30.68493913623279568 ) ) ;
#32322=CARTESIAN_POINT ( 'NONE',  ( -3.500000000000000000, 19.52072594216371826, -121.0443141357548598 ) ) ;
#32327=CARTESIAN_POINT ( 'NONE',  ( -3.310556943750001313, 17.50000000000001776, -79.76410580289946495 ) ) ;
#32328=DIRECTION ( 'NONE',  ( -0.000000000000000000, 1.259100132267607459E-16, -1.000000000000000000 ) ) ;
#32330=DIRECTION ( 'NONE',  ( -0.000000000000000000, 1.259100132267607459E-16, -1.000000000000000000 ) ) ;
#32331=CARTESIAN_POINT ( 'NONE',  ( 0.9378221735089300459, 21.00000000000001776, -87.25563900116003424 ) ) ;
#32332=ORIENTED_EDGE ( 'NONE', *, *, #17400, .F. ) ;
#32335=CARTESIAN_POINT ( 'NONE',  ( 3.310556943750001313, 19.41135094264166483, -90.18077246956615056 ) ) ;
#32338=ORIENTED_EDGE ( 'NONE', *, *, #9047, .T. ) ;
#32344=CARTESIAN_POINT ( 'NONE',  ( 4.648177544792955347E-16, 21.00000000000002132, -109.2109808024215170 ) ) ;
#32345=CARTESIAN_POINT ( 'NONE',  ( 0.000000000000000000, 17.50000000000002487, -149.5231586289125687 ) ) ;
#32347=CARTESIAN_POINT ( 'NONE',  ( -7.022189441860112050E-16, 13.67729811471672718, -129.5141058028994507 ) ) ;
#32348=EDGE_LOOP ( 'NONE', ( #28507, #2316, #20990, #17333 ) ) ;
#32349=CARTESIAN_POINT ( 'NONE',  ( 0.000000000000000000, 17.50000000000002487, -149.5231586289125687 ) ) ;
#32350=CARTESIAN_POINT ( 'NONE',  ( -1.655278471874999990, 20.36702641396249547, -120.0182724695661278 ) ) ;
#32351=CARTESIAN_POINT ( 'NONE',  ( -1.655278471875002211, 14.63297358603754184, -48.68493913623279923 ) ) ;
#32352=ORIENTED_EDGE ( 'NONE', *, *, #27300, .T. ) ;
#32353=CARTESIAN_POINT ( 'NONE',  ( 1.750000000000001110, 20.53108891324556140, -131.9880641367107614 ) ) ;
#32355=CARTESIAN_POINT ( 'NONE',  ( 3.310556943750001313, 17.50000000000001421, -74.35160580289947063 ) ) ;
#32356=CARTESIAN_POINT ( 'NONE',  ( 1.749999999999998224, 14.46891108675448656, -125.6276474690881599 ) ) ;
#32357=CARTESIAN_POINT ( 'NONE',  ( 3.310556943750001313, 19.41135094264166838, -105.1807724695661364 ) ) ;
#32358=DIRECTION ( 'NONE',  ( -0.000000000000000000, 1.259100132267607459E-16, -1.000000000000000000 ) ) ;
#32361=CARTESIAN_POINT ( 'NONE',  ( 3.500000000000000000, 15.47927405783632437, -74.54431413575483134 ) ) ;
#32362=CARTESIAN_POINT ( 'NONE',  ( 3.500000000000000000, 15.47927405783633503, -126.2380641367107614 ) ) ;
#32363=CARTESIAN_POINT ( 'NONE',  ( 1.655278471874998436, 14.63297358603754006, -44.43077246956614346 ) ) ;
#32364=CARTESIAN_POINT ( 'NONE',  ( 1.655278471875001101, 20.36702641396249192, -100.1849391362327992 ) ) ;
#32365=FACE_OUTER_BOUND ( 'NONE', #8695, .T. ) ;
#32366=CARTESIAN_POINT ( 'NONE',  ( -3.500000000000000888, 19.52072594216370760, -65.73806413671076143 ) ) ;
#32368=ORIENTED_EDGE ( 'NONE', *, *, #35628, .F. ) ;
#32369=CARTESIAN_POINT ( 'NONE',  ( 3.310556943750001313, 19.41135094264166838, -118.2682724695661278 ) ) ;
#32375=CARTESIAN_POINT ( 'NONE',  ( 1.655278471875001101, 20.36702641396249192, -97.09743913623280775 ) ) ;
#32378=ORIENTED_EDGE ( 'NONE', *, *, #26126, .T. ) ;
#32379=DIRECTION ( 'NONE',  ( -0.000000000000000000, 1.259100132267607459E-16, -1.000000000000000000 ) ) ;
#32381=CARTESIAN_POINT ( 'NONE',  ( -1.749999999999999778, 20.53108891324555785, -118.8213974700440900 ) ) ;
#32382=CARTESIAN_POINT ( 'NONE',  ( -3.500000000000002220, 15.47927405783633326, -105.5713974700441042 ) ) ;
#32386=CARTESIAN_POINT ( 'NONE',  ( 1.655278471874998436, 14.63297358603753828, -33.43077246956615056 ) ) ;
#32389=EDGE_LOOP ( 'NONE', ( #41029, #31552, #32234, #4027 ) ) ;
#32391=DIRECTION ( 'NONE',  ( -0.000000000000000000, 1.259100132267607459E-16, -1.000000000000000000 ) ) ;
#32393=CARTESIAN_POINT ( 'NONE',  ( -1.394453263437886604E-15, 14.00000000000001066, -37.40473080337743284 ) ) ;
#32394=CARTESIAN_POINT ( 'NONE',  ( -1.749999999999999778, 20.53108891324555429, -86.12764746908817415 ) ) ;
#32395=CARTESIAN_POINT ( 'NONE',  ( 2.474675557024783212E-16, 21.54145188432740099, -119.9047308033774470 ) ) ;
#32397=CARTESIAN_POINT ( 'NONE',  ( -1.655278471874999990, 20.36702641396249902, -134.0182724695661420 ) ) ;
#32398=CARTESIAN_POINT ( 'NONE',  ( -3.500000000000002220, 15.47927405783632082, -34.87764746908818125 ) ) ;
#32399=CARTESIAN_POINT ( 'NONE',  ( 0.000000000000000000, 17.50000000000002487, -149.5231586289125687 ) ) ;
#32401=CARTESIAN_POINT ( 'NONE',  ( -0.9378221735089291577, 21.00000000000001421, -65.86007260463890134 ) ) ;
#32403=CARTESIAN_POINT ( 'NONE',  ( 1.749999999999998224, 14.46891108675448834, -137.6276474690881741 ) ) ;
#32405=CARTESIAN_POINT ( 'NONE',  ( 3.310556943750001313, 19.41135094264165772, -38.18077246956614346 ) ) ;
#32406=CARTESIAN_POINT ( 'NONE',  ( -1.655278471874999990, 20.36702641396249547, -121.9307724695661364 ) ) ;
#32410=CARTESIAN_POINT ( 'NONE',  ( -3.500000000000002220, 15.47927405783632793, -90.87764746908817415 ) ) ;
#32411=DIRECTION ( 'NONE',  ( 0.000000000000000000, 1.000000000000000000, 0.000000000000000000 ) ) ;
#32412=CARTESIAN_POINT ( 'NONE',  ( 3.310556943750001313, 19.41135094264166128, -61.18077246956615056 ) ) ;
#32413=CARTESIAN_POINT ( 'NONE',  ( 2.340729813953370519E-16, 21.32270188528331900, -117.1016058028994564 ) ) ;
#32414=CARTESIAN_POINT ( 'NONE',  ( 1.749999999999998224, 14.46891108675447413, -31.32139747004410069 ) ) ;
#32415=CARTESIAN_POINT ( 'NONE',  ( 3.500000000000001332, 17.50000000000002487, -143.1547308033774186 ) ) ;
#32417=CARTESIAN_POINT ( 'NONE',  ( -3.310556943750001313, 17.50000000000002487, -134.8516058028994564 ) ) ;
#32422=CARTESIAN_POINT ( 'NONE',  ( 3.310556943750001313, 17.50000000000001421, -71.35160580289947063 ) ) ;
#32424=CARTESIAN_POINT ( 'NONE',  ( 2.340729813953370519E-16, 21.32270188528330834, -65.01410580289947916 ) ) ;
#32425=VERTEX_POINT ( 'NONE', #9978 ) ;
#32427=CARTESIAN_POINT ( 'NONE',  ( 1.655278471874998436, 14.63297358603754539, -86.51827246956612782 ) ) ;
#32428=EDGE_CURVE ( 'NONE', #1684, #11168, #7726, .T. ) ;
#32431=FACE_OUTER_BOUND ( 'NONE', #11776, .T. ) ;
#32432=CARTESIAN_POINT ( 'NONE',  ( -1.655278471874999990, 20.36702641396248836, -51.93077246956613635 ) ) ;
#32435=CARTESIAN_POINT ( 'NONE',  ( 3.310556943750001313, 17.50000000000002132, -103.2641058028994649 ) ) ;
#32437=ORIENTED_EDGE ( 'NONE', *, *, #12348, .F. ) ;
#32442=CARTESIAN_POINT ( 'NONE',  ( 1.655278471874998436, 14.63297358603754184, -56.43077246956614346 ) ) ;
#32446=CYLINDRICAL_SURFACE ( 'NONE', #3627, 3.499999999999999556 ) ;
#32449=ORIENTED_EDGE ( 'NONE', *, *, #32696, .F. ) ;
#32451=CARTESIAN_POINT ( 'NONE',  ( 3.310556943750001313, 19.41135094264166838, -126.1807724695661364 ) ) ;
#32454=CARTESIAN_POINT ( 'NONE',  ( -1.655278471874999990, 20.36702641396248481, -36.01827246956612782 ) ) ;
#32456=CARTESIAN_POINT ( 'NONE',  ( 1.655278471875001101, 20.36702641396248481, -27.18493913623279568 ) ) ;
#32457=CARTESIAN_POINT ( 'NONE',  ( 3.310556943750001313, 19.41135094264166483, -89.26827246956612782 ) ) ;
#32458=CARTESIAN_POINT ( 'NONE',  ( -3.310556943750002645, 15.58864905735837958, -139.6807724695661364 ) ) ;
#32461=CARTESIAN_POINT ( 'NONE',  ( 4.648177544792955347E-16, 21.00000000000001776, -75.90473080337740441 ) ) ;
#32463=CARTESIAN_POINT ( 'NONE',  ( 1.655278471875001101, 20.36702641396249902, -132.1849391362327992 ) ) ;
#32464=CARTESIAN_POINT ( 'NONE',  ( 4.648177544792955347E-16, 21.00000000000002487, -138.9047308033774186 ) ) ;
#32465=CARTESIAN_POINT ( 'NONE',  ( 3.310556943750001313, 17.50000000000001776, -92.26410580289947916 ) ) ;
#32467=CARTESIAN_POINT ( 'NONE',  ( -3.500000000000001332, 17.50000000000001776, -75.96098080242150274 ) ) ;
#32469=CARTESIAN_POINT ( 'NONE',  ( -1.750000000000002220, 14.46891108675448123, -75.48806413671076143 ) ) ;
#32471=CARTESIAN_POINT ( 'NONE',  ( -3.310556943750002201, 15.58864905735836892, -59.76827246956613493 ) ) ;
#32473=DIRECTION ( 'NONE',  ( -0.8660254037844367092, 0.000000000000000000, -0.5000000000000034417 ) ) ;
#32475=CARTESIAN_POINT ( 'NONE',  ( -1.655278471874999990, 20.36702641396249192, -85.01827246956612782 ) ) ;
#32477=CARTESIAN_POINT ( 'NONE',  ( -3.310556943750000425, 19.41135094264166838, -114.8474391362327793 ) ) ;
#32478=CARTESIAN_POINT ( 'NONE',  ( -1.655278471875002211, 14.63297358603754716, -81.59743913623280775 ) ) ;
#32481=CARTESIAN_POINT ( 'NONE',  ( 1.749999999999998224, 14.46891108675448301, -100.3213974700440900 ) ) ;
#32483=CARTESIAN_POINT ( 'NONE',  ( 1.750000000000001110, 20.53108891324555074, -71.29431413575483134 ) ) ;
#32484=CARTESIAN_POINT ( 'NONE',  ( -7.460324959392693302E-14, 21.00000000000001776, -87.90473080337741862 ) ) ;
#32486=CARTESIAN_POINT ( 'NONE',  ( 1.749999999999998224, 14.46891108675447768, -65.62764746908818836 ) ) ;
#32488=CARTESIAN_POINT ( 'NONE',  ( -7.022189441860112050E-16, 13.67729811471672186, -68.51410580289947916 ) ) ;
#32490=CARTESIAN_POINT ( 'NONE',  ( 3.310556943750001313, 19.41135094264166838, -122.1807724695661364 ) ) ;
#32492=( BOUNDED_CURVE ( )  B_SPLINE_CURVE ( 2, ( #13720, #16502, #19477, #3109, #36257, #322, #23078, #36044, #35644 ),
 .UNSPECIFIED., .F., .T. ) 
 B_SPLINE_CURVE_WITH_KNOTS ( ( 3, 2, 2, 2, 3 ),
 ( 0.5562500000000000222, 0.5569444444444444642, 0.5583333333333333481, 0.5597222222222222321, 0.5604166666666666741 ),
 .UNSPECIFIED. ) 
 CURVE ( )  GEOMETRIC_REPRESENTATION_ITEM ( )  RATIONAL_B_SPLINE_CURVE ( ( 0.9330127018922194093, 0.9330127018922194093, 1.000000000000000000, 0.8660254037844387076, 1.000000000000000000, 0.8660254037844387076, 1.000000000000000000, 0.9330127018922194093, 0.9330127018922194093 ) ) 
 REPRESENTATION_ITEM ( '' )  );
#32493=CARTESIAN_POINT ( 'NONE',  ( -0.9378221735089310451, 14.00000000000002309, -125.4493890021159643 ) ) ;
#32494=ORIENTED_EDGE ( 'NONE', *, *, #42041, .T. ) ;
#32495=CARTESIAN_POINT ( 'NONE',  ( 4.648177544792955347E-16, 21.00000000000001776, -76.21098080242148853 ) ) ;
#32497=CARTESIAN_POINT ( 'NONE',  ( -3.310556943750001313, 17.50000000000001421, -72.76410580289947916 ) ) ;
#32499=ORIENTED_EDGE ( 'NONE', *, *, #629, .T. ) ;
#32501=EDGE_CURVE ( 'NONE', #11372, #14304, #12053, .T. ) ;
#32502=CARTESIAN_POINT ( 'NONE',  ( -1.655278471875002211, 14.63297358603755427, -139.5974391362327935 ) ) ;
#32504=CARTESIAN_POINT ( 'NONE',  ( 3.500000000000001332, 19.52072594216371826, -134.3776474690881741 ) ) ;
#32505=CARTESIAN_POINT ( 'NONE',  ( 3.310556943750001313, 17.50000000000001066, -45.35160580289947063 ) ) ;
#32506=CARTESIAN_POINT ( 'NONE',  ( -3.310556943750001313, 17.50000000000002132, -102.8516058028994564 ) ) ;
#32507=CARTESIAN_POINT ( 'NONE',  ( 3.310556943750001313, 17.50000000000001066, -28.26410580289947916 ) ) ;
#32509=CARTESIAN_POINT ( 'NONE',  ( -1.749999999999999778, 20.53108891324555785, -104.1276474690881741 ) ) ;
#32511=CYLINDRICAL_SURFACE ( 'NONE', #4402, 3.499999999999999556 ) ;
#32512=CARTESIAN_POINT ( 'NONE',  ( 1.749999999999998224, 14.46891108675448123, -89.32139747004410424 ) ) ;
#32514=CARTESIAN_POINT ( 'NONE',  ( -0.9378221735089310451, 14.00000000000001599, -77.75563900116003424 ) ) ;
#32517=CARTESIAN_POINT ( 'NONE',  ( -7.424026671074350129E-16, 13.45854811567263454, -58.71098080242151696 ) ) ;
#32519=DIRECTION ( 'NONE',  ( 0.000000000000000000, 1.000000000000000000, 0.000000000000000000 ) ) ;
#32520=CARTESIAN_POINT ( 'NONE',  ( 2.474675557024783212E-16, 21.54145188432739388, -46.90473080337742573 ) ) ;
#32522=CARTESIAN_POINT ( 'NONE',  ( 3.310556943750001313, 17.50000000000001066, -33.35160580289946353 ) ) ;
#32524=CARTESIAN_POINT ( 'NONE',  ( 0.9378221735089281585, 14.00000000000001599, -75.36007260463890134 ) ) ;
#32529=CARTESIAN_POINT ( 'NONE',  ( 1.655278471874998436, 14.63297358603754539, -83.43077246956615056 ) ) ;
#32533=DIRECTION ( 'NONE',  ( -0.000000000000000000, 1.259100132267607459E-16, -1.000000000000000000 ) ) ;
#32536=CARTESIAN_POINT ( 'NONE',  ( 2.340729813953370519E-16, 21.32270188528331190, -90.01410580289947916 ) ) ;
#32537=ORIENTED_EDGE ( 'NONE', *, *, #38433, .T. ) ;
#32544=VECTOR ( 'NONE', #18717, 1000.000000000000000 ) ;
#32546=CARTESIAN_POINT ( 'NONE',  ( -1.655278471874999990, 20.36702641396249902, -129.9307724695661364 ) ) ;
#32548=VERTEX_POINT ( 'NONE', #20600 ) ;
#32549=CARTESIAN_POINT ( 'NONE',  ( 1.750000000000001110, 20.53108891324554719, -28.29431413575483845 ) ) ;
#32550=CARTESIAN_POINT ( 'NONE',  ( 3.310556943750001313, 19.41135094264166838, -120.2682724695661278 ) ) ;
#32552=CARTESIAN_POINT ( 'NONE',  ( 1.749999999999998224, 14.46891108675448656, -128.3213974700441042 ) ) ;
#32553=CARTESIAN_POINT ( 'NONE',  ( -3.310556943750001313, 17.50000000000001421, -71.85160580289947063 ) ) ;
#32554=CARTESIAN_POINT ( 'NONE',  ( 3.500000000000001776, 19.52072594216371826, -122.3776474690881741 ) ) ;
#32555=CARTESIAN_POINT ( 'NONE',  ( 3.310556943749999981, 15.58864905735837070, -104.3474391362328220 ) ) ;
#32559=CARTESIAN_POINT ( 'NONE',  ( -1.750000000000002220, 14.46891108675448123, -73.79431413575483134 ) ) ;
#32562=CARTESIAN_POINT ( 'NONE',  ( 3.310556943749999981, 15.58864905735836182, -37.34743913623281486 ) ) ;
#32563=CARTESIAN_POINT ( 'NONE',  ( -1.655278471874999990, 20.36702641396249192, -96.01827246956612782 ) ) ;
#32564=CARTESIAN_POINT ( 'NONE',  ( 3.500000000000001776, 19.52072594216370760, -64.07139747004410424 ) ) ;
#32566=CARTESIAN_POINT ( 'NONE',  ( 2.340729813953370519E-16, 21.32270188528331900, -120.1016058028994706 ) ) ;
#32567=FACE_OUTER_BOUND ( 'NONE', #11935, .T. ) ;
#32572=CARTESIAN_POINT ( 'NONE',  ( 2.340729813953370519E-16, 21.32270188528331190, -98.01410580289947916 ) ) ;
#32573=DIRECTION ( 'NONE',  ( -0.000000000000000000, 1.259100132267607459E-16, -1.000000000000000000 ) ) ;
#32576=CARTESIAN_POINT ( 'NONE',  ( 0.000000000000000000, 17.50000000000002487, -149.5231586289125687 ) ) ;
#32577=AXIS2_PLACEMENT_3D ( 'NONE', #5275, #18249, #15065 ) ;
#32578=EDGE_CURVE ( 'NONE', #6557, #37632, #36547, .T. ) ;
#32579=CARTESIAN_POINT ( 'NONE',  ( 4.286263797015738567E-16, 14.00000000000002665, -143.4609808024215170 ) ) ;
#32580=FACE_OUTER_BOUND ( 'NONE', #14658, .T. ) ;
#32582=CARTESIAN_POINT ( 'NONE',  ( -3.500000000000000000, 19.52072594216371826, -135.0443141357548598 ) ) ;
#32585=CARTESIAN_POINT ( 'NONE',  ( -3.310556943750001313, 17.50000000000001066, -26.76410580289947916 ) ) ;
#32586=ORIENTED_EDGE ( 'NONE', *, *, #9203, .T. ) ;
#32592=AXIS2_PLACEMENT_3D ( 'NONE', #22284, #32282, #35256 ) ;
#32594=CARTESIAN_POINT ( 'NONE',  ( -0.9378221735089640188, 20.99999999999999645, -86.16632260368299967 ) ) ;
#32596=CARTESIAN_POINT ( 'NONE',  ( -3.500000000000001332, 17.50000000000002132, -120.6547308033774328 ) ) ;
#32598=CARTESIAN_POINT ( 'NONE',  ( 2.340729813953370519E-16, 21.32270188528332255, -133.1016058028994564 ) ) ;
#32599=CARTESIAN_POINT ( 'NONE',  ( 2.474675557024783212E-16, 21.54145188432739033, -33.21098080242150274 ) ) ;
#32602=CARTESIAN_POINT ( 'NONE',  ( 0.000000000000000000, 21.00000000000002487, -149.5231586289125687 ) ) ;
#32603=AXIS2_PLACEMENT_3D ( 'NONE', #25553, #12624, #35374 ) ;
#32605=CARTESIAN_POINT ( 'NONE',  ( 3.500000000000001332, 19.52072594216371826, -118.3776474690881741 ) ) ;
#32607=CARTESIAN_POINT ( 'NONE',  ( -3.500000000000002220, 15.47927405783633503, -137.8776474690881741 ) ) ;
#32608=CARTESIAN_POINT ( 'NONE',  ( 3.310556943749999981, 15.58864905735837425, -123.3474391362327935 ) ) ;
#32612=CARTESIAN_POINT ( 'NONE',  ( -3.500000000000000888, 19.52072594216371115, -92.04431413575484555 ) ) ;
#32613=CARTESIAN_POINT ( 'NONE',  ( -7.022189441860112050E-16, 13.67729811471671830, -60.51410580289947205 ) ) ;
#32614=CARTESIAN_POINT ( 'NONE',  ( -7.022189441860112050E-16, 13.67729811471672718, -114.6016058028994564 ) ) ;
#32616=CARTESIAN_POINT ( 'NONE',  ( 3.500000000000001776, 19.52072594216370405, -31.07139747004410424 ) ) ;
#32619=CARTESIAN_POINT ( 'NONE',  ( 3.310556943750001313, 17.50000000000002487, -132.3516058028994564 ) ) ;
#32623=CARTESIAN_POINT ( 'NONE',  ( -7.022189441860112050E-16, 13.67729811471672186, -69.60160580289947063 ) ) ;
#32624=ADVANCED_FACE ( 'NONE', ( #40374 ), #11235, .T. ) ;
#32627=CARTESIAN_POINT ( 'NONE',  ( -7.022189441860112050E-16, 13.67729811471671830, -64.51410580289946495 ) ) ;
#32628=ORIENTED_EDGE ( 'NONE', *, *, #38296, .F. ) ;
#32629=CARTESIAN_POINT ( 'NONE',  ( 3.310556943750001313, 17.50000000000001776, -86.35160580289947063 ) ) ;
#32630=EDGE_CURVE ( 'NONE', #38091, #36251, #30164, .T. ) ;
#32632=CARTESIAN_POINT ( 'NONE',  ( -0.9378221735089291577, 21.00000000000002132, -103.8600726046389155 ) ) ;
#32634=CARTESIAN_POINT ( 'NONE',  ( 3.310556943750001313, 17.50000000000001066, -46.26410580289947205 ) ) ;
#32636=CARTESIAN_POINT ( 'NONE',  ( -7.022189441860112050E-16, 13.67729811471672541, -107.5141058028994507 ) ) ;
#32641=VERTEX_POINT ( 'NONE', #20178 ) ;
#32643=CARTESIAN_POINT ( 'NONE',  ( -3.310556943750002645, 15.58864905735836892, -55.68077246956614346 ) ) ;
#32644=ORIENTED_EDGE ( 'NONE', *, *, #22900, .F. ) ;
#32645=ORIENTED_EDGE ( 'NONE', *, *, #3045, .F. ) ;
#32647=CARTESIAN_POINT ( 'NONE',  ( -1.394453263437886604E-15, 14.00000000000001066, -31.71098080242150985 ) ) ;
#32651=ADVANCED_FACE ( 'NONE', ( #16987 ), #4438, .T. ) ;
#32652=CARTESIAN_POINT ( 'NONE',  ( -3.500000000000002220, 15.47927405783633503, -138.8776474690881741 ) ) ;
#32653=CARTESIAN_POINT ( 'NONE',  ( 3.310556943749999981, 15.58864905735837425, -126.3474391362328078 ) ) ;
#32655=CARTESIAN_POINT ( 'NONE',  ( 0.9378221735089281585, 14.00000000000002309, -125.6663226036829855 ) ) ;
#32658=CARTESIAN_POINT ( 'NONE',  ( -7.022189441860112050E-16, 13.67729811471671475, -34.60160580289946353 ) ) ;
#32660=CARTESIAN_POINT ( 'NONE',  ( -3.310556943750000425, 19.41135094264166483, -88.93493913623281344 ) ) ;
#32661=CARTESIAN_POINT ( 'NONE',  ( 2.340729813953370519E-16, 21.32270188528332255, -141.0141058028994792 ) ) ;
#32663=CARTESIAN_POINT ( 'NONE',  ( -0.9378221735089310451, 14.00000000000001599, -66.75563900116002003 ) ) ;
#32666=CARTESIAN_POINT ( 'NONE',  ( -7.022189441860112050E-16, 13.67729811471672718, -126.6016058028994848 ) ) ;
#32667=CARTESIAN_POINT ( 'NONE',  ( 0.9378221735089281585, 14.00000000000001243, -56.66632260368299256 ) ) ;
#32668=CARTESIAN_POINT ( 'NONE',  ( 3.310556943749999981, 15.58864905735836892, -92.34743913623282197 ) ) ;
#32670=DIRECTION ( 'NONE',  ( -0.000000000000000000, 1.259100132267607459E-16, -1.000000000000000000 ) ) ;
#32672=CARTESIAN_POINT ( 'NONE',  ( 1.749999999999998224, 14.46891108675447946, -76.32139747004410424 ) ) ;
#32673=CARTESIAN_POINT ( 'NONE',  ( 3.310556943750001313, 19.41135094264166483, -61.26827246956613493 ) ) ;
#32677=LINE ( 'NONE', #3538, #20003 ) ;
#32678=CARTESIAN_POINT ( 'NONE',  ( 3.310556943750001313, 19.41135094264166483, -87.26827246956612782 ) ) ;
#32681=CARTESIAN_POINT ( 'NONE',  ( -7.022189441860112050E-16, 13.67729811471672541, -106.5141058028994649 ) ) ;
#32682=CARTESIAN_POINT ( 'NONE',  ( -3.310556943750001313, 17.50000000000001776, -80.76410580289946495 ) ) ;
#32685=CARTESIAN_POINT ( 'NONE',  ( 2.340729813953370519E-16, 21.32270188528331190, -101.1016058028994706 ) ) ;
#32686=CARTESIAN_POINT ( 'NONE',  ( -3.500000000000000888, 19.52072594216371826, -102.7380641367107756 ) ) ;
#32689=CARTESIAN_POINT ( 'NONE',  ( 1.749999999999998224, 14.46891108675448301, -105.3213974700441042 ) ) ;
#32690=CARTESIAN_POINT ( 'NONE',  ( 1.750000000000001110, 20.53108891324555074, -53.98806413671076854 ) ) ;
#32692=CARTESIAN_POINT ( 'NONE',  ( 1.655278471874998436, 14.63297358603754184, -64.43077246956615056 ) ) ;
#32694=CARTESIAN_POINT ( 'NONE',  ( 1.655278471874998436, 14.63297358603755072, -123.4307724695661506 ) ) ;
#32695=DIRECTION ( 'NONE',  ( -0.000000000000000000, 1.259100132267607459E-16, -1.000000000000000000 ) ) ;
#32696=EDGE_CURVE ( 'NONE', #22103, #3604, #36984, .T. ) ;
#32698=EDGE_LOOP ( 'NONE', ( #32644, #26387, #12284, #15946 ) ) ;
#32701=CARTESIAN_POINT ( 'NONE',  ( -3.500000000000000000, 19.52072594216371115, -90.04431413575483134 ) ) ;
#32702=CARTESIAN_POINT ( 'NONE',  ( -3.310556943750002645, 15.58864905735837070, -71.68077246956613635 ) ) ;
#32707=ADVANCED_FACE ( 'NONE', ( #4643 ), #33991, .T. ) ;
#32708=CARTESIAN_POINT ( 'NONE',  ( 3.310556943750001313, 17.50000000000002487, -143.2641058028994792 ) ) ;
#32710=CARTESIAN_POINT ( 'NONE',  ( 4.648177544792955347E-16, 21.00000000000002487, -134.2109808024215170 ) ) ;
#32711=CARTESIAN_POINT ( 'NONE',  ( -3.310556943750001313, 17.50000000000001066, -36.85160580289946353 ) ) ;
#32712=CARTESIAN_POINT ( 'NONE',  ( -7.022189441860112050E-16, 13.67729811471672541, -102.6016058028994706 ) ) ;
#32713=CARTESIAN_POINT ( 'NONE',  ( -1.655278471874999990, 20.36702641396248481, -26.93077246956613990 ) ) ;
#32715=CARTESIAN_POINT ( 'NONE',  ( -3.500000000000001332, 17.50000000000001776, -100.9609808024215170 ) ) ;
#32717=CARTESIAN_POINT ( 'NONE',  ( 4.286263797015737581E-16, 14.00000000000002487, -149.5231586289125687 ) ) ;
#32718=CARTESIAN_POINT ( 'NONE',  ( -3.500000000000000888, 19.52072594216371115, -93.73806413671076143 ) ) ;
#32722=CARTESIAN_POINT ( 'NONE',  ( 3.500000000000001332, 17.50000000000001421, -56.46098080242150985 ) ) ;
#32724=DIRECTION ( 'NONE',  ( -0.000000000000000000, 1.259100132267607459E-16, -1.000000000000000000 ) ) ;
#32726=CARTESIAN_POINT ( 'NONE',  ( 1.750000000000001110, 20.53108891324554719, -40.98806413671076143 ) ) ;
#32727=CARTESIAN_POINT ( 'NONE',  ( -1.394453263437886604E-15, 14.00000000000001776, -106.7109808024215027 ) ) ;
#32728=CARTESIAN_POINT ( 'NONE',  ( 3.310556943749999981, 15.58864905735836182, -27.43493913623279212 ) ) ;
#32731=CARTESIAN_POINT ( 'NONE',  ( -1.394453263437886604E-15, 14.00000000000001421, -60.40473080337743284 ) ) ;
#32733=CARTESIAN_POINT ( 'NONE',  ( 3.500000000000001332, 17.50000000000002132, -102.1547308033774186 ) ) ;
#32735=CARTESIAN_POINT ( 'NONE',  ( -1.655278471874999990, 20.36702641396249192, -80.93077246956615056 ) ) ;
#32737=ORIENTED_EDGE ( 'NONE', *, *, #26427, .T. ) ;
#32738=CARTESIAN_POINT ( 'NONE',  ( 4.648177544792955347E-16, 21.00000000000001066, -35.90473080337743284 ) ) ;
#32739=CARTESIAN_POINT ( 'NONE',  ( 3.500000000000000000, 15.47927405783632615, -80.54431413575484555 ) ) ;
#32742=CARTESIAN_POINT ( 'NONE',  ( -3.310556943750001313, 17.50000000000001776, -91.76410580289947916 ) ) ;
#32743=AXIS2_PLACEMENT_3D ( 'NONE', #6792, #36786, #30187 ) ;
#32744=ORIENTED_EDGE ( 'NONE', *, *, #3457, .F. ) ;
#32745=ORIENTED_EDGE ( 'NONE', *, *, #41968, .T. ) ;
#32747=EDGE_CURVE ( 'NONE', #25797, #12462, #35419, .T. ) ;
#32750=CARTESIAN_POINT ( 'NONE',  ( 2.340729813953370519E-16, 21.32270188528331900, -129.0141058028994507 ) ) ;
#32753=CARTESIAN_POINT ( 'NONE',  ( 3.500000000000000000, 15.47927405783632437, -64.23806413671076143 ) ) ;
#32754=CARTESIAN_POINT ( 'NONE',  ( -3.310556943750002645, 15.58864905735837780, -120.7682724695661420 ) ) ;
#32755=EDGE_LOOP ( 'NONE', ( #25487, #4828, #24410, #4825 ) ) ;
#32756=ORIENTED_EDGE ( 'NONE', *, *, #33525, .F. ) ;
#32757=CARTESIAN_POINT ( 'NONE',  ( -3.500000000000000888, 19.52072594216372181, -132.7380641367107899 ) ) ;
#32759=CARTESIAN_POINT ( 'NONE',  ( -3.310556943750000425, 19.41135094264166128, -71.93493913623279923 ) ) ;
#32760=CARTESIAN_POINT ( 'NONE',  ( -1.750000000000002220, 14.46891108675448656, -116.7943141357548313 ) ) ;
#32761=CARTESIAN_POINT ( 'NONE',  ( 1.655278471875001101, 20.36702641396249192, -100.0974391362328078 ) ) ;
#32764=CARTESIAN_POINT ( 'NONE',  ( 0.000000000000000000, 17.50000000000002487, -149.5231586289125687 ) ) ;
#32765=AXIS2_PLACEMENT_3D ( 'NONE', #35015, #28415, #5453 ) ;
#32768=CARTESIAN_POINT ( 'NONE',  ( 3.500000000000001776, 19.52072594216370760, -70.37764746908817415 ) ) ;
#32770=CARTESIAN_POINT ( 'NONE',  ( 3.310556943749999981, 15.58864905735836182, -36.34743913623281486 ) ) ;
#32771=CARTESIAN_POINT ( 'NONE',  ( 1.655278471875001101, 20.36702641396249192, -98.18493913623279923 ) ) ;
#32772=CARTESIAN_POINT ( 'NONE',  ( -3.500000000000001332, 17.50000000000001421, -60.65473080337742573 ) ) ;
#32774=CARTESIAN_POINT ( 'NONE',  ( -1.655278471875002211, 14.63297358603755072, -115.6849391362327850 ) ) ;
#32779=CARTESIAN_POINT ( 'NONE',  ( 1.750000000000001110, 20.53108891324555429, -79.29431413575484555 ) ) ;
#32780=CARTESIAN_POINT ( 'NONE',  ( 2.340729813953370519E-16, 21.32270188528331190, -96.01410580289946495 ) ) ;
#32783=CARTESIAN_POINT ( 'NONE',  ( 1.743066579297357930E-14, 14.00000000000002132, -134.7109808024214885 ) ) ;
#32784=CARTESIAN_POINT ( 'NONE',  ( -3.500000000000000000, 19.52072594216371826, -118.7380641367107614 ) ) ;
#32785=CARTESIAN_POINT ( 'NONE',  ( -1.749999999999999778, 20.53108891324555785, -105.8213974700441042 ) ) ;
#32786=ORIENTED_EDGE ( 'NONE', *, *, #38624, .T. ) ;
#32790=CARTESIAN_POINT ( 'NONE',  ( 3.310556943750001313, 19.41135094264166128, -27.18077246956614346 ) ) ;
#32791=ORIENTED_EDGE ( 'NONE', *, *, #25346, .T. ) ;
#32792=CARTESIAN_POINT ( 'NONE',  ( -1.749999999999999778, 20.53108891324555785, -123.8213974700440900 ) ) ;
#32796=CARTESIAN_POINT ( 'NONE',  ( -1.394453263437886604E-15, 14.00000000000001421, -57.71098080242150274 ) ) ;
#32798=VERTEX_POINT ( 'NONE', #21222 ) ;
#32799=CARTESIAN_POINT ( 'NONE',  ( 3.310556943750001313, 17.50000000000002487, -143.3078558028994394 ) ) ;
#32801=EDGE_CURVE ( 'NONE', #13507, #37791, #37803, .T. ) ;
#32803=CARTESIAN_POINT ( 'NONE',  ( 2.474675557024783212E-16, 21.54145188432740099, -117.9047308033774186 ) ) ;
#32805=CARTESIAN_POINT ( 'NONE',  ( 3.310556943749999981, 15.58864905735837425, -134.4349391362327992 ) ) ;
#32806=CARTESIAN_POINT ( 'NONE',  ( 1.749999999999998224, 14.46891108675447235, -25.62764746908817415 ) ) ;
#32808=CARTESIAN_POINT ( 'NONE',  ( 0.9378221735089300459, 21.00000000000001066, -32.25563900116002714 ) ) ;
#32809=CARTESIAN_POINT ( 'NONE',  ( 4.648177544792955347E-16, 21.00000000000001066, -41.21098080242150274 ) ) ;
#32811=CARTESIAN_POINT ( 'NONE',  ( 1.749999999999998224, 14.46891108675448656, -131.6276474690881741 ) ) ;
#32812=CARTESIAN_POINT ( 'NONE',  ( -1.655278471875002211, 14.63297358603755072, -118.5974391362328078 ) ) ;
#32817=CARTESIAN_POINT ( 'NONE',  ( -1.750000000000002220, 14.46891108675448301, -92.79431413575484555 ) ) ;
#32818=CARTESIAN_POINT ( 'NONE',  ( -1.749999999999999778, 20.53108891324554719, -41.12764746908817415 ) ) ;
#32819=CARTESIAN_POINT ( 'NONE',  ( -7.022189441860112050E-16, 13.67729811471671830, -55.51410580289947916 ) ) ;
#32820=CARTESIAN_POINT ( 'NONE',  ( -1.655278471875002211, 14.63297358603755072, -114.6849391362327850 ) ) ;
#32822=CARTESIAN_POINT ( 'NONE',  ( -3.500000000000000888, 19.52072594216370405, -27.73806413671076143 ) ) ;
#32824=CARTESIAN_POINT ( 'NONE',  ( 4.648177544792955347E-16, 21.00000000000002132, -108.9047308033774328 ) ) ;
#32826=CARTESIAN_POINT ( 'NONE',  ( -1.655278471875002211, 14.63297358603755249, -131.6849391362327992 ) ) ;
#32830=CARTESIAN_POINT ( 'NONE',  ( 3.310556943749999981, 15.58864905735836537, -62.43493913623279923 ) ) ;
#32832=CARTESIAN_POINT ( 'NONE',  ( 3.310556943750001313, 17.50000000000001421, -67.26410580289947916 ) ) ;
#32834=CARTESIAN_POINT ( 'NONE',  ( 2.340729813953370519E-16, 21.32270188528331190, -84.10160580289947063 ) ) ;
#32839=CARTESIAN_POINT ( 'NONE',  ( -1.655278471875002211, 14.63297358603754184, -44.59743913623280775 ) ) ;
#32842=CARTESIAN_POINT ( 'NONE',  ( -3.310556943750002645, 15.58864905735837425, -98.68077246956613635 ) ) ;
#32844=( BOUNDED_CURVE ( )  B_SPLINE_CURVE ( 2, ( #17967, #12204, #18595, #21572, #27551, #31145, #24778, #37741, #24356 ),
 .UNSPECIFIED., .F., .F. ) 
 B_SPLINE_CURVE_WITH_KNOTS ( ( 3, 2, 2, 2, 3 ),
 ( 0.4479166666666666852, 0.4486111111111111271, 0.4500000000000000111, 0.4513888888888888951, 0.4520833333333333370 ),
 .UNSPECIFIED. ) 
 CURVE ( )  GEOMETRIC_REPRESENTATION_ITEM ( )  RATIONAL_B_SPLINE_CURVE ( ( 0.9330127018922194093, 0.9330127018922194093, 1.000000000000000000, 0.8660254037844387076, 1.000000000000000000, 0.8660254037844387076, 1.000000000000000000, 0.9330127018922194093, 0.9330127018922194093 ) ) 
 REPRESENTATION_ITEM ( '' )  );
#32850=CARTESIAN_POINT ( 'NONE',  ( -3.310556943750001313, 17.50000000000001421, -56.76410580289947916 ) ) ;
#32852=VERTEX_POINT ( 'NONE', #28018 ) ;
#32860=EDGE_LOOP ( 'NONE', ( #686, #6703, #29131, #6805 ) ) ;
#32861=CARTESIAN_POINT ( 'NONE',  ( -1.749999999999999778, 20.53108891324554719, -43.12764746908817415 ) ) ;
#32862=CARTESIAN_POINT ( 'NONE',  ( -1.655278471875002211, 14.63297358603754184, -43.59743913623280775 ) ) ;
#32866=CARTESIAN_POINT ( 'NONE',  ( -0.9378221735089291577, 21.00000000000002132, -117.8600726046389013 ) ) ;
#32869=CARTESIAN_POINT ( 'NONE',  ( 1.655278471874998436, 14.63297358603753828, -33.51827246956613493 ) ) ;
#32871=CARTESIAN_POINT ( 'NONE',  ( -1.655278471874999990, 20.36702641396249192, -84.01827246956614204 ) ) ;
#32872=CARTESIAN_POINT ( 'NONE',  ( 3.310556943750001313, 19.41135094264167549, -135.1807724695661364 ) ) ;
#32875=CARTESIAN_POINT ( 'NONE',  ( 1.749999999999998224, 14.46891108675448478, -114.3213974700440900 ) ) ;
#32876=CARTESIAN_POINT ( 'NONE',  ( -1.655278471875002211, 14.63297358603755249, -129.6849391362327992 ) ) ;
#32877=CYLINDRICAL_SURFACE ( 'NONE', #6463, 3.499999999999999556 ) ;
#32878=CARTESIAN_POINT ( 'NONE',  ( 1.655278471875001101, 20.36702641396249192, -89.09743913623280775 ) ) ;
#32879=LINE ( 'NONE', #39898, #32140 ) ;
#32880=LINE ( 'NONE', #41851, #11659 ) ;
#32881=CYLINDRICAL_SURFACE ( 'NONE', #14604, 3.499999999999999556 ) ;
#32882=CARTESIAN_POINT ( 'NONE',  ( 3.500000000000001332, 17.50000000000001421, -74.15473080337743284 ) ) ;
#32883=CARTESIAN_POINT ( 'NONE',  ( -3.310556943750001313, 17.50000000000001421, -60.85160580289945642 ) ) ;
#32888=CARTESIAN_POINT ( 'NONE',  ( -7.022189441860112050E-16, 13.67729811471672363, -82.60160580289945642 ) ) ;
#32891=CARTESIAN_POINT ( 'NONE',  ( 3.310556943750001313, 17.50000000000002132, -108.2641058028994649 ) ) ;
#32892=CARTESIAN_POINT ( 'NONE',  ( 3.310556943749999981, 15.58864905735836714, -78.34743913623280775 ) ) ;
#32893=VERTEX_POINT ( 'NONE', #5053 ) ;
#32894=CARTESIAN_POINT ( 'NONE',  ( 3.310556943750001313, 17.50000000000001776, -100.3516058028994706 ) ) ;
#32895=CARTESIAN_POINT ( 'NONE',  ( 2.474675557024783212E-16, 21.54145188432740099, -104.9047308033774328 ) ) ;
#32898=CARTESIAN_POINT ( 'NONE',  ( 4.648177544792955347E-16, 21.00000000000002132, -120.9047308033774328 ) ) ;
#32899=FACE_OUTER_BOUND ( 'NONE', #22765, .T. ) ;
#32902=CARTESIAN_POINT ( 'NONE',  ( 1.655278471874998436, 14.63297358603754184, -58.43077246956614346 ) ) ;
#32904=CARTESIAN_POINT ( 'NONE',  ( 3.310556943750001313, 17.50000000000002132, -122.2641058028994792 ) ) ;
#32908=ORIENTED_EDGE ( 'NONE', *, *, #18391, .T. ) ;
#32912=CARTESIAN_POINT ( 'NONE',  ( 0.9378221735089300459, 21.00000000000001776, -78.94938900211593591 ) ) ;
#32913=CARTESIAN_POINT ( 'NONE',  ( -1.655278471875002211, 14.63297358603754539, -72.59743913623280775 ) ) ;
#32914=EDGE_LOOP ( 'NONE', ( #27024, #18560, #41753, #24451 ) ) ;
#32918=CARTESIAN_POINT ( 'NONE',  ( 1.655278471875001101, 20.36702641396249902, -139.0974391362327935 ) ) ;
#32920=CARTESIAN_POINT ( 'NONE',  ( 0.000000000000000000, 21.00000000000002487, -149.5231586289125687 ) ) ;
#32921=AXIS2_PLACEMENT_3D ( 'NONE', #4053, #36165, #3632 ) ;
#32922=CARTESIAN_POINT ( 'NONE',  ( 3.500000000000001332, 17.50000000000001066, -41.15473080337743284 ) ) ;
#32923=CARTESIAN_POINT ( 'NONE',  ( -1.655278471874999990, 20.36702641396248481, -40.01827246956612782 ) ) ;
#32924=CARTESIAN_POINT ( 'NONE',  ( -3.310556943750001313, 17.50000000000002132, -103.8516058028994564 ) ) ;
#32925=( BOUNDED_CURVE ( )  B_SPLINE_CURVE ( 2, ( #39223, #4133, #17118, #7542, #30083, #26901, #39868, #23069, #10729 ),
 .UNSPECIFIED., .F., .F. ) 
 B_SPLINE_CURVE_WITH_KNOTS ( ( 3, 2, 2, 2, 3 ),
 ( 0.8395833333333333481, 0.8402777777777777901, 0.8416666666666666741, 0.8430555555555555580, 0.8437500000000000000 ),
 .UNSPECIFIED. ) 
 CURVE ( )  GEOMETRIC_REPRESENTATION_ITEM ( )  RATIONAL_B_SPLINE_CURVE ( ( 0.9330127018922194093, 0.9330127018922194093, 1.000000000000000000, 0.8660254037844387076, 1.000000000000000000, 0.8660254037844387076, 1.000000000000000000, 0.9330127018922194093, 0.9330127018922194093 ) ) 
 REPRESENTATION_ITEM ( '' )  );
#32929=CARTESIAN_POINT ( 'NONE',  ( 1.655278471874998436, 14.63297358603755249, -142.5182724695661420 ) ) ;
#32930=CARTESIAN_POINT ( 'NONE',  ( 1.750000000000001110, 20.53108891324555429, -100.2943141357548456 ) ) ;
#32932=EDGE_CURVE ( 'NONE', #16808, #19667, #39772, .T. ) ;
#32933=CARTESIAN_POINT ( 'NONE',  ( -1.975475456537005874E-15, 21.00000000000002487, -141.9047308033773902 ) ) ;
#32934=CARTESIAN_POINT ( 'NONE',  ( -3.500000000000001332, 17.50000000000001776, -90.65473080337743284 ) ) ;
#32939=CARTESIAN_POINT ( 'NONE',  ( -7.424026671074350129E-16, 13.45854811567263276, -52.71098080242150985 ) ) ;
#32940=CARTESIAN_POINT ( 'NONE',  ( -3.500000000000002220, 15.47927405783632082, -30.57139747004410069 ) ) ;
#32941=CARTESIAN_POINT ( 'NONE',  ( -3.500000000000001332, 17.50000000000001066, -24.96098080242151340 ) ) ;
#32942=CARTESIAN_POINT ( 'NONE',  ( 2.474675557024783212E-16, 21.54145188432739033, -45.90473080337742573 ) ) ;
#32944=CARTESIAN_POINT ( 'NONE',  ( -1.655278471875002211, 14.63297358603754006, -27.68493913623279568 ) ) ;
#32947=CARTESIAN_POINT ( 'NONE',  ( -3.500000000000000000, 19.52072594216370760, -60.73806413671076143 ) ) ;
#32949=CARTESIAN_POINT ( 'NONE',  ( -0.9378221735089310451, 14.00000000000001066, -33.44938900211595012 ) ) ;
#32951=CARTESIAN_POINT ( 'NONE',  ( -3.310556943750000425, 19.41135094264166838, -75.84743913623279354 ) ) ;
#32952=CARTESIAN_POINT ( 'NONE',  ( -3.500000000000000000, 19.52072594216371826, -141.7380641367107614 ) ) ;
#32953=ORIENTED_EDGE ( 'NONE', *, *, #23088, .F. ) ;
#32954=CARTESIAN_POINT ( 'NONE',  ( -0.9378221735089465882, 21.00000000000001066, -124.1663226036829855 ) ) ;
#32957=AXIS2_PLACEMENT_3D ( 'NONE', #39883, #36055, #33505 ) ;
#32958=EDGE_LOOP ( 'NONE', ( #7599, #11758, #26481, #13097 ) ) ;
#32960=CARTESIAN_POINT ( 'NONE',  ( 3.310556943749999981, 15.58864905735836892, -92.34743913623282197 ) ) ;
#32961=ORIENTED_EDGE ( 'NONE', *, *, #22675, .T. ) ;
#32966=CARTESIAN_POINT ( 'NONE',  ( 1.749999999999998224, 14.46891108675448478, -115.6276474690881741 ) ) ;
#32967=CARTESIAN_POINT ( 'NONE',  ( -3.310556943750002645, 15.58864905735837780, -124.6807724695661364 ) ) ;
#32968=ORIENTED_EDGE ( 'NONE', *, *, #3368, .F. ) ;
#32969=CARTESIAN_POINT ( 'NONE',  ( -3.500000000000001332, 17.50000000000001776, -94.96098080242150274 ) ) ;
#32970=CARTESIAN_POINT ( 'NONE',  ( 2.340729813953370519E-16, 21.32270188528330834, -54.10160580289947063 ) ) ;
#32971=CARTESIAN_POINT ( 'NONE',  ( -3.310556943750000425, 19.41135094264166838, -120.9349391362327992 ) ) ;
#32974=CARTESIAN_POINT ( 'NONE',  ( -3.500000000000000888, 19.52072594216371826, -124.7380641367107756 ) ) ;
#32975=( BOUNDED_CURVE ( )  B_SPLINE_CURVE ( 2, ( #24469, #23638, #31053, #33832, #30426, #27247, #1502, #1905, #7465 ),
 .UNSPECIFIED., .F., .F. ) 
 B_SPLINE_CURVE_WITH_KNOTS ( ( 3, 2, 2, 2, 3 ),
 ( 0.3729166666666666741, 0.3736111111111111160, 0.3750000000000000000, 0.3763888888888888840, 0.3770833333333333259 ),
 .UNSPECIFIED. ) 
 CURVE ( )  GEOMETRIC_REPRESENTATION_ITEM ( )  RATIONAL_B_SPLINE_CURVE ( ( 0.9330127018922194093, 0.9330127018922194093, 1.000000000000000000, 0.8660254037844387076, 1.000000000000000000, 0.8660254037844387076, 1.000000000000000000, 0.9330127018922194093, 0.9330127018922194093 ) ) 
 REPRESENTATION_ITEM ( '' )  );
#32976=CARTESIAN_POINT ( 'NONE',  ( 2.340729813953370519E-16, 21.32270188528330834, -74.10160580289947063 ) ) ;
#32977=CARTESIAN_POINT ( 'NONE',  ( -1.749999999999999778, 20.53108891324555785, -118.1276474690881741 ) ) ;
#32979=CARTESIAN_POINT ( 'NONE',  ( 1.655278471874998436, 14.63297358603754716, -100.4307724695661364 ) ) ;
#32983=CARTESIAN_POINT ( 'NONE',  ( 3.500000000000001332, 17.50000000000001421, -68.46098080242150274 ) ) ;
#32985=CARTESIAN_POINT ( 'NONE',  ( 2.340729813953370519E-16, 21.32270188528330479, -39.01410580289947916 ) ) ;
#32986=CARTESIAN_POINT ( 'NONE',  ( -3.310556943750000425, 19.41135094264166483, -93.93493913623279923 ) ) ;
#32987=CARTESIAN_POINT ( 'NONE',  ( 1.749999999999998224, 14.46891108675447768, -58.32139747004409713 ) ) ;
#32989=CARTESIAN_POINT ( 'NONE',  ( 3.310556943750001313, 17.50000000000002132, -114.3516058028994706 ) ) ;
#32990=CARTESIAN_POINT ( 'NONE',  ( 1.655278471874998436, 14.63297358603754006, -42.51827246956613493 ) ) ;
#32992=CARTESIAN_POINT ( 'NONE',  ( 0.9378221735089300459, 21.00000000000002132, -127.2556390011600200 ) ) ;
#32997=CARTESIAN_POINT ( 'NONE',  ( 4.648177544792955347E-16, 21.00000000000001421, -61.21098080242150985 ) ) ;
#32998=CARTESIAN_POINT ( 'NONE',  ( 3.310556943749999981, 15.58864905735837070, -98.34743913623282197 ) ) ;
#33002=CARTESIAN_POINT ( 'NONE',  ( -3.500000000000001332, 17.50000000000001776, -87.65473080337743284 ) ) ;
#33004=LINE ( 'NONE', #26010, #21047 ) ;
#33006=CYLINDRICAL_SURFACE ( 'NONE', #12378, 3.499999999999999556 ) ;
#33009=CARTESIAN_POINT ( 'NONE',  ( 2.340729813953370519E-16, 21.32270188528330834, -29.01410580289948271 ) ) ;
#33010=EDGE_LOOP ( 'NONE', ( #6027, #40770, #12365, #34995 ) ) ;
#33011=CARTESIAN_POINT ( 'NONE',  ( -3.500000000000002220, 15.47927405783633503, -109.5713974700441042 ) ) ;
#33015=ORIENTED_EDGE ( 'NONE', *, *, #6204, .F. ) ;
#33016=LINE ( 'NONE', #22612, #37554 ) ;
#33018=CARTESIAN_POINT ( 'NONE',  ( -3.310556943750000425, 19.41135094264167549, -139.8474391362327935 ) ) ;
#33022=CARTESIAN_POINT ( 'NONE',  ( -3.310556943750002645, 15.58864905735837780, -135.7682724695661136 ) ) ;
#33023=CARTESIAN_POINT ( 'NONE',  ( -3.500000000000000888, 19.52072594216370405, -29.04431413575483845 ) ) ;
#33028=CARTESIAN_POINT ( 'NONE',  ( -1.750000000000002220, 14.46891108675448834, -131.7943141357548598 ) ) ;
#33029=CARTESIAN_POINT ( 'NONE',  ( -3.310556943750002645, 15.58864905735837780, -119.6807724695661506 ) ) ;
#33033=CARTESIAN_POINT ( 'NONE',  ( -3.500000000000002220, 15.47927405783632793, -84.87764746908817415 ) ) ;
#33034=CARTESIAN_POINT ( 'NONE',  ( 0.000000000000000000, 17.50000000000002487, -149.5231586289125687 ) ) ;
#33035=CARTESIAN_POINT ( 'NONE',  ( -1.655278471874999990, 20.36702641396248836, -50.93077246956613635 ) ) ;
#33036=CARTESIAN_POINT ( 'NONE',  ( 3.310556943749999981, 15.58864905735837247, -113.4349391362328134 ) ) ;
#33037=CARTESIAN_POINT ( 'NONE',  ( -0.9378221735089291577, 21.00000000000001776, -94.16632260368298546 ) ) ;
#33038=CARTESIAN_POINT ( 'NONE',  ( -3.500000000000002220, 15.47927405783632082, -28.57139747004410069 ) ) ;
#33041=CARTESIAN_POINT ( 'NONE',  ( -1.655278471875002211, 14.63297358603755249, -132.6849391362327992 ) ) ;
#33046=CARTESIAN_POINT ( 'NONE',  ( -1.655278471874999990, 20.36702641396248836, -64.01827246956614204 ) ) ;
#33048=CARTESIAN_POINT ( 'NONE',  ( 3.310556943750001313, 19.41135094264166128, -64.18077246956613635 ) ) ;
#33049=ORIENTED_EDGE ( 'NONE', *, *, #40479, .F. ) ;
#33050=CARTESIAN_POINT ( 'NONE',  ( 3.310556943750001313, 19.41135094264166838, -85.26827246956612782 ) ) ;
#33052=CARTESIAN_POINT ( 'NONE',  ( -1.394453263437886604E-15, 14.00000000000001776, -84.71098080242150274 ) ) ;
#33054=CARTESIAN_POINT ( 'NONE',  ( 1.655278471874998436, 14.63297358603754006, -45.43077246956614346 ) ) ;
#33056=CARTESIAN_POINT ( 'NONE',  ( 3.310556943750001313, 17.50000000000002132, -102.2641058028994649 ) ) ;
#33057=CARTESIAN_POINT ( 'NONE',  ( 0.000000000000000000, 21.00000000000002487, -149.5231586289125687 ) ) ;
#33060=EDGE_LOOP ( 'NONE', ( #30726, #31171, #33558, #1281 ) ) ;
#33062=CARTESIAN_POINT ( 'NONE',  ( 1.655278471874998436, 14.63297358603754006, -50.43077246956613635 ) ) ;
#33065=CARTESIAN_POINT ( 'NONE',  ( 0.000000000000000000, 17.50000000000002487, -149.5231586289125687 ) ) ;
#33066=CARTESIAN_POINT ( 'NONE',  ( -0.9378221735089291577, 21.00000000000001776, -96.16632260368297125 ) ) ;
#33069=CARTESIAN_POINT ( 'NONE',  ( 0.9378221735089281585, 14.00000000000002132, -114.6663226036829997 ) ) ;
#33072=CARTESIAN_POINT ( 'NONE',  ( 3.500000000000001332, 17.50000000000001066, -41.46098080242150985 ) ) ;
#33073=CARTESIAN_POINT ( 'NONE',  ( -1.655278471875002211, 14.63297358603754184, -44.59743913623280775 ) ) ;
#33074=CARTESIAN_POINT ( 'NONE',  ( 3.500000000000000000, 15.47927405783632082, -35.23806413671076854 ) ) ;
#33078=CARTESIAN_POINT ( 'NONE',  ( 3.310556943749999981, 15.58864905735836182, -29.43493913623279923 ) ) ;
#33080=CARTESIAN_POINT ( 'NONE',  ( -1.655278471875002211, 14.63297358603754716, -82.68493913623278502 ) ) ;
#33081=CARTESIAN_POINT ( 'NONE',  ( 3.310556943749999981, 15.58864905735837425, -133.3474391362328220 ) ) ;
#33083=DIRECTION ( 'NONE',  ( -0.000000000000000000, 1.259100132267607459E-16, -1.000000000000000000 ) ) ;
#33084=CARTESIAN_POINT ( 'NONE',  ( 0.9378221735089300459, 21.00000000000002132, -113.9493890021159501 ) ) ;
#33085=CARTESIAN_POINT ( 'NONE',  ( -1.655278471875002211, 14.63297358603755249, -130.6849391362327992 ) ) ;
#33087=CARTESIAN_POINT ( 'NONE',  ( -1.655278471874999990, 20.36702641396249192, -86.93077246956613635 ) ) ;
#33089=LINE ( 'NONE', #39472, #23229 ) ;
#33090=CARTESIAN_POINT ( 'NONE',  ( -1.394453263437886604E-15, 14.00000000000002132, -111.7109808024214885 ) ) ;
#33091=CARTESIAN_POINT ( 'NONE',  ( 3.500000000000000000, 15.47927405783632437, -74.23806413671074722 ) ) ;
#33092=CARTESIAN_POINT ( 'NONE',  ( 3.310556943749999981, 15.58864905735836537, -57.43493913623279212 ) ) ;
#33096=CARTESIAN_POINT ( 'NONE',  ( 3.310556943749999981, 15.58864905735836892, -82.43493913623278502 ) ) ;
#33097=CARTESIAN_POINT ( 'NONE',  ( -7.022189441860112050E-16, 13.67729811471672896, -138.6016058028994564 ) ) ;
#33099=CARTESIAN_POINT ( 'NONE',  ( -1.655278471875002211, 14.63297358603754894, -108.5974391362328078 ) ) ;
#33100=CARTESIAN_POINT ( 'NONE',  ( -1.655278471874999990, 20.36702641396249192, -80.93077246956615056 ) ) ;
#33101=CARTESIAN_POINT ( 'NONE',  ( -1.394453263437886604E-15, 14.00000000000001776, -86.71098080242151696 ) ) ;
#33102=ORIENTED_EDGE ( 'NONE', *, *, #17742, .F. ) ;
#33103=CARTESIAN_POINT ( 'NONE',  ( 3.310556943750001313, 19.41135094264166838, -99.26827246956612782 ) ) ;
#33104=CARTESIAN_POINT ( 'NONE',  ( -7.424026671074350129E-16, 13.45854811567263809, -105.4047308033774186 ) ) ;
#33105=( BOUNDED_CURVE ( )  B_SPLINE_CURVE ( 2, ( #11674, #37222, #15091, #34029, #14678, #30834, #7880, #8075, #24673 ),
 .UNSPECIFIED., .F., .F. ) 
 B_SPLINE_CURVE_WITH_KNOTS ( ( 3, 2, 2, 2, 3 ),
 ( 0.1354166666666666574, 0.1361111111111110994, 0.1375000000000000111, 0.1388888888888888951, 0.1395833333333333370 ),
 .UNSPECIFIED. ) 
 CURVE ( )  GEOMETRIC_REPRESENTATION_ITEM ( )  RATIONAL_B_SPLINE_CURVE ( ( 0.9330127018922194093, 0.9330127018922194093, 1.000000000000000000, 0.8660254037844387076, 1.000000000000000000, 0.8660254037844387076, 1.000000000000000000, 0.9330127018922194093, 0.9330127018922194093 ) ) 
 REPRESENTATION_ITEM ( '' )  );
#33107=DIRECTION ( 'NONE',  ( -0.000000000000000000, 1.259100132267607459E-16, -1.000000000000000000 ) ) ;
#33108=CARTESIAN_POINT ( 'NONE',  ( 3.500000000000001332, 19.52072594216371826, -105.0713974700441042 ) ) ;
#33111=CARTESIAN_POINT ( 'NONE',  ( 1.655278471874998436, 14.63297358603754184, -60.43077246956614346 ) ) ;
#33113=EDGE_CURVE ( 'NONE', #15239, #40713, #10699, .T. ) ;
#33114=CARTESIAN_POINT ( 'NONE',  ( -3.310556943750001313, 17.50000000000002132, -113.7641058028994792 ) ) ;
#33117=VERTEX_POINT ( 'NONE', #344 ) ;
#33118=ADVANCED_FACE ( 'NONE', ( #13322 ), #6312, .T. ) ;
#33122=CARTESIAN_POINT ( 'NONE',  ( 2.340729813953370519E-16, 21.32270188528330834, -74.01410580289947916 ) ) ;
#33129=CARTESIAN_POINT ( 'NONE',  ( -3.310556943750002201, 15.58864905735837780, -133.6807724695661364 ) ) ;
#33131=CARTESIAN_POINT ( 'NONE',  ( 1.655278471874998436, 14.63297358603754006, -45.51827246956613493 ) ) ;
#33132=CARTESIAN_POINT ( 'NONE',  ( 3.500000000000001332, 19.52072594216370405, -41.07139747004409003 ) ) ;
#33133=CARTESIAN_POINT ( 'NONE',  ( 3.310556943749999981, 15.58864905735836182, -36.43493913623279923 ) ) ;
#33134=CARTESIAN_POINT ( 'NONE',  ( 1.655278471875001101, 20.36702641396249192, -97.18493913623279923 ) ) ;
#33135=ADVANCED_FACE ( 'NONE', ( #38849 ), #32877, .T. ) ;
#33137=EDGE_CURVE ( 'NONE', #27019, #34378, #13113, .T. ) ;
#33138=CARTESIAN_POINT ( 'NONE',  ( 3.310556943750001313, 19.41135094264165772, -26.18077246956613990 ) ) ;
#33140=CARTESIAN_POINT ( 'NONE',  ( -7.424026671074350129E-16, 13.45854811567263809, -99.71098080242151696 ) ) ;
#33141=CARTESIAN_POINT ( 'NONE',  ( 1.749999999999998224, 14.46891108675448301, -100.3213974700440900 ) ) ;
#33143=CARTESIAN_POINT ( 'NONE',  ( -3.500000000000001332, 17.50000000000001776, -89.65473080337743284 ) ) ;
#33148=CARTESIAN_POINT ( 'NONE',  ( 2.474675557024783212E-16, 21.54145188432739388, -56.21098080242151696 ) ) ;
#33149=CARTESIAN_POINT ( 'NONE',  ( 4.648177544792955347E-16, 21.00000000000001421, -74.21098080242151696 ) ) ;
#33150=CARTESIAN_POINT ( 'NONE',  ( 3.310556943750001313, 17.50000000000001066, -23.26410580289947561 ) ) ;
#33152=CARTESIAN_POINT ( 'NONE',  ( -3.500000000000000888, 19.52072594216370405, -42.73806413671076143 ) ) ;
#33154=CARTESIAN_POINT ( 'NONE',  ( -1.655278471874999990, 20.36702641396248481, -25.01827246956613138 ) ) ;
#33155=CARTESIAN_POINT ( 'NONE',  ( -1.749999999999999778, 20.53108891324554719, -39.82139747004409713 ) ) ;
#33158=CARTESIAN_POINT ( 'NONE',  ( -3.500000000000001332, 17.50000000000001066, -33.65473080337742573 ) ) ;
#33160=CARTESIAN_POINT ( 'NONE',  ( 2.340729813953370519E-16, 21.32270188528331190, -78.01410580289946495 ) ) ;
#33164=CARTESIAN_POINT ( 'NONE',  ( -3.500000000000001332, 17.50000000000001066, -44.96098080242151696 ) ) ;
#33165=EDGE_CURVE ( 'NONE', #17995, #12942, #15050, .T. ) ;
#33167=CARTESIAN_POINT ( 'NONE',  ( -7.460324959392693302E-14, 21.00000000000001776, -88.21098080242150274 ) ) ;
#33168=CARTESIAN_POINT ( 'NONE',  ( 3.310556943749999981, 15.58864905735836892, -89.34743913623279354 ) ) ;
#33169=VERTEX_POINT ( 'NONE', #32464 ) ;
#33172=( BOUNDED_CURVE ( )  B_SPLINE_CURVE ( 2, ( #27878, #17898, #41068, #25118, #28088, #34472, #34680, #41492, #37667 ),
 .UNSPECIFIED., .F., .T. ) 
 B_SPLINE_CURVE_WITH_KNOTS ( ( 3, 2, 2, 2, 3 ),
 ( 0.7687500000000000444, 0.7694444444444444864, 0.7708333333333333703, 0.7722222222222222543, 0.7729166666666666963 ),
 .UNSPECIFIED. ) 
 CURVE ( )  GEOMETRIC_REPRESENTATION_ITEM ( )  RATIONAL_B_SPLINE_CURVE ( ( 0.9330127018922194093, 0.9330127018922194093, 1.000000000000000000, 0.8660254037844387076, 1.000000000000000000, 0.8660254037844387076, 1.000000000000000000, 0.9330127018922194093, 0.9330127018922194093 ) ) 
 REPRESENTATION_ITEM ( '' )  );
#33174=CARTESIAN_POINT ( 'NONE',  ( 0.9378221735089300459, 21.00000000000002132, -115.2556390011600200 ) ) ;
#33176=CARTESIAN_POINT ( 'NONE',  ( 3.310556943750001313, 19.41135094264166838, -126.1807724695661221 ) ) ;
#33178=CARTESIAN_POINT ( 'NONE',  ( 3.310556943749999981, 15.58864905735836182, -52.43493913623280633 ) ) ;
#33179=CARTESIAN_POINT ( 'NONE',  ( 1.655278471875001101, 20.36702641396249547, -115.1849391362327850 ) ) ;
#33180=ORIENTED_EDGE ( 'NONE', *, *, #41968, .F. ) ;
#33183=CARTESIAN_POINT ( 'NONE',  ( 3.500000000000001776, 19.52072594216371826, -123.0713974700441042 ) ) ;
#33185=CARTESIAN_POINT ( 'NONE',  ( -7.022189441860112050E-16, 13.67729811471671653, -41.51410580289947916 ) ) ;
#33186=CARTESIAN_POINT ( 'NONE',  ( 3.310556943749999981, 15.58864905735836714, -73.43493913623279923 ) ) ;
#33187=CARTESIAN_POINT ( 'NONE',  ( 3.500000000000001332, 17.50000000000002132, -115.4609808024215027 ) ) ;
#33188=CARTESIAN_POINT ( 'NONE',  ( -1.655278471875002211, 14.63297358603754894, -101.5974391362328078 ) ) ;
#33189=DIRECTION ( 'NONE',  ( -0.000000000000000000, 1.259100132267607459E-16, -1.000000000000000000 ) ) ;
#33190=CARTESIAN_POINT ( 'NONE',  ( 0.000000000000000000, 21.00000000000002487, -149.5231586289125687 ) ) ;
#33192=CARTESIAN_POINT ( 'NONE',  ( -3.500000000000002220, 15.47927405783632615, -67.87764746908817415 ) ) ;
#33193=FACE_OUTER_BOUND ( 'NONE', #2467, .T. ) ;
#33194=CARTESIAN_POINT ( 'NONE',  ( -1.655278471874999990, 20.36702641396248481, -34.93077246956615056 ) ) ;
#33195=CARTESIAN_POINT ( 'NONE',  ( 3.310556943750001313, 19.41135094264166483, -96.26827246956612782 ) ) ;
#33196=CARTESIAN_POINT ( 'NONE',  ( 1.750000000000001110, 20.53108891324555074, -58.98806413671076143 ) ) ;
#33198=CARTESIAN_POINT ( 'NONE',  ( 3.310556943750001313, 19.41135094264166838, -113.2682724695661562 ) ) ;
#33199=CARTESIAN_POINT ( 'NONE',  ( 3.310556943750001313, 19.41135094264166128, -42.26827246956613493 ) ) ;
#33201=CARTESIAN_POINT ( 'NONE',  ( -1.394453263437886604E-15, 14.00000000000001421, -62.40473080337742573 ) ) ;
#33206=CARTESIAN_POINT ( 'NONE',  ( -7.022189441860112050E-16, 13.67729811471672363, -90.51410580289947916 ) ) ;
#33207=LINE ( 'NONE', #7485, #36227 ) ;
#33213=CARTESIAN_POINT ( 'NONE',  ( 0.000000000000000000, 21.00000000000002487, -149.5231586289125687 ) ) ;
#33217=CARTESIAN_POINT ( 'NONE',  ( 3.310556943750001313, 19.41135094264166128, -31.18077246956615056 ) ) ;
#33220=EDGE_CURVE ( 'NONE', #5763, #11460, #19385, .T. ) ;
#33221=VECTOR ( 'NONE', #29048, 1000.000000000000000 ) ;
#33226=ORIENTED_EDGE ( 'NONE', *, *, #27063, .T. ) ;
#33227=CARTESIAN_POINT ( 'NONE',  ( -0.9378221735089310451, 14.00000000000001066, -53.75563900116004135 ) ) ;
#33228=( BOUNDED_CURVE ( )  B_SPLINE_CURVE ( 2, ( #7873, #27016, #24243, #4669, #37624, #30825, #21457, #27431, #10843 ),
 .UNSPECIFIED., .F., .T. ) 
 B_SPLINE_CURVE_WITH_KNOTS ( ( 3, 2, 2, 2, 3 ),
 ( 0.4562499999999999889, 0.4569444444444444309, 0.4583333333333333148, 0.4597222222222221988, 0.4604166666666666963 ),
 .UNSPECIFIED. ) 
 CURVE ( )  GEOMETRIC_REPRESENTATION_ITEM ( )  RATIONAL_B_SPLINE_CURVE ( ( 0.9330127018922194093, 0.9330127018922194093, 1.000000000000000000, 0.8660254037844387076, 1.000000000000000000, 0.8660254037844387076, 1.000000000000000000, 0.9330127018922167448, 0.9330127018922194093 ) ) 
 REPRESENTATION_ITEM ( '' )  );
#33230=CARTESIAN_POINT ( 'NONE',  ( -1.655278471875002211, 14.63297358603755427, -141.5974391362327935 ) ) ;
#33233=CARTESIAN_POINT ( 'NONE',  ( -3.310556943750001313, 17.50000000000002487, -136.8516058028994564 ) ) ;
#33234=CARTESIAN_POINT ( 'NONE',  ( 3.500000000000001332, 17.50000000000001066, -27.46098080242151340 ) ) ;
#33236=CARTESIAN_POINT ( 'NONE',  ( 3.500000000000001332, 17.50000000000002487, -141.1547308033774186 ) ) ;
#33239=CARTESIAN_POINT ( 'NONE',  ( -3.500000000000001332, 17.50000000000002487, -132.9609808024214885 ) ) ;
#33240=CARTESIAN_POINT ( 'NONE',  ( 1.655278471874998436, 14.63297358603754894, -120.4307724695661364 ) ) ;
#33242=CARTESIAN_POINT ( 'NONE',  ( 4.286263797015737581E-16, 14.00000000000002487, -149.5231586289125687 ) ) ;
#33243=CARTESIAN_POINT ( 'NONE',  ( 3.500000000000001776, 19.52072594216371115, -85.37764746908817415 ) ) ;
#33244=CARTESIAN_POINT ( 'NONE',  ( -1.750000000000002220, 14.46891108675448123, -69.48806413671077564 ) ) ;
#33245=CARTESIAN_POINT ( 'NONE',  ( -7.022189441860112050E-16, 13.67729811471671653, -52.51410580289947205 ) ) ;
#33247=CARTESIAN_POINT ( 'NONE',  ( -3.310556943750001313, 17.50000000000002132, -111.8516058028994564 ) ) ;
#33249=CARTESIAN_POINT ( 'NONE',  ( 3.500000000000001776, 19.52072594216370405, -29.07139747004410069 ) ) ;
#33251=CARTESIAN_POINT ( 'NONE',  ( -1.655278471875002211, 14.63297358603755249, -129.6849391362327992 ) ) ;
#33255=CARTESIAN_POINT ( 'NONE',  ( 1.655278471874998436, 14.63297358603754184, -64.51827246956614204 ) ) ;
#33257=CARTESIAN_POINT ( 'NONE',  ( -1.655278471875002211, 14.63297358603754361, -61.59743913623280775 ) ) ;
#33259=CARTESIAN_POINT ( 'NONE',  ( -3.310556943750002201, 15.58864905735837070, -79.76827246956615625 ) ) ;
#33263=ADVANCED_FACE ( 'NONE', ( #27137 ), #20764, .T. ) ;
#33266=CARTESIAN_POINT ( 'NONE',  ( 2.340729813953370519E-16, 21.32270188528330834, -43.01410580289947205 ) ) ;
#33268=CARTESIAN_POINT ( 'NONE',  ( -3.310556943750000425, 19.41135094264166838, -102.8474391362328220 ) ) ;
#33269=DIRECTION ( 'NONE',  ( -0.000000000000000000, 1.259100132267607459E-16, -1.000000000000000000 ) ) ;
#33271=EDGE_LOOP ( 'NONE', ( #14193, #34793, #25073, #20531 ) ) ;
#33275=CARTESIAN_POINT ( 'NONE',  ( -7.022189441860112050E-16, 13.67729811471671653, -52.51410580289947205 ) ) ;
#33279=CARTESIAN_POINT ( 'NONE',  ( -1.394453263437886604E-15, 14.00000000000002132, -125.4047308033774186 ) ) ;
#33281=DIRECTION ( 'NONE',  ( 0.000000000000000000, 1.000000000000000000, 0.000000000000000000 ) ) ;
#33282=ADVANCED_FACE ( 'NONE', ( #4796 ), #30111, .T. ) ;
#33283=ORIENTED_EDGE ( 'NONE', *, *, #39972, .T. ) ;
#33284=CARTESIAN_POINT ( 'NONE',  ( 3.500000000000001332, 17.50000000000001066, -44.46098080242151696 ) ) ;
#33285=CARTESIAN_POINT ( 'NONE',  ( 3.500000000000000000, 15.47927405783632970, -108.5443141357548598 ) ) ;
#33287=CARTESIAN_POINT ( 'NONE',  ( 4.648177544792955347E-16, 21.00000000000001776, -77.90473080337740441 ) ) ;
#33289=CARTESIAN_POINT ( 'NONE',  ( -1.655278471875002211, 14.63297358603754006, -27.68493913623279568 ) ) ;
#33291=CARTESIAN_POINT ( 'NONE',  ( -3.310556943750000425, 19.41135094264166483, -84.93493913623279923 ) ) ;
#33292=CARTESIAN_POINT ( 'NONE',  ( -1.655278471875002211, 14.63297358603755249, -133.5974391362328220 ) ) ;
#33298=CARTESIAN_POINT ( 'NONE',  ( 3.310556943749999981, 15.58864905735837425, -126.4349391362327992 ) ) ;
#33299=CARTESIAN_POINT ( 'NONE',  ( -3.500000000000002220, 15.47927405783632793, -68.87764746908817415 ) ) ;
#33300=CARTESIAN_POINT ( 'NONE',  ( -3.310556943750002645, 15.58864905735837247, -88.68077246956613635 ) ) ;
#33301=DIRECTION ( 'NONE',  ( -0.000000000000000000, 1.259100132267607459E-16, -1.000000000000000000 ) ) ;
#33302=CARTESIAN_POINT ( 'NONE',  ( 1.750000000000001110, 20.53108891324555429, -100.9880641367107756 ) ) ;
#33303=CARTESIAN_POINT ( 'NONE',  ( 4.286263797015737581E-16, 14.00000000000002487, -149.5231586289125687 ) ) ;
#33304=CARTESIAN_POINT ( 'NONE',  ( -1.750000000000002220, 14.46891108675448123, -73.48806413671076143 ) ) ;
#33305=CARTESIAN_POINT ( 'NONE',  ( 1.655278471875001101, 20.36702641396248836, -52.18493913623279923 ) ) ;
#33307=CARTESIAN_POINT ( 'NONE',  ( -0.9378221735089310451, 14.00000000000001599, -67.44938900211595012 ) ) ;
#33309=CARTESIAN_POINT ( 'NONE',  ( 1.655278471874998436, 14.63297358603754539, -81.51827246956614204 ) ) ;
#33310=CARTESIAN_POINT ( 'NONE',  ( 2.340729813953370519E-16, 21.32270188528332255, -142.1016058028994564 ) ) ;
#33312=CARTESIAN_POINT ( 'NONE',  ( 1.655278471875001101, 20.36702641396249547, -108.0974391362328078 ) ) ;
#33313=CARTESIAN_POINT ( 'NONE',  ( 3.310556943749999981, 15.58864905735836714, -73.34743913623280775 ) ) ;
#33314=LINE ( 'NONE', #31536, #10432 ) ;
#33317=CARTESIAN_POINT ( 'NONE',  ( -1.655278471875002211, 14.63297358603754894, -102.6849391362327992 ) ) ;
#33318=CARTESIAN_POINT ( 'NONE',  ( -1.750000000000002220, 14.46891108675448478, -100.4880641367107756 ) ) ;
#33320=CARTESIAN_POINT ( 'NONE',  ( 3.500000000000000000, 15.47927405783632615, -71.54431413575483134 ) ) ;
#33322=LINE ( 'NONE', #39709, #120 ) ;
#33323=CARTESIAN_POINT ( 'NONE',  ( -1.655278471875002211, 14.63297358603754361, -63.59743913623280775 ) ) ;
#33324=CARTESIAN_POINT ( 'NONE',  ( 4.648177544792955347E-16, 21.00000000000001421, -46.90473080337742573 ) ) ;
#33325=CARTESIAN_POINT ( 'NONE',  ( 3.310556943750001313, 17.50000000000002132, -118.2641058028994792 ) ) ;
#33328=ORIENTED_EDGE ( 'NONE', *, *, #4289, .F. ) ;
#33333=CARTESIAN_POINT ( 'NONE',  ( -1.655278471875002211, 14.63297358603754539, -69.59743913623280775 ) ) ;
#33334=ORIENTED_EDGE ( 'NONE', *, *, #15656, .T. ) ;
#33335=ORIENTED_EDGE ( 'NONE', *, *, #15287, .T. ) ;
#33337=AXIS2_PLACEMENT_3D ( 'NONE', #40546, #23981, #23762 ) ;
#33339=CYLINDRICAL_SURFACE ( 'NONE', #11981, 3.499999999999999556 ) ;
#33342=VERTEX_POINT ( 'NONE', #20332 ) ;
#33343=CARTESIAN_POINT ( 'NONE',  ( 1.655278471875001101, 20.36702641396249902, -135.0974391362328220 ) ) ;
#33345=CARTESIAN_POINT ( 'NONE',  ( 1.655278471875001101, 20.36702641396248481, -44.18493913623279212 ) ) ;
#33346=CARTESIAN_POINT ( 'NONE',  ( 4.648177544792955347E-16, 21.00000000000001066, -40.90473080337742573 ) ) ;
#33347=CARTESIAN_POINT ( 'NONE',  ( 1.655278471874998436, 14.63297358603753828, -38.51827246956612782 ) ) ;
#33348=CARTESIAN_POINT ( 'NONE',  ( 1.655278471874998436, 14.63297358603754716, -98.51827246956612782 ) ) ;
#33350=( BOUNDED_CURVE ( )  B_SPLINE_CURVE ( 2, ( #13251, #32594, #32394, #26235, #19621, #38567, #39185, #35590, #10064 ),
 .UNSPECIFIED., .F., .T. ) 
 B_SPLINE_CURVE_WITH_KNOTS ( ( 3, 2, 2, 2, 3 ),
 ( 0.4770833333333333592, 0.4777777777777778012, 0.4791666666666666852, 0.4805555555555555691, 0.4812500000000000111 ),
 .UNSPECIFIED. ) 
 CURVE ( )  GEOMETRIC_REPRESENTATION_ITEM ( )  RATIONAL_B_SPLINE_CURVE ( ( 0.9330127018922194093, 0.9330127018922220739, 1.000000000000000000, 0.8660254037844387076, 1.000000000000000000, 0.8660254037844387076, 1.000000000000000000, 0.9330127018922194093, 0.9330127018922194093 ) ) 
 REPRESENTATION_ITEM ( '' )  );
#33351=CARTESIAN_POINT ( 'NONE',  ( 2.340729813953370519E-16, 21.32270188528330479, -25.01410580289947561 ) ) ;
#33352=DIRECTION ( 'NONE',  ( -0.000000000000000000, 1.259100132267607459E-16, -1.000000000000000000 ) ) ;
#33353=CARTESIAN_POINT ( 'NONE',  ( -7.424026671074350129E-16, 13.45854811567263809, -102.7109808024215027 ) ) ;
#33354=CARTESIAN_POINT ( 'NONE',  ( -3.500000000000001332, 17.50000000000001421, -73.65473080337743284 ) ) ;
#33355=CARTESIAN_POINT ( 'NONE',  ( 0.000000000000000000, 17.50000000000002487, -149.5231586289125687 ) ) ;
#33356=CARTESIAN_POINT ( 'NONE',  ( 3.500000000000001776, 19.52072594216371115, -89.07139747004409003 ) ) ;
#33360=DIRECTION ( 'NONE',  ( -0.000000000000000000, 1.259100132267607459E-16, -1.000000000000000000 ) ) ;
#33361=CARTESIAN_POINT ( 'NONE',  ( -1.749999999999999778, 20.53108891324555074, -55.12764746908817415 ) ) ;
#33363=CARTESIAN_POINT ( 'NONE',  ( -0.9378221735089291577, 21.00000000000001421, -74.16632260368299967 ) ) ;
#33364=CARTESIAN_POINT ( 'NONE',  ( -0.9378221735089310451, 14.00000000000000888, -24.75563900116003424 ) ) ;
#33365=CARTESIAN_POINT ( 'NONE',  ( -3.500000000000002220, 15.47927405783632082, -34.87764746908818125 ) ) ;
#33366=ORIENTED_EDGE ( 'NONE', *, *, #2554, .F. ) ;
#33367=CARTESIAN_POINT ( 'NONE',  ( -1.749999999999999778, 20.53108891324554719, -42.82139747004409713 ) ) ;
#33369=CARTESIAN_POINT ( 'NONE',  ( -3.310556943750002201, 15.58864905735836182, -25.76827246956613493 ) ) ;
#33370=CYLINDRICAL_SURFACE ( 'NONE', #33523, 3.499999999999999556 ) ;
#33371=CARTESIAN_POINT ( 'NONE',  ( -1.750000000000002220, 14.46891108675447946, -56.79431413575483845 ) ) ;
#33376=CARTESIAN_POINT ( 'NONE',  ( -7.022189441860112050E-16, 13.67729811471672186, -78.51410580289946495 ) ) ;
#33379=DIRECTION ( 'NONE',  ( -0.000000000000000000, 1.259100132267607459E-16, -1.000000000000000000 ) ) ;
#33381=CARTESIAN_POINT ( 'NONE',  ( 1.749999999999998224, 14.46891108675448123, -90.32139747004410424 ) ) ;
#33384=CARTESIAN_POINT ( 'NONE',  ( 3.310556943750001313, 19.41135094264166483, -82.18077246956616477 ) ) ;
#33385=EDGE_CURVE ( 'NONE', #29038, #22244, #26935, .T. ) ;
#33386=ORIENTED_EDGE ( 'NONE', *, *, #18698, .F. ) ;
#33390=CARTESIAN_POINT ( 'NONE',  ( 3.500000000000001332, 17.50000000000002132, -115.4609808024215027 ) ) ;
#33391=CARTESIAN_POINT ( 'NONE',  ( -7.022189441860112050E-16, 13.67729811471672718, -127.5141058028994649 ) ) ;
#33392=ORIENTED_EDGE ( 'NONE', *, *, #21188, .T. ) ;
#33393=CARTESIAN_POINT ( 'NONE',  ( -3.500000000000002220, 15.47927405783632082, -31.57139747004410069 ) ) ;
#33394=CARTESIAN_POINT ( 'NONE',  ( 1.655278471874998436, 14.63297358603754006, -53.51827246956612782 ) ) ;
#33395=CARTESIAN_POINT ( 'NONE',  ( -7.022189441860112050E-16, 13.67729811471672718, -112.6016058028994564 ) ) ;
#33396=EDGE_LOOP ( 'NONE', ( #15877, #36368, #18527, #15346 ) ) ;
#33397=ORIENTED_EDGE ( 'NONE', *, *, #19775, .T. ) ;
#33399=CARTESIAN_POINT ( 'NONE',  ( -3.500000000000001332, 17.50000000000002132, -127.6547308033774186 ) ) ;
#33402=CARTESIAN_POINT ( 'NONE',  ( -3.310556943750001313, 17.50000000000001066, -39.76410580289947916 ) ) ;
#33403=CARTESIAN_POINT ( 'NONE',  ( -1.655278471875002211, 14.63297358603754539, -68.68493913623279923 ) ) ;
#33404=CARTESIAN_POINT ( 'NONE',  ( -3.500000000000002220, 15.47927405783633503, -118.8776474690881884 ) ) ;
#33405=CARTESIAN_POINT ( 'NONE',  ( 1.655278471874998436, 14.63297358603754716, -103.4307724695661364 ) ) ;
#33408=CARTESIAN_POINT ( 'NONE',  ( -1.749999999999999778, 20.53108891324555074, -70.82139747004409003 ) ) ;
#33410=CARTESIAN_POINT ( 'NONE',  ( -3.500000000000001332, 17.50000000000001421, -69.96098080242151696 ) ) ;
#33411=CARTESIAN_POINT ( 'NONE',  ( 4.286263797015737581E-16, 14.00000000000002487, -149.5231586289125687 ) ) ;
#33412=CARTESIAN_POINT ( 'NONE',  ( -3.310556943750002645, 15.58864905735836537, -35.68077246956613635 ) ) ;
#33413=CARTESIAN_POINT ( 'NONE',  ( 1.655278471875001101, 20.36702641396249192, -91.18493913623279923 ) ) ;
#33414=CARTESIAN_POINT ( 'NONE',  ( 1.750000000000001110, 20.53108891324555074, -57.98806413671076143 ) ) ;
#33416=CARTESIAN_POINT ( 'NONE',  ( -1.655278471875002211, 14.63297358603755072, -113.6849391362327992 ) ) ;
#33417=CARTESIAN_POINT ( 'NONE',  ( -3.310556943750001313, 17.50000000000001066, -40.85160580289947063 ) ) ;
#33419=CARTESIAN_POINT ( 'NONE',  ( -3.500000000000001332, 17.50000000000001421, -62.65473080337742573 ) ) ;
#33425=CARTESIAN_POINT ( 'NONE',  ( 3.310556943749999981, 15.58864905735837070, -95.34743913623282197 ) ) ;
#33426=AXIS2_PLACEMENT_3D ( 'NONE', #9037, #37967, #12223 ) ;
#33429=FACE_OUTER_BOUND ( 'NONE', #35013, .T. ) ;
#33435=CARTESIAN_POINT ( 'NONE',  ( -7.022189441860112050E-16, 13.67729811471671653, -29.51410580289948982 ) ) ;
#33436=EDGE_CURVE ( 'NONE', #3726, #25228, #3369, .T. ) ;
#33438=EDGE_CURVE ( 'NONE', #16907, #25161, #34970, .T. ) ;
#33441=ADVANCED_FACE ( 'NONE', ( #12217 ), #41161, .T. ) ;
#33445=ORIENTED_EDGE ( 'NONE', *, *, #24367, .F. ) ;
#33446=CARTESIAN_POINT ( 'NONE',  ( 1.743066579297357930E-14, 14.00000000000002132, -129.4047308033774186 ) ) ;
#33450=CARTESIAN_POINT ( 'NONE',  ( -3.500000000000002220, 15.47927405783632793, -80.87764746908817415 ) ) ;
#33451=CARTESIAN_POINT ( 'NONE',  ( -1.655278471875002211, 14.63297358603755249, -130.6849391362327992 ) ) ;
#33452=CARTESIAN_POINT ( 'NONE',  ( -1.749999999999999778, 20.53108891324554719, -26.12764746908817415 ) ) ;
#33453=VECTOR ( 'NONE', #20053, 1000.000000000000000 ) ;
#33455=CARTESIAN_POINT ( 'NONE',  ( -3.500000000000000888, 19.52072594216372181, -140.7380641367107614 ) ) ;
#33456=CARTESIAN_POINT ( 'NONE',  ( 3.500000000000001332, 17.50000000000002132, -123.4609808024215027 ) ) ;
#33458=CARTESIAN_POINT ( 'NONE',  ( 1.750000000000001110, 20.53108891324556140, -135.2943141357548598 ) ) ;
#33459=CARTESIAN_POINT ( 'NONE',  ( -7.022189441860112050E-16, 13.67729811471672718, -120.5141058028994649 ) ) ;
#33462=CARTESIAN_POINT ( 'NONE',  ( 1.750000000000001110, 20.53108891324555429, -88.29431413575483134 ) ) ;
#33464=CARTESIAN_POINT ( 'NONE',  ( 4.286263797015737581E-16, 14.00000000000002487, -149.5231586289125687 ) ) ;
#33465=CARTESIAN_POINT ( 'NONE',  ( 3.310556943750001313, 19.41135094264166128, -55.18077246956614346 ) ) ;
#33466=CARTESIAN_POINT ( 'NONE',  ( -7.022189441860112050E-16, 13.67729811471672718, -110.6016058028994706 ) ) ;
#33469=EDGE_CURVE ( 'NONE', #39287, #13090, #24672, .T. ) ;
#33470=CARTESIAN_POINT ( 'NONE',  ( -1.655278471874999990, 20.36702641396249902, -130.0182724695661136 ) ) ;
#33473=CARTESIAN_POINT ( 'NONE',  ( 3.500000000000000000, 15.47927405783633503, -124.2380641367107756 ) ) ;
#33474=DIRECTION ( 'NONE',  ( -0.000000000000000000, 1.259100132267607459E-16, -1.000000000000000000 ) ) ;
#33475=CARTESIAN_POINT ( 'NONE',  ( 3.310556943750001313, 19.41135094264166128, -63.26827246956613493 ) ) ;
#33478=CARTESIAN_POINT ( 'NONE',  ( 3.310556943750001313, 17.50000000000001776, -82.35160580289945642 ) ) ;
#33482=EDGE_CURVE ( 'NONE', #2211, #40707, #15212, .T. ) ;
#33485=CARTESIAN_POINT ( 'NONE',  ( 3.310556943749999981, 15.58864905735836182, -43.34743913623280775 ) ) ;
#33487=CARTESIAN_POINT ( 'NONE',  ( -3.310556943750001313, 17.50000000000002132, -102.7641058028994649 ) ) ;
#33488=CARTESIAN_POINT ( 'NONE',  ( -1.394453263437886604E-15, 14.00000000000001776, -82.71098080242150274 ) ) ;
#33489=( BOUNDED_CURVE ( )  B_SPLINE_CURVE ( 2, ( #29583, #3427, #12592, #35964, #18973, #447, #16209, #9617, #22581 ),
 .UNSPECIFIED., .F., .T. ) 
 B_SPLINE_CURVE_WITH_KNOTS ( ( 3, 2, 2, 2, 3 ),
 ( 0.7687500000000000444, 0.7694444444444444864, 0.7708333333333333703, 0.7722222222222222543, 0.7729166666666666963 ),
 .UNSPECIFIED. ) 
 CURVE ( )  GEOMETRIC_REPRESENTATION_ITEM ( )  RATIONAL_B_SPLINE_CURVE ( ( 0.9330127018922194093, 0.9330127018922194093, 1.000000000000000000, 0.8660254037844387076, 1.000000000000000000, 0.8660254037844387076, 1.000000000000000000, 0.9330127018922194093, 0.9330127018922194093 ) ) 
 REPRESENTATION_ITEM ( '' )  );
#33490=EDGE_CURVE ( 'NONE', #10427, #34369, #5912, .T. ) ;
#33495=CARTESIAN_POINT ( 'NONE',  ( 3.310556943749999981, 15.58864905735836182, -51.34743913623281486 ) ) ;
#33496=ORIENTED_EDGE ( 'NONE', *, *, #33783, .F. ) ;
#33497=ORIENTED_EDGE ( 'NONE', *, *, #14263, .F. ) ;
#33498=CARTESIAN_POINT ( 'NONE',  ( 3.500000000000001332, 17.50000000000001776, -93.46098080242151696 ) ) ;
#33501=CARTESIAN_POINT ( 'NONE',  ( 4.286263797015737581E-16, 14.00000000000002487, -149.5231586289125687 ) ) ;
#33502=EDGE_LOOP ( 'NONE', ( #28052, #13073, #10168, #24603 ) ) ;
#33504=CARTESIAN_POINT ( 'NONE',  ( -3.500000000000001332, 17.50000000000001066, -45.96098080242150274 ) ) ;
#33505=DIRECTION ( 'NONE',  ( 0.000000000000000000, 1.000000000000000000, 0.000000000000000000 ) ) ;
#33509=CARTESIAN_POINT ( 'NONE',  ( -7.022189441860112050E-16, 13.67729811471671475, -31.60160580289945997 ) ) ;
#33511=AXIS2_PLACEMENT_3D ( 'NONE', #7574, #4385, #17364 ) ;
#33512=CARTESIAN_POINT ( 'NONE',  ( 3.310556943750001313, 17.50000000000001776, -84.35160580289947063 ) ) ;
#33513=CARTESIAN_POINT ( 'NONE',  ( 1.655278471875001101, 20.36702641396249902, -134.0974391362328220 ) ) ;
#33516=AXIS2_PLACEMENT_3D ( 'NONE', #31388, #41391, #2254 ) ;
#33517=CARTESIAN_POINT ( 'NONE',  ( -3.500000000000002220, 15.47927405783632082, -38.57139747004409003 ) ) ;
#33519=CARTESIAN_POINT ( 'NONE',  ( 3.310556943750001313, 17.50000000000002487, -130.3516058028994564 ) ) ;
#33520=CARTESIAN_POINT ( 'NONE',  ( 0.000000000000000000, 17.50000000000002487, -149.5231586289125687 ) ) ;
#33521=CARTESIAN_POINT ( 'NONE',  ( 1.655278471874998436, 14.63297358603754539, -85.43077246956613635 ) ) ;
#33523=AXIS2_PLACEMENT_3D ( 'NONE', #4020, #39316, #23166 ) ;
#33525=EDGE_CURVE ( 'NONE', #16808, #12464, #34139, .T. ) ;
#33526=DIRECTION ( 'NONE',  ( 0.000000000000000000, 1.000000000000000000, 0.000000000000000000 ) ) ;
#33527=CARTESIAN_POINT ( 'NONE',  ( -3.500000000000001332, 17.50000000000001421, -68.65473080337743284 ) ) ;
#33528=CARTESIAN_POINT ( 'NONE',  ( 3.310556943750001313, 17.50000000000001421, -52.35160580289946353 ) ) ;
#33531=CARTESIAN_POINT ( 'NONE',  ( -1.394453263437886604E-15, 14.00000000000001776, -107.7109808024215170 ) ) ;
#33532=CARTESIAN_POINT ( 'NONE',  ( -1.655278471875002211, 14.63297358603754539, -79.68493913623279923 ) ) ;
#33533=CARTESIAN_POINT ( 'NONE',  ( -3.310556943750002645, 15.58864905735837958, -141.7682724695661420 ) ) ;
#33535=CARTESIAN_POINT ( 'NONE',  ( -3.310556943750001313, 17.50000000000002132, -106.7641058028994649 ) ) ;
#33536=CARTESIAN_POINT ( 'NONE',  ( -7.022189441860112050E-16, 13.67729811471672186, -77.51410580289945074 ) ) ;
#33537=DIRECTION ( 'NONE',  ( 0.000000000000000000, 1.000000000000000000, 0.000000000000000000 ) ) ;
#33539=CARTESIAN_POINT ( 'NONE',  ( -3.310556943750002201, 15.58864905735837247, -94.76827246956612782 ) ) ;
#33540=CARTESIAN_POINT ( 'NONE',  ( 3.500000000000001332, 17.50000000000001776, -100.1547308033774328 ) ) ;
#33542=CARTESIAN_POINT ( 'NONE',  ( 3.500000000000001332, 17.50000000000001776, -91.46098080242151696 ) ) ;
#33543=CARTESIAN_POINT ( 'NONE',  ( -3.500000000000000000, 19.52072594216370760, -52.04431413575484555 ) ) ;
#33546=CARTESIAN_POINT ( 'NONE',  ( 1.655278471875001101, 20.36702641396248836, -59.09743913623280775 ) ) ;
#33548=CARTESIAN_POINT ( 'NONE',  ( 3.310556943750001313, 19.41135094264166838, -115.1807724695661364 ) ) ;
#33553=ORIENTED_EDGE ( 'NONE', *, *, #10865, .T. ) ;
#33557=CARTESIAN_POINT ( 'NONE',  ( 1.655278471875001101, 20.36702641396248836, -68.09743913623280775 ) ) ;
#33558=ORIENTED_EDGE ( 'NONE', *, *, #1068, .T. ) ;
#33561=CARTESIAN_POINT ( 'NONE',  ( 7.785697387528201340E-15, 14.00000000000002487, -137.7109808024215170 ) ) ;
#33564=ORIENTED_EDGE ( 'NONE', *, *, #14683, .F. ) ;
#33565=CARTESIAN_POINT ( 'NONE',  ( 0.000000000000000000, 21.00000000000002487, -149.5231586289125687 ) ) ;
#33567=CARTESIAN_POINT ( 'NONE',  ( -1.655278471874999990, 20.36702641396249902, -135.9307724695661364 ) ) ;
#33568=CARTESIAN_POINT ( 'NONE',  ( -3.500000000000001332, 17.50000000000001776, -74.65473080337743284 ) ) ;
#33569=CARTESIAN_POINT ( 'NONE',  ( -7.022189441860112050E-16, 13.67729811471671653, -47.60160580289946353 ) ) ;
#33570=LINE ( 'NONE', #41357, #4410 ) ;
#33571=CARTESIAN_POINT ( 'NONE',  ( 3.310556943749999981, 15.58864905735836182, -39.43493913623280633 ) ) ;
#33572=CARTESIAN_POINT ( 'NONE',  ( -7.022189441860112050E-16, 13.67729811471672541, -100.6016058028994564 ) ) ;
#33575=CARTESIAN_POINT ( 'NONE',  ( -7.022189441860112050E-16, 13.67729811471672896, -142.6016058028994564 ) ) ;
#33579=CARTESIAN_POINT ( 'NONE',  ( -3.500000000000000888, 19.52072594216371115, -99.04431413575484555 ) ) ;
#33581=CARTESIAN_POINT ( 'NONE',  ( 0.9378221735089281585, 14.00000000000001243, -64.66632260368298546 ) ) ;
#33582=CARTESIAN_POINT ( 'NONE',  ( -7.424026671074350129E-16, 13.45854811567263631, -86.40473080337743284 ) ) ;
#33583=CARTESIAN_POINT ( 'NONE',  ( 2.340729813953370519E-16, 21.32270188528331190, -69.10160580289947063 ) ) ;
#33587=CARTESIAN_POINT ( 'NONE',  ( -3.500000000000000000, 19.52072594216371826, -120.0443141357548313 ) ) ;
#33588=CARTESIAN_POINT ( 'NONE',  ( 1.749999999999998224, 14.46891108675447590, -52.62764746908817415 ) ) ;
#33592=CARTESIAN_POINT ( 'NONE',  ( -3.500000000000000888, 19.52072594216370405, -41.73806413671076143 ) ) ;
#33594=AXIS2_PLACEMENT_3D ( 'NONE', #24812, #35000, #2037 ) ;
#33595=CARTESIAN_POINT ( 'NONE',  ( 2.340729813953370519E-16, 21.32270188528330834, -24.10160580289946708 ) ) ;
#33596=CARTESIAN_POINT ( 'NONE',  ( -0.9378221735089310451, 14.00000000000001066, -39.44938900211595012 ) ) ;
#33597=CARTESIAN_POINT ( 'NONE',  ( -3.500000000000001332, 17.50000000000001776, -90.65473080337743284 ) ) ;
#33600=CARTESIAN_POINT ( 'NONE',  ( 4.648177544792955347E-16, 21.00000000000001776, -84.90473080337743284 ) ) ;
#33602=CARTESIAN_POINT ( 'NONE',  ( 3.310556943750001313, 17.50000000000001776, -78.26410580289946495 ) ) ;
#33603=CARTESIAN_POINT ( 'NONE',  ( 3.602337597214540226E-14, 14.00000000000002132, -116.4047308033774328 ) ) ;
#33605=CARTESIAN_POINT ( 'NONE',  ( -1.394453263437886604E-15, 14.00000000000001776, -97.71098080242148853 ) ) ;
#33606=CARTESIAN_POINT ( 'NONE',  ( -1.750000000000002220, 14.46891108675447946, -54.48806413671076854 ) ) ;
#33608=CARTESIAN_POINT ( 'NONE',  ( -1.749999999999999778, 20.53108891324555785, -120.8213974700441042 ) ) ;
#33609=CARTESIAN_POINT ( 'NONE',  ( -3.310556943750002645, 15.58864905735837247, -84.68077246956613635 ) ) ;
#33610=ORIENTED_EDGE ( 'NONE', *, *, #4289, .T. ) ;
#33614=CARTESIAN_POINT ( 'NONE',  ( 4.648177544792955347E-16, 21.00000000000001421, -59.21098080242150274 ) ) ;
#33615=( BOUNDED_CURVE ( )  B_SPLINE_CURVE ( 2, ( #1334, #13664, #26647, #39607, #5773, #37477, #18750, #2373, #25344 ),
 .UNSPECIFIED., .F., .T. ) 
 B_SPLINE_CURVE_WITH_KNOTS ( ( 3, 2, 2, 2, 3 ),
 ( 0.06458333333333333981, 0.06527777777777778179, 0.06666666666666666574, 0.06805555555555554970, 0.06875000000000000555 ),
 .UNSPECIFIED. ) 
 CURVE ( )  GEOMETRIC_REPRESENTATION_ITEM ( )  RATIONAL_B_SPLINE_CURVE ( ( 0.9330127018922194093, 0.9330127018922200755, 1.000000000000000000, 0.8660254037844387076, 1.000000000000000000, 0.8660254037844387076, 1.000000000000000000, 0.9330127018922187432, 0.9330127018922194093 ) ) 
 REPRESENTATION_ITEM ( '' )  );
#33616=VECTOR ( 'NONE', #37022, 1000.000000000000000 ) ;
#33617=CARTESIAN_POINT ( 'NONE',  ( 1.655278471874998436, 14.63297358603755072, -126.4307724695661364 ) ) ;
#33618=( BOUNDED_CURVE ( )  B_SPLINE_CURVE ( 2, ( #4931, #24722, #1750, #24510, #30676, #14731, #37684, #5146, #21105 ),
 .UNSPECIFIED., .F., .T. ) 
 B_SPLINE_CURVE_WITH_KNOTS ( ( 3, 2, 2, 2, 3 ),
 ( 0.02291666666666666852, 0.02361111111111111049, 0.02500000000000000139, 0.02638888888888888881, 0.02708333333333333426 ),
 .UNSPECIFIED. ) 
 CURVE ( )  GEOMETRIC_REPRESENTATION_ITEM ( )  RATIONAL_B_SPLINE_CURVE ( ( 0.9330127018922194093, 0.9330127018922195203, 1.000000000000000000, 0.8660254037844387076, 1.000000000000000000, 0.8660254037844387076, 1.000000000000000000, 0.9330127018922191873, 0.9330127018922194093 ) ) 
 REPRESENTATION_ITEM ( '' )  );
#33619=AXIS2_PLACEMENT_3D ( 'NONE', #29161, #41957, #5803 ) ;
#33620=CARTESIAN_POINT ( 'NONE',  ( -1.394453263437886604E-15, 14.00000000000001066, -31.40473080337742573 ) ) ;
#33621=CARTESIAN_POINT ( 'NONE',  ( -3.310556943750000425, 19.41135094264166128, -52.93493913623280633 ) ) ;
#33622=CARTESIAN_POINT ( 'NONE',  ( 2.340729813953370519E-16, 21.32270188528331900, -114.1016058028994564 ) ) ;
#33623=VERTEX_POINT ( 'NONE', #9455 ) ;
#33624=CARTESIAN_POINT ( 'NONE',  ( -7.424026671074350129E-16, 13.45854811567264164, -124.4047308033774328 ) ) ;
#33625=CARTESIAN_POINT ( 'NONE',  ( -3.310556943750001313, 17.50000000000001066, -38.76410580289947916 ) ) ;
#33626=CARTESIAN_POINT ( 'NONE',  ( 3.310556943749999981, 15.58864905735836537, -67.43493913623279923 ) ) ;
#33627=CARTESIAN_POINT ( 'NONE',  ( -3.500000000000002220, 15.47927405783633503, -116.8776474690881599 ) ) ;
#33628=CARTESIAN_POINT ( 'NONE',  ( -3.310556943750001313, 17.50000000000001776, -94.76410580289946495 ) ) ;
#33629=CYLINDRICAL_SURFACE ( 'NONE', #30783, 3.499999999999999556 ) ;
#33630=EDGE_CURVE ( 'NONE', #11167, #25797, #27888, .T. ) ;
#33631=DIRECTION ( 'NONE',  ( 0.000000000000000000, 1.000000000000000000, 0.000000000000000000 ) ) ;
#33634=CARTESIAN_POINT ( 'NONE',  ( -3.500000000000000888, 19.52072594216370760, -72.04431413575483134 ) ) ;
#33635=CARTESIAN_POINT ( 'NONE',  ( 0.000000000000000000, 21.00000000000002487, -149.5231586289125687 ) ) ;
#33636=CARTESIAN_POINT ( 'NONE',  ( 1.655278471875001101, 20.36702641396248481, -30.09743913623280775 ) ) ;
#33637=CARTESIAN_POINT ( 'NONE',  ( -1.655278471874999990, 20.36702641396249192, -92.01827246956611361 ) ) ;
#33639=CARTESIAN_POINT ( 'NONE',  ( 3.500000000000000000, 15.47927405783632260, -57.23806413671076143 ) ) ;
#33641=CARTESIAN_POINT ( 'NONE',  ( -3.310556943750000425, 19.41135094264166838, -110.9349391362327850 ) ) ;
#33642=CARTESIAN_POINT ( 'NONE',  ( 1.655278471874998436, 14.63297358603754006, -43.51827246956613493 ) ) ;
#33644=CARTESIAN_POINT ( 'NONE',  ( -0.9378221735089310451, 14.00000000000001599, -62.44938900211595723 ) ) ;
#33649=CARTESIAN_POINT ( 'NONE',  ( 1.655278471875001101, 20.36702641396249192, -95.09743913623280775 ) ) ;
#33652=ORIENTED_EDGE ( 'NONE', *, *, #29322, .T. ) ;
#33654=CARTESIAN_POINT ( 'NONE',  ( 1.749999999999998224, 14.46891108675447768, -57.62764746908817415 ) ) ;
#33656=CYLINDRICAL_SURFACE ( 'NONE', #31810, 3.499999999999999556 ) ;
#33657=ORIENTED_EDGE ( 'NONE', *, *, #20402, .T. ) ;
#33661=ADVANCED_FACE ( 'NONE', ( #2648 ), #35399, .T. ) ;
#33662=CARTESIAN_POINT ( 'NONE',  ( 4.648177544792955347E-16, 21.00000000000001776, -81.90473080337743284 ) ) ;
#33670=CARTESIAN_POINT ( 'NONE',  ( 3.500000000000001332, 17.50000000000002487, -137.1547308033774186 ) ) ;
#33671=CARTESIAN_POINT ( 'NONE',  ( 4.648177544792955347E-16, 21.00000000000001421, -64.90473080337743284 ) ) ;
#33673=CARTESIAN_POINT ( 'NONE',  ( -1.655278471874999990, 20.36702641396249902, -132.0182724695661420 ) ) ;
#33674=CARTESIAN_POINT ( 'NONE',  ( 1.750000000000001110, 20.53108891324554719, -26.29431413575483845 ) ) ;
#33676=CARTESIAN_POINT ( 'NONE',  ( 3.500000000000000000, 15.47927405783633503, -142.2380641367107614 ) ) ;
#33678=CARTESIAN_POINT ( 'NONE',  ( 0.9378221735089281585, 14.00000000000001066, -43.36007260463891555 ) ) ;
#33680=CARTESIAN_POINT ( 'NONE',  ( -1.749999999999999778, 20.53108891324556140, -134.1276474690881741 ) ) ;
#33681=ADVANCED_FACE ( 'NONE', ( #22637 ), #19238, .T. ) ;
#33682=CARTESIAN_POINT ( 'NONE',  ( -3.310556943750000425, 19.41135094264166838, -115.8474391362327935 ) ) ;
#33684=CARTESIAN_POINT ( 'NONE',  ( 3.500000000000001332, 19.52072594216371826, -128.3776474690881741 ) ) ;
#33685=CARTESIAN_POINT ( 'NONE',  ( 3.500000000000000000, 15.47927405783632615, -87.54431413575483134 ) ) ;
#33687=CARTESIAN_POINT ( 'NONE',  ( 3.310556943749999981, 15.58864905735836182, -50.34743913623281486 ) ) ;
#33689=CARTESIAN_POINT ( 'NONE',  ( 1.655278471874998436, 14.63297358603754716, -105.5182724695661278 ) ) ;
#33690=CARTESIAN_POINT ( 'NONE',  ( -1.749999999999999778, 20.53108891324555429, -94.12764746908815994 ) ) ;
#33693=CARTESIAN_POINT ( 'NONE',  ( -1.655278471874999990, 20.36702641396249547, -129.0182724695661136 ) ) ;
#33696=DIRECTION ( 'NONE',  ( -0.000000000000000000, 1.259100132267607459E-16, -1.000000000000000000 ) ) ;
#33697=CARTESIAN_POINT ( 'NONE',  ( 3.500000000000001332, 19.52072594216370760, -58.37764746908817415 ) ) ;
#33698=( BOUNDED_SURFACE ( )  B_SPLINE_SURFACE ( 1, 2, ( 
 ( #26649, #30042, #10694, #20896, #697, #39609, #7293, #23893, #16865, #4729, #23678, #27496, #14100, #4312, #7720, #10481, #36428, #20263, #1540, #36860, #33230, #17293, #7505, #20693, #36205, #20483, #30257, #3886, #40038, #4521, #30466, #1336, #14308, #7077, #27287, #20055, #40250, #11121, #24103, #29830, #37075, #33018, #7930, #14523, #40464, #11319, #21106, #15364, #15141, #31711, #41513, #27897, #34078, #37480, #21520, #18125, #8127, #31296, #28312, #34490, #24723, #24932, #2579, #40872, #12144, #27691, #40661, #24511, #41297, #28105, #41089, #1752, #38102, #34907, #37685, #34283, #5348, #8960, #5564, #14930, #31094, #25137, #11518, #18537, #1949, #21930, #37890, #18325, #31506, #5775, #11724, #18752, #15563, #28521, #11938, #8333, #8542, #24305, #2155, #21312, #8750, #21724, #37274, #2375, #34699, #4932, #14732, #17914, #30891, #5147, #216, #35539, #15, #12995, #25975, #25559, #39136, #19784, #26186, #28725, #16404, #41933, #12780, #15995, #35748, #29138, #25765, #6610, #9601, #9171, #19374, #22349, #31921, #19166, #3001, #3412, #6191, #10016, #6402, #29347, #15776, #28936, #16196, #25347, #13198, #32137, #38305, #41720, #12574, #3617, #38519, #19573, #38730, #9386, #18956, #38938, #2792, #29566, #22146, #22979, #32546, #16607, #9815, #22561, #12363, #32347, #35946, #35326, #3212, #22776, #6810, #32750, #35118, #5982, #1079, #7666, #27023, #17456, #36375, #10853, #639, #36152, #7451, #7025, #14256, #26386, #36806, #30202, #30415, #33391, #17024, #430, #7243, #20639, #13614, #29987, #16812, #4258, #4475, #23410, #20214, #14052, #33617, #39986, #1286, #33176, #23838, #10216, #29777, #860, #10431, #39338, #39780, #13403, #10647, #13832, #17241, #23187, #26813, #20002, #4042, #23624, #36586, #32967, #3834, #26596, #20428, #39555, #6963, #9753, #6337, #19521, #10159, #19726, #29082, #32287, #29501, #41874, #32694, #3154, #23127, #9963, #6554, #3556, #26331, #42078, #19939, #29716, #39277, #29286, #22495, #16144, #32904, #32490, #25703, #12934, #13139, #36094, #16550, #16343, #26124, #15928, #3769, #25912, #13349, #16754, #3356, #39081, #22923, #35888, #9537, #578, #13550, #38459, #12725, #372, #38877, #22713, #35692, #9322, #6752, #158, #22289, #35263, #6124, #19103, #19311, #28877, #32070, #2939, #38667, #35478, #40347, #7596, #30558, #29927, #30137, #30347, #39496, #17591, #33325, #10370, #799, #13772, #17796, #39712, #33760, #39922, #1426, #36734, #26960, #27165, #33961, #1014, #14399, #26750, #10585, #23563, #27375, #1220, #17387, #3978, #11212, #37163, #10784, #36522, #20571, #24196, #7815, #17177, #20359, #8014, #7385, #20790, #4193, #20986, #40131, #33548, #4613, #4820, #13982, #30769, #1630, #26538, #14189, #23767, #4409, #23345, #10999, #23986, #36954, #36308, #7181, #20154, #33114, #16960, #34164, #15449, #2040, #31598, #2465, #37777, #2255, #15236, #28196, #27783, #41392, #22030, #28404, #30981, #18633, #15023, #27988, #18212, #37983, #31389, #40967, #8842, #11820, #11407, #21605, #24602, #5022, #21398, #5236, #5657, #8420, #12240, #8632, #25226, #18003, #31180, #18421, #27584, #38190, #34377, #40552, #1837, #14817, #5867, #40752, #21820, #24816, #11608, #21190, #41184, #37567, #31798, #24392, #9054, #34791, #18839, #12029, #34579, #14611, #5443, #35003, #25022, #37361, #8216, #29226, #39222, #9477, #22442, #9908, #310, #6695, #10104, #35421, #32636, #12459, #15875, #42027, #38612, #28615, #9698, #19664, #6070, #6284, #6496, #15658, #35832, #19259, #41603, #19049, #32018, #36036, #28820, #22864, #16090, #41819, #9268, #16285, #22236, #19876, #25442, #16492, #3500, #6902, #102, #29030, #2671, #32230, #29441, #12672, #12878, #2885, #13083, #23068, #3098, #25858, #13292, #26276, #38404, #35206, #38821, #25651, #22658, #35633, #19467, #32435, #3298, #26066, #39023, #955, #33268, #33487, #40291, #36466, #20732, #36246, #7119, #33056, #36897, #36677, #23714, #10308, #4560, #1371, #4132, #736, #13921, #17536, #14133, #23504, #39651, #23927, #20092, #27108, #10522, #30502, #4350, #26900, #40076, #33708, #7330, #14346, #24143, #27325, #7541, #16903, #20300, #11160, #39867, #3922, #17117, #20515, #37113, #10943, #10728, #17330, #23281, #7966, #30082, #7759, #32842, #1164, #3709, #29654, #519, #29869, #13491, #26477, #39433, #13710, #25546, #8943, #21915, #25122, #2776, #38290, #34893, #15759, #18737, #17745, #28505, #31492, #40500, #28300, #12127, #12559, #15351, #35314, #2567, #41283, #6178, #31907, #22337, #33906, #18524, #15550, #5761, #24343, #31699, #38087, #21709, #37876, #5550, #2359, #34684, #8735, #32123, #30718, #38507, #41496, #12346, #19152, #25332, #12771, #28926, #28711, #11359, #2986, #4766, #41923, #9156, #22133, #14561, #15978, #35105, #5966, #41705, #9372, #18940, #25752, #38718, #20935, #1583, #27535, #853, #38928, #32960, #10425, #13396, #10210, #17016, #29557, #19777, #32742, #19995, #23179, #36144, #6387, #7237, #7016, #26589, #10005, #16393, #26377, #29128, #29338, #19565, #36367, #16188, #4, #22763, #39329, #32335, #20207, #32536, #13826, #421, #3610, #3826, #12984, #25965, #9804, #33168, #16806, #35738, #16602, #208, #29768, #9588, #13188, #26176, #19360, #6599, #39126, #628, #22968, #35937, #22546, #13605, #35529, #39547, #23402, #6802, #3202, #4033, #29979, #26807, #24043, #11261, #14045, #36577, #30826, #30615, #5082, #14871, #1279, #27017, #33815, #23831, #4468, #20631, #37419, #1482, #37213, #21043, #14248, #40190, #14459, #27432, #17235, #11459, #8277, #11060, #7657, #20841, #24450, #34021, #30408, #33609, #1686, #1070, #4875, #17450, #21252, #24244, #7874, #17853, #27631, #27226, #34221, #31034, #40603, #40400, #36796, #37012, #18061, #4670, #39980, #17650, #8069, #1889, #14670, #39771, #10640, #30195, #23618, #7444, #20419, #33384, #4251, #10844, #15507, #28462, #41027, #12519, #35270, #41663, #2097, #31862, #15299, #28255, #31444, #9112, #2522, #41240, #22090, #25075, #24664, #34848, #37831, #5291, #34637, #18477, #18897, #21659, #25502, #8902, #2732, #31235, #2314, #31655, #40812, #15716, #5502, #11665, #15081, #28045, #19111, #11878, #35063, #12084, #24870, #34431, #41449, #18264, #2945, #37625, #38467, #5924, #32076, #25283, #38039, #27838, #21873, #9330, #8686, #5716, #18693, #12299, #22295, #38250, #28669, #6130, #8479, #21458, #23355, #6561, #3778, #25710, #29088, #13145, #9761, #41880, #22929, #6973, #26133, #16350, #16558, #36317, #19527, #16763, #19317, #32294, #16150, #19947, #28883, #3159, #42087, #7190, #12940, #23134, #29293, #25920, #22502, #29510, #35487, #33122, #12730, #29724, #36101, #20162, #13356, #165, #15936, #35698, #587, #38883, #39087, #22720, #380, #10378, #32497, #3364, #32913, #13560, #26546, #38672, #9968, #39504, #9544, #35895, #6759, #19732, #6344, #32702, #3562, #26338, #39286, #10166, #11413, #7604, #33967, #7395, #20368, #4202, #8022, #7825, #36964, #23574, #17803, #14620, #17396, #13993, #27174, #30776, #27382, #36742, #39931, #37170, #33333, #40355, #10793, #1637, #17602, #14198, #11219, #4827, #20582, #27591, #37369, #40559, #20797, #30145, #23777, #24400, #40140, #17184, #33557, #33768, #8223, #24202, #23994, #4622, #36530, #21200, #4418, #20996, #3987, #11007, #30567, #1433, #14407, #1023, #16969, #29936, #807, #26967, #13779, #30357, #1228, #26759, #39722, #10593, #5450, #28411, #31395, #30987, #41191, #2047, #11617, #40974, #24824, #25233, #27995, #5874, #15245, #38197, #37574, #37783, #37989, #5030, #9061, #11827, #8852, #25028, #24608, #18846, #2680, #18427, #15030, #28205, #31805, #15456, #8640, #21612, #22037, #8427, #41400, #34587, #15666, #5664, #2262, #12248, #35012, #12036, #28622, #25450, #41611, #21826, #18219, #34798, #12466, #18642, #21406, #31607, #2472, #38411, #9276, #34170, #18010, #34383, #1844, #14823, #27790, #40760, #5243, #31187, #9915, #22873, #35428, #6909, #29661, #36041, #38618, #26281, #9704, #22665, #25863, #3507, #39030, #35641, #16499, #19474, #19055, #29233, #32237, #41827, #29036, #12885, #13299, #16097, #19884, #3305, #39230, #25657, #38827, #26073, #35214, #10111, #42033, #6076, #9485, #22448, #13498, #6290, #29448, #6506, #19264, #28827, #35840, #12678, #39442, #32025, #32850, #319, #26486, #19671, #32442, #22242, #16293, #3715, #3106, #109, #13089, #6702, #16703, #32643, #23075, #526, #2891, #15883, #17752, #961, #40296, #20099, #23511, #7548, #4140, #36253, #17337, #1376, #20523, #10735, #10949, #30724, #13928, #11166, #13716, #26695, #10528, #14352, #36684, #23935, #39657, #7126, #27330, #1170, #1588, #27543, #26908, #36473, #4356, #7336, #17124, #33275, #7971, #14139, #7766, #33714, #39873, #23720, #30088, #24150, #20739, #37119, #23288, #20306, #30299, #33495, #27114, #40083, #36904, #4565, #17542, #30508, #20940, #33911, #4771, #14566, #33062, #10315, #3929, #16909, #29877, #744, #31755, #5822, #21772, #30936, #12195, #24349, #18795, #34537, #8378, #34120, #25188, #18374, #27736, #5613, #15407, #37733, #28359, #38148, #1794, #9006, #8801, #2625, #40705, #34744, #41345, #2207, #41138, #15611, #31345, #8591, #21563, #18587, #11985, #24978, #37318, #21984, #37939, #34953, #40917, #5193, #15187, #17958, #34331, #21357, #40507, #4978, #14775, #11562, #28150, #21146, #11364, #18169, #8170, #31550, #5396, #2419, #24555, #37521, #31138, #1994, #14978, #27944, #11774, #24770, #33073, #36053, #13510, #26498, #19897, #29673, #538, #3939, #3728, #16712, #6919, #754, #32862, #39668, #36483, #16921, #36266, #39453, #20110, #29887, #10328, #13726, #26706, #10542, #23521, #20222, #4481, #14475, #26821, #39789, #27242, #17665, #24060, #27447, #10654, #7885, #29785, #33185, #17249, #13839, #3842, #27032, #11074, #30211, #20435, #20647, #40416, #23633, #20853, #23418, #36383, #4049, #37027, #23849, #10861, #39563, #33827, #30631, #33402, #29997, #1088, #4685, #1292, #36596, #7461, #1496, #7250, #14264, #4265, #11274, #33625, #14059, #40206, #24257, #39994, #37227, #19435, #32405, #36814, #17034, #7674, #16822, #17463, #867, #30422, #649, #13622, #26605, #10441, #24883, #27644, #8912, #37638, #25089, #38053, #31250, #37846, #8701, #21677, #21265, #34860, #15517, #21884, #24464, #12097, #8494, #21472, #11679, #31458, #34650, #34444, #2327, #5305, #4889, #15097, #18076, #40614, #14882, #40827, #41251, #1900, #5730, #2112, #18707, #11472, #24677, #11892, #21059, #31666, #27850, #34035, #37434, #8289, #41463, #34236, #15314, #18278, #5097, #14686, #5517, #31048, #25297, #17868, #2533, #28269, #12314, #18489, #28057, #28474, #8082, #30842, #1704, #41039, #16160, #6356, #19330, #6571, #38896, #9775, #35075, #35907, #22732, #13157, #38685, #2958, #42099, #15728, #32090, #6145, #22939, #2745, #28683, #9342, #25932, #18908, #6773, #19125, #29524, #29100, #32303, #35709, #41674, #12530, #25514, #19746, #12952, #38479, #3172, #15947, #19536, #38260, #28897, #41893, #5935, #22307, #35282, #32507, #12742, #25722, #9124, #3378, #22104, #16363, #29306, #9556, #31875, #178, #22513, #35498, #26145, #39096, #9977, #32713, #3576, #16570, #392, #13367, #29949, #13575, #20385, #10395, #33138, #7205, #24013, #17201, #23797, #7624, #822, #26775, #4001, #40160, #36761, #27194, #39300, #23369, #33351, #13795, #29736, #23587, #39740, #26559, #600, #36335, #20177, #39516, #16986, #36983, #36115, #30376, #36546, #10608, #11027, #7413, #17620, #33786, #20599, #16778 ),
 ( #4219, #30162, #26984, #26349, #1039, #14013, #6987, #39946, #10811, #33575, #32929, #4436, #10180, #17417, #23147, #1246, #14215, #7842, #19963, #20813, #3793, #4642, #30585, #1454, #30796, #11233, #5471, #5261, #21845, #31626, #18030, #1655, #8448, #40574, #21221, #37388, #12055, #18236, #11845, #37802, #31007, #14841, #34192, #28225, #24844, #15266, #27403, #11429, #21428, #1861, #17823, #11635, #27810, #14642, #27607, #24421, #8245, #5051, #40782, #25047, #24216, #18448, #24631, #37595, #41212, #34401, #5687, #34819, #8657, #4844, #38009, #40373, #18661, #31207, #2067, #8040, #8873, #15052, #28017, #21629, #31417, #40996, #2283, #14428, #34607, #37185, #21014, #33990, #31828, #25885, #3329, #6311, #3126, #9936, #22468, #12700, #25679, #12907, #16117, #29058, #41419, #130, #42053, #19493, #2913, #9297, #19286, #18865, #13112, #32259, #9080, #38639, #12485, #38848, #2491, #25469, #38434, #12268, #2699, #15686, #9726, #22059, #5893, #15476, #22686, #28430, #9507, #35662, #22262, #38219, #6525, #25253, #35030, #28848, #32463, #28642, #41631, #16317, #35450, #22894, #19698, #6096, #35235, #29258, #19077, #32044, #15902, #26095, #39053, #35859, #6723, #41847, #33085, #39468, #4382, #987, #33519, #3528, #29688, #26723, #20122, #36067, #29900, #36279, #32876, #6934, #16725, #552, #3739, #19911, #1193, #342, #36707, #770, #13522, #17361, #23319, #23958, #40105, #13955, #23099, #30322, #16524, #10973, #39685, #26510, #26305, #14160, #10555, #10342, #39895, #7571, #13743, #20544, #27136, #7153, #36925, #26932, #7788, #3952, #10757, #32666, #36497, #33298, #29472, #23536, #7358, #20331, #23740, #4164, #17145, #13320, #39250, #30110, #10132, #16933, #27561, #24578, #40322, #14588, #30744, #5418, #27348, #11186, #33936, #8395, #1400, #18396, #1608, #12007, #40728, #30957, #34354, #24169, #37139, #31368, #11584, #18187, #2016, #24370, #21166, #40528, #34557, #31156, #21583, #33736, #17773, #14793, #8192, #7992, #17980, #37340, #20963, #4795, #11385, #34138, #4999, #1813, #2230, #30531, #24792, #27757, #37541, #15210, #21375, #24999, #28174, #15000, #5212, #41160, #4588, #37961, #27965, #40941, #14375, #20763, #11797, #37755, #8611, #17567, #6048, #38800, #22636, #12216, #35612, #19237, #81, #38167, #32209, #9673, #12649, #9454, #16265, #28796, #19026, #31995, #3074, #22421, #35398, #5634, #6475, #6263, #25835, #9244, #15635, #25628, #28380, #2647, #18815, #19445, #15426, #41367, #22008, #38588, #31574, #32413, #31775, #13061, #41795, #2861, #16067, #25205, #9028, #34981, #3279, #29009, #5844, #15851, #28592, #42004, #8822, #41579, #12433, #18610, #25417, #38382, #12854, #22214, #35182, #21795, #29205, #34765, #26044, #2442, #32820, #32614, #20281, #22843, #29419, #23257, #10500, #13272, #35812, #30058, #29848, #4328, #14115, #500, #26255, #33036, #23047, #3690, #19853, #13471, #26880, #289, #39203, #10083, #933, #714, #13686, #16470, #10710, #7524, #10288, #6879, #20074, #23696, #33247, #29635, #16678, #13899, #36016, #4111, #26456, #36660, #23483, #7097, #17095, #39849, #39411, #20497, #30274, #33466, #26667, #36223, #3902, #17313, #16884, #39627, #36446, #7309, #1146, #39006, #9887, #6674, #19646, #3479, #14541, #1967, #14952, #8148, #14752, #27708, #40682, #40271, #11747, #34509, #40892, #1353, #31112, #27514, #40482, #30695, #8352, #1770, #11336, #21331, #24324, #23909, #34094, #37092, #4539, #33887, #17725, #18142, #20914, #24742, #21123, #27918, #30484, #1563, #30911, #40057, #37708, #4748, #10925, #14326, #27306, #18346, #11140, #34306, #37293, #24122, #33689, #11538, #17518, #2179, #36877, #8565, #5169, #31320, #24530, #4952, #27090, #17934, #21541, #7948, #37497, #5367, #7738, #20712, #21953, #34927, #22369, #12799, #19185, #22583, #5798, #3021, #24953, #28333, #12383, #8981, #41111, #22168, #6211, #25369, #15583, #15796, #35558, #5999, #34717, #28955, #25782, #28542, #25158, #38328, #41951, #38538, #18770, #31729, #32157, #18557, #9405, #2597, #38749, #28743, #9191, #35347, #16013, #41530, #9619, #6420, #19392, #18975, #41319, #35137, #32364, #31942, #2394, #2813, #41739, #15161, #28125, #12595, #25577, #5586, #11959, #37913, #8771, #21744, #31526, #15385, #12167, #38122, #16422, #30007, #10665, #17044, #19590, #7261, #32771, #3638, #6829, #26616, #20021, #16625, #39577, #449, #33, #10236, #13219, #22793, #10035, #35966, #36394, #39153, #880, #26406, #20233, #6627, #19801, #7043, #16211, #33195, #22995, #29155, #32563, #3430, #36608, #29369, #10452, #29585, #237, #9835, #16832, #35766, #20447, #13014, #13850, #23428, #7473, #660, #13420, #3228, #39356, #26831, #26205, #23205, #36172, #29795, #39800, #32986, #3853, #4060, #23646, #25994, #38959, #13633, #21280, #1099, #4492, #30645, #27256, #17261, #40426, #24477, #1509, #33838, #34045, #41429, #37038, #34249, #36825, #7686, #33637, #37446, #37240, #14276, #14070, #17475, #30434, #4901, #40006, #20659, #33413, #17882, #4278, #27460, #30855, #40217, #27043, #14698, #30222, #23861, #17678, #1715, #1303, #10874, #8301, #24270, #12278, #9091, #7897, #11088, #11285, #24072, #20867, #4697, #31060, #8094, #27656, #40627, #14489, #21072, #11487, #5109, #18088, #1912, #15486, #28440, #25262, #38229, #25481, #19296, #25688, #22272, #38445, #6107, #19087, #35245, #9307, #32678, #31841, #26106, #32270, #32055, #6735, #12710, #13333, #29484, #3339, #12495, #35870, #5902, #354, #16128, #2923, #15696, #19709, #42062, #15912, #29269, #39064, #3137, #9948, #3540, #28859, #16534, #32475, #26315, #41859, #16327, #22906, #25895, #22697, #39262, #12917, #29068, #38861, #142, #35675, #6538, #18876, #22070, #19504, #35041, #22479, #38650, #9737, #41643, #9517, #35461, #2710, #28650, #6321, #13124, #39907, #32888, #7800, #33096, #1411, #30122, #20342, #23752, #16737, #563, #26521, #20775, #26945, #29700, #33309, #20136, #10769, #10142, #3963, #30542, #4176, #16943, #3752, #36938, #998, #39480, #17372, #27148, #7369, #40115, #23972, #13533, #33745, #20557, #14385, #10354, #33532, #10984, #13966, #36717, #17578, #7582, #17159, #4394, #30332, #1205, #14172, #6947, #4599, #27362, #23110, #10568, #29911, #36078, #23330, #781, #13756, #19922, #36291, #7165, #26735, #39695, #23548, #36507, #21176, #31585, #18199, #8408, #11807, #4805, #30756, #14598, #8831, #15010, #17784, #21385, #8203, #40955, #40334, #34152, #5010, #8003, #40539, #11395, #24803, #1619, #27572, #11197, #37765, #24181, #34365, #8620, #17991, #33946, #21593, #37151, #24380, #24590, #34567, #37349, #20973, #31377, #31167, #5646, #15438, #1825, #30968, #5223, #14804, #27769, #40739, #37971, #2027, #5429, #18407, #11595, #37555, #27974, #12017, #2242, #41171, #15222, #28184, #25009, #21806, #34776, #18621, #2452, #28603, #31787, #12447, #25430, #41590, #2659, #39014, #38177, #32422, #25639, #38393, #13070, #19037, #19654, #35822, #9684, #18826, #90, #12227, #35622, #41806, #9255, #34992, #42014, #5856, #3489, #25215, #26055, #6485, #32623, #25845, #12660, #28392, #6059, #9896, #22225, #38600, #35193, #12865, #22852, #32006, #2872, #19455, #6684, #3288, #41378, #15863, #16274, #9042, #28809, #9465, #22431, #22019, #35409, #29215, #6273, #19248, #29018, #15645, #32219, #3085, #16077, #38810, #22647, #20505, #20289, #7319, #36026, #30283, #27099, #29858, #26466, #39637, #1156, #39857, #7107, #10297, #7533, #19863, #10717, #23266, #14124, #30068, #26676, #23705, #4338, #20082, #40067, #7748, #17322, #33255, #508, #36234, #10934, #10511, #3699, #33046, #4120, #23918, #36669, #36455, #17105, #6888, #36886, #3911, #33475, #20723, #23492, #943, #13909, #26890, #29644, #33699, #16479, #29430, #32830, #300, #16892, #723, #13696, #13281, #26264, #39212, #10093, #23057, #16688, #13480, #39421, #11150, #1574, #27524, #31122, #14551, #27928, #4962, #1976, #24134, #40491, #14762, #17528, #18151, #11347, #30493, #37102, #7958, #5379, #20924, #8361, #40900, #1362, #4757, #17943, #24333, #33898, #21131, #37302, #17734, #30707, #8157, #34103, #30921, #1779, #24754, #14336, #14961, #27720, #40691, #11757, #11546, #18357, #21549, #21342, #24539, #37720, #27315, #34520, #37505, #34315, #40281, #8575, #5179, #4549, #7668, #17458, #39783, #30418, #14259, #3837, #27237, #10856, #33822, #29780, #23840, #1288, #4260, #1082, #7881, #20430, #10649, #23627, #36808, #14054, #27026, #39341, #40199, #39989, #11070, #862, #7245, #17244, #20006, #36378, #10435, #24053, #7028, #32970, #13616, #30206, #23190, #37023, #23413, #4681, #33394, #36591, #20642, #16815, #642, #26599, #20849, #33621, #39558, #7454, #20218, #4477, #433, #33178, #4044, #10219, #17026, #29990, #17660, #13834, #26815, #13406, #26389, #36154, #24674, #2108, #24460, #24253, #11888, #14468, #21054, #14878, #15092, #4883, #27443, #21670, #21466, #38048, #5725, #34233, #17864, #37634, #14679, #37429, #11469, #28264, #34441, #28054, #24880, #5091, #31043, #8285, #2324, #31247, #1700, #15311, #8909, #41248, #30835, #34647, #18072, #1897, #27847, #37840, #5300, #40823, #8697, #11675, #40410, #8491, #40611, #8076, #21261, #18274, #5512, #41036, #12091, #18486, #31454, #34030, #25085, #21881, #1491, #34857, #30625, #11270, #27641, #37223, #9974, #31871, #25929, #32087, #15725, #25294, #32301, #38257, #35903, #2529, #32505, #38893, #22937, #16158, #2953, #18704, #38475, #3374, #2740, #15944, #18904, #3167, #13155, #25511, #9339, #9772, #16361, #22729, #26142, #22303, #6569, #28469, #28678, #28894, #12527, #15514, #25718, #35706, #41888, #19120, #19326, #39094, #35277, #19534, #22100, #35072, #41671, #29304, #22511, #9553, #9120, #173, #31663, #12738, #6141, #38681, #41460, #42096, #35495, #6354, #12309, #5932, #12950, #29096, #20596, #20381, #16981, #1035, #36758, #39513, #30372, #40155, #7619, #39735, #32923, #13572, #1243, #818, #36112, #23366, #23584, #33571, #30159, #26771, #36543, #26346, #4432, #36329, #23791, #17412, #29945, #7407, #33347, #14211, #13792, #6985, #7201, #4215, #27189, #14009, #10606, #17198, #39295, #11022, #20174, #24009, #6770, #26980, #39943, #10807, #19743, #19960, #32711, #3574, #16567, #23145, #29522, #33133, #3997, #10391, #388, #13365, #10177, #3790, #16773, #29733, #596, #26556, #14421, #1651, #27603, #28010, #30790, #8652, #18023, #40991, #40369, #11425, #40776, #7839, #11840, #14636, #20809, #11230, #24214, #28219, #8036, #2061, #8240, #33984, #1451, #8442, #27399, #12048, #33782, #21624, #24838, #41207, #34396, #21214, #36979, #24415, #34601, #21009, #34186, #37182, #21419, #31409, #37383, #5044, #37796, #5464, #18442, #2278, #31002, #15261, #4639, #4841, #1856, #14836, #17617, #27804, #30581, #24624, #37590, #5256, #17817, #18231, #31201, #28424, #41413, #25247, #29051, #28842, #15898, #2486, #38841, #35656, #38427, #35025, #6091, #9717, #6303, #15679, #18860, #16110, #12262, #19280, #31821, #22680, #38633, #35230, #32253, #12900, #28637, #6519, #16310, #25879, #41841, #9076, #2692, #5887, #19487, #31621, #15470, #38212, #12692, #5681, #32456, #41623, #29250, #2906, #19069, #9500, #22051, #12479, #25464, #3321, #25673, #9291, #32039, #22257, #22462, #25041, #35443, #3119, #34812, #42048, #124, #38004, #8865, #21840, #13102, #26712, #26088, #7146, #39678, #6928, #6717, #36489, #39046, #3522, #39461, #10547, #29465, #9930, #4156, #3944, #20537, #30315, #16719, #334, #20116, #39244, #19903 ) ),
 .UNSPECIFIED., .F., .F., .T. ) 
 B_SPLINE_SURFACE_WITH_KNOTS ( ( 2, 2 ),
 ( 3, 2, 2, 2, 2, 2, 2, 2, 2, 2, 2, 2, 2, 2, 2, 2, 2, 2, 2, 2, 2, 2, 2, 2, 2, 2, 2, 2, 2, 2, 2, 2, 2, 2, 2, 2, 2, 2, 2, 2, 2, 2, 2, 2, 2, 2, 2, 2, 2, 2, 2, 2, 2, 2, 2, 2, 2, 2, 2, 2, 2, 2, 2, 2, 2, 2, 2, 2, 2, 2, 2, 2, 2, 2, 2, 2, 2, 2, 2, 2, 2, 2, 2, 2, 2, 2, 2, 2, 2, 2, 2, 2, 2, 2, 2, 2, 2, 2, 2, 2, 2, 2, 2, 2, 2, 2, 2, 2, 2, 2, 2, 2, 2, 2, 2, 2, 2, 2, 2, 2, 2, 2, 2, 2, 2, 2, 2, 2, 2, 2, 2, 2, 2, 2, 2, 2, 2, 2, 2, 2, 2, 2, 2, 2, 2, 2, 2, 2, 2, 2, 2, 2, 2, 2, 2, 2, 2, 2, 2, 2, 2, 2, 2, 2, 2, 2, 2, 2, 2, 2, 2, 2, 2, 2, 2, 2, 2, 2, 2, 2, 2, 2, 2, 2, 2, 2, 2, 2, 2, 2, 2, 2, 2, 2, 2, 2, 2, 2, 2, 2, 2, 2, 2, 2, 2, 2, 2, 2, 2, 2, 2, 2, 2, 2, 2, 2, 2, 2, 2, 2, 2, 2, 2, 2, 2, 2, 2, 2, 2, 2, 2, 2, 2, 2, 2, 2, 2, 2, 2, 2, 2, 2, 2, 2, 2, 2, 2, 2, 2, 2, 2, 2, 2, 2, 2, 2, 2, 2, 2, 2, 2, 2, 2, 2, 2, 2, 2, 2, 2, 2, 2, 2, 2, 2, 2, 2, 2, 2, 2, 2, 2, 2, 2, 2, 2, 2, 2, 2, 2, 2, 2, 2, 2, 2, 2, 2, 2, 2, 2, 2, 2, 2, 2, 2, 2, 2, 2, 2, 2, 2, 2, 2, 2, 2, 2, 2, 2, 2, 2, 2, 2, 2, 2, 2, 2, 2, 2, 2, 2, 2, 2, 2, 2, 2, 2, 2, 2, 2, 2, 2, 2, 2, 2, 2, 2, 2, 2, 2, 2, 2, 2, 2, 2, 2, 2, 2, 2, 2, 2, 2, 2, 2, 2, 2, 2, 2, 2, 2, 2, 2, 2, 2, 2, 2, 2, 2, 2, 2, 2, 2, 2, 2, 2, 2, 2, 2, 2, 2, 2, 2, 2, 2, 2, 2, 2, 2, 2, 2, 2, 2, 2, 2, 2, 2, 2, 2, 2, 2, 2, 2, 2, 2, 2, 2, 2, 2, 2, 2, 2, 2, 2, 2, 2, 2, 2, 2, 2, 2, 2, 2, 2, 2, 2, 2, 2, 2, 2, 2, 2, 2, 2, 2, 2, 2, 2, 2, 2, 2, 2, 2, 2, 2, 2, 2, 2, 2, 2, 2, 2, 2, 2, 2, 2, 2, 2, 2, 2, 2, 2, 2, 2, 2, 2, 2, 2, 2, 2, 2, 2, 2, 2, 2, 2, 2, 2, 2, 2, 2, 2, 2, 2, 2, 2, 2, 2, 2, 2, 2, 2, 2, 2, 2, 2, 2, 2, 2, 2, 2, 2, 2, 2, 2, 2, 2, 2, 2, 2, 2, 2, 2, 2, 2, 2, 2, 2, 2, 2, 2, 2, 2, 2, 2, 2, 2, 2, 2, 2, 2, 2, 2, 2, 2, 2, 2, 2, 2, 2, 2, 2, 2, 2, 2, 2, 2, 2, 2, 2, 2, 2, 2, 2, 2, 2, 2, 2, 2, 2, 2, 2, 2, 2, 2, 2, 2, 2, 2, 2, 2, 2, 2, 2, 2, 2, 2, 2, 2, 2, 2, 2, 2, 2, 2, 2, 2, 2, 2, 2, 2, 2, 2, 2, 2, 2, 2, 2, 2, 2, 2, 2, 2, 2, 2, 2, 2, 2, 2, 2, 2, 2, 2, 2, 2, 2, 2, 2, 2, 2, 2, 2, 2, 2, 2, 2, 2, 2, 2, 2, 2, 2, 2, 2, 2, 2, 2, 2, 2, 2, 2, 2, 2, 2, 2, 2, 2, 2, 2, 2, 2, 2, 2, 2, 2, 2, 2, 2, 2, 2, 2, 2, 2, 2, 2, 2, 2, 2, 2, 2, 2, 2, 2, 2, 2, 2, 2, 2, 2, 2, 2, 2, 2, 2, 2, 2, 2, 2, 2, 2, 2, 2, 2, 2, 2, 2, 2, 2, 2, 2, 2, 2, 2, 2, 2, 2, 2, 2, 2, 2, 2, 2, 2, 3 ),
 ( 0.000000000000000000, 1.000000000000000000 ),
 ( 0.000000000000000000, 0.001388888888888888942, 0.002777777777777777884, 0.004166666666666666609, 0.005555555555555555768, 0.006944444444444444059, 0.008333333333333333218, 0.009722222222222222376, 0.01111111111111111154, 0.01250000000000000069, 0.01388888888888888812, 0.01527777777777777728, 0.01666666666666666644, 0.01805555555555555386, 0.01944444444444444475, 0.02083333333333333218, 0.02222222222222222307, 0.02361111111111111049, 0.02500000000000000139, 0.02638888888888888881, 0.02777777777777777624, 0.02916666666666666713, 0.03055555555555555455, 0.03194444444444444198, 0.03333333333333333287, 0.03472222222222222376, 0.03611111111111110772, 0.03749999999999999861, 0.03888888888888888951, 0.04027777777777778040, 0.04166666666666666435, 0.04305555555555555525, 0.04444444444444444614, 0.04583333333333333010, 0.04722222222222222099, 0.04861111111111111188, 0.05000000000000000278, 0.05138888888888888673, 0.05277777777777777762, 0.05416666666666666852, 0.05555555555555555247, 0.05694444444444444337, 0.05833333333333333426, 0.05972222222222222515, 0.06111111111111110911, 0.06250000000000000000, 0.06388888888888888395, 0.06527777777777778179, 0.06666666666666666574, 0.06805555555555554970, 0.06944444444444444753, 0.07083333333333333148, 0.07222222222222221544, 0.07361111111111111327, 0.07499999999999999722, 0.07638888888888889506, 0.07777777777777777901, 0.07916666666666666297, 0.08055555555555556080, 0.08194444444444444475, 0.08333333333333332871, 0.08472222222222222654, 0.08611111111111111049, 0.08749999999999999445, 0.08888888888888889228, 0.09027777777777777624, 0.09166666666666666019, 0.09305555555555555802, 0.09444444444444444198, 0.09583333333333333981, 0.09722222222222222376, 0.09861111111111110772, 0.1000000000000000056, 0.1013888888888888895, 0.1027777777777777735, 0.1041666666666666713, 0.1055555555555555552, 0.1069444444444444392, 0.1083333333333333370, 0.1097222222222222210, 0.1111111111111111049, 0.1125000000000000028, 0.1138888888888888867, 0.1152777777777777846, 0.1166666666666666685, 0.1180555555555555525, 0.1194444444444444503, 0.1208333333333333343, 0.1222222222222222182, 0.1236111111111111160, 0.1250000000000000000, 0.1263888888888888840, 0.1277777777777777679, 0.1291666666666666796, 0.1305555555555555636, 0.1319444444444444475, 0.1333333333333333315, 0.1347222222222222154, 0.1361111111111110994, 0.1375000000000000111, 0.1388888888888888951, 0.1402777777777777790, 0.1416666666666666630, 0.1430555555555555469, 0.1444444444444444309, 0.1458333333333333426, 0.1472222222222222265, 0.1486111111111111105, 0.1499999999999999944, 0.1513888888888888784, 0.1527777777777777901, 0.1541666666666666741, 0.1555555555555555580, 0.1569444444444444420, 0.1583333333333333259, 0.1597222222222222099, 0.1611111111111111216, 0.1625000000000000056, 0.1638888888888888895, 0.1652777777777777735, 0.1666666666666666574, 0.1680555555555555691, 0.1694444444444444531, 0.1708333333333333370, 0.1722222222222222210, 0.1736111111111111049, 0.1749999999999999889, 0.1763888888888889006, 0.1777777777777777846, 0.1791666666666666685, 0.1805555555555555525, 0.1819444444444444364, 0.1833333333333333204, 0.1847222222222222321, 0.1861111111111111160, 0.1875000000000000000, 0.1888888888888888840, 0.1902777777777777679, 0.1916666666666666796, 0.1930555555555555636, 0.1944444444444444475, 0.1958333333333333315, 0.1972222222222222154, 0.1986111111111110994, 0.2000000000000000111, 0.2013888888888888951, 0.2027777777777777790, 0.2041666666666666630, 0.2055555555555555469, 0.2069444444444444309, 0.2083333333333333426, 0.2097222222222222265, 0.2111111111111111105, 0.2124999999999999944, 0.2138888888888888784, 0.2152777777777777901, 0.2166666666666666741, 0.2180555555555555580, 0.2194444444444444420, 0.2208333333333333259, 0.2222222222222222099, 0.2236111111111111216, 0.2250000000000000056, 0.2263888888888888895, 0.2277777777777777735, 0.2291666666666666574, 0.2305555555555555691, 0.2319444444444444531, 0.2333333333333333370, 0.2347222222222222210, 0.2361111111111111049, 0.2374999999999999889, 0.2388888888888889006, 0.2402777777777777846, 0.2416666666666666685, 0.2430555555555555525, 0.2444444444444444364, 0.2458333333333333204, 0.2472222222222222321, 0.2486111111111111160, 0.2500000000000000000, 0.2513888888888888840, 0.2527777777777777679, 0.2541666666666666519, 0.2555555555555555358, 0.2569444444444444198, 0.2583333333333333592, 0.2597222222222222432, 0.2611111111111111271, 0.2625000000000000111, 0.2638888888888888951, 0.2652777777777777790, 0.2666666666666666630, 0.2680555555555555469, 0.2694444444444444309, 0.2708333333333333148, 0.2722222222222221988, 0.2736111111111111382, 0.2750000000000000222, 0.2763888888888889062, 0.2777777777777777901, 0.2791666666666666741, 0.2805555555555555580, 0.2819444444444444420, 0.2833333333333333259, 0.2847222222222222099, 0.2861111111111110938, 0.2874999999999999778, 0.2888888888888888618, 0.2902777777777778012, 0.2916666666666666852, 0.2930555555555555691, 0.2944444444444444531, 0.2958333333333333370, 0.2972222222222222210, 0.2986111111111111049, 0.2999999999999999889, 0.3013888888888888729, 0.3027777777777777568, 0.3041666666666666408, 0.3055555555555555802, 0.3069444444444444642, 0.3083333333333333481, 0.3097222222222222321, 0.3111111111111111160, 0.3125000000000000000, 0.3138888888888888840, 0.3152777777777777679, 0.3166666666666666519, 0.3180555555555555358, 0.3194444444444444198, 0.3208333333333333592, 0.3222222222222222432, 0.3236111111111111271, 0.3250000000000000111, 0.3263888888888888951, 0.3277777777777777790, 0.3291666666666666630, 0.3305555555555555469, 0.3319444444444444309, 0.3333333333333333148, 0.3347222222222221988, 0.3361111111111111382, 0.3375000000000000222, 0.3388888888888889062, 0.3402777777777777901, 0.3416666666666666741, 0.3430555555555555580, 0.3444444444444444420, 0.3458333333333333259, 0.3472222222222222099, 0.3486111111111110938, 0.3499999999999999778, 0.3513888888888888618, 0.3527777777777778012, 0.3541666666666666852, 0.3555555555555555691, 0.3569444444444444531, 0.3583333333333333370, 0.3597222222222222210, 0.3611111111111111049, 0.3624999999999999889, 0.3638888888888888729, 0.3652777777777777568, 0.3666666666666666408, 0.3680555555555555802, 0.3694444444444444642, 0.3708333333333333481, 0.3722222222222222321, 0.3736111111111111160, 0.3750000000000000000, 0.3763888888888888840, 0.3777777777777777679, 0.3791666666666666519, 0.3805555555555555358, 0.3819444444444444198, 0.3833333333333333592, 0.3847222222222222432, 0.3861111111111111271, 0.3875000000000000111, 0.3888888888888888951, 0.3902777777777777790, 0.3916666666666666630, 0.3930555555555555469, 0.3944444444444444309, 0.3958333333333333148, 0.3972222222222221988, 0.3986111111111111382, 0.4000000000000000222, 0.4013888888888889062, 0.4027777777777777901, 0.4041666666666666741, 0.4055555555555555580, 0.4069444444444444420, 0.4083333333333333259, 0.4097222222222222099, 0.4111111111111110938, 0.4124999999999999778, 0.4138888888888888618, 0.4152777777777778012, 0.4166666666666666852, 0.4180555555555555691, 0.4194444444444444531, 0.4208333333333333370, 0.4222222222222222210, 0.4236111111111111049, 0.4249999999999999889, 0.4263888888888888729, 0.4277777777777777568, 0.4291666666666666408, 0.4305555555555555802, 0.4319444444444444642, 0.4333333333333333481, 0.4347222222222222321, 0.4361111111111111160, 0.4375000000000000000, 0.4388888888888888840, 0.4402777777777777679, 0.4416666666666666519, 0.4430555555555555358, 0.4444444444444444198, 0.4458333333333333592, 0.4472222222222222432, 0.4486111111111111271, 0.4500000000000000111, 0.4513888888888888951, 0.4527777777777777790, 0.4541666666666666630, 0.4555555555555555469, 0.4569444444444444309, 0.4583333333333333148, 0.4597222222222221988, 0.4611111111111111382, 0.4625000000000000222, 0.4638888888888889062, 0.4652777777777777901, 0.4666666666666666741, 0.4680555555555555580, 0.4694444444444444420, 0.4708333333333333259, 0.4722222222222222099, 0.4736111111111110938, 0.4749999999999999778, 0.4763888888888888618, 0.4777777777777778012, 0.4791666666666666852, 0.4805555555555555691, 0.4819444444444444531, 0.4833333333333333370, 0.4847222222222222210, 0.4861111111111111049, 0.4874999999999999889, 0.4888888888888888729, 0.4902777777777777568, 0.4916666666666666408, 0.4930555555555555802, 0.4944444444444444642, 0.4958333333333333481, 0.4972222222222222321, 0.4986111111111111160, 0.5000000000000000000, 0.5013888888888888840, 0.5027777777777777679, 0.5041666666666666519, 0.5055555555555555358, 0.5069444444444444198, 0.5083333333333333037, 0.5097222222222221877, 0.5111111111111110716, 0.5124999999999999556, 0.5138888888888888395, 0.5152777777777777235, 0.5166666666666667185, 0.5180555555555556024, 0.5194444444444444864, 0.5208333333333333703, 0.5222222222222222543, 0.5236111111111111382, 0.5250000000000000222, 0.5263888888888889062, 0.5277777777777777901, 0.5291666666666666741, 0.5305555555555555580, 0.5319444444444444420, 0.5333333333333333259, 0.5347222222222222099, 0.5361111111111110938, 0.5374999999999999778, 0.5388888888888888618, 0.5402777777777777457, 0.5416666666666666297, 0.5430555555555555136, 0.5444444444444443976, 0.5458333333333332815, 0.5472222222222222765, 0.5486111111111111605, 0.5500000000000000444, 0.5513888888888889284, 0.5527777777777778123, 0.5541666666666666963, 0.5555555555555555802, 0.5569444444444444642, 0.5583333333333333481, 0.5597222222222222321, 0.5611111111111111160, 0.5625000000000000000, 0.5638888888888888840, 0.5652777777777777679, 0.5666666666666666519, 0.5680555555555555358, 0.5694444444444444198, 0.5708333333333333037, 0.5722222222222221877, 0.5736111111111110716, 0.5749999999999999556, 0.5763888888888888395, 0.5777777777777777235, 0.5791666666666667185, 0.5805555555555556024, 0.5819444444444444864, 0.5833333333333333703, 0.5847222222222222543, 0.5861111111111111382, 0.5875000000000000222, 0.5888888888888889062, 0.5902777777777777901, 0.5916666666666666741, 0.5930555555555555580, 0.5944444444444444420, 0.5958333333333333259, 0.5972222222222222099, 0.5986111111111110938, 0.5999999999999999778, 0.6013888888888888618, 0.6027777777777777457, 0.6041666666666666297, 0.6055555555555555136, 0.6069444444444443976, 0.6083333333333332815, 0.6097222222222222765, 0.6111111111111111605, 0.6125000000000000444, 0.6138888888888889284, 0.6152777777777778123, 0.6166666666666666963, 0.6180555555555555802, 0.6194444444444444642, 0.6208333333333333481, 0.6222222222222222321, 0.6236111111111111160, 0.6250000000000000000, 0.6263888888888888840, 0.6277777777777777679, 0.6291666666666666519, 0.6305555555555555358, 0.6319444444444444198, 0.6333333333333333037, 0.6347222222222221877, 0.6361111111111110716, 0.6374999999999999556, 0.6388888888888888395, 0.6402777777777777235, 0.6416666666666667185, 0.6430555555555556024, 0.6444444444444444864, 0.6458333333333333703, 0.6472222222222222543, 0.6486111111111111382, 0.6500000000000000222, 0.6513888888888889062, 0.6527777777777777901, 0.6541666666666666741, 0.6555555555555555580, 0.6569444444444444420, 0.6583333333333333259, 0.6597222222222222099, 0.6611111111111110938, 0.6624999999999999778, 0.6638888888888888618, 0.6652777777777777457, 0.6666666666666666297, 0.6680555555555555136, 0.6694444444444443976, 0.6708333333333332815, 0.6722222222222222765, 0.6736111111111111605, 0.6750000000000000444, 0.6763888888888889284, 0.6777777777777778123, 0.6791666666666666963, 0.6805555555555555802, 0.6819444444444444642, 0.6833333333333333481, 0.6847222222222222321, 0.6861111111111111160, 0.6875000000000000000, 0.6888888888888888840, 0.6902777777777777679, 0.6916666666666666519, 0.6930555555555555358, 0.6944444444444444198, 0.6958333333333333037, 0.6972222222222221877, 0.6986111111111110716, 0.6999999999999999556, 0.7013888888888888395, 0.7027777777777777235, 0.7041666666666667185, 0.7055555555555556024, 0.7069444444444444864, 0.7083333333333333703, 0.7097222222222222543, 0.7111111111111111382, 0.7125000000000000222, 0.7138888888888889062, 0.7152777777777777901, 0.7166666666666666741, 0.7180555555555555580, 0.7194444444444444420, 0.7208333333333333259, 0.7222222222222222099, 0.7236111111111110938, 0.7249999999999999778, 0.7263888888888888618, 0.7277777777777777457, 0.7291666666666666297, 0.7305555555555555136, 0.7319444444444443976, 0.7333333333333332815, 0.7347222222222222765, 0.7361111111111111605, 0.7375000000000000444, 0.7388888888888889284, 0.7402777777777778123, 0.7416666666666666963, 0.7430555555555555802, 0.7444444444444444642, 0.7458333333333333481, 0.7472222222222222321, 0.7486111111111111160, 0.7500000000000000000, 0.7513888888888888840, 0.7527777777777777679, 0.7541666666666666519, 0.7555555555555555358, 0.7569444444444444198, 0.7583333333333333037, 0.7597222222222221877, 0.7611111111111110716, 0.7624999999999999556, 0.7638888888888888395, 0.7652777777777777235, 0.7666666666666667185, 0.7680555555555556024, 0.7694444444444444864, 0.7708333333333333703, 0.7722222222222222543, 0.7736111111111111382, 0.7750000000000000222, 0.7763888888888889062, 0.7777777777777777901, 0.7791666666666666741, 0.7805555555555555580, 0.7819444444444444420, 0.7833333333333333259, 0.7847222222222222099, 0.7861111111111110938, 0.7874999999999999778, 0.7888888888888888618, 0.7902777777777777457, 0.7916666666666666297, 0.7930555555555555136, 0.7944444444444443976, 0.7958333333333332815, 0.7972222222222222765, 0.7986111111111111605, 0.8000000000000000444, 0.8013888888888889284, 0.8027777777777778123, 0.8041666666666666963, 0.8055555555555555802, 0.8069444444444444642, 0.8083333333333333481, 0.8097222222222222321, 0.8111111111111111160, 0.8125000000000000000, 0.8138888888888888840, 0.8152777777777777679, 0.8166666666666666519, 0.8180555555555555358, 0.8194444444444444198, 0.8208333333333333037, 0.8222222222222221877, 0.8236111111111110716, 0.8249999999999999556, 0.8263888888888888395, 0.8277777777777777235, 0.8291666666666667185, 0.8305555555555556024, 0.8319444444444444864, 0.8333333333333333703, 0.8347222222222222543, 0.8361111111111111382, 0.8375000000000000222, 0.8388888888888889062, 0.8402777777777777901, 0.8416666666666666741, 0.8430555555555555580, 0.8444444444444444420, 0.8458333333333333259, 0.8472222222222222099, 0.8486111111111110938, 0.8499999999999999778, 0.8513888888888888618, 0.8527777777777777457, 0.8541666666666666297, 0.8555555555555555136, 0.8569444444444443976, 0.8583333333333332815, 0.8597222222222222765, 0.8611111111111111605, 0.8625000000000000444, 0.8638888888888889284, 0.8652777777777778123, 0.8666666666666666963, 0.8680555555555555802, 0.8694444444444444642, 0.8708333333333333481, 0.8722222222222222321, 0.8736111111111111160, 0.8750000000000000000, 0.8763888888888888840, 0.8777777777777777679, 0.8791666666666666519, 0.8805555555555555358, 0.8819444444444444198, 0.8833333333333333037, 0.8847222222222221877, 0.8861111111111110716, 0.8874999999999999556, 0.8888888888888888395, 0.8902777777777777235, 0.8916666666666667185, 0.8930555555555556024, 0.8944444444444444864, 0.8958333333333333703, 0.8972222222222222543, 0.8986111111111111382, 0.9000000000000000222, 0.9013888888888889062, 0.9027777777777777901, 0.9041666666666666741, 0.9055555555555555580, 0.9069444444444444420, 0.9083333333333333259, 0.9097222222222222099, 0.9111111111111110938, 0.9124999999999999778, 0.9138888888888888618, 0.9152777777777777457, 0.9166666666666666297, 0.9180555555555555136, 0.9194444444444443976, 0.9208333333333332815, 0.9222222222222222765, 0.9236111111111111605, 0.9250000000000000444, 0.9263888888888889284, 0.9277777777777778123, 0.9291666666666666963, 0.9305555555555555802, 0.9319444444444444642, 0.9333333333333333481, 0.9347222222222222321, 0.9361111111111111160, 0.9375000000000000000, 0.9388888888888888840, 0.9402777777777777679, 0.9416666666666666519, 0.9430555555555555358, 0.9444444444444444198, 0.9458333333333333037, 0.9472222222222221877, 0.9486111111111110716, 0.9499999999999999556, 0.9513888888888888395, 0.9527777777777777235, 0.9541666666666667185, 0.9555555555555556024, 0.9569444444444444864, 0.9583333333333333703, 0.9597222222222222543, 0.9611111111111111382, 0.9625000000000000222, 0.9638888888888889062, 0.9652777777777777901, 0.9666666666666666741, 0.9680555555555555580, 0.9694444444444444420, 0.9708333333333333259, 0.9722222222222222099, 0.9736111111111110938, 0.9749999999999999778, 0.9763888888888888618, 0.9777777777777777457, 0.9791666666666666297, 0.9805555555555555136, 0.9819444444444443976, 0.9833333333333332815, 0.9847222222222222765, 0.9861111111111111605, 0.9875000000000000444, 0.9888888888888889284, 0.9902777777777778123, 0.9916666666666666963, 0.9930555555555555802, 0.9944444444444444642, 0.9958333333333333481, 0.9972222222222222321, 0.9986111111111111160, 1.000000000000000000 ),
 .UNSPECIFIED. ) 
 GEOMETRIC_REPRESENTATION_ITEM ( )  RATIONAL_B_SPLINE_SURFACE ( (
 ( 1.000000000000000000, 0.8660254037844387076, 1.000000000000000000, 0.8660254037844387076, 1.000000000000000000, 0.8660254037844387076, 1.000000000000000000, 0.8660254037844387076, 1.000000000000000000, 0.8660254037844387076, 1.000000000000000000, 0.8660254037844387076, 1.000000000000000000, 0.8660254037844387076, 1.000000000000000000, 0.8660254037844387076, 1.000000000000000000, 0.8660254037844387076, 1.000000000000000000, 0.8660254037844387076, 1.000000000000000000, 0.8660254037844387076, 1.000000000000000000, 0.8660254037844387076, 1.000000000000000000, 0.8660254037844387076, 1.000000000000000000, 0.8660254037844387076, 1.000000000000000000, 0.8660254037844387076, 1.000000000000000000, 0.8660254037844387076, 1.000000000000000000, 0.8660254037844387076, 1.000000000000000000, 0.8660254037844387076, 1.000000000000000000, 0.8660254037844387076, 1.000000000000000000, 0.8660254037844387076, 1.000000000000000000, 0.8660254037844387076, 1.000000000000000000, 0.8660254037844387076, 1.000000000000000000, 0.8660254037844387076, 1.000000000000000000, 0.8660254037844387076, 1.000000000000000000, 0.8660254037844387076, 1.000000000000000000, 0.8660254037844387076, 1.000000000000000000, 0.8660254037844387076, 1.000000000000000000, 0.8660254037844387076, 1.000000000000000000, 0.8660254037844387076, 1.000000000000000000, 0.8660254037844387076, 1.000000000000000000, 0.8660254037844387076, 1.000000000000000000, 0.8660254037844387076, 1.000000000000000000, 0.8660254037844387076, 1.000000000000000000, 0.8660254037844387076, 1.000000000000000000, 0.8660254037844387076, 1.000000000000000000, 0.8660254037844387076, 1.000000000000000000, 0.8660254037844387076, 1.000000000000000000, 0.8660254037844387076, 1.000000000000000000, 0.8660254037844387076, 1.000000000000000000, 0.8660254037844387076, 1.000000000000000000, 0.8660254037844387076, 1.000000000000000000, 0.8660254037844387076, 1.000000000000000000, 0.8660254037844387076, 1.000000000000000000, 0.8660254037844387076, 1.000000000000000000, 0.8660254037844387076, 1.000000000000000000, 0.8660254037844387076, 1.000000000000000000, 0.8660254037844387076, 1.000000000000000000, 0.8660254037844387076, 1.000000000000000000, 0.8660254037844387076, 1.000000000000000000, 0.8660254037844387076, 1.000000000000000000, 0.8660254037844387076, 1.000000000000000000, 0.8660254037844387076, 1.000000000000000000, 0.8660254037844387076, 1.000000000000000000, 0.8660254037844387076, 1.000000000000000000, 0.8660254037844387076, 1.000000000000000000, 0.8660254037844387076, 1.000000000000000000, 0.8660254037844387076, 1.000000000000000000, 0.8660254037844387076, 1.000000000000000000, 0.8660254037844387076, 1.000000000000000000, 0.8660254037844387076, 1.000000000000000000, 0.8660254037844387076, 1.000000000000000000, 0.8660254037844387076, 1.000000000000000000, 0.8660254037844387076, 1.000000000000000000, 0.8660254037844387076, 1.000000000000000000, 0.8660254037844387076, 1.000000000000000000, 0.8660254037844387076, 1.000000000000000000, 0.8660254037844387076, 1.000000000000000000, 0.8660254037844387076, 1.000000000000000000, 0.8660254037844387076, 1.000000000000000000, 0.8660254037844387076, 1.000000000000000000, 0.8660254037844387076, 1.000000000000000000, 0.8660254037844387076, 1.000000000000000000, 0.8660254037844387076, 1.000000000000000000, 0.8660254037844387076, 1.000000000000000000, 0.8660254037844387076, 1.000000000000000000, 0.8660254037844387076, 1.000000000000000000, 0.8660254037844387076, 1.000000000000000000, 0.8660254037844387076, 1.000000000000000000, 0.8660254037844387076, 1.000000000000000000, 0.8660254037844387076, 1.000000000000000000, 0.8660254037844387076, 1.000000000000000000, 0.8660254037844387076, 1.000000000000000000, 0.8660254037844387076, 1.000000000000000000, 0.8660254037844387076, 1.000000000000000000, 0.8660254037844387076, 1.000000000000000000, 0.8660254037844387076, 1.000000000000000000, 0.8660254037844387076, 1.000000000000000000, 0.8660254037844387076, 1.000000000000000000, 0.8660254037844387076, 1.000000000000000000, 0.8660254037844387076, 1.000000000000000000, 0.8660254037844387076, 1.000000000000000000, 0.8660254037844387076, 1.000000000000000000, 0.8660254037844387076, 1.000000000000000000, 0.8660254037844387076, 1.000000000000000000, 0.8660254037844387076, 1.000000000000000000, 0.8660254037844387076, 1.000000000000000000, 0.8660254037844387076, 1.000000000000000000, 0.8660254037844387076, 1.000000000000000000, 0.8660254037844387076, 1.000000000000000000, 0.8660254037844387076, 1.000000000000000000, 0.8660254037844387076, 1.000000000000000000, 0.8660254037844387076, 1.000000000000000000, 0.8660254037844387076, 1.000000000000000000, 0.8660254037844387076, 1.000000000000000000, 0.8660254037844387076, 1.000000000000000000, 0.8660254037844387076, 1.000000000000000000, 0.8660254037844387076, 1.000000000000000000, 0.8660254037844387076, 1.000000000000000000, 0.8660254037844387076, 1.000000000000000000, 0.8660254037844387076, 1.000000000000000000, 0.8660254037844387076, 1.000000000000000000, 0.8660254037844387076, 1.000000000000000000, 0.8660254037844387076, 1.000000000000000000, 0.8660254037844387076, 1.000000000000000000, 0.8660254037844387076, 1.000000000000000000, 0.8660254037844387076, 1.000000000000000000, 0.8660254037844387076, 1.000000000000000000, 0.8660254037844387076, 1.000000000000000000, 0.8660254037844387076, 1.000000000000000000, 0.8660254037844387076, 1.000000000000000000, 0.8660254037844387076, 1.000000000000000000, 0.8660254037844387076, 1.000000000000000000, 0.8660254037844387076, 1.000000000000000000, 0.8660254037844387076, 1.000000000000000000, 0.8660254037844387076, 1.000000000000000000, 0.8660254037844387076, 1.000000000000000000, 0.8660254037844387076, 1.000000000000000000, 0.8660254037844387076, 1.000000000000000000, 0.8660254037844387076, 1.000000000000000000, 0.8660254037844387076, 1.000000000000000000, 0.8660254037844387076, 1.000000000000000000, 0.8660254037844387076, 1.000000000000000000, 0.8660254037844387076, 1.000000000000000000, 0.8660254037844387076, 1.000000000000000000, 0.8660254037844387076, 1.000000000000000000, 0.8660254037844387076, 1.000000000000000000, 0.8660254037844387076, 1.000000000000000000, 0.8660254037844387076, 1.000000000000000000, 0.8660254037844387076, 1.000000000000000000, 0.8660254037844387076, 1.000000000000000000, 0.8660254037844387076, 1.000000000000000000, 0.8660254037844387076, 1.000000000000000000, 0.8660254037844387076, 1.000000000000000000, 0.8660254037844387076, 1.000000000000000000, 0.8660254037844387076, 1.000000000000000000, 0.8660254037844387076, 1.000000000000000000, 0.8660254037844387076, 1.000000000000000000, 0.8660254037844387076, 1.000000000000000000, 0.8660254037844387076, 1.000000000000000000, 0.8660254037844387076, 1.000000000000000000, 0.8660254037844387076, 1.000000000000000000, 0.8660254037844387076, 1.000000000000000000, 0.8660254037844387076, 1.000000000000000000, 0.8660254037844387076, 1.000000000000000000, 0.8660254037844387076, 1.000000000000000000, 0.8660254037844387076, 1.000000000000000000, 0.8660254037844387076, 1.000000000000000000, 0.8660254037844387076, 1.000000000000000000, 0.8660254037844387076, 1.000000000000000000, 0.8660254037844387076, 1.000000000000000000, 0.8660254037844387076, 1.000000000000000000, 0.8660254037844387076, 1.000000000000000000, 0.8660254037844387076, 1.000000000000000000, 0.8660254037844387076, 1.000000000000000000, 0.8660254037844387076, 1.000000000000000000, 0.8660254037844387076, 1.000000000000000000, 0.8660254037844387076, 1.000000000000000000, 0.8660254037844387076, 1.000000000000000000, 0.8660254037844387076, 1.000000000000000000, 0.8660254037844387076, 1.000000000000000000, 0.8660254037844387076, 1.000000000000000000, 0.8660254037844387076, 1.000000000000000000, 0.8660254037844387076, 1.000000000000000000, 0.8660254037844387076, 1.000000000000000000, 0.8660254037844387076, 1.000000000000000000, 0.8660254037844387076, 1.000000000000000000, 0.8660254037844387076, 1.000000000000000000, 0.8660254037844387076, 1.000000000000000000, 0.8660254037844387076, 1.000000000000000000, 0.8660254037844387076, 1.000000000000000000, 0.8660254037844387076, 1.000000000000000000, 0.8660254037844387076, 1.000000000000000000, 0.8660254037844387076, 1.000000000000000000, 0.8660254037844387076, 1.000000000000000000, 0.8660254037844387076, 1.000000000000000000, 0.8660254037844387076, 1.000000000000000000, 0.8660254037844387076, 1.000000000000000000, 0.8660254037844387076, 1.000000000000000000, 0.8660254037844387076, 1.000000000000000000, 0.8660254037844387076, 1.000000000000000000, 0.8660254037844387076, 1.000000000000000000, 0.8660254037844387076, 1.000000000000000000, 0.8660254037844387076, 1.000000000000000000, 0.8660254037844387076, 1.000000000000000000, 0.8660254037844387076, 1.000000000000000000, 0.8660254037844387076, 1.000000000000000000, 0.8660254037844387076, 1.000000000000000000, 0.8660254037844387076, 1.000000000000000000, 0.8660254037844387076, 1.000000000000000000, 0.8660254037844387076, 1.000000000000000000, 0.8660254037844387076, 1.000000000000000000, 0.8660254037844387076, 1.000000000000000000, 0.8660254037844387076, 1.000000000000000000, 0.8660254037844387076, 1.000000000000000000, 0.8660254037844387076, 1.000000000000000000, 0.8660254037844387076, 1.000000000000000000, 0.8660254037844387076, 1.000000000000000000, 0.8660254037844387076, 1.000000000000000000, 0.8660254037844387076, 1.000000000000000000, 0.8660254037844387076, 1.000000000000000000, 0.8660254037844387076, 1.000000000000000000, 0.8660254037844387076, 1.000000000000000000, 0.8660254037844387076, 1.000000000000000000, 0.8660254037844387076, 1.000000000000000000, 0.8660254037844387076, 1.000000000000000000, 0.8660254037844387076, 1.000000000000000000, 0.8660254037844387076, 1.000000000000000000, 0.8660254037844387076, 1.000000000000000000, 0.8660254037844387076, 1.000000000000000000, 0.8660254037844387076, 1.000000000000000000, 0.8660254037844387076, 1.000000000000000000, 0.8660254037844387076, 1.000000000000000000, 0.8660254037844387076, 1.000000000000000000, 0.8660254037844387076, 1.000000000000000000, 0.8660254037844387076, 1.000000000000000000, 0.8660254037844387076, 1.000000000000000000, 0.8660254037844387076, 1.000000000000000000, 0.8660254037844387076, 1.000000000000000000, 0.8660254037844387076, 1.000000000000000000, 0.8660254037844387076, 1.000000000000000000, 0.8660254037844387076, 1.000000000000000000, 0.8660254037844387076, 1.000000000000000000, 0.8660254037844387076, 1.000000000000000000, 0.8660254037844387076, 1.000000000000000000, 0.8660254037844387076, 1.000000000000000000, 0.8660254037844387076, 1.000000000000000000, 0.8660254037844387076, 1.000000000000000000, 0.8660254037844387076, 1.000000000000000000, 0.8660254037844387076, 1.000000000000000000, 0.8660254037844387076, 1.000000000000000000, 0.8660254037844387076, 1.000000000000000000, 0.8660254037844387076, 1.000000000000000000, 0.8660254037844387076, 1.000000000000000000, 0.8660254037844387076, 1.000000000000000000, 0.8660254037844387076, 1.000000000000000000, 0.8660254037844387076, 1.000000000000000000, 0.8660254037844387076, 1.000000000000000000, 0.8660254037844387076, 1.000000000000000000, 0.8660254037844387076, 1.000000000000000000, 0.8660254037844387076, 1.000000000000000000, 0.8660254037844387076, 1.000000000000000000, 0.8660254037844387076, 1.000000000000000000, 0.8660254037844387076, 1.000000000000000000, 0.8660254037844387076, 1.000000000000000000, 0.8660254037844387076, 1.000000000000000000, 0.8660254037844387076, 1.000000000000000000, 0.8660254037844387076, 1.000000000000000000, 0.8660254037844387076, 1.000000000000000000, 0.8660254037844387076, 1.000000000000000000, 0.8660254037844387076, 1.000000000000000000, 0.8660254037844387076, 1.000000000000000000, 0.8660254037844387076, 1.000000000000000000, 0.8660254037844387076, 1.000000000000000000, 0.8660254037844387076, 1.000000000000000000, 0.8660254037844387076, 1.000000000000000000, 0.8660254037844387076, 1.000000000000000000, 0.8660254037844387076, 1.000000000000000000, 0.8660254037844387076, 1.000000000000000000, 0.8660254037844387076, 1.000000000000000000, 0.8660254037844387076, 1.000000000000000000, 0.8660254037844387076, 1.000000000000000000, 0.8660254037844387076, 1.000000000000000000, 0.8660254037844387076, 1.000000000000000000, 0.8660254037844387076, 1.000000000000000000, 0.8660254037844387076, 1.000000000000000000, 0.8660254037844387076, 1.000000000000000000, 0.8660254037844387076, 1.000000000000000000, 0.8660254037844387076, 1.000000000000000000, 0.8660254037844387076, 1.000000000000000000, 0.8660254037844387076, 1.000000000000000000, 0.8660254037844387076, 1.000000000000000000, 0.8660254037844387076, 1.000000000000000000, 0.8660254037844387076, 1.000000000000000000, 0.8660254037844387076, 1.000000000000000000, 0.8660254037844387076, 1.000000000000000000, 0.8660254037844387076, 1.000000000000000000, 0.8660254037844387076, 1.000000000000000000, 0.8660254037844387076, 1.000000000000000000, 0.8660254037844387076, 1.000000000000000000, 0.8660254037844387076, 1.000000000000000000, 0.8660254037844387076, 1.000000000000000000, 0.8660254037844387076, 1.000000000000000000, 0.8660254037844387076, 1.000000000000000000, 0.8660254037844387076, 1.000000000000000000, 0.8660254037844387076, 1.000000000000000000, 0.8660254037844387076, 1.000000000000000000, 0.8660254037844387076, 1.000000000000000000, 0.8660254037844387076, 1.000000000000000000, 0.8660254037844387076, 1.000000000000000000, 0.8660254037844387076, 1.000000000000000000, 0.8660254037844387076, 1.000000000000000000, 0.8660254037844387076, 1.000000000000000000, 0.8660254037844387076, 1.000000000000000000, 0.8660254037844387076, 1.000000000000000000, 0.8660254037844387076, 1.000000000000000000, 0.8660254037844387076, 1.000000000000000000, 0.8660254037844387076, 1.000000000000000000, 0.8660254037844387076, 1.000000000000000000, 0.8660254037844387076, 1.000000000000000000, 0.8660254037844387076, 1.000000000000000000, 0.8660254037844387076, 1.000000000000000000, 0.8660254037844387076, 1.000000000000000000, 0.8660254037844387076, 1.000000000000000000, 0.8660254037844387076, 1.000000000000000000, 0.8660254037844387076, 1.000000000000000000, 0.8660254037844387076, 1.000000000000000000, 0.8660254037844387076, 1.000000000000000000, 0.8660254037844387076, 1.000000000000000000, 0.8660254037844387076, 1.000000000000000000, 0.8660254037844387076, 1.000000000000000000, 0.8660254037844387076, 1.000000000000000000, 0.8660254037844387076, 1.000000000000000000, 0.8660254037844387076, 1.000000000000000000, 0.8660254037844387076, 1.000000000000000000, 0.8660254037844387076, 1.000000000000000000, 0.8660254037844387076, 1.000000000000000000, 0.8660254037844387076, 1.000000000000000000, 0.8660254037844387076, 1.000000000000000000, 0.8660254037844387076, 1.000000000000000000, 0.8660254037844387076, 1.000000000000000000, 0.8660254037844387076, 1.000000000000000000, 0.8660254037844387076, 1.000000000000000000, 0.8660254037844387076, 1.000000000000000000, 0.8660254037844387076, 1.000000000000000000, 0.8660254037844387076, 1.000000000000000000, 0.8660254037844387076, 1.000000000000000000, 0.8660254037844387076, 1.000000000000000000, 0.8660254037844387076, 1.000000000000000000, 0.8660254037844387076, 1.000000000000000000, 0.8660254037844387076, 1.000000000000000000, 0.8660254037844387076, 1.000000000000000000, 0.8660254037844387076, 1.000000000000000000, 0.8660254037844387076, 1.000000000000000000, 0.8660254037844387076, 1.000000000000000000, 0.8660254037844387076, 1.000000000000000000, 0.8660254037844387076, 1.000000000000000000, 0.8660254037844387076, 1.000000000000000000, 0.8660254037844387076, 1.000000000000000000, 0.8660254037844387076, 1.000000000000000000, 0.8660254037844387076, 1.000000000000000000, 0.8660254037844387076, 1.000000000000000000, 0.8660254037844387076, 1.000000000000000000, 0.8660254037844387076, 1.000000000000000000, 0.8660254037844387076, 1.000000000000000000, 0.8660254037844387076, 1.000000000000000000, 0.8660254037844387076, 1.000000000000000000, 0.8660254037844387076, 1.000000000000000000, 0.8660254037844387076, 1.000000000000000000, 0.8660254037844387076, 1.000000000000000000, 0.8660254037844387076, 1.000000000000000000, 0.8660254037844387076, 1.000000000000000000, 0.8660254037844387076, 1.000000000000000000, 0.8660254037844387076, 1.000000000000000000, 0.8660254037844387076, 1.000000000000000000, 0.8660254037844387076, 1.000000000000000000, 0.8660254037844387076, 1.000000000000000000, 0.8660254037844387076, 1.000000000000000000, 0.8660254037844387076, 1.000000000000000000, 0.8660254037844387076, 1.000000000000000000, 0.8660254037844387076, 1.000000000000000000, 0.8660254037844387076, 1.000000000000000000, 0.8660254037844387076, 1.000000000000000000, 0.8660254037844387076, 1.000000000000000000, 0.8660254037844387076, 1.000000000000000000, 0.8660254037844387076, 1.000000000000000000, 0.8660254037844387076, 1.000000000000000000, 0.8660254037844387076, 1.000000000000000000, 0.8660254037844387076, 1.000000000000000000, 0.8660254037844387076, 1.000000000000000000, 0.8660254037844387076, 1.000000000000000000, 0.8660254037844387076, 1.000000000000000000, 0.8660254037844387076, 1.000000000000000000, 0.8660254037844387076, 1.000000000000000000, 0.8660254037844387076, 1.000000000000000000, 0.8660254037844387076, 1.000000000000000000, 0.8660254037844387076, 1.000000000000000000, 0.8660254037844387076, 1.000000000000000000, 0.8660254037844387076, 1.000000000000000000, 0.8660254037844387076, 1.000000000000000000, 0.8660254037844387076, 1.000000000000000000, 0.8660254037844387076, 1.000000000000000000, 0.8660254037844387076, 1.000000000000000000, 0.8660254037844387076, 1.000000000000000000, 0.8660254037844387076, 1.000000000000000000, 0.8660254037844387076, 1.000000000000000000, 0.8660254037844387076, 1.000000000000000000, 0.8660254037844387076, 1.000000000000000000, 0.8660254037844387076, 1.000000000000000000, 0.8660254037844387076, 1.000000000000000000, 0.8660254037844387076, 1.000000000000000000, 0.8660254037844387076, 1.000000000000000000, 0.8660254037844387076, 1.000000000000000000, 0.8660254037844387076, 1.000000000000000000, 0.8660254037844387076, 1.000000000000000000, 0.8660254037844387076, 1.000000000000000000, 0.8660254037844387076, 1.000000000000000000, 0.8660254037844387076, 1.000000000000000000, 0.8660254037844387076, 1.000000000000000000, 0.8660254037844387076, 1.000000000000000000, 0.8660254037844387076, 1.000000000000000000, 0.8660254037844387076, 1.000000000000000000, 0.8660254037844387076, 1.000000000000000000, 0.8660254037844387076, 1.000000000000000000, 0.8660254037844387076, 1.000000000000000000, 0.8660254037844387076, 1.000000000000000000, 0.8660254037844387076, 1.000000000000000000, 0.8660254037844387076, 1.000000000000000000, 0.8660254037844387076, 1.000000000000000000, 0.8660254037844387076, 1.000000000000000000, 0.8660254037844387076, 1.000000000000000000, 0.8660254037844387076, 1.000000000000000000, 0.8660254037844387076, 1.000000000000000000, 0.8660254037844387076, 1.000000000000000000, 0.8660254037844387076, 1.000000000000000000, 0.8660254037844387076, 1.000000000000000000, 0.8660254037844387076, 1.000000000000000000, 0.8660254037844387076, 1.000000000000000000, 0.8660254037844387076, 1.000000000000000000, 0.8660254037844387076, 1.000000000000000000, 0.8660254037844387076, 1.000000000000000000, 0.8660254037844387076, 1.000000000000000000, 0.8660254037844387076, 1.000000000000000000, 0.8660254037844387076, 1.000000000000000000, 0.8660254037844387076, 1.000000000000000000, 0.8660254037844387076, 1.000000000000000000, 0.8660254037844387076, 1.000000000000000000, 0.8660254037844387076, 1.000000000000000000, 0.8660254037844387076, 1.000000000000000000, 0.8660254037844387076, 1.000000000000000000, 0.8660254037844387076, 1.000000000000000000, 0.8660254037844387076, 1.000000000000000000, 0.8660254037844387076, 1.000000000000000000, 0.8660254037844387076, 1.000000000000000000, 0.8660254037844387076, 1.000000000000000000, 0.8660254037844387076, 1.000000000000000000, 0.8660254037844387076, 1.000000000000000000, 0.8660254037844387076, 1.000000000000000000, 0.8660254037844387076, 1.000000000000000000, 0.8660254037844387076, 1.000000000000000000, 0.8660254037844387076, 1.000000000000000000, 0.8660254037844387076, 1.000000000000000000, 0.8660254037844387076, 1.000000000000000000, 0.8660254037844387076, 1.000000000000000000, 0.8660254037844387076, 1.000000000000000000, 0.8660254037844387076, 1.000000000000000000, 0.8660254037844387076, 1.000000000000000000, 0.8660254037844387076, 1.000000000000000000, 0.8660254037844387076, 1.000000000000000000, 0.8660254037844387076, 1.000000000000000000, 0.8660254037844387076, 1.000000000000000000, 0.8660254037844387076, 1.000000000000000000, 0.8660254037844387076, 1.000000000000000000, 0.8660254037844387076, 1.000000000000000000, 0.8660254037844387076, 1.000000000000000000, 0.8660254037844387076, 1.000000000000000000, 0.8660254037844387076, 1.000000000000000000, 0.8660254037844387076, 1.000000000000000000, 0.8660254037844387076, 1.000000000000000000, 0.8660254037844387076, 1.000000000000000000, 0.8660254037844387076, 1.000000000000000000, 0.8660254037844387076, 1.000000000000000000, 0.8660254037844387076, 1.000000000000000000, 0.8660254037844387076, 1.000000000000000000, 0.8660254037844387076, 1.000000000000000000, 0.8660254037844387076, 1.000000000000000000, 0.8660254037844387076, 1.000000000000000000, 0.8660254037844387076, 1.000000000000000000, 0.8660254037844387076, 1.000000000000000000, 0.8660254037844387076, 1.000000000000000000, 0.8660254037844387076, 1.000000000000000000, 0.8660254037844387076, 1.000000000000000000, 0.8660254037844387076, 1.000000000000000000, 0.8660254037844387076, 1.000000000000000000, 0.8660254037844387076, 1.000000000000000000, 0.8660254037844387076, 1.000000000000000000, 0.8660254037844387076, 1.000000000000000000, 0.8660254037844387076, 1.000000000000000000, 0.8660254037844387076, 1.000000000000000000, 0.8660254037844387076, 1.000000000000000000, 0.8660254037844387076, 1.000000000000000000, 0.8660254037844387076, 1.000000000000000000, 0.8660254037844387076, 1.000000000000000000, 0.8660254037844387076, 1.000000000000000000, 0.8660254037844387076, 1.000000000000000000, 0.8660254037844387076, 1.000000000000000000, 0.8660254037844387076, 1.000000000000000000, 0.8660254037844387076, 1.000000000000000000, 0.8660254037844387076, 1.000000000000000000, 0.8660254037844387076, 1.000000000000000000, 0.8660254037844387076, 1.000000000000000000, 0.8660254037844387076, 1.000000000000000000, 0.8660254037844387076, 1.000000000000000000, 0.8660254037844387076, 1.000000000000000000, 0.8660254037844387076, 1.000000000000000000, 0.8660254037844387076, 1.000000000000000000, 0.8660254037844387076, 1.000000000000000000, 0.8660254037844387076, 1.000000000000000000, 0.8660254037844387076, 1.000000000000000000, 0.8660254037844387076, 1.000000000000000000, 0.8660254037844387076, 1.000000000000000000, 0.8660254037844387076, 1.000000000000000000, 0.8660254037844387076, 1.000000000000000000, 0.8660254037844387076, 1.000000000000000000, 0.8660254037844387076, 1.000000000000000000, 0.8660254037844387076, 1.000000000000000000, 0.8660254037844387076, 1.000000000000000000, 0.8660254037844387076, 1.000000000000000000, 0.8660254037844387076, 1.000000000000000000, 0.8660254037844387076, 1.000000000000000000, 0.8660254037844387076, 1.000000000000000000, 0.8660254037844387076, 1.000000000000000000, 0.8660254037844387076, 1.000000000000000000, 0.8660254037844387076, 1.000000000000000000, 0.8660254037844387076, 1.000000000000000000, 0.8660254037844387076, 1.000000000000000000, 0.8660254037844387076, 1.000000000000000000, 0.8660254037844387076, 1.000000000000000000, 0.8660254037844387076, 1.000000000000000000, 0.8660254037844387076, 1.000000000000000000, 0.8660254037844387076, 1.000000000000000000, 0.8660254037844387076, 1.000000000000000000, 0.8660254037844387076, 1.000000000000000000, 0.8660254037844387076, 1.000000000000000000, 0.8660254037844387076, 1.000000000000000000, 0.8660254037844387076, 1.000000000000000000, 0.8660254037844387076, 1.000000000000000000, 0.8660254037844387076, 1.000000000000000000, 0.8660254037844387076, 1.000000000000000000, 0.8660254037844387076, 1.000000000000000000, 0.8660254037844387076, 1.000000000000000000, 0.8660254037844387076, 1.000000000000000000, 0.8660254037844387076, 1.000000000000000000, 0.8660254037844387076, 1.000000000000000000, 0.8660254037844387076, 1.000000000000000000, 0.8660254037844387076, 1.000000000000000000, 0.8660254037844387076, 1.000000000000000000, 0.8660254037844387076, 1.000000000000000000, 0.8660254037844387076, 1.000000000000000000, 0.8660254037844387076, 1.000000000000000000, 0.8660254037844387076, 1.000000000000000000, 0.8660254037844387076, 1.000000000000000000, 0.8660254037844387076, 1.000000000000000000, 0.8660254037844387076, 1.000000000000000000, 0.8660254037844387076, 1.000000000000000000, 0.8660254037844387076, 1.000000000000000000, 0.8660254037844387076, 1.000000000000000000, 0.8660254037844387076, 1.000000000000000000, 0.8660254037844387076, 1.000000000000000000, 0.8660254037844387076, 1.000000000000000000, 0.8660254037844387076, 1.000000000000000000, 0.8660254037844387076, 1.000000000000000000, 0.8660254037844387076, 1.000000000000000000, 0.8660254037844387076, 1.000000000000000000, 0.8660254037844387076, 1.000000000000000000, 0.8660254037844387076, 1.000000000000000000, 0.8660254037844387076, 1.000000000000000000, 0.8660254037844387076, 1.000000000000000000, 0.8660254037844387076, 1.000000000000000000, 0.8660254037844387076, 1.000000000000000000, 0.8660254037844387076, 1.000000000000000000, 0.8660254037844387076, 1.000000000000000000, 0.8660254037844387076, 1.000000000000000000, 0.8660254037844387076, 1.000000000000000000, 0.8660254037844387076, 1.000000000000000000, 0.8660254037844387076, 1.000000000000000000, 0.8660254037844387076, 1.000000000000000000, 0.8660254037844387076, 1.000000000000000000, 0.8660254037844387076, 1.000000000000000000, 0.8660254037844387076, 1.000000000000000000, 0.8660254037844387076, 1.000000000000000000, 0.8660254037844387076, 1.000000000000000000, 0.8660254037844387076, 1.000000000000000000, 0.8660254037844387076, 1.000000000000000000, 0.8660254037844387076, 1.000000000000000000, 0.8660254037844387076, 1.000000000000000000, 0.8660254037844387076, 1.000000000000000000, 0.8660254037844387076, 1.000000000000000000, 0.8660254037844387076, 1.000000000000000000, 0.8660254037844387076, 1.000000000000000000, 0.8660254037844387076, 1.000000000000000000, 0.8660254037844387076, 1.000000000000000000, 0.8660254037844387076, 1.000000000000000000, 0.8660254037844387076, 1.000000000000000000, 0.8660254037844387076, 1.000000000000000000, 0.8660254037844387076, 1.000000000000000000, 0.8660254037844387076, 1.000000000000000000, 0.8660254037844387076, 1.000000000000000000, 0.8660254037844387076, 1.000000000000000000, 0.8660254037844387076, 1.000000000000000000, 0.8660254037844387076, 1.000000000000000000, 0.8660254037844387076, 1.000000000000000000, 0.8660254037844387076, 1.000000000000000000, 0.8660254037844387076, 1.000000000000000000, 0.8660254037844387076, 1.000000000000000000, 0.8660254037844387076, 1.000000000000000000, 0.8660254037844387076, 1.000000000000000000, 0.8660254037844387076, 1.000000000000000000, 0.8660254037844387076, 1.000000000000000000, 0.8660254037844387076, 1.000000000000000000, 0.8660254037844387076, 1.000000000000000000, 0.8660254037844387076, 1.000000000000000000, 0.8660254037844387076, 1.000000000000000000, 0.8660254037844387076, 1.000000000000000000, 0.8660254037844387076, 1.000000000000000000, 0.8660254037844387076, 1.000000000000000000, 0.8660254037844387076, 1.000000000000000000, 0.8660254037844387076, 1.000000000000000000, 0.8660254037844387076, 1.000000000000000000, 0.8660254037844387076, 1.000000000000000000, 0.8660254037844387076, 1.000000000000000000, 0.8660254037844387076, 1.000000000000000000, 0.8660254037844387076, 1.000000000000000000, 0.8660254037844387076, 1.000000000000000000, 0.8660254037844387076, 1.000000000000000000, 0.8660254037844387076, 1.000000000000000000, 0.8660254037844387076, 1.000000000000000000, 0.8660254037844387076, 1.000000000000000000, 0.8660254037844387076, 1.000000000000000000, 0.8660254037844387076, 1.000000000000000000, 0.8660254037844387076, 1.000000000000000000, 0.8660254037844387076, 1.000000000000000000, 0.8660254037844387076, 1.000000000000000000, 0.8660254037844387076, 1.000000000000000000, 0.8660254037844387076, 1.000000000000000000, 0.8660254037844387076, 1.000000000000000000, 0.8660254037844387076, 1.000000000000000000, 0.8660254037844387076, 1.000000000000000000, 0.8660254037844387076, 1.000000000000000000, 0.8660254037844387076, 1.000000000000000000, 0.8660254037844387076, 1.000000000000000000, 0.8660254037844387076, 1.000000000000000000, 0.8660254037844387076, 1.000000000000000000, 0.8660254037844387076, 1.000000000000000000, 0.8660254037844387076, 1.000000000000000000, 0.8660254037844387076, 1.000000000000000000, 0.8660254037844387076, 1.000000000000000000, 0.8660254037844387076, 1.000000000000000000, 0.8660254037844387076, 1.000000000000000000, 0.8660254037844387076, 1.000000000000000000, 0.8660254037844387076, 1.000000000000000000, 0.8660254037844387076, 1.000000000000000000, 0.8660254037844387076, 1.000000000000000000, 0.8660254037844387076, 1.000000000000000000, 0.8660254037844387076, 1.000000000000000000, 0.8660254037844387076, 1.000000000000000000, 0.8660254037844387076, 1.000000000000000000, 0.8660254037844387076, 1.000000000000000000, 0.8660254037844387076, 1.000000000000000000, 0.8660254037844387076, 1.000000000000000000, 0.8660254037844387076, 1.000000000000000000, 0.8660254037844387076, 1.000000000000000000, 0.8660254037844387076, 1.000000000000000000, 0.8660254037844387076, 1.000000000000000000, 0.8660254037844387076, 1.000000000000000000, 0.8660254037844387076, 1.000000000000000000, 0.8660254037844387076, 1.000000000000000000, 0.8660254037844387076, 1.000000000000000000, 0.8660254037844387076, 1.000000000000000000, 0.8660254037844387076, 1.000000000000000000, 0.8660254037844387076, 1.000000000000000000, 0.8660254037844387076, 1.000000000000000000, 0.8660254037844387076, 1.000000000000000000, 0.8660254037844387076, 1.000000000000000000, 0.8660254037844387076, 1.000000000000000000, 0.8660254037844387076, 1.000000000000000000, 0.8660254037844387076, 1.000000000000000000, 0.8660254037844387076, 1.000000000000000000, 0.8660254037844387076, 1.000000000000000000, 0.8660254037844387076, 1.000000000000000000, 0.8660254037844387076, 1.000000000000000000, 0.8660254037844387076, 1.000000000000000000, 0.8660254037844387076, 1.000000000000000000, 0.8660254037844387076, 1.000000000000000000, 0.8660254037844387076, 1.000000000000000000, 0.8660254037844387076, 1.000000000000000000, 0.8660254037844387076, 1.000000000000000000, 0.8660254037844387076, 1.000000000000000000, 0.8660254037844387076, 1.000000000000000000, 0.8660254037844387076, 1.000000000000000000, 0.8660254037844387076, 1.000000000000000000, 0.8660254037844387076, 1.000000000000000000, 0.8660254037844387076, 1.000000000000000000, 0.8660254037844387076, 1.000000000000000000, 0.8660254037844387076, 1.000000000000000000, 0.8660254037844387076, 1.000000000000000000, 0.8660254037844387076, 1.000000000000000000, 0.8660254037844387076, 1.000000000000000000, 0.8660254037844387076, 1.000000000000000000, 0.8660254037844387076, 1.000000000000000000, 0.8660254037844387076, 1.000000000000000000, 0.8660254037844387076, 1.000000000000000000, 0.8660254037844387076, 1.000000000000000000, 0.8660254037844387076, 1.000000000000000000, 0.8660254037844387076, 1.000000000000000000, 0.8660254037844387076, 1.000000000000000000, 0.8660254037844387076, 1.000000000000000000, 0.8660254037844387076, 1.000000000000000000, 0.8660254037844387076, 1.000000000000000000, 0.8660254037844387076, 1.000000000000000000, 0.8660254037844387076, 1.000000000000000000, 0.8660254037844387076, 1.000000000000000000, 0.8660254037844387076, 1.000000000000000000, 0.8660254037844387076, 1.000000000000000000, 0.8660254037844387076, 1.000000000000000000, 0.8660254037844387076, 1.000000000000000000, 0.8660254037844387076, 1.000000000000000000, 0.8660254037844387076, 1.000000000000000000, 0.8660254037844387076, 1.000000000000000000, 0.8660254037844387076, 1.000000000000000000, 0.8660254037844387076, 1.000000000000000000),
 ( 1.000000000000000000, 0.8660254037844387076, 1.000000000000000000, 0.8660254037844387076, 1.000000000000000000, 0.8660254037844387076, 1.000000000000000000, 0.8660254037844387076, 1.000000000000000000, 0.8660254037844387076, 1.000000000000000000, 0.8660254037844387076, 1.000000000000000000, 0.8660254037844387076, 1.000000000000000000, 0.8660254037844387076, 1.000000000000000000, 0.8660254037844387076, 1.000000000000000000, 0.8660254037844387076, 1.000000000000000000, 0.8660254037844387076, 1.000000000000000000, 0.8660254037844387076, 1.000000000000000000, 0.8660254037844387076, 1.000000000000000000, 0.8660254037844387076, 1.000000000000000000, 0.8660254037844387076, 1.000000000000000000, 0.8660254037844387076, 1.000000000000000000, 0.8660254037844387076, 1.000000000000000000, 0.8660254037844387076, 1.000000000000000000, 0.8660254037844387076, 1.000000000000000000, 0.8660254037844387076, 1.000000000000000000, 0.8660254037844387076, 1.000000000000000000, 0.8660254037844387076, 1.000000000000000000, 0.8660254037844387076, 1.000000000000000000, 0.8660254037844387076, 1.000000000000000000, 0.8660254037844387076, 1.000000000000000000, 0.8660254037844387076, 1.000000000000000000, 0.8660254037844387076, 1.000000000000000000, 0.8660254037844387076, 1.000000000000000000, 0.8660254037844387076, 1.000000000000000000, 0.8660254037844387076, 1.000000000000000000, 0.8660254037844387076, 1.000000000000000000, 0.8660254037844387076, 1.000000000000000000, 0.8660254037844387076, 1.000000000000000000, 0.8660254037844387076, 1.000000000000000000, 0.8660254037844387076, 1.000000000000000000, 0.8660254037844387076, 1.000000000000000000, 0.8660254037844387076, 1.000000000000000000, 0.8660254037844387076, 1.000000000000000000, 0.8660254037844387076, 1.000000000000000000, 0.8660254037844387076, 1.000000000000000000, 0.8660254037844387076, 1.000000000000000000, 0.8660254037844387076, 1.000000000000000000, 0.8660254037844387076, 1.000000000000000000, 0.8660254037844387076, 1.000000000000000000, 0.8660254037844387076, 1.000000000000000000, 0.8660254037844387076, 1.000000000000000000, 0.8660254037844387076, 1.000000000000000000, 0.8660254037844387076, 1.000000000000000000, 0.8660254037844387076, 1.000000000000000000, 0.8660254037844387076, 1.000000000000000000, 0.8660254037844387076, 1.000000000000000000, 0.8660254037844387076, 1.000000000000000000, 0.8660254037844387076, 1.000000000000000000, 0.8660254037844387076, 1.000000000000000000, 0.8660254037844387076, 1.000000000000000000, 0.8660254037844387076, 1.000000000000000000, 0.8660254037844387076, 1.000000000000000000, 0.8660254037844387076, 1.000000000000000000, 0.8660254037844387076, 1.000000000000000000, 0.8660254037844387076, 1.000000000000000000, 0.8660254037844387076, 1.000000000000000000, 0.8660254037844387076, 1.000000000000000000, 0.8660254037844387076, 1.000000000000000000, 0.8660254037844387076, 1.000000000000000000, 0.8660254037844387076, 1.000000000000000000, 0.8660254037844387076, 1.000000000000000000, 0.8660254037844387076, 1.000000000000000000, 0.8660254037844387076, 1.000000000000000000, 0.8660254037844387076, 1.000000000000000000, 0.8660254037844387076, 1.000000000000000000, 0.8660254037844387076, 1.000000000000000000, 0.8660254037844387076, 1.000000000000000000, 0.8660254037844387076, 1.000000000000000000, 0.8660254037844387076, 1.000000000000000000, 0.8660254037844387076, 1.000000000000000000, 0.8660254037844387076, 1.000000000000000000, 0.8660254037844387076, 1.000000000000000000, 0.8660254037844387076, 1.000000000000000000, 0.8660254037844387076, 1.000000000000000000, 0.8660254037844387076, 1.000000000000000000, 0.8660254037844387076, 1.000000000000000000, 0.8660254037844387076, 1.000000000000000000, 0.8660254037844387076, 1.000000000000000000, 0.8660254037844387076, 1.000000000000000000, 0.8660254037844387076, 1.000000000000000000, 0.8660254037844387076, 1.000000000000000000, 0.8660254037844387076, 1.000000000000000000, 0.8660254037844387076, 1.000000000000000000, 0.8660254037844387076, 1.000000000000000000, 0.8660254037844387076, 1.000000000000000000, 0.8660254037844387076, 1.000000000000000000, 0.8660254037844387076, 1.000000000000000000, 0.8660254037844387076, 1.000000000000000000, 0.8660254037844387076, 1.000000000000000000, 0.8660254037844387076, 1.000000000000000000, 0.8660254037844387076, 1.000000000000000000, 0.8660254037844387076, 1.000000000000000000, 0.8660254037844387076, 1.000000000000000000, 0.8660254037844387076, 1.000000000000000000, 0.8660254037844387076, 1.000000000000000000, 0.8660254037844387076, 1.000000000000000000, 0.8660254037844387076, 1.000000000000000000, 0.8660254037844387076, 1.000000000000000000, 0.8660254037844387076, 1.000000000000000000, 0.8660254037844387076, 1.000000000000000000, 0.8660254037844387076, 1.000000000000000000, 0.8660254037844387076, 1.000000000000000000, 0.8660254037844387076, 1.000000000000000000, 0.8660254037844387076, 1.000000000000000000, 0.8660254037844387076, 1.000000000000000000, 0.8660254037844387076, 1.000000000000000000, 0.8660254037844387076, 1.000000000000000000, 0.8660254037844387076, 1.000000000000000000, 0.8660254037844387076, 1.000000000000000000, 0.8660254037844387076, 1.000000000000000000, 0.8660254037844387076, 1.000000000000000000, 0.8660254037844387076, 1.000000000000000000, 0.8660254037844387076, 1.000000000000000000, 0.8660254037844387076, 1.000000000000000000, 0.8660254037844387076, 1.000000000000000000, 0.8660254037844387076, 1.000000000000000000, 0.8660254037844387076, 1.000000000000000000, 0.8660254037844387076, 1.000000000000000000, 0.8660254037844387076, 1.000000000000000000, 0.8660254037844387076, 1.000000000000000000, 0.8660254037844387076, 1.000000000000000000, 0.8660254037844387076, 1.000000000000000000, 0.8660254037844387076, 1.000000000000000000, 0.8660254037844387076, 1.000000000000000000, 0.8660254037844387076, 1.000000000000000000, 0.8660254037844387076, 1.000000000000000000, 0.8660254037844387076, 1.000000000000000000, 0.8660254037844387076, 1.000000000000000000, 0.8660254037844387076, 1.000000000000000000, 0.8660254037844387076, 1.000000000000000000, 0.8660254037844387076, 1.000000000000000000, 0.8660254037844387076, 1.000000000000000000, 0.8660254037844387076, 1.000000000000000000, 0.8660254037844387076, 1.000000000000000000, 0.8660254037844387076, 1.000000000000000000, 0.8660254037844387076, 1.000000000000000000, 0.8660254037844387076, 1.000000000000000000, 0.8660254037844387076, 1.000000000000000000, 0.8660254037844387076, 1.000000000000000000, 0.8660254037844387076, 1.000000000000000000, 0.8660254037844387076, 1.000000000000000000, 0.8660254037844387076, 1.000000000000000000, 0.8660254037844387076, 1.000000000000000000, 0.8660254037844387076, 1.000000000000000000, 0.8660254037844387076, 1.000000000000000000, 0.8660254037844387076, 1.000000000000000000, 0.8660254037844387076, 1.000000000000000000, 0.8660254037844387076, 1.000000000000000000, 0.8660254037844387076, 1.000000000000000000, 0.8660254037844387076, 1.000000000000000000, 0.8660254037844387076, 1.000000000000000000, 0.8660254037844387076, 1.000000000000000000, 0.8660254037844387076, 1.000000000000000000, 0.8660254037844387076, 1.000000000000000000, 0.8660254037844387076, 1.000000000000000000, 0.8660254037844387076, 1.000000000000000000, 0.8660254037844387076, 1.000000000000000000, 0.8660254037844387076, 1.000000000000000000, 0.8660254037844387076, 1.000000000000000000, 0.8660254037844387076, 1.000000000000000000, 0.8660254037844387076, 1.000000000000000000, 0.8660254037844387076, 1.000000000000000000, 0.8660254037844387076, 1.000000000000000000, 0.8660254037844387076, 1.000000000000000000, 0.8660254037844387076, 1.000000000000000000, 0.8660254037844387076, 1.000000000000000000, 0.8660254037844387076, 1.000000000000000000, 0.8660254037844387076, 1.000000000000000000, 0.8660254037844387076, 1.000000000000000000, 0.8660254037844387076, 1.000000000000000000, 0.8660254037844387076, 1.000000000000000000, 0.8660254037844387076, 1.000000000000000000, 0.8660254037844387076, 1.000000000000000000, 0.8660254037844387076, 1.000000000000000000, 0.8660254037844387076, 1.000000000000000000, 0.8660254037844387076, 1.000000000000000000, 0.8660254037844387076, 1.000000000000000000, 0.8660254037844387076, 1.000000000000000000, 0.8660254037844387076, 1.000000000000000000, 0.8660254037844387076, 1.000000000000000000, 0.8660254037844387076, 1.000000000000000000, 0.8660254037844387076, 1.000000000000000000, 0.8660254037844387076, 1.000000000000000000, 0.8660254037844387076, 1.000000000000000000, 0.8660254037844387076, 1.000000000000000000, 0.8660254037844387076, 1.000000000000000000, 0.8660254037844387076, 1.000000000000000000, 0.8660254037844387076, 1.000000000000000000, 0.8660254037844387076, 1.000000000000000000, 0.8660254037844387076, 1.000000000000000000, 0.8660254037844387076, 1.000000000000000000, 0.8660254037844387076, 1.000000000000000000, 0.8660254037844387076, 1.000000000000000000, 0.8660254037844387076, 1.000000000000000000, 0.8660254037844387076, 1.000000000000000000, 0.8660254037844387076, 1.000000000000000000, 0.8660254037844387076, 1.000000000000000000, 0.8660254037844387076, 1.000000000000000000, 0.8660254037844387076, 1.000000000000000000, 0.8660254037844387076, 1.000000000000000000, 0.8660254037844387076, 1.000000000000000000, 0.8660254037844387076, 1.000000000000000000, 0.8660254037844387076, 1.000000000000000000, 0.8660254037844387076, 1.000000000000000000, 0.8660254037844387076, 1.000000000000000000, 0.8660254037844387076, 1.000000000000000000, 0.8660254037844387076, 1.000000000000000000, 0.8660254037844387076, 1.000000000000000000, 0.8660254037844387076, 1.000000000000000000, 0.8660254037844387076, 1.000000000000000000, 0.8660254037844387076, 1.000000000000000000, 0.8660254037844387076, 1.000000000000000000, 0.8660254037844387076, 1.000000000000000000, 0.8660254037844387076, 1.000000000000000000, 0.8660254037844387076, 1.000000000000000000, 0.8660254037844387076, 1.000000000000000000, 0.8660254037844387076, 1.000000000000000000, 0.8660254037844387076, 1.000000000000000000, 0.8660254037844387076, 1.000000000000000000, 0.8660254037844387076, 1.000000000000000000, 0.8660254037844387076, 1.000000000000000000, 0.8660254037844387076, 1.000000000000000000, 0.8660254037844387076, 1.000000000000000000, 0.8660254037844387076, 1.000000000000000000, 0.8660254037844387076, 1.000000000000000000, 0.8660254037844387076, 1.000000000000000000, 0.8660254037844387076, 1.000000000000000000, 0.8660254037844387076, 1.000000000000000000, 0.8660254037844387076, 1.000000000000000000, 0.8660254037844387076, 1.000000000000000000, 0.8660254037844387076, 1.000000000000000000, 0.8660254037844387076, 1.000000000000000000, 0.8660254037844387076, 1.000000000000000000, 0.8660254037844387076, 1.000000000000000000, 0.8660254037844387076, 1.000000000000000000, 0.8660254037844387076, 1.000000000000000000, 0.8660254037844387076, 1.000000000000000000, 0.8660254037844387076, 1.000000000000000000, 0.8660254037844387076, 1.000000000000000000, 0.8660254037844387076, 1.000000000000000000, 0.8660254037844387076, 1.000000000000000000, 0.8660254037844387076, 1.000000000000000000, 0.8660254037844387076, 1.000000000000000000, 0.8660254037844387076, 1.000000000000000000, 0.8660254037844387076, 1.000000000000000000, 0.8660254037844387076, 1.000000000000000000, 0.8660254037844387076, 1.000000000000000000, 0.8660254037844387076, 1.000000000000000000, 0.8660254037844387076, 1.000000000000000000, 0.8660254037844387076, 1.000000000000000000, 0.8660254037844387076, 1.000000000000000000, 0.8660254037844387076, 1.000000000000000000, 0.8660254037844387076, 1.000000000000000000, 0.8660254037844387076, 1.000000000000000000, 0.8660254037844387076, 1.000000000000000000, 0.8660254037844387076, 1.000000000000000000, 0.8660254037844387076, 1.000000000000000000, 0.8660254037844387076, 1.000000000000000000, 0.8660254037844387076, 1.000000000000000000, 0.8660254037844387076, 1.000000000000000000, 0.8660254037844387076, 1.000000000000000000, 0.8660254037844387076, 1.000000000000000000, 0.8660254037844387076, 1.000000000000000000, 0.8660254037844387076, 1.000000000000000000, 0.8660254037844387076, 1.000000000000000000, 0.8660254037844387076, 1.000000000000000000, 0.8660254037844387076, 1.000000000000000000, 0.8660254037844387076, 1.000000000000000000, 0.8660254037844387076, 1.000000000000000000, 0.8660254037844387076, 1.000000000000000000, 0.8660254037844387076, 1.000000000000000000, 0.8660254037844387076, 1.000000000000000000, 0.8660254037844387076, 1.000000000000000000, 0.8660254037844387076, 1.000000000000000000, 0.8660254037844387076, 1.000000000000000000, 0.8660254037844387076, 1.000000000000000000, 0.8660254037844387076, 1.000000000000000000, 0.8660254037844387076, 1.000000000000000000, 0.8660254037844387076, 1.000000000000000000, 0.8660254037844387076, 1.000000000000000000, 0.8660254037844387076, 1.000000000000000000, 0.8660254037844387076, 1.000000000000000000, 0.8660254037844387076, 1.000000000000000000, 0.8660254037844387076, 1.000000000000000000, 0.8660254037844387076, 1.000000000000000000, 0.8660254037844387076, 1.000000000000000000, 0.8660254037844387076, 1.000000000000000000, 0.8660254037844387076, 1.000000000000000000, 0.8660254037844387076, 1.000000000000000000, 0.8660254037844387076, 1.000000000000000000, 0.8660254037844387076, 1.000000000000000000, 0.8660254037844387076, 1.000000000000000000, 0.8660254037844387076, 1.000000000000000000, 0.8660254037844387076, 1.000000000000000000, 0.8660254037844387076, 1.000000000000000000, 0.8660254037844387076, 1.000000000000000000, 0.8660254037844387076, 1.000000000000000000, 0.8660254037844387076, 1.000000000000000000, 0.8660254037844387076, 1.000000000000000000, 0.8660254037844387076, 1.000000000000000000, 0.8660254037844387076, 1.000000000000000000, 0.8660254037844387076, 1.000000000000000000, 0.8660254037844387076, 1.000000000000000000, 0.8660254037844387076, 1.000000000000000000, 0.8660254037844387076, 1.000000000000000000, 0.8660254037844387076, 1.000000000000000000, 0.8660254037844387076, 1.000000000000000000, 0.8660254037844387076, 1.000000000000000000, 0.8660254037844387076, 1.000000000000000000, 0.8660254037844387076, 1.000000000000000000, 0.8660254037844387076, 1.000000000000000000, 0.8660254037844387076, 1.000000000000000000, 0.8660254037844387076, 1.000000000000000000, 0.8660254037844387076, 1.000000000000000000, 0.8660254037844387076, 1.000000000000000000, 0.8660254037844387076, 1.000000000000000000, 0.8660254037844387076, 1.000000000000000000, 0.8660254037844387076, 1.000000000000000000, 0.8660254037844387076, 1.000000000000000000, 0.8660254037844387076, 1.000000000000000000, 0.8660254037844387076, 1.000000000000000000, 0.8660254037844387076, 1.000000000000000000, 0.8660254037844387076, 1.000000000000000000, 0.8660254037844387076, 1.000000000000000000, 0.8660254037844387076, 1.000000000000000000, 0.8660254037844387076, 1.000000000000000000, 0.8660254037844387076, 1.000000000000000000, 0.8660254037844387076, 1.000000000000000000, 0.8660254037844387076, 1.000000000000000000, 0.8660254037844387076, 1.000000000000000000, 0.8660254037844387076, 1.000000000000000000, 0.8660254037844387076, 1.000000000000000000, 0.8660254037844387076, 1.000000000000000000, 0.8660254037844387076, 1.000000000000000000, 0.8660254037844387076, 1.000000000000000000, 0.8660254037844387076, 1.000000000000000000, 0.8660254037844387076, 1.000000000000000000, 0.8660254037844387076, 1.000000000000000000, 0.8660254037844387076, 1.000000000000000000, 0.8660254037844387076, 1.000000000000000000, 0.8660254037844387076, 1.000000000000000000, 0.8660254037844387076, 1.000000000000000000, 0.8660254037844387076, 1.000000000000000000, 0.8660254037844387076, 1.000000000000000000, 0.8660254037844387076, 1.000000000000000000, 0.8660254037844387076, 1.000000000000000000, 0.8660254037844387076, 1.000000000000000000, 0.8660254037844387076, 1.000000000000000000, 0.8660254037844387076, 1.000000000000000000, 0.8660254037844387076, 1.000000000000000000, 0.8660254037844387076, 1.000000000000000000, 0.8660254037844387076, 1.000000000000000000, 0.8660254037844387076, 1.000000000000000000, 0.8660254037844387076, 1.000000000000000000, 0.8660254037844387076, 1.000000000000000000, 0.8660254037844387076, 1.000000000000000000, 0.8660254037844387076, 1.000000000000000000, 0.8660254037844387076, 1.000000000000000000, 0.8660254037844387076, 1.000000000000000000, 0.8660254037844387076, 1.000000000000000000, 0.8660254037844387076, 1.000000000000000000, 0.8660254037844387076, 1.000000000000000000, 0.8660254037844387076, 1.000000000000000000, 0.8660254037844387076, 1.000000000000000000, 0.8660254037844387076, 1.000000000000000000, 0.8660254037844387076, 1.000000000000000000, 0.8660254037844387076, 1.000000000000000000, 0.8660254037844387076, 1.000000000000000000, 0.8660254037844387076, 1.000000000000000000, 0.8660254037844387076, 1.000000000000000000, 0.8660254037844387076, 1.000000000000000000, 0.8660254037844387076, 1.000000000000000000, 0.8660254037844387076, 1.000000000000000000, 0.8660254037844387076, 1.000000000000000000, 0.8660254037844387076, 1.000000000000000000, 0.8660254037844387076, 1.000000000000000000, 0.8660254037844387076, 1.000000000000000000, 0.8660254037844387076, 1.000000000000000000, 0.8660254037844387076, 1.000000000000000000, 0.8660254037844387076, 1.000000000000000000, 0.8660254037844387076, 1.000000000000000000, 0.8660254037844387076, 1.000000000000000000, 0.8660254037844387076, 1.000000000000000000, 0.8660254037844387076, 1.000000000000000000, 0.8660254037844387076, 1.000000000000000000, 0.8660254037844387076, 1.000000000000000000, 0.8660254037844387076, 1.000000000000000000, 0.8660254037844387076, 1.000000000000000000, 0.8660254037844387076, 1.000000000000000000, 0.8660254037844387076, 1.000000000000000000, 0.8660254037844387076, 1.000000000000000000, 0.8660254037844387076, 1.000000000000000000, 0.8660254037844387076, 1.000000000000000000, 0.8660254037844387076, 1.000000000000000000, 0.8660254037844387076, 1.000000000000000000, 0.8660254037844387076, 1.000000000000000000, 0.8660254037844387076, 1.000000000000000000, 0.8660254037844387076, 1.000000000000000000, 0.8660254037844387076, 1.000000000000000000, 0.8660254037844387076, 1.000000000000000000, 0.8660254037844387076, 1.000000000000000000, 0.8660254037844387076, 1.000000000000000000, 0.8660254037844387076, 1.000000000000000000, 0.8660254037844387076, 1.000000000000000000, 0.8660254037844387076, 1.000000000000000000, 0.8660254037844387076, 1.000000000000000000, 0.8660254037844387076, 1.000000000000000000, 0.8660254037844387076, 1.000000000000000000, 0.8660254037844387076, 1.000000000000000000, 0.8660254037844387076, 1.000000000000000000, 0.8660254037844387076, 1.000000000000000000, 0.8660254037844387076, 1.000000000000000000, 0.8660254037844387076, 1.000000000000000000, 0.8660254037844387076, 1.000000000000000000, 0.8660254037844387076, 1.000000000000000000, 0.8660254037844387076, 1.000000000000000000, 0.8660254037844387076, 1.000000000000000000, 0.8660254037844387076, 1.000000000000000000, 0.8660254037844387076, 1.000000000000000000, 0.8660254037844387076, 1.000000000000000000, 0.8660254037844387076, 1.000000000000000000, 0.8660254037844387076, 1.000000000000000000, 0.8660254037844387076, 1.000000000000000000, 0.8660254037844387076, 1.000000000000000000, 0.8660254037844387076, 1.000000000000000000, 0.8660254037844387076, 1.000000000000000000, 0.8660254037844387076, 1.000000000000000000, 0.8660254037844387076, 1.000000000000000000, 0.8660254037844387076, 1.000000000000000000, 0.8660254037844387076, 1.000000000000000000, 0.8660254037844387076, 1.000000000000000000, 0.8660254037844387076, 1.000000000000000000, 0.8660254037844387076, 1.000000000000000000, 0.8660254037844387076, 1.000000000000000000, 0.8660254037844387076, 1.000000000000000000, 0.8660254037844387076, 1.000000000000000000, 0.8660254037844387076, 1.000000000000000000, 0.8660254037844387076, 1.000000000000000000, 0.8660254037844387076, 1.000000000000000000, 0.8660254037844387076, 1.000000000000000000, 0.8660254037844387076, 1.000000000000000000, 0.8660254037844387076, 1.000000000000000000, 0.8660254037844387076, 1.000000000000000000, 0.8660254037844387076, 1.000000000000000000, 0.8660254037844387076, 1.000000000000000000, 0.8660254037844387076, 1.000000000000000000, 0.8660254037844387076, 1.000000000000000000, 0.8660254037844387076, 1.000000000000000000, 0.8660254037844387076, 1.000000000000000000, 0.8660254037844387076, 1.000000000000000000, 0.8660254037844387076, 1.000000000000000000, 0.8660254037844387076, 1.000000000000000000, 0.8660254037844387076, 1.000000000000000000, 0.8660254037844387076, 1.000000000000000000, 0.8660254037844387076, 1.000000000000000000, 0.8660254037844387076, 1.000000000000000000, 0.8660254037844387076, 1.000000000000000000, 0.8660254037844387076, 1.000000000000000000, 0.8660254037844387076, 1.000000000000000000, 0.8660254037844387076, 1.000000000000000000, 0.8660254037844387076, 1.000000000000000000, 0.8660254037844387076, 1.000000000000000000, 0.8660254037844387076, 1.000000000000000000, 0.8660254037844387076, 1.000000000000000000, 0.8660254037844387076, 1.000000000000000000, 0.8660254037844387076, 1.000000000000000000, 0.8660254037844387076, 1.000000000000000000, 0.8660254037844387076, 1.000000000000000000, 0.8660254037844387076, 1.000000000000000000, 0.8660254037844387076, 1.000000000000000000, 0.8660254037844387076, 1.000000000000000000, 0.8660254037844387076, 1.000000000000000000, 0.8660254037844387076, 1.000000000000000000, 0.8660254037844387076, 1.000000000000000000, 0.8660254037844387076, 1.000000000000000000, 0.8660254037844387076, 1.000000000000000000, 0.8660254037844387076, 1.000000000000000000, 0.8660254037844387076, 1.000000000000000000, 0.8660254037844387076, 1.000000000000000000, 0.8660254037844387076, 1.000000000000000000, 0.8660254037844387076, 1.000000000000000000, 0.8660254037844387076, 1.000000000000000000, 0.8660254037844387076, 1.000000000000000000, 0.8660254037844387076, 1.000000000000000000, 0.8660254037844387076, 1.000000000000000000, 0.8660254037844387076, 1.000000000000000000, 0.8660254037844387076, 1.000000000000000000, 0.8660254037844387076, 1.000000000000000000, 0.8660254037844387076, 1.000000000000000000, 0.8660254037844387076, 1.000000000000000000, 0.8660254037844387076, 1.000000000000000000, 0.8660254037844387076, 1.000000000000000000, 0.8660254037844387076, 1.000000000000000000, 0.8660254037844387076, 1.000000000000000000, 0.8660254037844387076, 1.000000000000000000, 0.8660254037844387076, 1.000000000000000000, 0.8660254037844387076, 1.000000000000000000, 0.8660254037844387076, 1.000000000000000000, 0.8660254037844387076, 1.000000000000000000, 0.8660254037844387076, 1.000000000000000000, 0.8660254037844387076, 1.000000000000000000, 0.8660254037844387076, 1.000000000000000000, 0.8660254037844387076, 1.000000000000000000, 0.8660254037844387076, 1.000000000000000000, 0.8660254037844387076, 1.000000000000000000, 0.8660254037844387076, 1.000000000000000000, 0.8660254037844387076, 1.000000000000000000, 0.8660254037844387076, 1.000000000000000000, 0.8660254037844387076, 1.000000000000000000, 0.8660254037844387076, 1.000000000000000000, 0.8660254037844387076, 1.000000000000000000, 0.8660254037844387076, 1.000000000000000000, 0.8660254037844387076, 1.000000000000000000, 0.8660254037844387076, 1.000000000000000000, 0.8660254037844387076, 1.000000000000000000, 0.8660254037844387076, 1.000000000000000000, 0.8660254037844387076, 1.000000000000000000, 0.8660254037844387076, 1.000000000000000000, 0.8660254037844387076, 1.000000000000000000, 0.8660254037844387076, 1.000000000000000000, 0.8660254037844387076, 1.000000000000000000, 0.8660254037844387076, 1.000000000000000000, 0.8660254037844387076, 1.000000000000000000, 0.8660254037844387076, 1.000000000000000000, 0.8660254037844387076, 1.000000000000000000, 0.8660254037844387076, 1.000000000000000000, 0.8660254037844387076, 1.000000000000000000, 0.8660254037844387076, 1.000000000000000000, 0.8660254037844387076, 1.000000000000000000, 0.8660254037844387076, 1.000000000000000000, 0.8660254037844387076, 1.000000000000000000, 0.8660254037844387076, 1.000000000000000000, 0.8660254037844387076, 1.000000000000000000, 0.8660254037844387076, 1.000000000000000000, 0.8660254037844387076, 1.000000000000000000, 0.8660254037844387076, 1.000000000000000000, 0.8660254037844387076, 1.000000000000000000, 0.8660254037844387076, 1.000000000000000000, 0.8660254037844387076, 1.000000000000000000, 0.8660254037844387076, 1.000000000000000000, 0.8660254037844387076, 1.000000000000000000, 0.8660254037844387076, 1.000000000000000000, 0.8660254037844387076, 1.000000000000000000, 0.8660254037844387076, 1.000000000000000000, 0.8660254037844387076, 1.000000000000000000, 0.8660254037844387076, 1.000000000000000000, 0.8660254037844387076, 1.000000000000000000, 0.8660254037844387076, 1.000000000000000000, 0.8660254037844387076, 1.000000000000000000, 0.8660254037844387076, 1.000000000000000000, 0.8660254037844387076, 1.000000000000000000, 0.8660254037844387076, 1.000000000000000000, 0.8660254037844387076, 1.000000000000000000, 0.8660254037844387076, 1.000000000000000000, 0.8660254037844387076, 1.000000000000000000, 0.8660254037844387076, 1.000000000000000000, 0.8660254037844387076, 1.000000000000000000, 0.8660254037844387076, 1.000000000000000000, 0.8660254037844387076, 1.000000000000000000, 0.8660254037844387076, 1.000000000000000000, 0.8660254037844387076, 1.000000000000000000, 0.8660254037844387076, 1.000000000000000000, 0.8660254037844387076, 1.000000000000000000, 0.8660254037844387076, 1.000000000000000000, 0.8660254037844387076, 1.000000000000000000, 0.8660254037844387076, 1.000000000000000000, 0.8660254037844387076, 1.000000000000000000, 0.8660254037844387076, 1.000000000000000000, 0.8660254037844387076, 1.000000000000000000, 0.8660254037844387076, 1.000000000000000000, 0.8660254037844387076, 1.000000000000000000, 0.8660254037844387076, 1.000000000000000000, 0.8660254037844387076, 1.000000000000000000, 0.8660254037844387076, 1.000000000000000000, 0.8660254037844387076, 1.000000000000000000, 0.8660254037844387076, 1.000000000000000000, 0.8660254037844387076, 1.000000000000000000, 0.8660254037844387076, 1.000000000000000000, 0.8660254037844387076, 1.000000000000000000, 0.8660254037844387076, 1.000000000000000000, 0.8660254037844387076, 1.000000000000000000, 0.8660254037844387076, 1.000000000000000000, 0.8660254037844387076, 1.000000000000000000, 0.8660254037844387076, 1.000000000000000000, 0.8660254037844387076, 1.000000000000000000, 0.8660254037844387076, 1.000000000000000000, 0.8660254037844387076, 1.000000000000000000, 0.8660254037844387076, 1.000000000000000000, 0.8660254037844387076, 1.000000000000000000, 0.8660254037844387076, 1.000000000000000000, 0.8660254037844387076, 1.000000000000000000, 0.8660254037844387076, 1.000000000000000000, 0.8660254037844387076, 1.000000000000000000, 0.8660254037844387076, 1.000000000000000000, 0.8660254037844387076, 1.000000000000000000, 0.8660254037844387076, 1.000000000000000000, 0.8660254037844387076, 1.000000000000000000, 0.8660254037844387076, 1.000000000000000000, 0.8660254037844387076, 1.000000000000000000, 0.8660254037844387076, 1.000000000000000000, 0.8660254037844387076, 1.000000000000000000, 0.8660254037844387076, 1.000000000000000000, 0.8660254037844387076, 1.000000000000000000, 0.8660254037844387076, 1.000000000000000000, 0.8660254037844387076, 1.000000000000000000, 0.8660254037844387076, 1.000000000000000000, 0.8660254037844387076, 1.000000000000000000, 0.8660254037844387076, 1.000000000000000000, 0.8660254037844387076, 1.000000000000000000, 0.8660254037844387076, 1.000000000000000000, 0.8660254037844387076, 1.000000000000000000, 0.8660254037844387076, 1.000000000000000000, 0.8660254037844387076, 1.000000000000000000, 0.8660254037844387076, 1.000000000000000000, 0.8660254037844387076, 1.000000000000000000, 0.8660254037844387076, 1.000000000000000000, 0.8660254037844387076, 1.000000000000000000, 0.8660254037844387076, 1.000000000000000000, 0.8660254037844387076, 1.000000000000000000, 0.8660254037844387076, 1.000000000000000000, 0.8660254037844387076, 1.000000000000000000, 0.8660254037844387076, 1.000000000000000000, 0.8660254037844387076, 1.000000000000000000, 0.8660254037844387076, 1.000000000000000000, 0.8660254037844387076, 1.000000000000000000, 0.8660254037844387076, 1.000000000000000000, 0.8660254037844387076, 1.000000000000000000, 0.8660254037844387076, 1.000000000000000000, 0.8660254037844387076, 1.000000000000000000, 0.8660254037844387076, 1.000000000000000000, 0.8660254037844387076, 1.000000000000000000, 0.8660254037844387076, 1.000000000000000000, 0.8660254037844387076, 1.000000000000000000, 0.8660254037844387076, 1.000000000000000000, 0.8660254037844387076, 1.000000000000000000, 0.8660254037844387076, 1.000000000000000000, 0.8660254037844387076, 1.000000000000000000, 0.8660254037844387076, 1.000000000000000000, 0.8660254037844387076, 1.000000000000000000, 0.8660254037844387076, 1.000000000000000000, 0.8660254037844387076, 1.000000000000000000, 0.8660254037844387076, 1.000000000000000000, 0.8660254037844387076, 1.000000000000000000, 0.8660254037844387076, 1.000000000000000000, 0.8660254037844387076, 1.000000000000000000, 0.8660254037844387076, 1.000000000000000000, 0.8660254037844387076, 1.000000000000000000, 0.8660254037844387076, 1.000000000000000000, 0.8660254037844387076, 1.000000000000000000, 0.8660254037844387076, 1.000000000000000000, 0.8660254037844387076, 1.000000000000000000, 0.8660254037844387076, 1.000000000000000000, 0.8660254037844387076, 1.000000000000000000, 0.8660254037844387076, 1.000000000000000000, 0.8660254037844387076, 1.000000000000000000, 0.8660254037844387076, 1.000000000000000000, 0.8660254037844387076, 1.000000000000000000, 0.8660254037844387076, 1.000000000000000000, 0.8660254037844387076, 1.000000000000000000, 0.8660254037844387076, 1.000000000000000000, 0.8660254037844387076, 1.000000000000000000, 0.8660254037844387076, 1.000000000000000000, 0.8660254037844387076, 1.000000000000000000, 0.8660254037844387076, 1.000000000000000000, 0.8660254037844387076, 1.000000000000000000, 0.8660254037844387076, 1.000000000000000000, 0.8660254037844387076, 1.000000000000000000, 0.8660254037844387076, 1.000000000000000000, 0.8660254037844387076, 1.000000000000000000, 0.8660254037844387076, 1.000000000000000000, 0.8660254037844387076, 1.000000000000000000, 0.8660254037844387076, 1.000000000000000000, 0.8660254037844387076, 1.000000000000000000, 0.8660254037844387076, 1.000000000000000000, 0.8660254037844387076, 1.000000000000000000, 0.8660254037844387076, 1.000000000000000000, 0.8660254037844387076, 1.000000000000000000, 0.8660254037844387076, 1.000000000000000000, 0.8660254037844387076, 1.000000000000000000, 0.8660254037844387076, 1.000000000000000000, 0.8660254037844387076, 1.000000000000000000, 0.8660254037844387076, 1.000000000000000000, 0.8660254037844387076, 1.000000000000000000, 0.8660254037844387076, 1.000000000000000000, 0.8660254037844387076, 1.000000000000000000, 0.8660254037844387076, 1.000000000000000000, 0.8660254037844387076, 1.000000000000000000, 0.8660254037844387076, 1.000000000000000000, 0.8660254037844387076, 1.000000000000000000, 0.8660254037844387076, 1.000000000000000000, 0.8660254037844387076, 1.000000000000000000, 0.8660254037844387076, 1.000000000000000000, 0.8660254037844387076, 1.000000000000000000, 0.8660254037844387076, 1.000000000000000000, 0.8660254037844387076, 1.000000000000000000, 0.8660254037844387076, 1.000000000000000000, 0.8660254037844387076, 1.000000000000000000, 0.8660254037844387076, 1.000000000000000000, 0.8660254037844387076, 1.000000000000000000, 0.8660254037844387076, 1.000000000000000000, 0.8660254037844387076, 1.000000000000000000, 0.8660254037844387076, 1.000000000000000000, 0.8660254037844387076, 1.000000000000000000, 0.8660254037844387076, 1.000000000000000000, 0.8660254037844387076, 1.000000000000000000, 0.8660254037844387076, 1.000000000000000000, 0.8660254037844387076, 1.000000000000000000, 0.8660254037844387076, 1.000000000000000000, 0.8660254037844387076, 1.000000000000000000, 0.8660254037844387076, 1.000000000000000000, 0.8660254037844387076, 1.000000000000000000, 0.8660254037844387076, 1.000000000000000000, 0.8660254037844387076, 1.000000000000000000, 0.8660254037844387076, 1.000000000000000000, 0.8660254037844387076, 1.000000000000000000) ) ) 
 REPRESENTATION_ITEM ( '' )  SURFACE ( )  );
#33699=CARTESIAN_POINT ( 'NONE',  ( -1.655278471875002211, 14.63297358603754361, -62.68493913623279923 ) ) ;
#33700=ORIENTED_EDGE ( 'NONE', *, *, #16228, .T. ) ;
#33701=CARTESIAN_POINT ( 'NONE',  ( 3.310556943750001313, 17.50000000000001776, -81.35160580289945642 ) ) ;
#33702=CARTESIAN_POINT ( 'NONE',  ( 3.500000000000001332, 19.52072594216371115, -77.07139747004410424 ) ) ;
#33703=CARTESIAN_POINT ( 'NONE',  ( 1.749999999999998224, 14.46891108675447590, -44.62764746908817415 ) ) ;
#33704=DIRECTION ( 'NONE',  ( -0.000000000000000000, 1.259100132267607459E-16, -1.000000000000000000 ) ) ;
#33705=LINE ( 'NONE', #13705, #30629 ) ;
#33707=CARTESIAN_POINT ( 'NONE',  ( 3.310556943749999981, 15.58864905735836182, -40.34743913623281486 ) ) ;
#33708=CARTESIAN_POINT ( 'NONE',  ( 1.655278471874998436, 14.63297358603754716, -100.4307724695661364 ) ) ;
#33709=CARTESIAN_POINT ( 'NONE',  ( -1.749999999999999778, 20.53108891324555429, -93.82139747004409003 ) ) ;
#33714=CARTESIAN_POINT ( 'NONE',  ( 3.310556943750001313, 19.41135094264166128, -52.18077246956612925 ) ) ;
#33716=ORIENTED_EDGE ( 'NONE', *, *, #38909, .T. ) ;
#33720=CARTESIAN_POINT ( 'NONE',  ( 0.000000000000000000, 17.50000000000002487, -149.5231586289125687 ) ) ;
#33722=EDGE_LOOP ( 'NONE', ( #35271, #10795, #37816, #30033 ) ) ;
#33723=CARTESIAN_POINT ( 'NONE',  ( -1.750000000000002220, 14.46891108675447768, -43.79431413575483845 ) ) ;
#33724=CARTESIAN_POINT ( 'NONE',  ( 3.500000000000000000, 15.47927405783632970, -97.23806413671074722 ) ) ;
#33727=CARTESIAN_POINT ( 'NONE',  ( -3.310556943750000425, 19.41135094264165772, -31.93493913623279568 ) ) ;
#33728=CARTESIAN_POINT ( 'NONE',  ( -1.394453263437886604E-15, 14.00000000000001776, -106.4047308033774328 ) ) ;
#33729=CARTESIAN_POINT ( 'NONE',  ( 1.655278471874998436, 14.63297358603754361, -80.51827246956614204 ) ) ;
#33730=CARTESIAN_POINT ( 'NONE',  ( 3.310556943750001313, 17.50000000000002487, -134.2641058028994507 ) ) ;
#33734=CARTESIAN_POINT ( 'NONE',  ( 3.500000000000000000, 15.47927405783631727, -24.23806413671077209 ) ) ;
#33736=CARTESIAN_POINT ( 'NONE',  ( -3.310556943750000425, 19.41135094264166838, -122.9349391362327992 ) ) ;
#33738=CARTESIAN_POINT ( 'NONE',  ( -1.655278471875002211, 14.63297358603754716, -84.59743913623279354 ) ) ;
#33739=CARTESIAN_POINT ( 'NONE',  ( 0.9378221735089300459, 21.00000000000001066, -24.25563900116003779 ) ) ;
#33740=CARTESIAN_POINT ( 'NONE',  ( 3.500000000000001332, 17.50000000000001421, -71.15473080337743284 ) ) ;
#33741=CARTESIAN_POINT ( 'NONE',  ( 3.310556943750001313, 17.50000000000001421, -53.35160580289946353 ) ) ;
#33743=CARTESIAN_POINT ( 'NONE',  ( 0.000000000000000000, 17.50000000000002487, -149.5231586289125687 ) ) ;
#33744=CARTESIAN_POINT ( 'NONE',  ( -0.9378221735089291577, 21.00000000000001776, -99.16632260368299967 ) ) ;
#33745=CARTESIAN_POINT ( 'NONE',  ( -1.655278471874999990, 20.36702641396249192, -80.01827246956614204 ) ) ;
#33746=CARTESIAN_POINT ( 'NONE',  ( 3.310556943750001313, 17.50000000000002487, -140.3516058028994564 ) ) ;
#33748=CARTESIAN_POINT ( 'NONE',  ( -7.022189441860112050E-16, 13.67729811471672541, -103.5141058028994649 ) ) ;
#33749=CARTESIAN_POINT ( 'NONE',  ( 2.340729813953370519E-16, 21.32270188528331190, -77.01410580289946495 ) ) ;
#33750=ORIENTED_EDGE ( 'NONE', *, *, #11380, .F. ) ;
#33752=( BOUNDED_CURVE ( )  B_SPLINE_CURVE ( 2, ( #40733, #11589, #27354, #1818, #17366, #23745, #992, #30750, #20549 ),
 .UNSPECIFIED., .F., .T. ) 
 B_SPLINE_CURVE_WITH_KNOTS ( ( 3, 2, 2, 2, 3 ),
 ( 0.4479166666666666852, 0.4486111111111111271, 0.4500000000000000111, 0.4513888888888888951, 0.4520833333333333370 ),
 .UNSPECIFIED. ) 
 CURVE ( )  GEOMETRIC_REPRESENTATION_ITEM ( )  RATIONAL_B_SPLINE_CURVE ( ( 0.9330127018922194093, 0.9330127018922194093, 1.000000000000000000, 0.8660254037844387076, 1.000000000000000000, 0.8660254037844387076, 1.000000000000000000, 0.9330127018922194093, 0.9330127018922194093 ) ) 
 REPRESENTATION_ITEM ( '' )  );
#33753=CARTESIAN_POINT ( 'NONE',  ( -1.655278471874999990, 20.36702641396249192, -99.01827246956612782 ) ) ;
#33755=CARTESIAN_POINT ( 'NONE',  ( -7.460324959392693302E-14, 21.00000000000001776, -85.90473080337741862 ) ) ;
#33756=CARTESIAN_POINT ( 'NONE',  ( 1.750000000000001110, 20.53108891324555074, -50.98806413671076854 ) ) ;
#33758=CARTESIAN_POINT ( 'NONE',  ( 1.655278471875001101, 20.36702641396248836, -61.09743913623280775 ) ) ;
#33760=CARTESIAN_POINT ( 'NONE',  ( -3.310556943750001313, 17.50000000000002132, -117.7641058028994792 ) ) ;
#33763=ORIENTED_EDGE ( 'NONE', *, *, #26126, .F. ) ;
#33764=ORIENTED_EDGE ( 'NONE', *, *, #13497, .F. ) ;
#33766=ORIENTED_EDGE ( 'NONE', *, *, #41296, .T. ) ;
#33768=CARTESIAN_POINT ( 'NONE',  ( 2.340729813953370519E-16, 21.32270188528330834, -68.01410580289947916 ) ) ;
#33769=VERTEX_POINT ( 'NONE', #15852 ) ;
#33770=VERTEX_POINT ( 'NONE', #19647 ) ;
#33771=CARTESIAN_POINT ( 'NONE',  ( -1.750000000000002220, 14.46891108675448834, -130.7943141357548598 ) ) ;
#33772=EDGE_CURVE ( 'NONE', #33859, #34171, #41796, .T. ) ;
#33775=ADVANCED_FACE ( 'NONE', ( #13062 ), #6675, .T. ) ;
#33776=ORIENTED_EDGE ( 'NONE', *, *, #9722, .T. ) ;
#33778=CARTESIAN_POINT ( 'NONE',  ( 3.310556943749999981, 15.58864905735837780, -138.3474391362328220 ) ) ;
#33780=CARTESIAN_POINT ( 'NONE',  ( -3.310556943750001313, 17.50000000000001066, -45.85160580289945642 ) ) ;
#33781=CARTESIAN_POINT ( 'NONE',  ( 0.9378221735089281585, 14.00000000000002132, -96.66632260368298546 ) ) ;
#33782=CARTESIAN_POINT ( 'NONE',  ( 3.310556943750001313, 17.50000000000001066, -33.35160580289946353 ) ) ;
#33783=EDGE_CURVE ( 'NONE', #17606, #37828, #32243, .T. ) ;
#33784=CARTESIAN_POINT ( 'NONE',  ( -3.310556943750002645, 15.58864905735837425, -96.76827246956612782 ) ) ;
#33786=CARTESIAN_POINT ( 'NONE',  ( 1.655278471874998436, 14.63297358603753651, -23.43077246956613990 ) ) ;
#33788=CARTESIAN_POINT ( 'NONE',  ( 2.474675557024783212E-16, 21.54145188432739744, -96.21098080242150274 ) ) ;
#33789=CARTESIAN_POINT ( 'NONE',  ( 3.500000000000000000, 15.47927405783632970, -100.2380641367107756 ) ) ;
#33790=CARTESIAN_POINT ( 'NONE',  ( -1.749999999999999778, 20.53108891324555074, -61.82139747004410424 ) ) ;
#33791=CARTESIAN_POINT ( 'NONE',  ( -1.750000000000002220, 14.46891108675448301, -83.48806413671076143 ) ) ;
#33792=CARTESIAN_POINT ( 'NONE',  ( -1.655278471875002211, 14.63297358603754539, -70.68493913623278502 ) ) ;
#33794=CARTESIAN_POINT ( 'NONE',  ( -3.500000000000001332, 17.50000000000002132, -111.6547308033774328 ) ) ;
#33797=CARTESIAN_POINT ( 'NONE',  ( 3.500000000000001776, 19.52072594216370760, -48.37764746908817415 ) ) ;
#33799=LINE ( 'NONE', #36995, #40754 ) ;
#33800=CARTESIAN_POINT ( 'NONE',  ( -0.9378221735089291577, 21.00000000000001066, -35.16632260368299256 ) ) ;
#33801=ORIENTED_EDGE ( 'NONE', *, *, #13613, .F. ) ;
#33802=CARTESIAN_POINT ( 'NONE',  ( -7.424026671074350129E-16, 13.45854811567263987, -115.4047308033774328 ) ) ;
#33804=DIRECTION ( 'NONE',  ( 0.000000000000000000, 1.000000000000000000, 0.000000000000000000 ) ) ;
#33808=CARTESIAN_POINT ( 'NONE',  ( -1.655278471874999990, 20.36702641396249192, -74.93077246956613635 ) ) ;
#33809=CARTESIAN_POINT ( 'NONE',  ( -0.9378221735089291577, 21.00000000000001776, -97.16632260368297125 ) ) ;
#33810=DIRECTION ( 'NONE',  ( -0.000000000000000000, 1.259100132267607459E-16, -1.000000000000000000 ) ) ;
#33814=CARTESIAN_POINT ( 'NONE',  ( 4.648177544792955347E-16, 21.00000000000002132, -120.9047308033774328 ) ) ;
#33815=CARTESIAN_POINT ( 'NONE',  ( 1.655278471874998436, 14.63297358603754539, -86.43077246956613635 ) ) ;
#33816=VERTEX_POINT ( 'NONE', #10289 ) ;
#33820=DIRECTION ( 'NONE',  ( 0.000000000000000000, 1.000000000000000000, 0.000000000000000000 ) ) ;
#33821=CYLINDRICAL_SURFACE ( 'NONE', #15984, 3.499999999999999556 ) ;
#33822=CARTESIAN_POINT ( 'NONE',  ( 1.655278471875001101, 20.36702641396248836, -56.18493913623279212 ) ) ;
#33823=EDGE_CURVE ( 'NONE', #35046, #7402, #15985, .T. ) ;
#33824=CARTESIAN_POINT ( 'NONE',  ( 3.310556943750001313, 19.41135094264166838, -114.2682724695661136 ) ) ;
#33825=ORIENTED_EDGE ( 'NONE', *, *, #7989, .T. ) ;
#33826=CARTESIAN_POINT ( 'NONE',  ( 1.750000000000001110, 20.53108891324555785, -122.9880641367107614 ) ) ;
#33827=CARTESIAN_POINT ( 'NONE',  ( -1.655278471874999990, 20.36702641396248481, -39.93077246956613635 ) ) ;
#33828=CARTESIAN_POINT ( 'NONE',  ( -3.310556943750002645, 15.58864905735836892, -64.76827246956614204 ) ) ;
#33829=CARTESIAN_POINT ( 'NONE',  ( 1.749999999999998224, 14.46891108675448478, -110.6276474690881741 ) ) ;
#33831=CARTESIAN_POINT ( 'NONE',  ( -7.022189441860112050E-16, 13.67729811471672363, -94.51410580289946495 ) ) ;
#33832=CARTESIAN_POINT ( 'NONE',  ( 3.500000000000000000, 15.47927405783632970, -98.23806413671076143 ) ) ;
#33834=CARTESIAN_POINT ( 'NONE',  ( -3.500000000000001332, 17.50000000000001421, -70.65473080337743284 ) ) ;
#33836=CARTESIAN_POINT ( 'NONE',  ( -1.750000000000002220, 14.46891108675447946, -65.79431413575484555 ) ) ;
#33837=CARTESIAN_POINT ( 'NONE',  ( 3.310556943750001313, 17.50000000000001066, -32.26410580289947205 ) ) ;
#33838=CARTESIAN_POINT ( 'NONE',  ( -7.022189441860112050E-16, 13.67729811471672363, -92.60160580289947063 ) ) ;
#33839=CARTESIAN_POINT ( 'NONE',  ( -3.500000000000001332, 17.50000000000001421, -53.65473080337743284 ) ) ;
#33840=CARTESIAN_POINT ( 'NONE',  ( 2.340729813953370519E-16, 21.32270188528331900, -110.1016058028994706 ) ) ;
#33841=CARTESIAN_POINT ( 'NONE',  ( -3.310556943750002201, 15.58864905735836537, -35.76827246956612782 ) ) ;
#33843=DIRECTION ( 'NONE',  ( -0.000000000000000000, 1.259100132267607459E-16, -1.000000000000000000 ) ) ;
#33848=CARTESIAN_POINT ( 'NONE',  ( -3.310556943750000425, 19.41135094264166838, -94.84743913623280775 ) ) ;
#33859=VERTEX_POINT ( 'NONE', #20498 ) ;
#33862=( BOUNDED_CURVE ( )  B_SPLINE_CURVE ( 2, ( #18321, #31504, #5346, #27688, #25135, #37888, #2152, #15139, #28103 ),
 .UNSPECIFIED., .F., .F. ) 
 B_SPLINE_CURVE_WITH_KNOTS ( ( 3, 2, 2, 2, 3 ),
 ( 0.4312500000000000222, 0.4319444444444444642, 0.4333333333333333481, 0.4347222222222222321, 0.4354166666666666741 ),
 .UNSPECIFIED. ) 
 CURVE ( )  GEOMETRIC_REPRESENTATION_ITEM ( )  RATIONAL_B_SPLINE_CURVE ( ( 0.9330127018922194093, 0.9330127018922194093, 1.000000000000000000, 0.8660254037844387076, 1.000000000000000000, 0.8660254037844387076, 1.000000000000000000, 0.9330127018922194093, 0.9330127018922194093 ) ) 
 REPRESENTATION_ITEM ( '' )  );
#33866=EDGE_LOOP ( 'NONE', ( #14200, #18171, #29930, #22984 ) ) ;
#33867=CARTESIAN_POINT ( 'NONE',  ( -0.9378221735089291577, 21.00000000000001421, -54.16632260368298546 ) ) ;
#33869=CARTESIAN_POINT ( 'NONE',  ( 1.749999999999998224, 14.46891108675448834, -137.3213974700441042 ) ) ;
#33870=DIRECTION ( 'NONE',  ( -0.000000000000000000, 1.259100132267607459E-16, -1.000000000000000000 ) ) ;
#33871=CARTESIAN_POINT ( 'NONE',  ( 0.9378221735089281585, 14.00000000000002132, -101.6663226036829855 ) ) ;
#33872=CARTESIAN_POINT ( 'NONE',  ( -3.310556943750000425, 19.41135094264167549, -130.9349391362327992 ) ) ;
#33873=CARTESIAN_POINT ( 'NONE',  ( -7.022189441860112050E-16, 13.67729811471671830, -57.60160580289946353 ) ) ;
#33876=CARTESIAN_POINT ( 'NONE',  ( -3.500000000000001332, 17.50000000000001066, -44.65473080337743994 ) ) ;
#33877=CARTESIAN_POINT ( 'NONE',  ( 0.9378221735089300459, 21.00000000000002132, -123.2556390011600342 ) ) ;
#33879=CARTESIAN_POINT ( 'NONE',  ( -1.750000000000002220, 14.46891108675448834, -129.7943141357548598 ) ) ;
#33880=CARTESIAN_POINT ( 'NONE',  ( 2.340729813953370519E-16, 21.32270188528331900, -114.0141058028994792 ) ) ;
#33883=CARTESIAN_POINT ( 'NONE',  ( -3.500000000000001332, 17.50000000000001776, -86.96098080242151696 ) ) ;
#33884=VECTOR ( 'NONE', #18163, 1000.000000000000000 ) ;
#33886=CARTESIAN_POINT ( 'NONE',  ( -3.310556943750001313, 17.50000000000001421, -50.76410580289947205 ) ) ;
#33887=CARTESIAN_POINT ( 'NONE',  ( 3.310556943750001313, 19.41135094264166838, -107.2682724695661420 ) ) ;
#33888=EDGE_CURVE ( 'NONE', #466, #36084, #13472, .T. ) ;
#33889=CARTESIAN_POINT ( 'NONE',  ( 0.9378221735089300459, 21.00000000000002132, -110.9493890021159359 ) ) ;
#33890=DIRECTION ( 'NONE',  ( 0.000000000000000000, 1.000000000000000000, 0.000000000000000000 ) ) ;
#33892=CARTESIAN_POINT ( 'NONE',  ( -3.500000000000000000, 19.52072594216370760, -72.73806413671076143 ) ) ;
#33893=CARTESIAN_POINT ( 'NONE',  ( -3.310556943750000425, 19.41135094264167549, -129.9349391362327992 ) ) ;
#33896=CYLINDRICAL_SURFACE ( 'NONE', #9922, 3.499999999999999556 ) ;
#33897=CARTESIAN_POINT ( 'NONE',  ( 4.648177544792955347E-16, 21.00000000000001421, -58.21098080242150985 ) ) ;
#33898=CARTESIAN_POINT ( 'NONE',  ( 3.310556943750001313, 19.41135094264166128, -59.26827246956613493 ) ) ;
#33900=CARTESIAN_POINT ( 'NONE',  ( 1.655278471875001101, 20.36702641396249192, -79.18493913623279923 ) ) ;
#33905=CARTESIAN_POINT ( 'NONE',  ( 3.310556943749999981, 15.58864905735836182, -39.34743913623281486 ) ) ;
#33906=CARTESIAN_POINT ( 'NONE',  ( -1.655278471874999990, 20.36702641396249192, -95.93077246956613635 ) ) ;
#33907=CARTESIAN_POINT ( 'NONE',  ( 4.286263797015737581E-16, 14.00000000000002487, -149.5231586289125687 ) ) ;
#33911=CARTESIAN_POINT ( 'NONE',  ( -3.310556943750002645, 15.58864905735836714, -50.68077246956613635 ) ) ;
#33913=ORIENTED_EDGE ( 'NONE', *, *, #3278, .F. ) ;
#33917=CARTESIAN_POINT ( 'NONE',  ( 0.9378221735089128375, 21.00000000000003553, -124.9493890021159359 ) ) ;
#33918=EDGE_CURVE ( 'NONE', #15353, #32548, #2931, .T. ) ;
#33920=CYLINDRICAL_SURFACE ( 'NONE', #2771, 3.499999999999999556 ) ;
#33923=CARTESIAN_POINT ( 'NONE',  ( -3.500000000000001332, 17.50000000000001066, -40.96098080242150985 ) ) ;
#33925=CARTESIAN_POINT ( 'NONE',  ( 0.000000000000000000, 17.50000000000002487, -149.5231586289125687 ) ) ;
#33928=CARTESIAN_POINT ( 'NONE',  ( -1.655278471875002211, 14.63297358603754006, -31.68493913623279923 ) ) ;
#33929=LINE ( 'NONE', #30951, #5469 ) ;
#33930=CARTESIAN_POINT ( 'NONE',  ( 3.310556943750001313, 17.50000000000002132, -126.2641058028994792 ) ) ;
#33933=( BOUNDED_CURVE ( )  B_SPLINE_CURVE ( 2, ( #29692, #12488, #25888, #9510, #32467, #22471, #38852, #9730, #25473 ),
 .UNSPECIFIED., .F., .T. ) 
 B_SPLINE_CURVE_WITH_KNOTS ( ( 3, 2, 2, 2, 3 ),
 ( 0.5604166666666666741, 0.5611111111111111160, 0.5625000000000000000, 0.5638888888888888840, 0.5645833333333333259 ),
 .UNSPECIFIED. ) 
 CURVE ( )  GEOMETRIC_REPRESENTATION_ITEM ( )  RATIONAL_B_SPLINE_CURVE ( ( 0.9330127018922194093, 0.9330127018922194093, 1.000000000000000000, 0.8660254037844387076, 1.000000000000000000, 0.8660254037844387076, 1.000000000000000000, 0.9330127018922194093, 0.9330127018922194093 ) ) 
 REPRESENTATION_ITEM ( '' )  );
#33934=EDGE_CURVE ( 'NONE', #7402, #15133, #37294, .T. ) ;
#33936=CARTESIAN_POINT ( 'NONE',  ( -1.655278471875002211, 14.63297358603755249, -124.6849391362327992 ) ) ;
#33938=CARTESIAN_POINT ( 'NONE',  ( 3.310556943750001313, 19.41135094264166483, -84.18077246956615056 ) ) ;
#33939=CARTESIAN_POINT ( 'NONE',  ( 3.500000000000000000, 15.47927405783633326, -115.2380641367107472 ) ) ;
#33941=DIRECTION ( 'NONE',  ( -0.000000000000000000, 1.259100132267607459E-16, -1.000000000000000000 ) ) ;
#33942=CARTESIAN_POINT ( 'NONE',  ( -1.749999999999999778, 20.53108891324555074, -68.82139747004409003 ) ) ;
#33943=CARTESIAN_POINT ( 'NONE',  ( 3.310556943750001313, 17.50000000000001421, -56.35160580289947063 ) ) ;
#33945=DIRECTION ( 'NONE',  ( -0.000000000000000000, 1.259100132267607459E-16, -1.000000000000000000 ) ) ;
#33946=CARTESIAN_POINT ( 'NONE',  ( -3.310556943750000425, 19.41135094264166483, -74.93493913623279923 ) ) ;
#33947=CARTESIAN_POINT ( 'NONE',  ( 3.310556943750001313, 17.50000000000002487, -139.3516058028994564 ) ) ;
#33948=VECTOR ( 'NONE', #27933, 1000.000000000000000 ) ;
#33950=CARTESIAN_POINT ( 'NONE',  ( 3.310556943750001313, 17.50000000000002132, -103.2641058028994649 ) ) ;
#33951=CARTESIAN_POINT ( 'NONE',  ( 3.310556943750001313, 19.41135094264166483, -78.18077246956613635 ) ) ;
#33952=VERTEX_POINT ( 'NONE', #27709 ) ;
#33953=CARTESIAN_POINT ( 'NONE',  ( 3.310556943750001313, 17.50000000000001776, -97.35160580289945642 ) ) ;
#33956=CARTESIAN_POINT ( 'NONE',  ( -0.9378221735089310451, 14.00000000000002132, -85.44938900211596433 ) ) ;
#33957=DIRECTION ( 'NONE',  ( 0.000000000000000000, 1.000000000000000000, 0.000000000000000000 ) ) ;
#33958=DIRECTION ( 'NONE',  ( 0.000000000000000000, 1.000000000000000000, 0.000000000000000000 ) ) ;
#33959=CARTESIAN_POINT ( 'NONE',  ( 3.310556943750001313, 19.41135094264166483, -53.18077246956613635 ) ) ;
#33960=CARTESIAN_POINT ( 'NONE',  ( -3.500000000000002220, 15.47927405783632793, -68.57139747004409003 ) ) ;
#33961=CARTESIAN_POINT ( 'NONE',  ( 3.310556943750001313, 17.50000000000002132, -117.2641058028994792 ) ) ;
#33963=ORIENTED_EDGE ( 'NONE', *, *, #2669, .F. ) ;
#33965=ORIENTED_EDGE ( 'NONE', *, *, #24994, .T. ) ;
#33966=CARTESIAN_POINT ( 'NONE',  ( -3.500000000000001332, 17.50000000000002132, -109.9609808024215027 ) ) ;
#33967=CARTESIAN_POINT ( 'NONE',  ( 1.655278471875001101, 20.36702641396248836, -71.09743913623280775 ) ) ;
#33969=ORIENTED_EDGE ( 'NONE', *, *, #39361, .T. ) ;
#33970=EDGE_CURVE ( 'NONE', #39141, #23881, #27639, .T. ) ;
#33973=DIRECTION ( 'NONE',  ( -0.000000000000000000, 1.259100132267607459E-16, -1.000000000000000000 ) ) ;
#33977=ORIENTED_EDGE ( 'NONE', *, *, #6621, .F. ) ;
#33979=CARTESIAN_POINT ( 'NONE',  ( 1.655278471875001101, 20.36702641396249902, -138.0974391362327935 ) ) ;
#33980=VECTOR ( 'NONE', #38809, 1000.000000000000000 ) ;
#33981=CARTESIAN_POINT ( 'NONE',  ( 0.9378221735089281585, 14.00000000000002132, -119.6663226036829855 ) ) ;
#33983=CARTESIAN_POINT ( 'NONE',  ( 1.655278471875001101, 20.36702641396248481, -45.18493913623279923 ) ) ;
#33984=CARTESIAN_POINT ( 'NONE',  ( -3.310556943750002645, 15.58864905735836537, -33.76827246956613493 ) ) ;
#33985=CARTESIAN_POINT ( 'NONE',  ( -3.310556943750000425, 19.41135094264166483, -99.93493913623281344 ) ) ;
#33987=( BOUNDED_CURVE ( )  B_SPLINE_CURVE ( 2, ( #30191, #24038, #17012, #36361, #13601, #7651, #20202, #23613, #33605 ),
 .UNSPECIFIED., .F., .F. ) 
 B_SPLINE_CURVE_WITH_KNOTS ( ( 3, 2, 2, 2, 3 ),
 ( 0.3770833333333333259, 0.3777777777777777679, 0.3791666666666666519, 0.3805555555555555358, 0.3812499999999999778 ),
 .UNSPECIFIED. ) 
 CURVE ( )  GEOMETRIC_REPRESENTATION_ITEM ( )  RATIONAL_B_SPLINE_CURVE ( ( 0.9330127018922194093, 0.9330127018922194093, 1.000000000000000000, 0.8660254037844387076, 1.000000000000000000, 0.8660254037844387076, 1.000000000000000000, 0.9330127018922194093, 0.9330127018922194093 ) ) 
 REPRESENTATION_ITEM ( '' )  );
#33990=CARTESIAN_POINT ( 'NONE',  ( 2.340729813953370519E-16, 21.32270188528332255, -136.1016058028994564 ) ) ;
#33991=CYLINDRICAL_SURFACE ( 'NONE', #21666, 3.499999999999999556 ) ;
#33992=CARTESIAN_POINT ( 'NONE',  ( 3.500000000000001332, 17.50000000000001776, -98.46098080242150274 ) ) ;
#33993=CARTESIAN_POINT ( 'NONE',  ( 1.750000000000001110, 20.53108891324555785, -124.2943141357548456 ) ) ;
#33994=CARTESIAN_POINT ( 'NONE',  ( -3.500000000000001332, 17.50000000000001421, -61.65473080337742573 ) ) ;
#33995=CARTESIAN_POINT ( 'NONE',  ( 1.750000000000001110, 20.53108891324555429, -87.98806413671076143 ) ) ;
#33996=CARTESIAN_POINT ( 'NONE',  ( 3.310556943750001313, 17.50000000000001421, -70.35160580289947063 ) ) ;
#34000=CARTESIAN_POINT ( 'NONE',  ( -1.750000000000002220, 14.46891108675448656, -119.7943141357548313 ) ) ;
#34001=CARTESIAN_POINT ( 'NONE',  ( -3.500000000000002220, 15.47927405783632260, -50.87764746908815994 ) ) ;
#34002=CARTESIAN_POINT ( 'NONE',  ( -3.310556943750002201, 15.58864905735837780, -118.6807724695661364 ) ) ;
#34003=DIRECTION ( 'NONE',  ( -0.000000000000000000, 1.259100132267607459E-16, -1.000000000000000000 ) ) ;
#34005=ADVANCED_FACE ( 'NONE', ( #21332 ), #11748, .T. ) ;
#34007=CARTESIAN_POINT ( 'NONE',  ( 2.474675557024783212E-16, 21.54145188432740099, -113.9047308033774328 ) ) ;
#34010=DIRECTION ( 'NONE',  ( -0.000000000000000000, 1.259100132267607459E-16, -1.000000000000000000 ) ) ;
#34011=CARTESIAN_POINT ( 'NONE',  ( -1.394453263437886604E-15, 14.00000000000001066, -37.71098080242150985 ) ) ;
#34014=CARTESIAN_POINT ( 'NONE',  ( 1.655278471874998436, 14.63297358603754361, -69.43077246956613635 ) ) ;
#34017=CARTESIAN_POINT ( 'NONE',  ( 4.286263797015737581E-16, 14.00000000000002487, -149.5231586289125687 ) ) ;
#34018=VERTEX_POINT ( 'NONE', #34307 ) ;
#34020=CARTESIAN_POINT ( 'NONE',  ( -1.394453263437886604E-15, 14.00000000000001421, -63.71098080242150274 ) ) ;
#34021=CARTESIAN_POINT ( 'NONE',  ( -3.310556943750000425, 19.41135094264166483, -84.84743913623279354 ) ) ;
#34024=AXIS2_PLACEMENT_3D ( 'NONE', #25608, #6243, #3055 ) ;
#34028=DIRECTION ( 'NONE',  ( -0.000000000000000000, 1.259100132267607459E-16, -1.000000000000000000 ) ) ;
#34029=CARTESIAN_POINT ( 'NONE',  ( -3.500000000000000000, 19.52072594216371826, -126.7380641367107614 ) ) ;
#34030=CARTESIAN_POINT ( 'NONE',  ( -3.310556943750000425, 19.41135094264166128, -46.93493913623279923 ) ) ;
#34031=CARTESIAN_POINT ( 'NONE',  ( 3.310556943750001313, 17.50000000000002132, -116.3516058028994706 ) ) ;
#34033=CARTESIAN_POINT ( 'NONE',  ( 3.500000000000001776, 19.52072594216371826, -122.0713974700441042 ) ) ;
#34035=CARTESIAN_POINT ( 'NONE',  ( -3.310556943750001313, 17.50000000000001066, -33.76410580289947205 ) ) ;
#34036=CARTESIAN_POINT ( 'NONE',  ( 3.310556943750001313, 19.41135094264166128, -66.26827246956612782 ) ) ;
#34037=CARTESIAN_POINT ( 'NONE',  ( 1.750000000000001110, 20.53108891324555785, -111.2943141357548456 ) ) ;
#34039=CARTESIAN_POINT ( 'NONE',  ( -1.655278471874999990, 20.36702641396249192, -97.93077246956613635 ) ) ;
#34040=CARTESIAN_POINT ( 'NONE',  ( -3.500000000000000000, 19.52072594216370760, -56.73806413671076143 ) ) ;
#34042=CARTESIAN_POINT ( 'NONE',  ( 3.500000000000000000, 15.47927405783632260, -66.54431413575484555 ) ) ;
#34044=CARTESIAN_POINT ( 'NONE',  ( 3.310556943750001313, 19.41135094264165772, -31.18077246956614701 ) ) ;
#34045=CARTESIAN_POINT ( 'NONE',  ( 1.655278471874998436, 14.63297358603754539, -92.51827246956611361 ) ) ;
#34046=CARTESIAN_POINT ( 'NONE',  ( -1.749999999999999778, 20.53108891324555074, -51.82139747004409003 ) ) ;
#34048=CARTESIAN_POINT ( 'NONE',  ( -7.022189441860112050E-16, 13.67729811471672541, -105.6016058028994706 ) ) ;
#34049=CARTESIAN_POINT ( 'NONE',  ( -3.310556943750001313, 17.50000000000001066, -38.85160580289946353 ) ) ;
#34055=CARTESIAN_POINT ( 'NONE',  ( -1.394453263437886604E-15, 14.00000000000001066, -49.71098080242150274 ) ) ;
#34056=CARTESIAN_POINT ( 'NONE',  ( -3.310556943750000425, 19.41135094264166838, -90.84743913623279354 ) ) ;
#34057=( BOUNDED_CURVE ( )  B_SPLINE_CURVE ( 2, ( #13652, #16850, #26632, #29814, #3445, #7280, #13869, #38975, #25071 ),
 .UNSPECIFIED., .F., .T. ) 
 B_SPLINE_CURVE_WITH_KNOTS ( ( 3, 2, 2, 2, 3 ),
 ( 0.1645833333333333315, 0.1652777777777777735, 0.1666666666666666574, 0.1680555555555555691, 0.1687500000000000111 ),
 .UNSPECIFIED. ) 
 CURVE ( )  GEOMETRIC_REPRESENTATION_ITEM ( )  RATIONAL_B_SPLINE_CURVE ( ( 0.9330127018922194093, 0.9330127018922194093, 1.000000000000000000, 0.8660254037844387076, 1.000000000000000000, 0.8660254037844387076, 1.000000000000000000, 0.9330127018922194093, 0.9330127018922194093 ) ) 
 REPRESENTATION_ITEM ( '' )  );
#34060=EDGE_LOOP ( 'NONE', ( #7587, #30772, #14125, #23361 ) ) ;
#34061=DIRECTION ( 'NONE',  ( -0.000000000000000000, 1.259100132267607459E-16, -1.000000000000000000 ) ) ;
#34062=CARTESIAN_POINT ( 'NONE',  ( -3.500000000000001332, 17.50000000000001421, -64.96098080242150274 ) ) ;
#34065=EDGE_CURVE ( 'NONE', #37987, #20991, #21922, .T. ) ;
#34071=CARTESIAN_POINT ( 'NONE',  ( 4.286263797015737581E-16, 14.00000000000002487, -149.5231586289125687 ) ) ;
#34074=EDGE_LOOP ( 'NONE', ( #20205, #5394, #13408, #33763 ) ) ;
#34075=CARTESIAN_POINT ( 'NONE',  ( -1.394453263437886604E-15, 14.00000000000001776, -94.40473080337743284 ) ) ;
#34077=CYLINDRICAL_SURFACE ( 'NONE', #35735, 3.499999999999999556 ) ;
#34078=CARTESIAN_POINT ( 'NONE',  ( -1.655278471874999990, 20.36702641396249902, -138.9307724695661364 ) ) ;
#34079=CARTESIAN_POINT ( 'NONE',  ( -1.750000000000002220, 14.46891108675448834, -132.4880641367107614 ) ) ;
#34080=CARTESIAN_POINT ( 'NONE',  ( 3.500000000000001332, 17.50000000000001421, -54.46098080242150985 ) ) ;
#34081=CARTESIAN_POINT ( 'NONE',  ( 1.655278471875001101, 20.36702641396249547, -129.1849391362327992 ) ) ;
#34082=CARTESIAN_POINT ( 'NONE',  ( 3.310556943750001313, 17.50000000000001421, -56.35160580289947063 ) ) ;
#34085=CARTESIAN_POINT ( 'NONE',  ( 3.500000000000001332, 17.50000000000002487, -134.1547308033774186 ) ) ;
#34087=CARTESIAN_POINT ( 'NONE',  ( -3.500000000000002220, 15.47927405783633503, -127.8776474690881599 ) ) ;
#34088=CARTESIAN_POINT ( 'NONE',  ( -3.310556943750000425, 19.41135094264166838, -114.8474391362327935 ) ) ;
#34091=CARTESIAN_POINT ( 'NONE',  ( 1.750000000000001110, 20.53108891324555429, -79.29431413575484555 ) ) ;
#34092=CARTESIAN_POINT ( 'NONE',  ( 3.500000000000001332, 17.50000000000001421, -51.46098080242150985 ) ) ;
#34093=CARTESIAN_POINT ( 'NONE',  ( -1.655278471874999990, 20.36702641396248836, -47.93077246956614346 ) ) ;
#34094=CARTESIAN_POINT ( 'NONE',  ( 1.655278471874998436, 14.63297358603754716, -107.5182724695661278 ) ) ;
#34096=CARTESIAN_POINT ( 'NONE',  ( -3.500000000000000000, 19.52072594216371115, -99.73806413671077564 ) ) ;
#34098=CARTESIAN_POINT ( 'NONE',  ( 2.340729813953370519E-16, 21.32270188528331900, -129.1016058028994848 ) ) ;
#34101=CARTESIAN_POINT ( 'NONE',  ( 4.648177544792955347E-16, 21.00000000000001066, -25.21098080242150985 ) ) ;
#34103=CARTESIAN_POINT ( 'NONE',  ( -3.310556943750002645, 15.58864905735836892, -58.76827246956612782 ) ) ;
#34104=VERTEX_POINT ( 'NONE', #18558 ) ;
#34107=CARTESIAN_POINT ( 'NONE',  ( -3.310556943750000425, 19.41135094264166838, -78.93493913623279923 ) ) ;
#34108=CARTESIAN_POINT ( 'NONE',  ( 4.648177544792955347E-16, 21.00000000000001776, -93.90473080337743284 ) ) ;
#34110=CARTESIAN_POINT ( 'NONE',  ( 0.000000000000000000, 17.50000000000002487, -149.5231586289125687 ) ) ;
#34112=EDGE_CURVE ( 'NONE', #5882, #31863, #17343, .T. ) ;
#34114=CARTESIAN_POINT ( 'NONE',  ( -3.310556943750000425, 19.41135094264166128, -41.84743913623280065 ) ) ;
#34120=CARTESIAN_POINT ( 'NONE',  ( 3.310556943750001313, 19.41135094264166128, -49.18077246956614346 ) ) ;
#34121=ORIENTED_EDGE ( 'NONE', *, *, #5491, .F. ) ;
#34122=ORIENTED_EDGE ( 'NONE', *, *, #13735, .F. ) ;
#34124=CARTESIAN_POINT ( 'NONE',  ( 3.500000000000000000, 15.47927405783631727, -24.54431413575485266 ) ) ;
#34126=CARTESIAN_POINT ( 'NONE',  ( 0.000000000000000000, 17.50000000000002487, -149.5231586289125687 ) ) ;
#34128=DIRECTION ( 'NONE',  ( 0.000000000000000000, 1.000000000000000000, 0.000000000000000000 ) ) ;
#34129=CARTESIAN_POINT ( 'NONE',  ( -3.500000000000001332, 17.50000000000001066, -36.96098080242150985 ) ) ;
#34131=CARTESIAN_POINT ( 'NONE',  ( 7.367361408496833051E-14, 14.00000000000002132, -110.4047308033774328 ) ) ;
#34133=CARTESIAN_POINT ( 'NONE',  ( -1.655278471874999990, 20.36702641396248481, -26.01827246956613138 ) ) ;
#34134=CARTESIAN_POINT ( 'NONE',  ( 1.655278471875001101, 20.36702641396249902, -131.0974391362328220 ) ) ;
#34137=CARTESIAN_POINT ( 'NONE',  ( 0.9378221735089281585, 14.00000000000000888, -29.36007260463891910 ) ) ;
#34138=CARTESIAN_POINT ( 'NONE',  ( 2.340729813953370519E-16, 21.32270188528331900, -122.1016058028994564 ) ) ;
#34139=LINE ( 'NONE', #21167, #18681 ) ;
#34140=CARTESIAN_POINT ( 'NONE',  ( 3.500000000000000000, 15.47927405783632082, -38.23806413671076854 ) ) ;
#34142=CARTESIAN_POINT ( 'NONE',  ( 0.9378221735089281585, 14.00000000000001066, -46.36007260463890844 ) ) ;
#34143=CARTESIAN_POINT ( 'NONE',  ( 0.9378221735089300459, 21.00000000000002487, -130.2556390011600342 ) ) ;
#34144=CARTESIAN_POINT ( 'NONE',  ( 1.655278471874998436, 14.63297358603755249, -142.5182724695661420 ) ) ;
#34145=CARTESIAN_POINT ( 'NONE',  ( 1.749999999999998224, 14.46891108675447946, -72.32139747004409003 ) ) ;
#34147=CARTESIAN_POINT ( 'NONE',  ( 4.648177544792955347E-16, 21.00000000000001066, -34.21098080242150985 ) ) ;
#34149=CARTESIAN_POINT ( 'NONE',  ( 3.310556943749999981, 15.58864905735836182, -53.43493913623279923 ) ) ;
#34152=CARTESIAN_POINT ( 'NONE',  ( 2.340729813953370519E-16, 21.32270188528331190, -76.10160580289945642 ) ) ;
#34154=CARTESIAN_POINT ( 'NONE',  ( -7.022189441860112050E-16, 13.67729811471672541, -105.5141058028994649 ) ) ;
#34155=CARTESIAN_POINT ( 'NONE',  ( -1.655278471875002211, 14.63297358603754539, -74.59743913623280775 ) ) ;
#34156=ORIENTED_EDGE ( 'NONE', *, *, #5631, .T. ) ;
#34157=CARTESIAN_POINT ( 'NONE',  ( 3.310556943750001313, 19.41135094264166838, -97.26827246956612782 ) ) ;
#34159=CARTESIAN_POINT ( 'NONE',  ( -3.500000000000001332, 17.50000000000001066, -32.96098080242150274 ) ) ;
#34160=CARTESIAN_POINT ( 'NONE',  ( 4.648177544792955347E-16, 21.00000000000001421, -52.21098080242150985 ) ) ;
#34162=CARTESIAN_POINT ( 'NONE',  ( 3.310556943750001313, 19.41135094264166483, -58.18077246956614346 ) ) ;
#34164=CARTESIAN_POINT ( 'NONE',  ( -1.655278471875002211, 14.63297358603755072, -113.5974391362328078 ) ) ;
#34165=ORIENTED_EDGE ( 'NONE', *, *, #39186, .T. ) ;
#34166=ORIENTED_EDGE ( 'NONE', *, *, #20013, .T. ) ;
#34168=VERTEX_POINT ( 'NONE', #13015 ) ;
#34169=CARTESIAN_POINT ( 'NONE',  ( 0.9378221735089281585, 14.00000000000000888, -33.66632260368299256 ) ) ;
#34170=CARTESIAN_POINT ( 'NONE',  ( 3.310556943749999981, 15.58864905735836537, -61.34743913623280775 ) ) ;
#34171=VERTEX_POINT ( 'NONE', #35348 ) ;
#34174=FACE_OUTER_BOUND ( 'NONE', #19481, .T. ) ;
#34176=EDGE_CURVE ( 'NONE', #4551, #31391, #40683, .T. ) ;
#34183=CARTESIAN_POINT ( 'NONE',  ( 3.310556943749999981, 15.58864905735837425, -131.3474391362328220 ) ) ;
#34184=CARTESIAN_POINT ( 'NONE',  ( -1.394453263437886604E-15, 14.00000000000002132, -115.7109808024214885 ) ) ;
#34185=CARTESIAN_POINT ( 'NONE',  ( -1.655278471874999990, 20.36702641396248481, -39.01827246956612782 ) ) ;
#34186=CARTESIAN_POINT ( 'NONE',  ( 1.655278471874998436, 14.63297358603753828, -32.51827246956613493 ) ) ;
#34187=CARTESIAN_POINT ( 'NONE',  ( 2.340729813953370519E-16, 21.32270188528331190, -92.10160580289947063 ) ) ;
#34188=CARTESIAN_POINT ( 'NONE',  ( -7.022189441860112050E-16, 13.67729811471672896, -142.5141058028994507 ) ) ;
#34189=ORIENTED_EDGE ( 'NONE', *, *, #17160, .F. ) ;
#34190=EDGE_CURVE ( 'NONE', #14503, #18588, #36587, .T. ) ;
#34192=CARTESIAN_POINT ( 'NONE',  ( -3.310556943750001313, 17.50000000000002487, -139.8516058028994564 ) ) ;
#34194=CARTESIAN_POINT ( 'NONE',  ( -3.500000000000002220, 15.47927405783632793, -94.87764746908815994 ) ) ;
#34196=CARTESIAN_POINT ( 'NONE',  ( -1.750000000000002220, 14.46891108675447946, -61.48806413671076143 ) ) ;
#34197=CARTESIAN_POINT ( 'NONE',  ( 3.500000000000000000, 15.47927405783632615, -86.23806413671076143 ) ) ;
#34198=CARTESIAN_POINT ( 'NONE',  ( -3.310556943750000425, 19.41135094264166483, -67.93493913623279923 ) ) ;
#34202=CARTESIAN_POINT ( 'NONE',  ( 0.9378221735089300459, 21.00000000000002132, -110.2556390011600200 ) ) ;
#34203=CARTESIAN_POINT ( 'NONE',  ( -7.424026671074350129E-16, 13.45854811567263276, -47.71098080242150274 ) ) ;
#34204=CARTESIAN_POINT ( 'NONE',  ( 1.655278471875001101, 20.36702641396249547, -118.0974391362328078 ) ) ;
#34205=DIRECTION ( 'NONE',  ( -0.000000000000000000, 1.259100132267607459E-16, -1.000000000000000000 ) ) ;
#34206=CARTESIAN_POINT ( 'NONE',  ( 0.9378221735089630196, 14.00000000000003730, -95.66632260368297125 ) ) ;
#34209=CARTESIAN_POINT ( 'NONE',  ( 3.500000000000000000, 15.47927405783632970, -112.2380641367107472 ) ) ;
#34210=CARTESIAN_POINT ( 'NONE',  ( 3.500000000000001332, 17.50000000000001421, -55.15473080337743284 ) ) ;
#34215=CARTESIAN_POINT ( 'NONE',  ( 3.310556943750001313, 17.50000000000001421, -72.26410580289947916 ) ) ;
#34217=CARTESIAN_POINT ( 'NONE',  ( 0.000000000000000000, 17.50000000000002487, -149.5231586289125687 ) ) ;
#34219=CARTESIAN_POINT ( 'NONE',  ( -3.310556943750001313, 17.50000000000001066, -23.76410580289947561 ) ) ;
#34221=CARTESIAN_POINT ( 'NONE',  ( -3.310556943750001313, 17.50000000000001776, -83.76410580289947916 ) ) ;
#34222=ORIENTED_EDGE ( 'NONE', *, *, #7390, .F. ) ;
#34223=ORIENTED_EDGE ( 'NONE', *, *, #1325, .F. ) ;
#34224=( BOUNDED_CURVE ( )  B_SPLINE_CURVE ( 2, ( #16426, #22799, #6217, #3234, #38544, #34932, #9625, #38755, #22375 ),
 .UNSPECIFIED., .F., .T. ) 
 B_SPLINE_CURVE_WITH_KNOTS ( ( 3, 2, 2, 2, 3 ),
 ( 0.05208333333333333565, 0.05277777777777777762, 0.05416666666666666852, 0.05555555555555555247, 0.05625000000000000139 ),
 .UNSPECIFIED. ) 
 CURVE ( )  GEOMETRIC_REPRESENTATION_ITEM ( )  RATIONAL_B_SPLINE_CURVE ( ( 0.9330127018922192983, 0.9330127018922196314, 1.000000000000000000, 0.8660254037844387076, 1.000000000000000000, 0.8660254037844387076, 1.000000000000000000, 0.9330127018922189652, 0.9330127018922192983 ) ) 
 REPRESENTATION_ITEM ( '' )  );
#34227=CARTESIAN_POINT ( 'NONE',  ( 4.648177544792955347E-16, 21.00000000000001776, -102.2109808024215027 ) ) ;
#34233=CARTESIAN_POINT ( 'NONE',  ( 3.310556943750001313, 19.41135094264166128, -50.26827246956614204 ) ) ;
#34234=CARTESIAN_POINT ( 'NONE',  ( 3.310556943750001313, 17.50000000000002132, -110.3516058028994564 ) ) ;
#34235=ORIENTED_EDGE ( 'NONE', *, *, #11218, .T. ) ;
#34236=CARTESIAN_POINT ( 'NONE',  ( 1.655278471874998436, 14.63297358603753828, -33.43077246956615056 ) ) ;
#34238=CARTESIAN_POINT ( 'NONE',  ( 1.655278471874998436, 14.63297358603754184, -67.51827246956612782 ) ) ;
#34239=CARTESIAN_POINT ( 'NONE',  ( -7.424026671074350129E-16, 13.45854811567263987, -112.7109808024215027 ) ) ;
#34241=CARTESIAN_POINT ( 'NONE',  ( 1.655278471874998436, 14.63297358603754539, -94.43077246956613635 ) ) ;
#34242=CARTESIAN_POINT ( 'NONE',  ( -1.749999999999999778, 20.53108891324555074, -47.82139747004410424 ) ) ;
#34243=CARTESIAN_POINT ( 'NONE',  ( 0.000000000000000000, 17.50000000000002487, -149.5231586289125687 ) ) ;
#34244=LINE ( 'NONE', #37852, #1478 ) ;
#34246=CARTESIAN_POINT ( 'NONE',  ( -1.749999999999999778, 20.53108891324555074, -66.12764746908817415 ) ) ;
#34248=CARTESIAN_POINT ( 'NONE',  ( 3.310556943750001313, 19.41135094264165772, -33.18077246956615056 ) ) ;
#34249=CARTESIAN_POINT ( 'NONE',  ( 3.310556943750001313, 19.41135094264166483, -92.26827246956612782 ) ) ;
#34250=EDGE_CURVE ( 'NONE', #36594, #29085, #8635, .T. ) ;
#34251=CARTESIAN_POINT ( 'NONE',  ( -3.500000000000000888, 19.52072594216370760, -53.73806413671077564 ) ) ;
#34253=CARTESIAN_POINT ( 'NONE',  ( -3.310556943750001313, 17.50000000000002132, -105.8516058028994564 ) ) ;
#34254=CARTESIAN_POINT ( 'NONE',  ( -3.310556943750000425, 19.41135094264166128, -36.93493913623279923 ) ) ;
#34262=CARTESIAN_POINT ( 'NONE',  ( -1.655278471874999990, 20.36702641396249192, -89.93077246956613635 ) ) ;
#34265=ORIENTED_EDGE ( 'NONE', *, *, #19775, .F. ) ;
#34267=VECTOR ( 'NONE', #30403, 1000.000000000000000 ) ;
#34270=CARTESIAN_POINT ( 'NONE',  ( 4.648177544792955347E-16, 21.00000000000001066, -31.21098080242150630 ) ) ;
#34273=ORIENTED_EDGE ( 'NONE', *, *, #34527, .T. ) ;
#34283=CARTESIAN_POINT ( 'NONE',  ( 2.340729813953370519E-16, 21.32270188528332255, -137.0141058028994792 ) ) ;
#34284=CARTESIAN_POINT ( 'NONE',  ( 4.648177544792955347E-16, 21.00000000000002487, -133.2109808024214885 ) ) ;
#34287=CARTESIAN_POINT ( 'NONE',  ( -1.655278471875002211, 14.63297358603755249, -127.6849391362327992 ) ) ;
#34288=CARTESIAN_POINT ( 'NONE',  ( 1.655278471874998436, 14.63297358603754006, -53.51827246956612782 ) ) ;
#34289=ORIENTED_EDGE ( 'NONE', *, *, #37800, .F. ) ;
#34291=CARTESIAN_POINT ( 'NONE',  ( -3.500000000000001332, 17.50000000000002487, -136.6547308033774186 ) ) ;
#34295=CARTESIAN_POINT ( 'NONE',  ( -1.749999999999999778, 20.53108891324556140, -130.1276474690881741 ) ) ;
#34296=CARTESIAN_POINT ( 'NONE',  ( 1.655278471874998436, 14.63297358603754894, -111.4307724695661506 ) ) ;
#34297=ADVANCED_FACE ( 'NONE', ( #32365 ), #31943, .T. ) ;
#34299=( BOUNDED_CURVE ( )  B_SPLINE_CURVE ( 2, ( #25549, #9375, #5969, #41077, #12350, #22340, #35317, #38293, #6181 ),
 .UNSPECIFIED., .F., .F. ) 
 B_SPLINE_CURVE_WITH_KNOTS ( ( 3, 2, 2, 2, 3 ),
 ( 0.1812499999999999944, 0.1819444444444444364, 0.1833333333333333204, 0.1847222222222222321, 0.1854166666666666741 ),
 .UNSPECIFIED. ) 
 CURVE ( )  GEOMETRIC_REPRESENTATION_ITEM ( )  RATIONAL_B_SPLINE_CURVE ( ( 0.9330127018922194093, 0.9330127018922194093, 1.000000000000000000, 0.8660254037844387076, 1.000000000000000000, 0.8660254037844387076, 1.000000000000000000, 0.9330127018922194093, 0.9330127018922194093 ) ) 
 REPRESENTATION_ITEM ( '' )  );
#34302=CARTESIAN_POINT ( 'NONE',  ( -1.749999999999999778, 20.53108891324555429, -80.12764746908817415 ) ) ;
#34304=CARTESIAN_POINT ( 'NONE',  ( 4.648177544792955347E-16, 21.00000000000001776, -83.21098080242150274 ) ) ;
#34305=CARTESIAN_POINT ( 'NONE',  ( -1.655278471875002211, 14.63297358603754184, -50.59743913623280775 ) ) ;
#34306=CARTESIAN_POINT ( 'NONE',  ( -3.310556943750002645, 15.58864905735837425, -105.7682724695661278 ) ) ;
#34307=CARTESIAN_POINT ( 'NONE',  ( 0.000000000000000000, 17.50000000000002487, -149.5231586289125687 ) ) ;
#34308=CARTESIAN_POINT ( 'NONE',  ( -3.500000000000002220, 15.47927405783632437, -42.57139747004410424 ) ) ;
#34310=CARTESIAN_POINT ( 'NONE',  ( -1.655278471875002211, 14.63297358603755072, -120.6849391362327992 ) ) ;
#34313=CARTESIAN_POINT ( 'NONE',  ( -0.9378221735089136146, 14.00000000000001066, -116.7556390011600200 ) ) ;
#34314=CARTESIAN_POINT ( 'NONE',  ( 4.648177544792955347E-16, 21.00000000000001421, -57.90473080337742573 ) ) ;
#34315=CARTESIAN_POINT ( 'NONE',  ( 3.310556943750001313, 19.41135094264166128, -57.26827246956612782 ) ) ;
#34316=ORIENTED_EDGE ( 'NONE', *, *, #9679, .T. ) ;
#34317=CARTESIAN_POINT ( 'NONE',  ( 3.310556943750001313, 17.50000000000001421, -74.35160580289947063 ) ) ;
#34318=CARTESIAN_POINT ( 'NONE',  ( -1.394453263437886604E-15, 14.00000000000001066, -40.71098080242150274 ) ) ;
#34324=CARTESIAN_POINT ( 'NONE',  ( 1.655278471875001101, 20.36702641396248481, -38.09743913623281486 ) ) ;
#34326=ORIENTED_EDGE ( 'NONE', *, *, #17820, .T. ) ;
#34327=VECTOR ( 'NONE', #14364, 1000.000000000000000 ) ;
#34331=CARTESIAN_POINT ( 'NONE',  ( 1.655278471874998436, 14.63297358603754006, -46.43077246956614346 ) ) ;
#34334=CARTESIAN_POINT ( 'NONE',  ( 0.000000000000000000, 17.50000000000002487, -149.5231586289125687 ) ) ;
#34335=( GEOMETRIC_REPRESENTATION_CONTEXT ( 3 ) GLOBAL_UNCERTAINTY_ASSIGNED_CONTEXT ( ( #29687 ) ) GLOBAL_UNIT_ASSIGNED_CONTEXT ( ( #14938, #5572, #5786 ) ) REPRESENTATION_CONTEXT ( 'NONE', 'WORKASPACE' ) );
#34336=CYLINDRICAL_SURFACE ( 'NONE', #31603, 3.499999999999999556 ) ;
#34340=EDGE_CURVE ( 'NONE', #12462, #7438, #30386, .T. ) ;
#34341=CARTESIAN_POINT ( 'NONE',  ( 3.500000000000001332, 19.52072594216370405, -43.37764746908817415 ) ) ;
#34342=CARTESIAN_POINT ( 'NONE',  ( 3.500000000000001332, 17.50000000000001066, -36.46098080242150985 ) ) ;
#34344=CARTESIAN_POINT ( 'NONE',  ( 3.500000000000000000, 15.47927405783632615, -70.54431413575484555 ) ) ;
#34346=CARTESIAN_POINT ( 'NONE',  ( 1.655278471875001101, 20.36702641396248481, -25.18493913623280633 ) ) ;
#34348=CARTESIAN_POINT ( 'NONE',  ( 1.655278471875001101, 20.36702641396249547, -129.0974391362328220 ) ) ;
#34349=EDGE_CURVE ( 'NONE', #28199, #15451, #10253, .T. ) ;
#34352=FACE_OUTER_BOUND ( 'NONE', #12937, .T. ) ;
#34354=CARTESIAN_POINT ( 'NONE',  ( -1.655278471874999990, 20.36702641396249547, -124.0182724695661278 ) ) ;
#34356=CARTESIAN_POINT ( 'NONE',  ( -7.424026671074350129E-16, 13.45854811567263098, -38.40473080337743284 ) ) ;
#34357=CARTESIAN_POINT ( 'NONE',  ( -0.9378221735089291577, 21.00000000000001421, -49.86007260463892266 ) ) ;
#34359=CARTESIAN_POINT ( 'NONE',  ( 3.310556943750001313, 19.41135094264167549, -140.2682724695661420 ) ) ;
#34360=CARTESIAN_POINT ( 'NONE',  ( 2.474675557024783212E-16, 21.54145188432739388, -71.90473080337743284 ) ) ;
#34362=CARTESIAN_POINT ( 'NONE',  ( 2.340729813953370519E-16, 21.32270188528331190, -48.10160580289946353 ) ) ;
#34364=CARTESIAN_POINT ( 'NONE',  ( 0.9378221735089281585, 14.00000000000002132, -104.6663226036829997 ) ) ;
#34365=CARTESIAN_POINT ( 'NONE',  ( 1.655278471875001101, 20.36702641396249192, -75.18493913623279923 ) ) ;
#34367=CARTESIAN_POINT ( 'NONE',  ( -3.310556943750001313, 17.50000000000002132, -105.7641058028994649 ) ) ;
#34368=CARTESIAN_POINT ( 'NONE',  ( -3.310556943750001313, 17.50000000000001421, -68.76410580289947916 ) ) ;
#34369=VERTEX_POINT ( 'NONE', #8050 ) ;
#34370=CARTESIAN_POINT ( 'NONE',  ( 1.655278471874998436, 14.63297358603754716, -96.51827246956612782 ) ) ;
#34373=CARTESIAN_POINT ( 'NONE',  ( 3.500000000000001332, 17.50000000000001066, -26.46098080242151340 ) ) ;
#34375=CARTESIAN_POINT ( 'NONE',  ( 2.340729813953370519E-16, 21.32270188528331190, -54.01410580289948626 ) ) ;
#34376=CARTESIAN_POINT ( 'NONE',  ( -1.749999999999999778, 20.53108891324556140, -137.8213974700441042 ) ) ;
#34377=CARTESIAN_POINT ( 'NONE',  ( 3.310556943749999981, 15.58864905735837247, -110.3474391362327935 ) ) ;
#34378=VERTEX_POINT ( 'NONE', #20608 ) ;
#34379=ORIENTED_EDGE ( 'NONE', *, *, #30701, .F. ) ;
#34383=CARTESIAN_POINT ( 'NONE',  ( 3.310556943750001313, 19.41135094264166128, -61.18077246956615056 ) ) ;
#34384=ORIENTED_EDGE ( 'NONE', *, *, #5094, .T. ) ;
#34385=VERTEX_POINT ( 'NONE', #39750 ) ;
#34387=CARTESIAN_POINT ( 'NONE',  ( -3.500000000000000000, 19.52072594216371826, -142.7380641367107614 ) ) ;
#34390=VERTEX_POINT ( 'NONE', #7422 ) ;
#34392=CARTESIAN_POINT ( 'NONE',  ( -1.655278471875002211, 14.63297358603755249, -129.5974391362328220 ) ) ;
#34395=CARTESIAN_POINT ( 'NONE',  ( 1.655278471874998436, 14.63297358603753828, -37.51827246956612782 ) ) ;
#34396=CARTESIAN_POINT ( 'NONE',  ( -1.655278471874999990, 20.36702641396248481, -33.01827246956613493 ) ) ;
#34397=CARTESIAN_POINT ( 'NONE',  ( 2.340729813953370519E-16, 21.32270188528331190, -95.10160580289944221 ) ) ;
#34398=CARTESIAN_POINT ( 'NONE',  ( -1.749999999999999778, 20.53108891324554719, -26.82139747004409713 ) ) ;
#34399=VERTEX_POINT ( 'NONE', #23597 ) ;
#34401=CARTESIAN_POINT ( 'NONE',  ( -3.310556943750000425, 19.41135094264167549, -137.9349391362327708 ) ) ;
#34403=CARTESIAN_POINT ( 'NONE',  ( 2.474675557024783212E-16, 21.54145188432739744, -95.21098080242150274 ) ) ;
#34404=CARTESIAN_POINT ( 'NONE',  ( -1.750000000000002220, 14.46891108675448656, -122.7943141357548456 ) ) ;
#34405=CARTESIAN_POINT ( 'NONE',  ( 3.310556943750001313, 17.50000000000001421, -59.26410580289947916 ) ) ;
#34407=CARTESIAN_POINT ( 'NONE',  ( -3.500000000000001332, 17.50000000000001776, -87.65473080337743284 ) ) ;
#34408=CARTESIAN_POINT ( 'NONE',  ( -3.310556943750002201, 15.58864905735837070, -69.76827246956612782 ) ) ;
#34413=CARTESIAN_POINT ( 'NONE',  ( -3.500000000000002220, 15.47927405783632260, -48.87764746908818125 ) ) ;
#34414=CARTESIAN_POINT ( 'NONE',  ( -3.310556943750001313, 17.50000000000002132, -119.7641058028994792 ) ) ;
#34415=CYLINDRICAL_SURFACE ( 'NONE', #32577, 3.499999999999999556 ) ;
#34419=CARTESIAN_POINT ( 'NONE',  ( -3.500000000000000888, 19.52072594216371826, -111.7380641367107756 ) ) ;
#34421=CARTESIAN_POINT ( 'NONE',  ( -0.9378221735089291577, 21.00000000000001776, -83.86007260463891555 ) ) ;
#34425=CARTESIAN_POINT ( 'NONE',  ( 3.310556943750001313, 17.50000000000001421, -70.26410580289947916 ) ) ;
#34427=DIRECTION ( 'NONE',  ( -0.000000000000000000, 1.259100132267607459E-16, -1.000000000000000000 ) ) ;
#34429=CARTESIAN_POINT ( 'NONE',  ( 3.310556943750001313, 17.50000000000001066, -26.26410580289947916 ) ) ;
#34431=CARTESIAN_POINT ( 'NONE',  ( -7.022189441860112050E-16, 13.67729811471672186, -78.51410580289946495 ) ) ;
#34432=ORIENTED_EDGE ( 'NONE', *, *, #24409, .T. ) ;
#34434=CYLINDRICAL_SURFACE ( 'NONE', #40503, 3.499999999999999556 ) ;
#34437=CARTESIAN_POINT ( 'NONE',  ( 1.750000000000001110, 20.53108891324555785, -102.2943141357548456 ) ) ;
#34438=ADVANCED_FACE ( 'NONE', ( #40584 ), #4448, .T. ) ;
#34439=EDGE_LOOP ( 'NONE', ( #19189, #22587, #25859, #37316 ) ) ;
#34441=CARTESIAN_POINT ( 'NONE',  ( -1.655278471875002211, 14.63297358603754184, -49.68493913623279923 ) ) ;
#34442=CARTESIAN_POINT ( 'NONE',  ( 3.310556943750001313, 17.50000000000002132, -107.3516058028994564 ) ) ;
#34444=CARTESIAN_POINT ( 'NONE',  ( 1.655278471874998436, 14.63297358603753828, -35.43077246956613635 ) ) ;
#34445=CARTESIAN_POINT ( 'NONE',  ( -3.310556943750002645, 15.58864905735836892, -61.76827246956613493 ) ) ;
#34446=CARTESIAN_POINT ( 'NONE',  ( -3.500000000000000888, 19.52072594216371826, -112.0443141357548456 ) ) ;
#34448=CARTESIAN_POINT ( 'NONE',  ( -7.022189441860112050E-16, 13.67729811471672541, -98.51410580289947916 ) ) ;
#34449=CARTESIAN_POINT ( 'NONE',  ( -3.500000000000001332, 17.50000000000001066, -25.96098080242151340 ) ) ;
#34452=CARTESIAN_POINT ( 'NONE',  ( 1.750000000000001110, 20.53108891324555074, -65.29431413575484555 ) ) ;
#34454=CARTESIAN_POINT ( 'NONE',  ( 3.310556943749999981, 15.58864905735836182, -31.34743913623280775 ) ) ;
#34456=CARTESIAN_POINT ( 'NONE',  ( -1.749999999999999778, 20.53108891324555074, -54.82139747004409713 ) ) ;
#34458=CARTESIAN_POINT ( 'NONE',  ( 1.655278471875001101, 20.36702641396249547, -107.1849391362327992 ) ) ;
#34459=CARTESIAN_POINT ( 'NONE',  ( 3.310556943750001313, 17.50000000000001066, -37.35160580289946353 ) ) ;
#34461=CARTESIAN_POINT ( 'NONE',  ( 3.500000000000001332, 17.50000000000001421, -53.46098080242150985 ) ) ;
#34465=CARTESIAN_POINT ( 'NONE',  ( -3.500000000000002220, 15.47927405783632437, -49.87764746908817415 ) ) ;
#34467=CARTESIAN_POINT ( 'NONE',  ( -3.310556943750000425, 19.41135094264166838, -85.84743913623279354 ) ) ;
#34468=DIRECTION ( 'NONE',  ( -0.000000000000000000, 1.259100132267607459E-16, -1.000000000000000000 ) ) ;
#34469=CARTESIAN_POINT ( 'NONE',  ( 0.9378221735089281585, 14.00000000000000711, -23.36007260463891200 ) ) ;
#34470=ORIENTED_EDGE ( 'NONE', *, *, #31572, .F. ) ;
#34472=CARTESIAN_POINT ( 'NONE',  ( -3.500000000000002220, 15.47927405783632437, -50.57139747004409003 ) ) ;
#34473=( BOUNDED_CURVE ( )  B_SPLINE_CURVE ( 2, ( #21996, #33781, #1450, #34549, #5410, #24784, #28582, #41569, #37953 ),
 .UNSPECIFIED., .F., .F. ) 
 B_SPLINE_CURVE_WITH_KNOTS ( ( 3, 2, 2, 2, 3 ),
 ( 0.3895833333333333370, 0.3902777777777777790, 0.3916666666666666630, 0.3930555555555555469, 0.3937499999999999889 ),
 .UNSPECIFIED. ) 
 CURVE ( )  GEOMETRIC_REPRESENTATION_ITEM ( )  RATIONAL_B_SPLINE_CURVE ( ( 0.9330127018922194093, 0.9330127018922194093, 1.000000000000000000, 0.8660254037844387076, 1.000000000000000000, 0.8660254037844387076, 1.000000000000000000, 0.9330127018922194093, 0.9330127018922194093 ) ) 
 REPRESENTATION_ITEM ( '' )  );
#34474=EDGE_LOOP ( 'NONE', ( #25334, #28361, #40192, #10000 ) ) ;
#34480=ORIENTED_EDGE ( 'NONE', *, *, #20859, .F. ) ;
#34487=ORIENTED_EDGE ( 'NONE', *, *, #9535, .F. ) ;
#34488=DIRECTION ( 'NONE',  ( -0.000000000000000000, 1.259100132267607459E-16, -1.000000000000000000 ) ) ;
#34489=ADVANCED_FACE ( 'NONE', ( #30174 ), #31017, .T. ) ;
#34490=CARTESIAN_POINT ( 'NONE',  ( 3.310556943749999981, 15.58864905735837780, -138.3474391362328220 ) ) ;
#34492=ORIENTED_EDGE ( 'NONE', *, *, #7412, .T. ) ;
#34494=CARTESIAN_POINT ( 'NONE',  ( -1.655278471875002211, 14.63297358603755249, -125.6849391362327992 ) ) ;
#34495=CARTESIAN_POINT ( 'NONE',  ( -3.310556943750002645, 15.58864905735836892, -57.76827246956613493 ) ) ;
#34496=ORIENTED_EDGE ( 'NONE', *, *, #16082, .F. ) ;
#34498=CARTESIAN_POINT ( 'NONE',  ( -3.500000000000001332, 17.50000000000002487, -137.6547308033774186 ) ) ;
#34500=CARTESIAN_POINT ( 'NONE',  ( 3.310556943750001313, 19.41135094264166483, -75.26827246956612782 ) ) ;
#34501=CARTESIAN_POINT ( 'NONE',  ( 3.500000000000000000, 15.47927405783633503, -129.5443141357548598 ) ) ;
#34502=CARTESIAN_POINT ( 'NONE',  ( -7.022189441860112050E-16, 13.67729811471672718, -112.5141058028994649 ) ) ;
#34506=CARTESIAN_POINT ( 'NONE',  ( -1.749999999999999778, 20.53108891324555429, -78.12764746908817415 ) ) ;
#34508=CARTESIAN_POINT ( 'NONE',  ( 2.340729813953370519E-16, 21.32270188528330479, -46.01410580289946495 ) ) ;
#34509=CARTESIAN_POINT ( 'NONE',  ( -7.022189441860112050E-16, 13.67729811471672541, -108.6016058028994422 ) ) ;
#34513=CARTESIAN_POINT ( 'NONE',  ( 3.310556943750001313, 17.50000000000002132, -123.3516058028994564 ) ) ;
#34514=CARTESIAN_POINT ( 'NONE',  ( 4.648177544792955347E-16, 21.00000000000002132, -119.9047308033774328 ) ) ;
#34519=CARTESIAN_POINT ( 'NONE',  ( 0.000000000000000000, 17.50000000000002487, -149.5231586289125687 ) ) ;
#34520=CARTESIAN_POINT ( 'NONE',  ( 3.310556943749999981, 15.58864905735836537, -57.43493913623279212 ) ) ;
#34522=CARTESIAN_POINT ( 'NONE',  ( -3.310556943750001313, 17.50000000000001776, -76.85160580289945642 ) ) ;
#34523=ADVANCED_FACE ( 'NONE', ( #17832 ), #30806, .T. ) ;
#34524=CARTESIAN_POINT ( 'NONE',  ( 0.000000000000000000, 21.00000000000002487, -149.5231586289125687 ) ) ;
#34525=CARTESIAN_POINT ( 'NONE',  ( 0.000000000000000000, 21.00000000000002487, -149.5231586289125687 ) ) ;
#34527=EDGE_CURVE ( 'NONE', #12774, #29810, #39299, .T. ) ;
#34529=CARTESIAN_POINT ( 'NONE',  ( 0.000000000000000000, 17.50000000000002487, -149.5231586289125687 ) ) ;
#34531=CARTESIAN_POINT ( 'NONE',  ( 3.310556943750001313, 19.41135094264166128, -42.18077246956614346 ) ) ;
#34534=ORIENTED_EDGE ( 'NONE', *, *, #28524, .F. ) ;
#34536=EDGE_CURVE ( 'NONE', #36906, #37838, #14439, .T. ) ;
#34537=CARTESIAN_POINT ( 'NONE',  ( 3.310556943749999981, 15.58864905735836182, -49.34743913623280775 ) ) ;
#34543=CYLINDRICAL_SURFACE ( 'NONE', #10505, 3.499999999999999556 ) ;
#34544=CARTESIAN_POINT ( 'NONE',  ( -1.750000000000002220, 14.46891108675447590, -36.79431413575484555 ) ) ;
#34545=( BOUNDED_CURVE ( )  B_SPLINE_CURVE ( 2, ( #18473, #31650, #37826, #24657, #15503, #18057, #8898, #24446, #11660 ),
 .UNSPECIFIED., .F., .F. ) 
 B_SPLINE_CURVE_WITH_KNOTS ( ( 3, 2, 2, 2, 3 ),
 ( 0.6145833333333333703, 0.6152777777777778123, 0.6166666666666666963, 0.6180555555555555802, 0.6187500000000000222 ),
 .UNSPECIFIED. ) 
 CURVE ( )  GEOMETRIC_REPRESENTATION_ITEM ( )  RATIONAL_B_SPLINE_CURVE ( ( 0.9330127018922194093, 0.9330127018922194093, 1.000000000000000000, 0.8660254037844387076, 1.000000000000000000, 0.8660254037844387076, 1.000000000000000000, 0.9330127018922194093, 0.9330127018922194093 ) ) 
 REPRESENTATION_ITEM ( '' )  );
#34547=CARTESIAN_POINT ( 'NONE',  ( 3.405278471875001323, 17.50000000000001066, -23.40629330266049024 ) ) ;
#34549=CARTESIAN_POINT ( 'NONE',  ( 3.500000000000000000, 15.47927405783632970, -96.54431413575484555 ) ) ;
#34551=CARTESIAN_POINT ( 'NONE',  ( -3.310556943750002645, 15.58864905735836537, -26.76827246956613493 ) ) ;
#34552=FACE_OUTER_BOUND ( 'NONE', #36319, .T. ) ;
#34553=CARTESIAN_POINT ( 'NONE',  ( -3.310556943750000425, 19.41135094264167549, -129.8474391362328220 ) ) ;
#34556=LINE ( 'NONE', #8821, #23860 ) ;
#34557=CARTESIAN_POINT ( 'NONE',  ( 1.655278471875001101, 20.36702641396249547, -123.1849391362327992 ) ) ;
#34558=CARTESIAN_POINT ( 'NONE',  ( -1.750000000000002220, 14.46891108675447946, -55.48806413671075433 ) ) ;
#34559=CARTESIAN_POINT ( 'NONE',  ( 3.500000000000000000, 15.47927405783632082, -39.23806413671076854 ) ) ;
#34562=CARTESIAN_POINT ( 'NONE',  ( 3.310556943749999981, 15.58864905735837780, -137.4349391362327992 ) ) ;
#34564=CARTESIAN_POINT ( 'NONE',  ( -1.655278471875002211, 14.63297358603754184, -46.68493913623279923 ) ) ;
#34566=CARTESIAN_POINT ( 'NONE',  ( 3.500000000000001332, 17.50000000000002132, -104.4609808024215027 ) ) ;
#34567=CARTESIAN_POINT ( 'NONE',  ( 1.655278471874998436, 14.63297358603754361, -74.51827246956612782 ) ) ;
#34569=CARTESIAN_POINT ( 'NONE',  ( 3.310556943749999981, 15.58864905735837070, -102.3474391362328220 ) ) ;
#34570=CARTESIAN_POINT ( 'NONE',  ( -1.655278471875002211, 14.63297358603754539, -70.59743913623280775 ) ) ;
#34571=ORIENTED_EDGE ( 'NONE', *, *, #35354, .F. ) ;
#34572=CARTESIAN_POINT ( 'NONE',  ( 3.310556943750001313, 17.50000000000001776, -92.35160580289947063 ) ) ;
#34575=CARTESIAN_POINT ( 'NONE',  ( -1.394453263437886604E-15, 14.00000000000001421, -77.71098080242148853 ) ) ;
#34577=CARTESIAN_POINT ( 'NONE',  ( -3.310556943750002201, 15.58864905735836892, -56.68077246956614346 ) ) ;
#34579=CARTESIAN_POINT ( 'NONE',  ( -3.310556943750000425, 19.41135094264166838, -108.8474391362328220 ) ) ;
#34581=EDGE_LOOP ( 'NONE', ( #30613, #34534, #30237, #1053 ) ) ;
#34582=ORIENTED_EDGE ( 'NONE', *, *, #17883, .T. ) ;
#34587=CARTESIAN_POINT ( 'NONE',  ( 2.340729813953370519E-16, 21.32270188528330834, -63.01410580289947205 ) ) ;
#34588=VERTEX_POINT ( 'NONE', #31425 ) ;
#34590=FACE_OUTER_BOUND ( 'NONE', #11062, .T. ) ;
#34592=CARTESIAN_POINT ( 'NONE',  ( 0.000000000000000000, 21.00000000000002487, -149.5231586289125687 ) ) ;
#34597=CARTESIAN_POINT ( 'NONE',  ( 1.655278471874998436, 14.63297358603755072, -128.4307724695661364 ) ) ;
#34598=CARTESIAN_POINT ( 'NONE',  ( -3.500000000000000000, 19.52072594216371826, -103.0443141357548456 ) ) ;
#34600=CARTESIAN_POINT ( 'NONE',  ( 3.310556943750001313, 17.50000000000001066, -40.35160580289947063 ) ) ;
#34601=CARTESIAN_POINT ( 'NONE',  ( -1.655278471875002211, 14.63297358603754006, -32.68493913623279923 ) ) ;
#34602=CARTESIAN_POINT ( 'NONE',  ( 1.655278471874998436, 14.63297358603754539, -94.51827246956612782 ) ) ;
#34603=CARTESIAN_POINT ( 'NONE',  ( -3.500000000000000888, 19.52072594216370405, -26.73806413671075788 ) ) ;
#34607=CARTESIAN_POINT ( 'NONE',  ( 3.310556943750001313, 17.50000000000002487, -136.3516058028994564 ) ) ;
#34608=DIRECTION ( 'NONE',  ( 0.8660254037844367092, 0.000000000000000000, -0.5000000000000034417 ) ) ;
#34609=CARTESIAN_POINT ( 'NONE',  ( 3.500000000000000000, 15.47927405783633503, -136.2380641367107614 ) ) ;
#34610=CARTESIAN_POINT ( 'NONE',  ( 3.310556943750001313, 19.41135094264166128, -59.18077246956614346 ) ) ;
#34611=CARTESIAN_POINT ( 'NONE',  ( 3.500000000000000000, 15.47927405783633503, -132.2380641367107614 ) ) ;
#34612=CARTESIAN_POINT ( 'NONE',  ( -3.500000000000001332, 17.50000000000001776, -79.65473080337743284 ) ) ;
#34613=CARTESIAN_POINT ( 'NONE',  ( -3.310556943750001313, 17.50000000000001421, -63.85160580289946353 ) ) ;
#34616=DIRECTION ( 'NONE',  ( -0.000000000000000000, 1.259100132267607459E-16, -1.000000000000000000 ) ) ;
#34618=CARTESIAN_POINT ( 'NONE',  ( 3.310556943749999981, 15.58864905735837247, -118.3474391362328078 ) ) ;
#34621=ORIENTED_EDGE ( 'NONE', *, *, #31920, .F. ) ;
#34623=CARTESIAN_POINT ( 'NONE',  ( -7.424026671074350129E-16, 13.45854811567263987, -112.4047308033774328 ) ) ;
#34626=CARTESIAN_POINT ( 'NONE',  ( 0.9378221735089300459, 21.00000000000001421, -60.94938900211594301 ) ) ;
#34629=CARTESIAN_POINT ( 'NONE',  ( -3.310556943750002201, 15.58864905735837070, -72.68077246956613635 ) ) ;
#34632=CARTESIAN_POINT ( 'NONE',  ( -3.500000000000000000, 19.52072594216371115, -79.04431413575484555 ) ) ;
#34635=CARTESIAN_POINT ( 'NONE',  ( 3.310556943749999981, 15.58864905735836004, -23.34743913623281486 ) ) ;
#34637=CARTESIAN_POINT ( 'NONE',  ( 3.310556943750001313, 17.50000000000001776, -80.26410580289946495 ) ) ;
#34638=EDGE_LOOP ( 'NONE', ( #1589, #32020, #26340, #32368 ) ) ;
#34643=CARTESIAN_POINT ( 'NONE',  ( 0.9378221735089300459, 21.00000000000002132, -102.2556390011600058 ) ) ;
#34645=ORIENTED_EDGE ( 'NONE', *, *, #31643, .F. ) ;
#34646=FACE_OUTER_BOUND ( 'NONE', #3716, .T. ) ;
#34647=CARTESIAN_POINT ( 'NONE',  ( -7.022189441860112050E-16, 13.67729811471671653, -48.60160580289946353 ) ) ;
#34648=CARTESIAN_POINT ( 'NONE',  ( 3.310556943749999981, 15.58864905735837070, -108.4349391362327850 ) ) ;
#34650=CARTESIAN_POINT ( 'NONE',  ( -7.022189441860112050E-16, 13.67729811471671475, -35.51410580289947205 ) ) ;
#34651=CARTESIAN_POINT ( 'NONE',  ( 2.340729813953370519E-16, 21.32270188528330834, -61.10160580289946353 ) ) ;
#34652=CARTESIAN_POINT ( 'NONE',  ( 2.474675557024783212E-16, 21.54145188432740099, -110.2109808024215170 ) ) ;
#34654=CARTESIAN_POINT ( 'NONE',  ( -3.310556943750002645, 15.58864905735837247, -91.68077246956613635 ) ) ;
#34658=CARTESIAN_POINT ( 'NONE',  ( 2.474675557024783212E-16, 21.54145188432739388, -63.21098080242150274 ) ) ;
#34661=CARTESIAN_POINT ( 'NONE',  ( 2.340729813953370519E-16, 21.32270188528330479, -27.01410580289947916 ) ) ;
#34662=CARTESIAN_POINT ( 'NONE',  ( 1.750000000000001110, 20.53108891324555074, -55.98806413671076143 ) ) ;
#34663=CARTESIAN_POINT ( 'NONE',  ( -3.500000000000002220, 15.47927405783632437, -45.87764746908818125 ) ) ;
#34664=CARTESIAN_POINT ( 'NONE',  ( -7.022189441860112050E-16, 13.67729811471672541, -104.6016058028994564 ) ) ;
#34665=CARTESIAN_POINT ( 'NONE',  ( 3.310556943749999981, 15.58864905735836182, -39.43493913623280633 ) ) ;
#34674=CARTESIAN_POINT ( 'NONE',  ( 3.310556943750001313, 19.41135094264166838, -86.18077246956613635 ) ) ;
#34676=CARTESIAN_POINT ( 'NONE',  ( -0.9378221735089291577, 21.00000000000001066, -24.16632260368299256 ) ) ;
#34677=ORIENTED_EDGE ( 'NONE', *, *, #22858, .T. ) ;
#34678=CARTESIAN_POINT ( 'NONE',  ( -0.9378221735089291577, 21.00000000000001776, -102.1663226036829855 ) ) ;
#34679=AXIS2_PLACEMENT_3D ( 'NONE', #23083, #42039, #13306 ) ;
#34680=CARTESIAN_POINT ( 'NONE',  ( -1.750000000000002220, 14.46891108675447768, -50.48806413671076854 ) ) ;
#34681=ORIENTED_EDGE ( 'NONE', *, *, #29935, .F. ) ;
#34684=CARTESIAN_POINT ( 'NONE',  ( 2.340729813953370519E-16, 21.32270188528331190, -95.01410580289946495 ) ) ;
#34686=ORIENTED_EDGE ( 'NONE', *, *, #9130, .T. ) ;
#34687=CARTESIAN_POINT ( 'NONE',  ( -3.500000000000002220, 15.47927405783632793, -78.57139747004410424 ) ) ;
#34688=VERTEX_POINT ( 'NONE', #25263 ) ;
#34690=CARTESIAN_POINT ( 'NONE',  ( 7.367361408496833051E-14, 14.00000000000002132, -110.4047308033774328 ) ) ;
#34693=ORIENTED_EDGE ( 'NONE', *, *, #38716, .T. ) ;
#34694=ADVANCED_FACE ( 'NONE', ( #5903 ), #21853, .T. ) ;
#34696=CYLINDRICAL_SURFACE ( 'NONE', #2946, 3.499999999999999556 ) ;
#34698=EDGE_CURVE ( 'NONE', #37319, #21407, #23295, .T. ) ;
#34699=CARTESIAN_POINT ( 'NONE',  ( -1.655278471875002211, 14.63297358603755249, -134.5974391362328220 ) ) ;
#34702=CARTESIAN_POINT ( 'NONE',  ( 3.500000000000000000, 15.47927405783632437, -54.54431413575484555 ) ) ;
#34703=CARTESIAN_POINT ( 'NONE',  ( 1.655278471874998436, 14.63297358603754184, -55.51827246956612782 ) ) ;
#34706=CARTESIAN_POINT ( 'NONE',  ( 1.750000000000001110, 20.53108891324556140, -135.9880641367107614 ) ) ;
#34707=VECTOR ( 'NONE', #8817, 1000.000000000000000 ) ;
#34709=CARTESIAN_POINT ( 'NONE',  ( 2.340729813953370519E-16, 21.32270188528331190, -76.10160580289945642 ) ) ;
#34710=CARTESIAN_POINT ( 'NONE',  ( -3.500000000000001332, 17.50000000000002132, -126.9609808024215170 ) ) ;
#34711=CARTESIAN_POINT ( 'NONE',  ( 3.310556943750001313, 19.41135094264166838, -112.1807724695661506 ) ) ;
#34714=CARTESIAN_POINT ( 'NONE',  ( -3.500000000000002220, 15.47927405783632615, -80.87764746908817415 ) ) ;
#34716=CARTESIAN_POINT ( 'NONE',  ( 3.310556943749999981, 15.58864905735836182, -41.34743913623280065 ) ) ;
#34717=CARTESIAN_POINT ( 'NONE',  ( 3.310556943750001313, 17.50000000000002132, -102.3516058028994564 ) ) ;
#34719=CARTESIAN_POINT ( 'NONE',  ( -0.9378221735089221633, 14.00000000000001599, -129.7556390011600058 ) ) ;
#34720=VERTEX_POINT ( 'NONE', #11857 ) ;
#34721=CARTESIAN_POINT ( 'NONE',  ( 3.310556943749999981, 15.58864905735837425, -124.4349391362327992 ) ) ;
#34722=CARTESIAN_POINT ( 'NONE',  ( -0.9378221735089221633, 14.00000000000001599, -129.4493890021159075 ) ) ;
#34727=EDGE_CURVE ( 'NONE', #3726, #17813, #8459, .T. ) ;
#34728=EDGE_LOOP ( 'NONE', ( #4986, #18445, #26854, #1890 ) ) ;
#34730=ORIENTED_EDGE ( 'NONE', *, *, #23347, .T. ) ;
#34731=CARTESIAN_POINT ( 'NONE',  ( -3.310556943750002201, 15.58864905735837070, -77.76827246956614204 ) ) ;
#34732=EDGE_CURVE ( 'NONE', #32852, #21810, #9092, .T. ) ;
#34733=CARTESIAN_POINT ( 'NONE',  ( 1.750000000000001110, 20.53108891324554719, -40.29431413575485266 ) ) ;
#34735=CARTESIAN_POINT ( 'NONE',  ( 0.9378221735089281585, 14.00000000000002132, -99.36007260463888713 ) ) ;
#34738=CARTESIAN_POINT ( 'NONE',  ( 3.310556943750001313, 19.41135094264166128, -33.18077246956615056 ) ) ;
#34739=CARTESIAN_POINT ( 'NONE',  ( 3.500000000000001332, 19.52072594216371826, -107.0713974700441042 ) ) ;
#34742=ORIENTED_EDGE ( 'NONE', *, *, #30885, .F. ) ;
#34744=CARTESIAN_POINT ( 'NONE',  ( 2.340729813953370519E-16, 21.32270188528330834, -48.01410580289946495 ) ) ;
#34747=CARTESIAN_POINT ( 'NONE',  ( -1.394453263437886604E-15, 14.00000000000001421, -56.40473080337742573 ) ) ;
#34750=CARTESIAN_POINT ( 'NONE',  ( 3.500000000000000000, 15.47927405783632437, -63.23806413671076143 ) ) ;
#34751=DIRECTION ( 'NONE',  ( -0.000000000000000000, 1.259100132267607459E-16, -1.000000000000000000 ) ) ;
#34752=CARTESIAN_POINT ( 'NONE',  ( -7.424026671074350129E-16, 13.45854811567263098, -39.71098080242151696 ) ) ;
#34753=CARTESIAN_POINT ( 'NONE',  ( -1.394453263437886604E-15, 14.00000000000002132, -114.4047308033774186 ) ) ;
#34754=CARTESIAN_POINT ( 'NONE',  ( -3.500000000000002220, 15.47927405783632615, -64.57139747004410424 ) ) ;
#34755=EDGE_CURVE ( 'NONE', #3982, #15014, #24923, .T. ) ;
#34758=CARTESIAN_POINT ( 'NONE',  ( -3.310556943750000425, 19.41135094264165772, -23.93493913623280278 ) ) ;
#34760=DIRECTION ( 'NONE',  ( -0.000000000000000000, 1.259100132267607459E-16, -1.000000000000000000 ) ) ;
#34761=CARTESIAN_POINT ( 'NONE',  ( 3.310556943750001313, 19.41135094264166838, -128.1807724695661364 ) ) ;
#34764=CARTESIAN_POINT ( 'NONE',  ( -1.749999999999999778, 20.53108891324555429, -76.82139747004410424 ) ) ;
#34765=CARTESIAN_POINT ( 'NONE',  ( -3.310556943750000425, 19.41135094264166838, -114.9349391362327992 ) ) ;
#34767=CARTESIAN_POINT ( 'NONE',  ( 1.750000000000001110, 20.53108891324554719, -36.98806413671076854 ) ) ;
#34768=CARTESIAN_POINT ( 'NONE',  ( 0.9378221735089281585, 14.00000000000001776, -92.36007260463891555 ) ) ;
#34769=FACE_OUTER_BOUND ( 'NONE', #12337, .T. ) ;
#34770=CARTESIAN_POINT ( 'NONE',  ( -3.310556943750002201, 15.58864905735837958, -141.7682724695661420 ) ) ;
#34773=CARTESIAN_POINT ( 'NONE',  ( -1.655278471875002211, 14.63297358603754184, -50.68493913623279923 ) ) ;
#34776=CARTESIAN_POINT ( 'NONE',  ( 3.310556943750001313, 19.41135094264166128, -72.26827246956612782 ) ) ;
#34778=CARTESIAN_POINT ( 'NONE',  ( 1.655278471874998436, 14.63297358603754716, -97.43077246956613635 ) ) ;
#34779=CARTESIAN_POINT ( 'NONE',  ( 1.655278471874998436, 14.63297358603754361, -70.43077246956613635 ) ) ;
#34780=ORIENTED_EDGE ( 'NONE', *, *, #31836, .T. ) ;
#34781=CARTESIAN_POINT ( 'NONE',  ( 3.310556943750001313, 17.50000000000001776, -90.35160580289947063 ) ) ;
#34786=VECTOR ( 'NONE', #9053, 1000.000000000000000 ) ;
#34788=CARTESIAN_POINT ( 'NONE',  ( -1.655278471875002211, 14.63297358603754184, -53.59743913623281486 ) ) ;
#34790=DIRECTION ( 'NONE',  ( -0.000000000000000000, 1.259100132267607459E-16, -1.000000000000000000 ) ) ;
#34791=CARTESIAN_POINT ( 'NONE',  ( 1.655278471875001101, 20.36702641396249547, -109.0974391362328078 ) ) ;
#34792=DIRECTION ( 'NONE',  ( 0.000000000000000000, 1.000000000000000000, 0.000000000000000000 ) ) ;
#34793=ORIENTED_EDGE ( 'NONE', *, *, #28515, .T. ) ;
#34794=ORIENTED_EDGE ( 'NONE', *, *, #22908, .T. ) ;
#34796=ORIENTED_EDGE ( 'NONE', *, *, #41610, .T. ) ;
#34798=CARTESIAN_POINT ( 'NONE',  ( 2.340729813953370519E-16, 21.32270188528330834, -62.01410580289947205 ) ) ;
#34799=( BOUNDED_CURVE ( )  B_SPLINE_CURVE ( 2, ( #27223, #40186, #33381, #39977, #10841, #7233, #849, #36793, #27429 ),
 .UNSPECIFIED., .F., .F. ) 
 B_SPLINE_CURVE_WITH_KNOTS ( ( 3, 2, 2, 2, 3 ),
 ( 0.4395833333333333259, 0.4402777777777777679, 0.4416666666666666519, 0.4430555555555555358, 0.4437499999999999778 ),
 .UNSPECIFIED. ) 
 CURVE ( )  GEOMETRIC_REPRESENTATION_ITEM ( )  RATIONAL_B_SPLINE_CURVE ( ( 0.9330127018922194093, 0.9330127018922194093, 1.000000000000000000, 0.8660254037844387076, 1.000000000000000000, 0.8660254037844387076, 1.000000000000000000, 0.9330127018922194093, 0.9330127018922194093 ) ) 
 REPRESENTATION_ITEM ( '' )  );
#34800=ORIENTED_EDGE ( 'NONE', *, *, #34065, .F. ) ;
#34803=CARTESIAN_POINT ( 'NONE',  ( -3.500000000000001332, 17.50000000000002487, -142.6547308033774186 ) ) ;
#34808=CARTESIAN_POINT ( 'NONE',  ( 3.310556943750001313, 17.50000000000002487, -130.2641058028994507 ) ) ;
#34810=CARTESIAN_POINT ( 'NONE',  ( -3.310556943750001313, 17.50000000000001066, -41.85160580289947063 ) ) ;
#34811=EDGE_CURVE ( 'NONE', #5754, #31901, #11865, .T. ) ;
#34812=CARTESIAN_POINT ( 'NONE',  ( -1.655278471875002211, 14.63297358603753828, -25.68493913623279212 ) ) ;
#34814=CARTESIAN_POINT ( 'NONE',  ( -7.022189441860112050E-16, 13.67729811471672363, -93.60160580289948484 ) ) ;
#34815=CARTESIAN_POINT ( 'NONE',  ( 3.500000000000001776, 19.52072594216370405, -26.07139747004409358 ) ) ;
#34819=CARTESIAN_POINT ( 'NONE',  ( -3.310556943750002645, 15.58864905735837958, -137.7682724695661420 ) ) ;
#34821=CARTESIAN_POINT ( 'NONE',  ( -3.500000000000002220, 15.47927405783633503, -122.8776474690881741 ) ) ;
#34822=CARTESIAN_POINT ( 'NONE',  ( 3.500000000000001332, 17.50000000000001776, -95.15473080337743284 ) ) ;
#34823=CARTESIAN_POINT ( 'NONE',  ( -3.500000000000000888, 19.52072594216371115, -78.73806413671076143 ) ) ;
#34824=ADVANCED_FACE ( 'NONE', ( #22907 ), #13534, .T. ) ;
#34825=CARTESIAN_POINT ( 'NONE',  ( 2.340729813953370519E-16, 21.32270188528331190, -66.10160580289945642 ) ) ;
#34829=CARTESIAN_POINT ( 'NONE',  ( -0.9378221735089291577, 21.00000000000001421, -48.16632260368299256 ) ) ;
#34831=CARTESIAN_POINT ( 'NONE',  ( 1.655278471875001101, 20.36702641396249547, -112.0974391362328078 ) ) ;
#34834=VERTEX_POINT ( 'NONE', #12711 ) ;
#34835=CARTESIAN_POINT ( 'NONE',  ( -1.749999999999999778, 20.53108891324555785, -107.8213974700441042 ) ) ;
#34837=CARTESIAN_POINT ( 'NONE',  ( -1.749999999999999778, 20.53108891324554719, -27.12764746908817415 ) ) ;
#34840=CARTESIAN_POINT ( 'NONE',  ( 1.655278471875001101, 20.36702641396248836, -71.09743913623280775 ) ) ;
#34842=DIRECTION ( 'NONE',  ( -0.000000000000000000, 1.259100132267607459E-16, -1.000000000000000000 ) ) ;
#34843=CARTESIAN_POINT ( 'NONE',  ( 0.9378221735089281585, 14.00000000000001599, -72.66632260368299967 ) ) ;
#34848=CARTESIAN_POINT ( 'NONE',  ( -7.022189441860112050E-16, 13.67729811471672186, -80.51410580289947916 ) ) ;
#34851=ORIENTED_EDGE ( 'NONE', *, *, #39042, .F. ) ;
#34855=CARTESIAN_POINT ( 'NONE',  ( 1.750000000000001110, 20.53108891324555785, -128.9880641367107614 ) ) ;
#34856=FACE_OUTER_BOUND ( 'NONE', #16288, .T. ) ;
#34857=CARTESIAN_POINT ( 'NONE',  ( -7.022189441860112050E-16, 13.67729811471671653, -46.60160580289946353 ) ) ;
#34858=CARTESIAN_POINT ( 'NONE',  ( -1.655278471875002211, 14.63297358603754894, -108.6849391362327992 ) ) ;
#34860=CARTESIAN_POINT ( 'NONE',  ( 3.310556943750001313, 17.50000000000001066, -36.26410580289947205 ) ) ;
#34861=CARTESIAN_POINT ( 'NONE',  ( -3.310556943750001313, 17.50000000000001421, -61.85160580289945642 ) ) ;
#34862=CARTESIAN_POINT ( 'NONE',  ( 1.749999999999998224, 14.46891108675448301, -108.6276474690881741 ) ) ;
#34864=CARTESIAN_POINT ( 'NONE',  ( -7.022189441860112050E-16, 13.67729811471672363, -91.51410580289947916 ) ) ;
#34866=CARTESIAN_POINT ( 'NONE',  ( -1.749999999999999778, 20.53108891324555429, -96.82139747004409003 ) ) ;
#34869=CARTESIAN_POINT ( 'NONE',  ( -1.394453263437886604E-15, 14.00000000000001066, -51.71098080242150985 ) ) ;
#34872=CARTESIAN_POINT ( 'NONE',  ( -1.749999999999999778, 20.53108891324555074, -59.12764746908817415 ) ) ;
#34873=CARTESIAN_POINT ( 'NONE',  ( -1.394453263437886604E-15, 14.00000000000001421, -71.71098080242150274 ) ) ;
#34874=CARTESIAN_POINT ( 'NONE',  ( -3.310556943750001313, 17.50000000000001066, -27.76410580289947916 ) ) ;
#34875=CARTESIAN_POINT ( 'NONE',  ( 1.749999999999998224, 14.46891108675447590, -50.32139747004409003 ) ) ;
#34878=CARTESIAN_POINT ( 'NONE',  ( 3.310556943750001313, 17.50000000000002132, -109.3516058028994564 ) ) ;
#34879=CARTESIAN_POINT ( 'NONE',  ( 3.310556943750001313, 19.41135094264166128, -30.26827246956613493 ) ) ;
#34885=CARTESIAN_POINT ( 'NONE',  ( 3.310556943750001313, 19.41135094264166838, -87.18077246956612214 ) ) ;
#34886=CYLINDRICAL_SURFACE ( 'NONE', #29660, 3.499999999999999556 ) ;
#34889=CARTESIAN_POINT ( 'NONE',  ( -1.394453263437886604E-15, 14.00000000000002132, -133.4047308033774186 ) ) ;
#34890=ORIENTED_EDGE ( 'NONE', *, *, #32293, .F. ) ;
#34893=CARTESIAN_POINT ( 'NONE',  ( 3.310556943749999981, 15.58864905735837070, -97.34743913623280775 ) ) ;
#34904=ORIENTED_EDGE ( 'NONE', *, *, #21794, .F. ) ;
#34905=CARTESIAN_POINT ( 'NONE',  ( 3.602337597214540226E-14, 14.00000000000002132, -116.4047308033774328 ) ) ;
#34907=CARTESIAN_POINT ( 'NONE',  ( 3.310556943750001313, 19.41135094264167549, -137.1807724695661364 ) ) ;
#34908=AXIS2_PLACEMENT_3D ( 'NONE', #13767, #26117, #6747 ) ;
#34909=CARTESIAN_POINT ( 'NONE',  ( 3.500000000000001332, 17.50000000000002487, -133.4609808024214885 ) ) ;
#34911=CARTESIAN_POINT ( 'NONE',  ( 4.648177544792955347E-16, 21.00000000000001421, -72.90473080337743284 ) ) ;
#34912=CARTESIAN_POINT ( 'NONE',  ( -1.655278471875002211, 14.63297358603755072, -122.6849391362327992 ) ) ;
#34913=CARTESIAN_POINT ( 'NONE',  ( 3.310556943750001313, 19.41135094264166128, -52.26827246956612782 ) ) ;
#34916=CARTESIAN_POINT ( 'NONE',  ( -1.750000000000002220, 14.46891108675448834, -133.4880641367107614 ) ) ;
#34918=CARTESIAN_POINT ( 'NONE',  ( -3.310556943750001313, 17.50000000000001776, -78.85160580289945642 ) ) ;
#34919=CARTESIAN_POINT ( 'NONE',  ( -3.500000000000002220, 15.47927405783633503, -120.8776474690881741 ) ) ;
#34920=CARTESIAN_POINT ( 'NONE',  ( -3.310556943750001313, 17.50000000000002132, -107.7641058028994649 ) ) ;
#34924=CARTESIAN_POINT ( 'NONE',  ( 3.500000000000001332, 17.50000000000001776, -81.46098080242150274 ) ) ;
#34926=CARTESIAN_POINT ( 'NONE',  ( 3.310556943750001313, 17.50000000000001066, -42.26410580289947916 ) ) ;
#34927=CARTESIAN_POINT ( 'NONE',  ( -3.310556943750000425, 19.41135094264166838, -103.9349391362328134 ) ) ;
#34931=CARTESIAN_POINT ( 'NONE',  ( -7.022189441860112050E-16, 13.67729811471672896, -124.6016058028994564 ) ) ;
#34932=CARTESIAN_POINT ( 'NONE',  ( -3.500000000000002220, 15.47927405783633503, -136.5713974700441042 ) ) ;
#34937=CARTESIAN_POINT ( 'NONE',  ( -1.750000000000002220, 14.46891108675447946, -62.79431413575483845 ) ) ;
#34938=EDGE_CURVE ( 'NONE', #37319, #17107, #36292, .T. ) ;
#34940=ORIENTED_EDGE ( 'NONE', *, *, #969, .F. ) ;
#34941=CARTESIAN_POINT ( 'NONE',  ( -1.655278471875002211, 14.63297358603754539, -74.68493913623279923 ) ) ;
#34942=ADVANCED_FACE ( 'NONE', ( #16535 ), #19923, .T. ) ;
#34943=CARTESIAN_POINT ( 'NONE',  ( 3.500000000000001332, 17.50000000000001066, -40.46098080242150985 ) ) ;
#34944=CARTESIAN_POINT ( 'NONE',  ( -0.9378221735089640188, 21.00000000000000000, -102.8600726046388871 ) ) ;
#34948=CARTESIAN_POINT ( 'NONE',  ( -3.310556943750002201, 15.58864905735836537, -36.68077246956613635 ) ) ;
#34953=CARTESIAN_POINT ( 'NONE',  ( -3.310556943750000425, 19.41135094264166128, -46.84743913623280065 ) ) ;
#34954=ORIENTED_EDGE ( 'NONE', *, *, #7209, .F. ) ;
#34956=CARTESIAN_POINT ( 'NONE',  ( 3.500000000000001332, 19.52072594216370760, -56.07139747004410424 ) ) ;
#34957=LINE ( 'NONE', #2213, #1735 ) ;
#34959=VECTOR ( 'NONE', #39524, 1000.000000000000000 ) ;
#34960=CARTESIAN_POINT ( 'NONE',  ( 3.500000000000000000, 15.47927405783632970, -97.54431413575484555 ) ) ;
#34963=CARTESIAN_POINT ( 'NONE',  ( -7.424026671074350129E-16, 13.45854811567263098, -34.71098080242150985 ) ) ;
#34964=EDGE_CURVE ( 'NONE', #10325, #10255, #18948, .T. ) ;
#34966=CARTESIAN_POINT ( 'NONE',  ( -1.394453263437886604E-15, 14.00000000000001421, -70.71098080242150274 ) ) ;
#34970=( BOUNDED_CURVE ( )  B_SPLINE_CURVE ( 2, ( #771, #26724, #39686, #10558, #23538, #14589, #17981, #31157, #40943 ),
 .UNSPECIFIED., .F., .T. ) 
 B_SPLINE_CURVE_WITH_KNOTS ( ( 3, 2, 2, 2, 3 ),
 ( 0.01458333333333333356, 0.01527777777777777728, 0.01666666666666666644, 0.01805555555555555386, 0.01874999999999999931 ),
 .UNSPECIFIED. ) 
 CURVE ( )  GEOMETRIC_REPRESENTATION_ITEM ( )  RATIONAL_B_SPLINE_CURVE ( ( 0.9330127018922192983, 0.9330127018922194093, 1.000000000000000000, 0.8660254037844387076, 1.000000000000000000, 0.8660254037844387076, 1.000000000000000000, 0.9330127018922194093, 0.9330127018922194093 ) ) 
 REPRESENTATION_ITEM ( '' )  );
#34971=AXIS2_PLACEMENT_3D ( 'NONE', #12908, #39251, #22687 ) ;
#34974=CARTESIAN_POINT ( 'NONE',  ( -3.500000000000001332, 17.50000000000002487, -141.9609808024215170 ) ) ;
#34976=CARTESIAN_POINT ( 'NONE',  ( -3.310556943750001313, 17.50000000000002132, -123.7641058028994649 ) ) ;
#34980=CARTESIAN_POINT ( 'NONE',  ( 4.648177544792955347E-16, 21.00000000000001776, -76.90473080337740441 ) ) ;
#34981=CARTESIAN_POINT ( 'NONE',  ( 3.310556943749999981, 15.58864905735837247, -116.4349391362327850 ) ) ;
#34982=DIRECTION ( 'NONE',  ( -0.000000000000000000, 1.259100132267607459E-16, -1.000000000000000000 ) ) ;
#34983=CARTESIAN_POINT ( 'NONE',  ( -1.750000000000002220, 14.46891108675447768, -40.48806413671076143 ) ) ;
#34986=CARTESIAN_POINT ( 'NONE',  ( 1.655278471875001101, 20.36702641396249902, -138.1849391362327992 ) ) ;
#34989=CARTESIAN_POINT ( 'NONE',  ( 2.340729813953370519E-16, 21.32270188528330834, -46.10160580289945642 ) ) ;
#34991=CARTESIAN_POINT ( 'NONE',  ( 4.648177544792955347E-16, 21.00000000000002132, -109.9047308033774186 ) ) ;
#34992=CARTESIAN_POINT ( 'NONE',  ( 1.655278471875001101, 20.36702641396248836, -70.18493913623279923 ) ) ;
#34994=CARTESIAN_POINT ( 'NONE',  ( 3.310556943749999981, 15.58864905735836714, -71.34743913623279354 ) ) ;
#34995=ORIENTED_EDGE ( 'NONE', *, *, #2010, .T. ) ;
#34996=CARTESIAN_POINT ( 'NONE',  ( -3.310556943750001313, 17.50000000000001776, -91.85160580289947063 ) ) ;
#34997=AXIS2_PLACEMENT_3D ( 'NONE', #28160, #37328, #27953 ) ;
#34999=CARTESIAN_POINT ( 'NONE',  ( -3.500000000000002220, 15.47927405783633326, -107.8776474690881741 ) ) ;
#35000=DIRECTION ( 'NONE',  ( -0.000000000000000000, 1.259100132267607459E-16, -1.000000000000000000 ) ) ;
#35001=CARTESIAN_POINT ( 'NONE',  ( 3.500000000000001332, 19.52072594216371826, -131.3776474690881741 ) ) ;
#35002=CARTESIAN_POINT ( 'NONE',  ( -3.310556943750000425, 19.41135094264166483, -51.84743913623281486 ) ) ;
#35003=CARTESIAN_POINT ( 'NONE',  ( -1.655278471875002211, 14.63297358603754894, -108.5974391362328078 ) ) ;
#35006=ORIENTED_EDGE ( 'NONE', *, *, #17066, .T. ) ;
#35008=ADVANCED_FACE ( 'NONE', ( #20137 ), #21667, .T. ) ;
#35012=CARTESIAN_POINT ( 'NONE',  ( -1.655278471875002211, 14.63297358603754361, -62.59743913623280775 ) ) ;
#35013=EDGE_LOOP ( 'NONE', ( #2281, #2788, #11446, #23455 ) ) ;
#35014=ORIENTED_EDGE ( 'NONE', *, *, #17648, .F. ) ;
#35015=CARTESIAN_POINT ( 'NONE',  ( 0.000000000000000000, 17.50000000000002487, -149.5231586289125687 ) ) ;
#35021=CARTESIAN_POINT ( 'NONE',  ( 1.655278471874998436, 14.63297358603755072, -123.4307724695661506 ) ) ;
#35023=EDGE_CURVE ( 'NONE', #30046, #38620, #34957, .T. ) ;
#35024=CARTESIAN_POINT ( 'NONE',  ( -1.655278471875002211, 14.63297358603754006, -39.68493913623280633 ) ) ;
#35025=CARTESIAN_POINT ( 'NONE',  ( -7.022189441860112050E-16, 13.67729811471671475, -29.60160580289947418 ) ) ;
#35026=CARTESIAN_POINT ( 'NONE',  ( 3.310556943749999981, 15.58864905735836892, -92.43493913623279923 ) ) ;
#35027=CARTESIAN_POINT ( 'NONE',  ( -7.424026671074350129E-16, 13.45854811567263098, -25.40473080337743639 ) ) ;
#35030=CARTESIAN_POINT ( 'NONE',  ( 3.310556943750001313, 17.50000000000002487, -132.3516058028994564 ) ) ;
#35033=FACE_OUTER_BOUND ( 'NONE', #40364, .T. ) ;
#35034=CARTESIAN_POINT ( 'NONE',  ( 4.286263797015737581E-16, 14.00000000000002487, -149.5231586289125687 ) ) ;
#35035=DIRECTION ( 'NONE',  ( -0.000000000000000000, 1.259100132267607459E-16, -1.000000000000000000 ) ) ;
#35036=CARTESIAN_POINT ( 'NONE',  ( 1.750000000000001110, 20.53108891324555429, -79.98806413671076143 ) ) ;
#35037=CARTESIAN_POINT ( 'NONE',  ( 1.655278471875001101, 20.36702641396248836, -67.18493913623279923 ) ) ;
#35040=CARTESIAN_POINT ( 'NONE',  ( -1.749999999999999778, 20.53108891324555074, -58.82139747004409713 ) ) ;
#35041=CARTESIAN_POINT ( 'NONE',  ( -7.022189441860112050E-16, 13.67729811471672363, -83.60160580289947063 ) ) ;
#35042=DIRECTION ( 'NONE',  ( -0.000000000000000000, 1.259100132267607459E-16, -1.000000000000000000 ) ) ;
#35043=CARTESIAN_POINT ( 'NONE',  ( 3.310556943749999981, 15.58864905735837247, -114.3474391362328078 ) ) ;
#35045=CARTESIAN_POINT ( 'NONE',  ( 4.648177544792955347E-16, 21.00000000000001421, -61.90473080337742573 ) ) ;
#35046=VERTEX_POINT ( 'NONE', #24560 ) ;
#35047=CARTESIAN_POINT ( 'NONE',  ( 3.500000000000001776, 19.52072594216371826, -109.0713974700441184 ) ) ;
#35049=( NAMED_UNIT ( * ) SI_UNIT ( $, .STERADIAN. ) SOLID_ANGLE_UNIT ( ) );
#35050=CARTESIAN_POINT ( 'NONE',  ( -1.394453263437886604E-15, 14.00000000000002132, -121.7109808024215170 ) ) ;
#35051=CARTESIAN_POINT ( 'NONE',  ( -3.500000000000002220, 15.47927405783632082, -32.57139747004410424 ) ) ;
#35053=CARTESIAN_POINT ( 'NONE',  ( -1.655278471874999990, 20.36702641396248836, -66.93077246956613635 ) ) ;
#35054=( BOUNDED_CURVE ( )  B_SPLINE_CURVE ( 2, ( #16229, #16641, #26009, #29172, #49, #25800, #22809, #35780, #21851 ),
 .UNSPECIFIED., .F., .T. ) 
 B_SPLINE_CURVE_WITH_KNOTS ( ( 3, 2, 2, 2, 3 ),
 ( 0.1354166666666666574, 0.1361111111111110994, 0.1375000000000000111, 0.1388888888888888951, 0.1395833333333333370 ),
 .UNSPECIFIED. ) 
 CURVE ( )  GEOMETRIC_REPRESENTATION_ITEM ( )  RATIONAL_B_SPLINE_CURVE ( ( 0.9330127018922194093, 0.9330127018922194093, 1.000000000000000000, 0.8660254037844387076, 1.000000000000000000, 0.8660254037844387076, 1.000000000000000000, 0.9330127018922194093, 0.9330127018922194093 ) ) 
 REPRESENTATION_ITEM ( '' )  );
#35055=CARTESIAN_POINT ( 'NONE',  ( -1.394453263437886604E-15, 14.00000000000001421, -59.71098080242150274 ) ) ;
#35056=CARTESIAN_POINT ( 'NONE',  ( 4.286263797015737581E-16, 14.00000000000002487, -149.5231586289125687 ) ) ;
#35057=ADVANCED_FACE ( 'NONE', ( #40923 ), #34336, .T. ) ;
#35060=ADVANCED_FACE ( 'NONE', ( #5618 ), #8595, .T. ) ;
#35061=CARTESIAN_POINT ( 'NONE',  ( 4.648177544792955347E-16, 21.00000000000001066, -28.90473080337742928 ) ) ;
#35063=CARTESIAN_POINT ( 'NONE',  ( -3.310556943750001313, 17.50000000000001776, -78.76410580289946495 ) ) ;
#35067=CARTESIAN_POINT ( 'NONE',  ( -3.500000000000001332, 17.50000000000002132, -127.9609808024215170 ) ) ;
#35072=CARTESIAN_POINT ( 'NONE',  ( 3.310556943749999981, 15.58864905735836182, -42.43493913623279212 ) ) ;
#35073=CARTESIAN_POINT ( 'NONE',  ( -1.655278471874999990, 20.36702641396249547, -108.0182724695661278 ) ) ;
#35074=ORIENTED_EDGE ( 'NONE', *, *, #39475, .F. ) ;
#35075=CARTESIAN_POINT ( 'NONE',  ( 3.310556943749999981, 15.58864905735836182, -31.34743913623280775 ) ) ;
#35076=CARTESIAN_POINT ( 'NONE',  ( 3.310556943750001313, 19.41135094264166128, -63.26827246956613493 ) ) ;
#35077=CARTESIAN_POINT ( 'NONE',  ( -3.500000000000001332, 17.50000000000002132, -104.9609808024215027 ) ) ;
#35079=CARTESIAN_POINT ( 'NONE',  ( 3.500000000000001776, 19.52072594216371115, -96.07139747004409003 ) ) ;
#35083=CARTESIAN_POINT ( 'NONE',  ( 3.500000000000001776, 19.52072594216370760, -57.37764746908817415 ) ) ;
#35084=CARTESIAN_POINT ( 'NONE',  ( -1.655278471875002211, 14.63297358603754006, -26.59743913623280420 ) ) ;
#35085=CARTESIAN_POINT ( 'NONE',  ( 3.500000000000001332, 17.50000000000001421, -49.15473080337742573 ) ) ;
#35086=CARTESIAN_POINT ( 'NONE',  ( 3.500000000000001332, 19.52072594216371115, -77.37764746908817415 ) ) ;
#35087=CARTESIAN_POINT ( 'NONE',  ( -3.310556943750002201, 15.58864905735837425, -103.7682724695661278 ) ) ;
#35089=CARTESIAN_POINT ( 'NONE',  ( 3.310556943749999981, 15.58864905735836182, -32.43493913623279923 ) ) ;
#35096=CARTESIAN_POINT ( 'NONE',  ( 1.655278471874998436, 14.63297358603754539, -87.43077246956613635 ) ) ;
#35100=( BOUNDED_CURVE ( )  B_SPLINE_CURVE ( 2, ( #7776, #16714, #540, #26499, #40518 ),
 .UNSPECIFIED., .F., .T. ) 
 B_SPLINE_CURVE_WITH_KNOTS ( ( 3, 2, 3 ),
 ( 0.9979166666666666741, 0.9986111111111111160, 1.000000000000000000 ),
 .UNSPECIFIED. ) 
 CURVE ( )  GEOMETRIC_REPRESENTATION_ITEM ( )  RATIONAL_B_SPLINE_CURVE ( ( 0.9330127018922194093, 0.9330127018922194093, 1.000000000000000000, 0.8660254037844387076, 1.000000000000000000 ) ) 
 REPRESENTATION_ITEM ( '' )  );
#35101=CARTESIAN_POINT ( 'NONE',  ( 4.648177544792955347E-16, 21.00000000000002132, -107.9047308033774328 ) ) ;
#35105=CARTESIAN_POINT ( 'NONE',  ( 3.310556943749999981, 15.58864905735836892, -93.34743913623279354 ) ) ;
#35108=DIRECTION ( 'NONE',  ( -0.000000000000000000, 1.259100132267607459E-16, -1.000000000000000000 ) ) ;
#35109=EDGE_LOOP ( 'NONE', ( #29332, #5397, #27722, #41924 ) ) ;
#35116=LINE ( 'NONE', #5980, #18545 ) ;
#35118=CARTESIAN_POINT ( 'NONE',  ( -1.655278471874999990, 20.36702641396249547, -128.9307724695661364 ) ) ;
#35119=CYLINDRICAL_SURFACE ( 'NONE', #27794, 3.499999999999999556 ) ;
#35120=ORIENTED_EDGE ( 'NONE', *, *, #28473, .T. ) ;
#35121=CARTESIAN_POINT ( 'NONE',  ( 3.500000000000000000, 15.47927405783632082, -28.54431413575483845 ) ) ;
#35122=CARTESIAN_POINT ( 'NONE',  ( 3.310556943750001313, 19.41135094264166838, -126.2682724695661278 ) ) ;
#35123=CARTESIAN_POINT ( 'NONE',  ( -3.310556943750001313, 17.50000000000001421, -48.85160580289946353 ) ) ;
#35124=ORIENTED_EDGE ( 'NONE', *, *, #8465, .T. ) ;
#35125=CARTESIAN_POINT ( 'NONE',  ( 3.500000000000000000, 15.47927405783633503, -129.2380641367107614 ) ) ;
#35128=CARTESIAN_POINT ( 'NONE',  ( -3.310556943750001313, 17.50000000000001776, -76.85160580289945642 ) ) ;
#35129=CARTESIAN_POINT ( 'NONE',  ( 3.500000000000001332, 17.50000000000002132, -122.4609808024215170 ) ) ;
#35130=CARTESIAN_POINT ( 'NONE',  ( 1.655278471874998436, 14.63297358603754716, -106.4307724695661364 ) ) ;
#35131=CARTESIAN_POINT ( 'NONE',  ( -1.394453263437886604E-15, 14.00000000000001776, -81.40473080337743284 ) ) ;
#35134=CARTESIAN_POINT ( 'NONE',  ( 2.474675557024783212E-16, 21.54145188432739388, -73.21098080242151696 ) ) ;
#35135=CARTESIAN_POINT ( 'NONE',  ( 0.9378221735089281585, 14.00000000000002309, -126.3600726046389155 ) ) ;
#35136=CARTESIAN_POINT ( 'NONE',  ( -3.310556943750000425, 19.41135094264165772, -41.84743913623280775 ) ) ;
#35137=CARTESIAN_POINT ( 'NONE',  ( 3.310556943750001313, 19.41135094264166483, -100.2682724695661278 ) ) ;
#35138=CARTESIAN_POINT ( 'NONE',  ( 3.500000000000001332, 17.50000000000001421, -68.15473080337743284 ) ) ;
#35139=CARTESIAN_POINT ( 'NONE',  ( -7.424026671074350129E-16, 13.45854811567263454, -65.40473080337741862 ) ) ;
#35142=CARTESIAN_POINT ( 'NONE',  ( -1.655278471875002211, 14.63297358603755249, -125.6849391362327992 ) ) ;
#35146=CARTESIAN_POINT ( 'NONE',  ( 0.9378221735089281585, 14.00000000000001066, -50.66632260368297835 ) ) ;
#35148=CARTESIAN_POINT ( 'NONE',  ( -3.500000000000002220, 15.47927405783632615, -62.87764746908818125 ) ) ;
#35150=ORIENTED_EDGE ( 'NONE', *, *, #33490, .T. ) ;
#35151=CARTESIAN_POINT ( 'NONE',  ( 1.655278471874998436, 14.63297358603754361, -75.51827246956612782 ) ) ;
#35152=CARTESIAN_POINT ( 'NONE',  ( 0.9378221735089300459, 21.00000000000001066, -40.25563900116002714 ) ) ;
#35154=CARTESIAN_POINT ( 'NONE',  ( -3.500000000000000000, 19.52072594216370760, -56.04431413575484555 ) ) ;
#35157=CARTESIAN_POINT ( 'NONE',  ( -3.310556943750001313, 17.50000000000001066, -31.76410580289946850 ) ) ;
#35158=CARTESIAN_POINT ( 'NONE',  ( -1.394453263437886604E-15, 14.00000000000001776, -107.4047308033774328 ) ) ;
#35165=CARTESIAN_POINT ( 'NONE',  ( -1.394453263437886604E-15, 14.00000000000001776, -90.71098080242150274 ) ) ;
#35167=CARTESIAN_POINT ( 'NONE',  ( -1.750000000000002220, 14.46891108675448478, -104.4880641367107614 ) ) ;
#35168=CARTESIAN_POINT ( 'NONE',  ( 3.500000000000001776, 19.52072594216371826, -120.0713974700440900 ) ) ;
#35169=CARTESIAN_POINT ( 'NONE',  ( -0.9378221735089291577, 21.00000000000001066, -34.16632260368298546 ) ) ;
#35170=CARTESIAN_POINT ( 'NONE',  ( 3.500000000000001776, 19.52072594216370405, -31.37764746908818125 ) ) ;
#35171=CARTESIAN_POINT ( 'NONE',  ( -0.9378221735089291577, 21.00000000000001421, -66.16632260368297125 ) ) ;
#35172=CARTESIAN_POINT ( 'NONE',  ( 0.9378221735089281585, 14.00000000000001776, -82.66632260368299967 ) ) ;
#35173=CARTESIAN_POINT ( 'NONE',  ( 3.500000000000001332, 17.50000000000002132, -106.1547308033774186 ) ) ;
#35175=CARTESIAN_POINT ( 'NONE',  ( 1.750000000000001110, 20.53108891324556140, -137.2943141357548598 ) ) ;
#35177=CARTESIAN_POINT ( 'NONE',  ( -1.655278471875002211, 14.63297358603755249, -123.5974391362328078 ) ) ;
#35180=CYLINDRICAL_SURFACE ( 'NONE', #30644, 3.499999999999999556 ) ;
#35181=CARTESIAN_POINT ( 'NONE',  ( 3.500000000000001332, 17.50000000000001776, -91.46098080242151696 ) ) ;
#35182=CARTESIAN_POINT ( 'NONE',  ( 1.655278471875001101, 20.36702641396249547, -115.1849391362327850 ) ) ;
#35183=DIRECTION ( 'NONE',  ( -0.000000000000000000, 1.259100132267607459E-16, -1.000000000000000000 ) ) ;
#35184=CARTESIAN_POINT ( 'NONE',  ( 1.750000000000001110, 20.53108891324554719, -30.98806413671076498 ) ) ;
#35185=DIRECTION ( 'NONE',  ( 0.000000000000000000, 1.000000000000000000, 0.000000000000000000 ) ) ;
#35187=CARTESIAN_POINT ( 'NONE',  ( 3.310556943750001313, 19.41135094264167549, -137.2682724695661420 ) ) ;
#35189=CARTESIAN_POINT ( 'NONE',  ( 0.000000000000000000, 17.50000000000002487, -149.5231586289125687 ) ) ;
#35190=CARTESIAN_POINT ( 'NONE',  ( -1.655278471874999990, 20.36702641396248836, -48.01827246956613493 ) ) ;
#35193=CARTESIAN_POINT ( 'NONE',  ( -3.310556943750000425, 19.41135094264166128, -68.93493913623279923 ) ) ;
#35195=CARTESIAN_POINT ( 'NONE',  ( 1.655278471875001101, 20.36702641396248836, -68.09743913623280775 ) ) ;
#35197=ORIENTED_EDGE ( 'NONE', *, *, #6369, .T. ) ;
#35198=CARTESIAN_POINT ( 'NONE',  ( -3.310556943750001313, 17.50000000000001776, -89.85160580289947063 ) ) ;
#35200=CARTESIAN_POINT ( 'NONE',  ( 0.9378221735089300459, 21.00000000000001421, -49.25563900116002003 ) ) ;
#35202=CARTESIAN_POINT ( 'NONE',  ( 4.648177544792955347E-16, 21.00000000000001421, -70.21098080242150274 ) ) ;
#35203=CARTESIAN_POINT ( 'NONE',  ( -3.310556943750001313, 17.50000000000001421, -48.76410580289947205 ) ) ;
#35204=EDGE_CURVE ( 'NONE', #25124, #34399, #22613, .T. ) ;
#35206=CARTESIAN_POINT ( 'NONE',  ( -3.310556943750001313, 17.50000000000002132, -103.7641058028994649 ) ) ;
#35207=CARTESIAN_POINT ( 'NONE',  ( -0.9378221735089291577, 21.00000000000001066, -36.16632260368298546 ) ) ;
#35208=EDGE_CURVE ( 'NONE', #1017, #33859, #33350, .T. ) ;
#35214=CARTESIAN_POINT ( 'NONE',  ( 1.655278471875001101, 20.36702641396248836, -58.09743913623280065 ) ) ;
#35215=ORIENTED_EDGE ( 'NONE', *, *, #13750, .T. ) ;
#35217=VECTOR ( 'NONE', #4554, 1000.000000000000000 ) ;
#35224=CARTESIAN_POINT ( 'NONE',  ( -1.655278471874999990, 20.36702641396249547, -124.9307724695661364 ) ) ;
#35226=CARTESIAN_POINT ( 'NONE',  ( -0.9378221735089221633, 14.00000000000001599, -128.4493890021159359 ) ) ;
#35227=EDGE_CURVE ( 'NONE', #9388, #24647, #16230, .T. ) ;
#35229=CARTESIAN_POINT ( 'NONE',  ( -3.310556943750002645, 15.58864905735836537, -34.76827246956614204 ) ) ;
#35230=CARTESIAN_POINT ( 'NONE',  ( -7.022189441860112050E-16, 13.67729811471671475, -28.60160580289947063 ) ) ;
#35231=CARTESIAN_POINT ( 'NONE',  ( 1.655278471875001101, 20.36702641396249192, -87.18493913623278502 ) ) ;
#35232=CARTESIAN_POINT ( 'NONE',  ( 1.655278471874998436, 14.63297358603755249, -141.4307724695661364 ) ) ;
#35235=CARTESIAN_POINT ( 'NONE',  ( 1.655278471874998436, 14.63297358603755072, -131.5182724695661136 ) ) ;
#35236=DIRECTION ( 'NONE',  ( 0.000000000000000000, 1.000000000000000000, 0.000000000000000000 ) ) ;
#35237=CYLINDRICAL_SURFACE ( 'NONE', #15178, 3.499999999999999556 ) ;
#35240=CARTESIAN_POINT ( 'NONE',  ( -1.750000000000002220, 14.46891108675448301, -81.48806413671076143 ) ) ;
#35241=CARTESIAN_POINT ( 'NONE',  ( 3.310556943750001313, 19.41135094264166483, -62.26827246956613493 ) ) ;
#35245=CARTESIAN_POINT ( 'NONE',  ( 3.310556943749999981, 15.58864905735836892, -87.43493913623278502 ) ) ;
#35246=CARTESIAN_POINT ( 'NONE',  ( -0.9378221735089136146, 14.00000000000001066, -116.4493890021159359 ) ) ;
#35247=VECTOR ( 'NONE', #13983, 1000.000000000000000 ) ;
#35248=CARTESIAN_POINT ( 'NONE',  ( 2.340729813953370519E-16, 21.32270188528331900, -112.0141058028994792 ) ) ;
#35252=CARTESIAN_POINT ( 'NONE',  ( -1.750000000000002220, 14.46891108675448656, -110.4880641367107614 ) ) ;
#35255=CARTESIAN_POINT ( 'NONE',  ( 4.648177544792955347E-16, 21.00000000000001421, -68.21098080242148853 ) ) ;
#35256=DIRECTION ( 'NONE',  ( 0.000000000000000000, 1.000000000000000000, 0.000000000000000000 ) ) ;
#35257=CARTESIAN_POINT ( 'NONE',  ( 0.9378221735089281585, 14.00000000000001243, -59.36007260463891555 ) ) ;
#35259=CARTESIAN_POINT ( 'NONE',  ( -3.310556943750002201, 15.58864905735836892, -65.68077246956613635 ) ) ;
#35260=ADVANCED_FACE ( 'NONE', ( #16044 ), #3670, .T. ) ;
#35261=EDGE_CURVE ( 'NONE', #1748, #16391, #14615, .T. ) ;
#35263=CARTESIAN_POINT ( 'NONE',  ( -3.310556943750002645, 15.58864905735837780, -119.6807724695661506 ) ) ;
#35267=EDGE_LOOP ( 'NONE', ( #5820, #36744, #12515, #34487 ) ) ;
#35270=CARTESIAN_POINT ( 'NONE',  ( -1.655278471875002211, 14.63297358603754716, -81.59743913623280775 ) ) ;
#35271=ORIENTED_EDGE ( 'NONE', *, *, #29040, .F. ) ;
#35272=VERTEX_POINT ( 'NONE', #19218 ) ;
#35273=DIRECTION ( 'NONE',  ( 0.000000000000000000, 1.000000000000000000, 0.000000000000000000 ) ) ;
#35274=CARTESIAN_POINT ( 'NONE',  ( -3.310556943750002201, 15.58864905735837958, -138.6807724695661364 ) ) ;
#35277=CARTESIAN_POINT ( 'NONE',  ( -1.655278471875002211, 14.63297358603754184, -42.68493913623279212 ) ) ;
#35278=CARTESIAN_POINT ( 'NONE',  ( 1.655278471874998436, 14.63297358603754716, -102.5182724695661278 ) ) ;
#35280=ADVANCED_FACE ( 'NONE', ( #9868 ), #28985, .T. ) ;
#35282=CARTESIAN_POINT ( 'NONE',  ( 3.310556943749999981, 15.58864905735836182, -28.34743913623280775 ) ) ;
#35283=CARTESIAN_POINT ( 'NONE',  ( -7.022189441860112050E-16, 13.67729811471671830, -63.60160580289946353 ) ) ;
#35284=CARTESIAN_POINT ( 'NONE',  ( 1.749999999999998224, 14.46891108675448301, -104.6276474690881741 ) ) ;
#35288=CARTESIAN_POINT ( 'NONE',  ( -3.500000000000001332, 17.50000000000001776, -96.65473080337743284 ) ) ;
#35289=CARTESIAN_POINT ( 'NONE',  ( 3.500000000000000000, 15.47927405783632437, -63.54431413575484555 ) ) ;
#35290=( BOUNDED_CURVE ( )  B_SPLINE_CURVE ( 2, ( #39394, #23237, #23679, #20264, #10270, #33450, #17504, #36642, #26863 ),
 .UNSPECIFIED., .F., .T. ) 
 B_SPLINE_CURVE_WITH_KNOTS ( ( 3, 2, 2, 2, 3 ),
 ( 0.5187500000000000444, 0.5194444444444444864, 0.5208333333333333703, 0.5222222222222222543, 0.5229166666666666963 ),
 .UNSPECIFIED. ) 
 CURVE ( )  GEOMETRIC_REPRESENTATION_ITEM ( )  RATIONAL_B_SPLINE_CURVE ( ( 0.9330127018922194093, 0.9330127018922194093, 1.000000000000000000, 0.8660254037844387076, 1.000000000000000000, 0.8660254037844387076, 1.000000000000000000, 0.9330127018922194093, 0.9330127018922194093 ) ) 
 REPRESENTATION_ITEM ( '' )  );
#35293=CARTESIAN_POINT ( 'NONE',  ( -7.424026671074350129E-16, 13.45854811567263454, -60.71098080242150274 ) ) ;
#35295=CARTESIAN_POINT ( 'NONE',  ( -3.310556943750000425, 19.41135094264165772, -26.84743913623280420 ) ) ;
#35296=CARTESIAN_POINT ( 'NONE',  ( 1.750000000000001110, 20.53108891324555074, -49.98806413671076854 ) ) ;
#35298=CARTESIAN_POINT ( 'NONE',  ( 3.310556943750001313, 19.41135094264166128, -34.26827246956613493 ) ) ;
#35304=DIRECTION ( 'NONE',  ( -0.000000000000000000, 1.259100132267607459E-16, -1.000000000000000000 ) ) ;
#35306=CARTESIAN_POINT ( 'NONE',  ( 1.655278471874998436, 14.63297358603754539, -84.43077246956613635 ) ) ;
#35307=ORIENTED_EDGE ( 'NONE', *, *, #35261, .T. ) ;
#35308=CARTESIAN_POINT ( 'NONE',  ( -0.9378221735089310451, 14.00000000000001066, -35.44938900211595723 ) ) ;
#35311=ORIENTED_EDGE ( 'NONE', *, *, #17648, .T. ) ;
#35314=CARTESIAN_POINT ( 'NONE',  ( 1.655278471874998436, 14.63297358603754716, -96.43077246956613635 ) ) ;
#35317=CARTESIAN_POINT ( 'NONE',  ( 1.750000000000001110, 20.53108891324555785, -120.9880641367107614 ) ) ;
#35321=CARTESIAN_POINT ( 'NONE',  ( -0.9378221735089291577, 21.00000000000001776, -84.86007260463890134 ) ) ;
#35325=CYLINDRICAL_SURFACE ( 'NONE', #36397, 3.499999999999999556 ) ;
#35326=CARTESIAN_POINT ( 'NONE',  ( 3.310556943749999981, 15.58864905735837425, -129.3474391362328220 ) ) ;
#35328=EDGE_LOOP ( 'NONE', ( #1434, #33700, #416, #38108 ) ) ;
#35329=CARTESIAN_POINT ( 'NONE',  ( 3.369928719974892676E-15, 14.00000000000002309, -139.4047308033773618 ) ) ;
#35330=CARTESIAN_POINT ( 'NONE',  ( -3.310556943750000425, 19.41135094264166838, -117.9349391362327992 ) ) ;
#35331=CARTESIAN_POINT ( 'NONE',  ( 2.340729813953370519E-16, 21.32270188528330834, -49.10160580289945642 ) ) ;
#35333=CARTESIAN_POINT ( 'NONE',  ( 1.749999999999998224, 14.46891108675448656, -131.3213974700441042 ) ) ;
#35334=AXIS2_PLACEMENT_3D ( 'NONE', #33743, #33945, #13964 ) ;
#35336=CARTESIAN_POINT ( 'NONE',  ( -7.022189441860112050E-16, 13.67729811471672186, -75.60160580289944221 ) ) ;
#35337=CARTESIAN_POINT ( 'NONE',  ( -3.500000000000001332, 17.50000000000002132, -122.9609808024215027 ) ) ;
#35338=CARTESIAN_POINT ( 'NONE',  ( 3.310556943749999981, 15.58864905735837070, -105.3474391362328078 ) ) ;
#35339=CARTESIAN_POINT ( 'NONE',  ( 4.648177544792955347E-16, 21.00000000000001776, -80.90473080337743284 ) ) ;
#35342=CARTESIAN_POINT ( 'NONE',  ( -3.500000000000000888, 19.52072594216370760, -74.04431413575484555 ) ) ;
#35345=CARTESIAN_POINT ( 'NONE',  ( 3.310556943749999981, 15.58864905735836182, -43.34743913623280775 ) ) ;
#35347=CARTESIAN_POINT ( 'NONE',  ( -3.310556943750000425, 19.41135094264166483, -100.9349391362328134 ) ) ;
#35348=CARTESIAN_POINT ( 'NONE',  ( -1.394453263437886604E-15, 14.00000000000001776, -86.40473080337743284 ) ) ;
#35349=CARTESIAN_POINT ( 'NONE',  ( -3.500000000000002220, 15.47927405783632437, -65.57139747004409003 ) ) ;
#35351=ORIENTED_EDGE ( 'NONE', *, *, #36045, .F. ) ;
#35352=CARTESIAN_POINT ( 'NONE',  ( 1.655278471874998436, 14.63297358603754894, -117.5182724695661278 ) ) ;
#35353=CARTESIAN_POINT ( 'NONE',  ( -3.500000000000000000, 19.52072594216370405, -28.04431413575483845 ) ) ;
#35354=EDGE_CURVE ( 'NONE', #5144, #40976, #14099, .T. ) ;
#35362=CARTESIAN_POINT ( 'NONE',  ( -3.500000000000000000, 19.52072594216370405, -29.04431413575483845 ) ) ;
#35363=CARTESIAN_POINT ( 'NONE',  ( 3.500000000000000000, 15.47927405783632793, -81.54431413575484555 ) ) ;
#35364=CARTESIAN_POINT ( 'NONE',  ( -1.394453263437886604E-15, 14.00000000000001421, -80.40473080337743284 ) ) ;
#35368=CARTESIAN_POINT ( 'NONE',  ( -3.310556943750002201, 15.58864905735836537, -34.68077246956615056 ) ) ;
#35369=CARTESIAN_POINT ( 'NONE',  ( 3.500000000000000000, 15.47927405783632615, -72.23806413671076143 ) ) ;
#35374=DIRECTION ( 'NONE',  ( 0.000000000000000000, 1.000000000000000000, 0.000000000000000000 ) ) ;
#35380=FACE_OUTER_BOUND ( 'NONE', #32009, .T. ) ;
#35381=CARTESIAN_POINT ( 'NONE',  ( -3.500000000000002220, 15.47927405783633503, -116.5713974700440900 ) ) ;
#35383=CARTESIAN_POINT ( 'NONE',  ( -3.500000000000002220, 15.47927405783632082, -35.87764746908816704 ) ) ;
#35384=FACE_OUTER_BOUND ( 'NONE', #35562, .T. ) ;
#35385=CARTESIAN_POINT ( 'NONE',  ( 3.500000000000001332, 17.50000000000001066, -32.46098080242150274 ) ) ;
#35386=CARTESIAN_POINT ( 'NONE',  ( 3.500000000000001332, 19.52072594216371826, -106.0713974700441184 ) ) ;
#35388=CARTESIAN_POINT ( 'NONE',  ( -1.749999999999999778, 20.53108891324556140, -141.1276474690881741 ) ) ;
#35389=CARTESIAN_POINT ( 'NONE',  ( -1.750000000000002220, 14.46891108675447768, -52.79431413575484555 ) ) ;
#35390=CARTESIAN_POINT ( 'NONE',  ( 3.310556943749999981, 15.58864905735837425, -125.3474391362328078 ) ) ;
#35395=CARTESIAN_POINT ( 'NONE',  ( -1.750000000000002220, 14.46891108675448301, -90.79431413575484555 ) ) ;
#35396=CARTESIAN_POINT ( 'NONE',  ( 3.500000000000001332, 19.52072594216370405, -33.07139747004410424 ) ) ;
#35397=CARTESIAN_POINT ( 'NONE',  ( 1.655278471874998436, 14.63297358603754184, -59.43077246956614346 ) ) ;
#35398=CARTESIAN_POINT ( 'NONE',  ( 1.655278471874998436, 14.63297358603754894, -118.5182724695661278 ) ) ;
#35399=CYLINDRICAL_SURFACE ( 'NONE', #2365, 3.499999999999999556 ) ;
#35400=CARTESIAN_POINT ( 'NONE',  ( 1.749999999999998224, 14.46891108675447413, -35.32139747004409003 ) ) ;
#35403=CARTESIAN_POINT ( 'NONE',  ( -3.310556943750002201, 15.58864905735837780, -133.7682724695661420 ) ) ;
#35404=EDGE_CURVE ( 'NONE', #6975, #31031, #33618, .T. ) ;
#35407=CARTESIAN_POINT ( 'NONE',  ( 1.655278471875001101, 20.36702641396248481, -45.18493913623279923 ) ) ;
#35409=CARTESIAN_POINT ( 'NONE',  ( -7.022189441860112050E-16, 13.67729811471672186, -67.60160580289947063 ) ) ;
#35411=CARTESIAN_POINT ( 'NONE',  ( -3.310556943750002645, 15.58864905735836892, -62.68077246956614346 ) ) ;
#35414=CARTESIAN_POINT ( 'NONE',  ( -1.655278471874999990, 20.36702641396249192, -90.01827246956612782 ) ) ;
#35417=CARTESIAN_POINT ( 'NONE',  ( 4.648177544792955347E-16, 21.00000000000002487, -131.2109808024214885 ) ) ;
#35418=CARTESIAN_POINT ( 'NONE',  ( 2.340729813953370519E-16, 21.32270188528331190, -53.01410580289947205 ) ) ;
#35419=( BOUNDED_CURVE ( )  B_SPLINE_CURVE ( 2, ( #17621, #20386, #40575, #11430, #24422, #7206, #4002, #26777, #39742 ),
 .UNSPECIFIED., .F., .F. ) 
 B_SPLINE_CURVE_WITH_KNOTS ( ( 3, 2, 2, 2, 3 ),
 ( 0.1812499999999999944, 0.1819444444444444364, 0.1833333333333333204, 0.1847222222222222321, 0.1854166666666666741 ),
 .UNSPECIFIED. ) 
 CURVE ( )  GEOMETRIC_REPRESENTATION_ITEM ( )  RATIONAL_B_SPLINE_CURVE ( ( 0.9330127018922194093, 0.9330127018922194093, 1.000000000000000000, 0.8660254037844387076, 1.000000000000000000, 0.8660254037844387076, 1.000000000000000000, 0.9330127018922194093, 0.9330127018922194093 ) ) 
 REPRESENTATION_ITEM ( '' )  );
#35421=CARTESIAN_POINT ( 'NONE',  ( -1.655278471875002211, 14.63297358603754894, -107.5974391362328078 ) ) ;
#35422=CARTESIAN_POINT ( 'NONE',  ( -1.750000000000002220, 14.46891108675447590, -35.79431413575484555 ) ) ;
#35428=CARTESIAN_POINT ( 'NONE',  ( 1.655278471874998436, 14.63297358603754184, -60.43077246956614346 ) ) ;
#35433=CARTESIAN_POINT ( 'NONE',  ( -0.9378221735089310451, 14.00000000000001066, -40.44938900211595723 ) ) ;
#35435=CYLINDRICAL_SURFACE ( 'NONE', #14317, 3.499999999999999556 ) ;
#35437=CARTESIAN_POINT ( 'NONE',  ( 1.749999999999998224, 14.46891108675447413, -35.32139747004409003 ) ) ;
#35438=CARTESIAN_POINT ( 'NONE',  ( -1.655278471874999990, 20.36702641396249547, -125.9307724695661364 ) ) ;
#35439=CARTESIAN_POINT ( 'NONE',  ( 0.000000000000000000, 21.00000000000002487, -149.5231586289125687 ) ) ;
#35442=CARTESIAN_POINT ( 'NONE',  ( 3.310556943749999981, 15.58864905735836182, -35.43493913623279923 ) ) ;
#35443=CARTESIAN_POINT ( 'NONE',  ( -3.310556943750001313, 17.50000000000001066, -25.85160580289947063 ) ) ;
#35444=CARTESIAN_POINT ( 'NONE',  ( -3.310556943750000425, 19.41135094264166483, -89.93493913623278502 ) ) ;
#35445=CARTESIAN_POINT ( 'NONE',  ( -3.310556943750001313, 17.50000000000002487, -136.7641058028994792 ) ) ;
#35448=CARTESIAN_POINT ( 'NONE',  ( 3.500000000000001332, 19.52072594216371826, -127.0713974700440900 ) ) ;
#35449=CARTESIAN_POINT ( 'NONE',  ( -1.750000000000002220, 14.46891108675447590, -34.48806413671076854 ) ) ;
#35450=CARTESIAN_POINT ( 'NONE',  ( -3.310556943750001313, 17.50000000000002487, -131.8516058028994564 ) ) ;
#35454=CARTESIAN_POINT ( 'NONE',  ( 4.648177544792955347E-16, 21.00000000000002132, -122.9047308033774044 ) ) ;
#35455=CARTESIAN_POINT ( 'NONE',  ( 3.500000000000001332, 17.50000000000001776, -80.15473080337743284 ) ) ;
#35456=CARTESIAN_POINT ( 'NONE',  ( 3.310556943750001313, 19.41135094264166483, -64.26827246956614204 ) ) ;
#35460=VECTOR ( 'NONE', #37372, 1000.000000000000000 ) ;
#35461=CARTESIAN_POINT ( 'NONE',  ( 2.340729813953370519E-16, 21.32270188528331190, -83.10160580289947063 ) ) ;
#35462=CARTESIAN_POINT ( 'NONE',  ( 4.648177544792955347E-16, 21.00000000000001776, -77.90473080337740441 ) ) ;
#35463=CARTESIAN_POINT ( 'NONE',  ( 2.340729813953370519E-16, 21.32270188528331900, -117.0141058028994792 ) ) ;
#35464=CARTESIAN_POINT ( 'NONE',  ( -1.655278471874999990, 20.36702641396249192, -78.93077246956615056 ) ) ;
#35465=CARTESIAN_POINT ( 'NONE',  ( -3.500000000000001332, 17.50000000000001776, -96.65473080337743284 ) ) ;
#35466=EDGE_LOOP ( 'NONE', ( #6507, #31640, #41877, #19824 ) ) ;
#35467=CARTESIAN_POINT ( 'NONE',  ( -3.500000000000002220, 15.47927405783632970, -108.5713974700441042 ) ) ;
#35470=DIRECTION ( 'NONE',  ( -0.000000000000000000, 1.259100132267607459E-16, -1.000000000000000000 ) ) ;
#35472=CARTESIAN_POINT ( 'NONE',  ( -0.9378221735089291577, 21.00000000000001066, -27.16632260368299256 ) ) ;
#35473=CARTESIAN_POINT ( 'NONE',  ( 3.500000000000001332, 17.50000000000001421, -65.46098080242150274 ) ) ;
#35475=CARTESIAN_POINT ( 'NONE',  ( 3.310556943749999981, 15.58864905735836537, -65.34743913623280775 ) ) ;
#35477=ADVANCED_FACE ( 'NONE', ( #12142 ), #24304, .T. ) ;
#35478=CARTESIAN_POINT ( 'NONE',  ( 2.340729813953370519E-16, 21.32270188528331900, -119.0141058028994792 ) ) ;
#35479=FACE_OUTER_BOUND ( 'NONE', #41829, .T. ) ;
#35480=( BOUNDED_CURVE ( )  B_SPLINE_CURVE ( 2, ( #23393, #23608, #30398, #26580, #10835, #26368, #39319, #23169, #27007 ),
 .UNSPECIFIED., .F., .T. ) 
 B_SPLINE_CURVE_WITH_KNOTS ( ( 3, 2, 2, 2, 3 ),
 ( 0.8895833333333332815, 0.8902777777777777235, 0.8916666666666667185, 0.8930555555555556024, 0.8937500000000000444 ),
 .UNSPECIFIED. ) 
 CURVE ( )  GEOMETRIC_REPRESENTATION_ITEM ( )  RATIONAL_B_SPLINE_CURVE ( ( 0.9330127018922194093, 0.9330127018922194093, 1.000000000000000000, 0.8660254037844387076, 1.000000000000000000, 0.8660254037844387076, 1.000000000000000000, 0.9330127018922194093, 0.9330127018922194093 ) ) 
 REPRESENTATION_ITEM ( '' )  );
#35483=EDGE_CURVE ( 'NONE', #1932, #19108, #15140, .T. ) ;
#35484=VERTEX_POINT ( 'NONE', #1947 ) ;
#35485=CARTESIAN_POINT ( 'NONE',  ( 1.750000000000001110, 20.53108891324555429, -99.29431413575484555 ) ) ;
#35486=CARTESIAN_POINT ( 'NONE',  ( -1.750000000000002220, 14.46891108675447590, -31.79431413575484200 ) ) ;
#35487=CARTESIAN_POINT ( 'NONE',  ( 1.655278471875001101, 20.36702641396248836, -74.09743913623280775 ) ) ;
#35488=EDGE_LOOP ( 'NONE', ( #28528, #33386, #5434, #10310 ) ) ;
#35492=CARTESIAN_POINT ( 'NONE',  ( 3.310556943750001313, 19.41135094264167549, -142.1807724695661364 ) ) ;
#35494=CARTESIAN_POINT ( 'NONE',  ( -1.394453263437886604E-15, 14.00000000000001776, -101.7109808024215027 ) ) ;
#35495=CARTESIAN_POINT ( 'NONE',  ( 3.310556943750001313, 17.50000000000001066, -41.35160580289947063 ) ) ;
#35496=CARTESIAN_POINT ( 'NONE',  ( -1.655278471875002211, 14.63297358603754894, -103.6849391362328134 ) ) ;
#35498=CARTESIAN_POINT ( 'NONE',  ( 3.310556943750001313, 17.50000000000001066, -27.26410580289947916 ) ) ;
#35499=CARTESIAN_POINT ( 'NONE',  ( -3.500000000000001332, 17.50000000000002132, -111.9609808024215027 ) ) ;
#35500=CARTESIAN_POINT ( 'NONE',  ( 2.474675557024783212E-16, 21.54145188432740099, -107.2109808024215027 ) ) ;
#35502=CARTESIAN_POINT ( 'NONE',  ( 1.749999999999998224, 14.46891108675448834, -142.3213974700441042 ) ) ;
#35503=CARTESIAN_POINT ( 'NONE',  ( -3.500000000000002220, 15.47927405783632970, -98.57139747004407582 ) ) ;
#35507=CARTESIAN_POINT ( 'NONE',  ( -3.500000000000001332, 17.50000000000001421, -56.96098080242150985 ) ) ;
#35508=CARTESIAN_POINT ( 'NONE',  ( 4.286263797015737581E-16, 14.00000000000002487, -149.5231586289125687 ) ) ;
#35509=CARTESIAN_POINT ( 'NONE',  ( 3.310556943750001313, 17.50000000000001066, -28.26410580289947916 ) ) ;
#35510=CARTESIAN_POINT ( 'NONE',  ( 3.500000000000001776, 19.52072594216370760, -50.07139747004410424 ) ) ;
#35511=CARTESIAN_POINT ( 'NONE',  ( 3.500000000000000000, 15.47927405783632970, -106.5443141357548456 ) ) ;
#35513=CARTESIAN_POINT ( 'NONE',  ( 1.655278471875001101, 20.36702641396248481, -35.18493913623279923 ) ) ;
#35515=CARTESIAN_POINT ( 'NONE',  ( 0.9378221735089300459, 21.00000000000001421, -65.94938900211595012 ) ) ;
#35516=CARTESIAN_POINT ( 'NONE',  ( -0.9378221735089291577, 21.00000000000002132, -121.1663226036829855 ) ) ;
#35521=CARTESIAN_POINT ( 'NONE',  ( 1.655278471875001101, 20.36702641396249192, -81.09743913623280775 ) ) ;
#35523=CARTESIAN_POINT ( 'NONE',  ( 1.750000000000001110, 20.53108891324555074, -52.29431413575484555 ) ) ;
#35525=CARTESIAN_POINT ( 'NONE',  ( 3.500000000000001332, 19.52072594216370405, -34.07139747004410424 ) ) ;
#35526=ORIENTED_EDGE ( 'NONE', *, *, #5077, .T. ) ;
#35529=CARTESIAN_POINT ( 'NONE',  ( -1.655278471874999990, 20.36702641396249192, -87.93077246956613635 ) ) ;
#35530=ORIENTED_EDGE ( 'NONE', *, *, #14862, .F. ) ;
#35534=ADVANCED_FACE ( 'NONE', ( #2374 ), #34077, .T. ) ;
#35536=VERTEX_POINT ( 'NONE', #40463 ) ;
#35539=CARTESIAN_POINT ( 'NONE',  ( 2.340729813953370519E-16, 21.32270188528332255, -134.0141058028994792 ) ) ;
#35540=ORIENTED_EDGE ( 'NONE', *, *, #16684, .T. ) ;
#35541=CARTESIAN_POINT ( 'NONE',  ( 1.749999999999998224, 14.46891108675448834, -139.3213974700441042 ) ) ;
#35542=CARTESIAN_POINT ( 'NONE',  ( 3.310556943749999981, 15.58864905735837247, -121.4349391362327992 ) ) ;
#35543=CARTESIAN_POINT ( 'NONE',  ( -1.655278471875002211, 14.63297358603754184, -51.68493913623279923 ) ) ;
#35545=EDGE_CURVE ( 'NONE', #6382, #19056, #38101, .T. ) ;
#35546=CARTESIAN_POINT ( 'NONE',  ( -7.424026671074350129E-16, 13.45854811567264164, -129.4047308033774186 ) ) ;
#35549=CARTESIAN_POINT ( 'NONE',  ( 1.655278471874998436, 14.63297358603754361, -72.51827246956612782 ) ) ;
#35550=CARTESIAN_POINT ( 'NONE',  ( -7.424026671074350129E-16, 13.45854811567264164, -123.7109808024215027 ) ) ;
#35551=CARTESIAN_POINT ( 'NONE',  ( -1.655278471875002211, 14.63297358603755072, -109.5974391362328078 ) ) ;
#35552=FACE_OUTER_BOUND ( 'NONE', #20674, .T. ) ;
#35555=CARTESIAN_POINT ( 'NONE',  ( 3.500000000000001332, 17.50000000000001776, -75.46098080242151696 ) ) ;
#35557=CARTESIAN_POINT ( 'NONE',  ( -7.022189441860112050E-16, 13.67729811471671653, -44.51410580289948626 ) ) ;
#35558=CARTESIAN_POINT ( 'NONE',  ( 1.655278471874998436, 14.63297358603754716, -102.5182724695661278 ) ) ;
#35559=CARTESIAN_POINT ( 'NONE',  ( -1.749999999999999778, 20.53108891324555785, -114.1276474690881741 ) ) ;
#35560=CARTESIAN_POINT ( 'NONE',  ( 3.500000000000001776, 19.52072594216370760, -65.07139747004410424 ) ) ;
#35561=DIRECTION ( 'NONE',  ( 0.000000000000000000, 1.000000000000000000, 0.000000000000000000 ) ) ;
#35562=EDGE_LOOP ( 'NONE', ( #7704, #28714, #11263, #29878 ) ) ;
#35563=CARTESIAN_POINT ( 'NONE',  ( 1.655278471874998436, 14.63297358603754894, -116.5182724695661278 ) ) ;
#35564=CARTESIAN_POINT ( 'NONE',  ( 4.648177544792955347E-16, 21.00000000000002132, -122.9047308033774044 ) ) ;
#35569=CARTESIAN_POINT ( 'NONE',  ( -7.022189441860112050E-16, 13.67729811471672541, -97.51410580289947916 ) ) ;
#35573=CARTESIAN_POINT ( 'NONE',  ( -1.749999999999999778, 20.53108891324554719, -29.12764746908817770 ) ) ;
#35574=CARTESIAN_POINT ( 'NONE',  ( -0.9378221735089291577, 21.00000000000002132, -118.8600726046389013 ) ) ;
#35575=VECTOR ( 'NONE', #36621, 1000.000000000000000 ) ;
#35576=CARTESIAN_POINT ( 'NONE',  ( -1.750000000000002220, 14.46891108675448656, -112.4880641367107614 ) ) ;
#35580=CARTESIAN_POINT ( 'NONE',  ( -3.310556943750001313, 17.50000000000001066, -36.76410580289947205 ) ) ;
#35581=CARTESIAN_POINT ( 'NONE',  ( 3.500000000000001332, 17.50000000000002132, -107.1547308033774186 ) ) ;
#35588=ORIENTED_EDGE ( 'NONE', *, *, #22519, .T. ) ;
#35590=CARTESIAN_POINT ( 'NONE',  ( -0.9378221735089310451, 14.00000000000002132, -85.75563900116002003 ) ) ;
#35591=( BOUNDED_CURVE ( )  B_SPLINE_CURVE ( 2, ( #6958, #38871, #793, #29922, #36517, #29280, #29496, #19514, #32484 ),
 .UNSPECIFIED., .F., .F. ) 
 B_SPLINE_CURVE_WITH_KNOTS ( ( 3, 2, 2, 2, 3 ),
 ( 0.4562499999999999889, 0.4569444444444444309, 0.4583333333333333148, 0.4597222222222221988, 0.4604166666666666963 ),
 .UNSPECIFIED. ) 
 CURVE ( )  GEOMETRIC_REPRESENTATION_ITEM ( )  RATIONAL_B_SPLINE_CURVE ( ( 0.9330127018922194093, 0.9330127018922194093, 1.000000000000000000, 0.8660254037844387076, 1.000000000000000000, 0.8660254037844387076, 1.000000000000000000, 0.9330127018922167448, 0.9330127018922194093 ) ) 
 REPRESENTATION_ITEM ( '' )  );
#35593=CARTESIAN_POINT ( 'NONE',  ( -7.424026671074350129E-16, 13.45854811567263987, -121.4047308033774470 ) ) ;
#35596=CARTESIAN_POINT ( 'NONE',  ( -3.310556943750001313, 17.50000000000002487, -135.8516058028994564 ) ) ;
#35597=CARTESIAN_POINT ( 'NONE',  ( 1.749999999999998224, 14.46891108675447413, -32.62764746908818125 ) ) ;
#35598=CARTESIAN_POINT ( 'NONE',  ( -1.394453263437886604E-15, 14.00000000000001066, -35.71098080242150985 ) ) ;
#35599=CARTESIAN_POINT ( 'NONE',  ( 1.749999999999998224, 14.46891108675447413, -32.62764746908818125 ) ) ;
#35600=( BOUNDED_CURVE ( )  B_SPLINE_CURVE ( 2, ( #23442, #36407, #27670, #18103, #14289, #24909, #37052, #30446, #41063 ),
 .UNSPECIFIED., .F., .T. ) 
 B_SPLINE_CURVE_WITH_KNOTS ( ( 3, 2, 2, 2, 3 ),
 ( 0.06041666666666666713, 0.06111111111111110911, 0.06250000000000000000, 0.06388888888888888395, 0.06458333333333333981 ),
 .UNSPECIFIED. ) 
 CURVE ( )  GEOMETRIC_REPRESENTATION_ITEM ( )  RATIONAL_B_SPLINE_CURVE ( ( 0.9330127018922194093, 0.9330127018922194093, 1.000000000000000000, 0.8660254037844387076, 1.000000000000000000, 0.8660254037844387076, 1.000000000000000000, 0.9330127018922187432, 0.9330127018922194093 ) ) 
 REPRESENTATION_ITEM ( '' )  );
#35604=CARTESIAN_POINT ( 'NONE',  ( 3.500000000000000000, 15.47927405783633503, -140.5443141357548313 ) ) ;
#35605=CARTESIAN_POINT ( 'NONE',  ( -1.655278471874999990, 20.36702641396249547, -125.9307724695661364 ) ) ;
#35608=CARTESIAN_POINT ( 'NONE',  ( 0.000000000000000000, 17.50000000000002487, -149.5231586289125687 ) ) ;
#35609=CARTESIAN_POINT ( 'NONE',  ( -3.500000000000002220, 15.47927405783632793, -89.87764746908817415 ) ) ;
#35611=CARTESIAN_POINT ( 'NONE',  ( -3.310556943750002645, 15.58864905735836892, -57.68077246956614346 ) ) ;
#35612=CARTESIAN_POINT ( 'NONE',  ( -1.655278471875002211, 14.63297358603755072, -119.6849391362327992 ) ) ;
#35613=DIRECTION ( 'NONE',  ( 0.000000000000000000, 1.000000000000000000, 0.000000000000000000 ) ) ;
#35614=CARTESIAN_POINT ( 'NONE',  ( 3.500000000000000000, 15.47927405783632082, -35.23806413671076854 ) ) ;
#35615=FACE_OUTER_BOUND ( 'NONE', #30244, .T. ) ;
#35617=CARTESIAN_POINT ( 'NONE',  ( 3.310556943749999981, 15.58864905735837425, -132.4349391362327992 ) ) ;
#35619=CARTESIAN_POINT ( 'NONE',  ( 4.648177544792955347E-16, 21.00000000000001066, -29.90473080337743639 ) ) ;
#35620=CARTESIAN_POINT ( 'NONE',  ( -3.310556943750000425, 19.41135094264166128, -43.93493913623279212 ) ) ;
#35621=CARTESIAN_POINT ( 'NONE',  ( 0.000000000000000000, 17.50000000000002487, -149.5231586289125687 ) ) ;
#35622=CARTESIAN_POINT ( 'NONE',  ( 3.310556943749999981, 15.58864905735836714, -70.43493913623281344 ) ) ;
#35624=CARTESIAN_POINT ( 'NONE',  ( 2.340729813953370519E-16, 21.32270188528330834, -66.01410580289946495 ) ) ;
#35625=ORIENTED_EDGE ( 'NONE', *, *, #18655, .T. ) ;
#35626=CARTESIAN_POINT ( 'NONE',  ( 3.310556943750001313, 17.50000000000001776, -83.35160580289947063 ) ) ;
#35628=EDGE_CURVE ( 'NONE', #28459, #11127, #30890, .T. ) ;
#35629=CARTESIAN_POINT ( 'NONE',  ( 1.743066579297357930E-14, 14.00000000000002132, -134.4047308033774186 ) ) ;
#35630=CARTESIAN_POINT ( 'NONE',  ( 0.9378221735089281585, 14.00000000000002309, -131.6663226036829712 ) ) ;
#35631=CARTESIAN_POINT ( 'NONE',  ( -3.310556943750002201, 15.58864905735836714, -52.68077246956613635 ) ) ;
#35633=CARTESIAN_POINT ( 'NONE',  ( 1.655278471874998436, 14.63297358603754716, -103.4307724695661364 ) ) ;
#35635=AXIS2_PLACEMENT_3D ( 'NONE', #36550, #183, #6777 ) ;
#35641=CARTESIAN_POINT ( 'NONE',  ( -7.022189441860112050E-16, 13.67729811471671830, -59.51410580289948626 ) ) ;
#35644=CARTESIAN_POINT ( 'NONE',  ( 4.648177544792955347E-16, 21.00000000000001776, -76.21098080242148853 ) ) ;
#35645=VECTOR ( 'NONE', #21575, 1000.000000000000000 ) ;
#35648=CARTESIAN_POINT ( 'NONE',  ( 0.000000000000000000, 21.00000000000002487, -149.5231586289125687 ) ) ;
#35650=EDGE_LOOP ( 'NONE', ( #18304, #38656, #8020, #27588 ) ) ;
#35652=CARTESIAN_POINT ( 'NONE',  ( 1.655278471874998436, 14.63297358603755072, -127.4307724695661364 ) ) ;
#35655=CARTESIAN_POINT ( 'NONE',  ( 2.340729813953370519E-16, 21.32270188528330479, -34.10160580289946353 ) ) ;
#35656=CARTESIAN_POINT ( 'NONE',  ( -3.310556943750002645, 15.58864905735836537, -29.76827246956613493 ) ) ;
#35657=CARTESIAN_POINT ( 'NONE',  ( -7.022189441860112050E-16, 13.67729811471672363, -89.60160580289947063 ) ) ;
#35658=CARTESIAN_POINT ( 'NONE',  ( 1.655278471874998436, 14.63297358603755249, -138.4307724695661364 ) ) ;
#35662=CARTESIAN_POINT ( 'NONE',  ( -3.310556943750002645, 15.58864905735837780, -132.7682724695661136 ) ) ;
#35663=AXIS2_PLACEMENT_3D ( 'NONE', #775, #26728, #9731 ) ;
#35665=CARTESIAN_POINT ( 'NONE',  ( -3.310556943750001313, 17.50000000000001776, -91.76410580289947916 ) ) ;
#35667=CARTESIAN_POINT ( 'NONE',  ( 4.648177544792955347E-16, 21.00000000000001776, -93.21098080242150274 ) ) ;
#35668=CARTESIAN_POINT ( 'NONE',  ( 4.648177544792955347E-16, 21.00000000000002132, -126.2109808024214885 ) ) ;
#35669=CARTESIAN_POINT ( 'NONE',  ( -3.500000000000002220, 15.47927405783632615, -73.57139747004409003 ) ) ;
#35670=CARTESIAN_POINT ( 'NONE',  ( -1.655278471875002211, 14.63297358603754361, -56.68493913623279212 ) ) ;
#35671=( BOUNDED_CURVE ( )  B_SPLINE_CURVE ( 2, ( #6957, #20353, #19513, #33320, #19933, #6548, #32483, #3763, #29710 ),
 .UNSPECIFIED., .F., .T. ) 
 B_SPLINE_CURVE_WITH_KNOTS ( ( 3, 2, 2, 2, 3 ),
 ( 0.5979166666666666519, 0.5986111111111110938, 0.5999999999999999778, 0.6013888888888888618, 0.6020833333333333037 ),
 .UNSPECIFIED. ) 
 CURVE ( )  GEOMETRIC_REPRESENTATION_ITEM ( )  RATIONAL_B_SPLINE_CURVE ( ( 0.9330127018922194093, 0.9330127018922194093, 1.000000000000000000, 0.8660254037844387076, 1.000000000000000000, 0.8660254037844387076, 1.000000000000000000, 0.9330127018922194093, 0.9330127018922194093 ) ) 
 REPRESENTATION_ITEM ( '' )  );
#35675=CARTESIAN_POINT ( 'NONE',  ( -1.655278471874999990, 20.36702641396249192, -84.01827246956614204 ) ) ;
#35676=CARTESIAN_POINT ( 'NONE',  ( -1.750000000000002220, 14.46891108675447946, -59.79431413575483845 ) ) ;
#35677=CARTESIAN_POINT ( 'NONE',  ( 3.310556943750001313, 17.50000000000002132, -112.2641058028994792 ) ) ;
#35678=CARTESIAN_POINT ( 'NONE',  ( 3.310556943750001313, 17.50000000000001776, -83.26410580289947916 ) ) ;
#35679=CARTESIAN_POINT ( 'NONE',  ( 3.500000000000001332, 19.52072594216371826, -138.3776474690881741 ) ) ;
#35682=CARTESIAN_POINT ( 'NONE',  ( 3.500000000000001776, 19.52072594216371826, -108.0713974700441042 ) ) ;
#35683=VECTOR ( 'NONE', #10974, 1000.000000000000000 ) ;
#35686=CARTESIAN_POINT ( 'NONE',  ( 3.500000000000000000, 15.47927405783632082, -44.23806413671075433 ) ) ;
#35690=CARTESIAN_POINT ( 'NONE',  ( -1.655278471875002211, 14.63297358603754539, -68.59743913623280775 ) ) ;
#35691=CARTESIAN_POINT ( 'NONE',  ( 0.9378221735089300459, 21.00000000000001421, -59.25563900116002003 ) ) ;
#35692=CARTESIAN_POINT ( 'NONE',  ( 1.655278471875001101, 20.36702641396249547, -120.0974391362328078 ) ) ;
#35693=CARTESIAN_POINT ( 'NONE',  ( 1.749999999999998224, 14.46891108675447946, -71.32139747004409003 ) ) ;
#35694=CARTESIAN_POINT ( 'NONE',  ( -1.749999999999999778, 20.53108891324555785, -125.8213974700440900 ) ) ;
#35695=ORIENTED_EDGE ( 'NONE', *, *, #25670, .T. ) ;
#35696=CARTESIAN_POINT ( 'NONE',  ( 3.500000000000001332, 17.50000000000001776, -99.46098080242150274 ) ) ;
#35697=CARTESIAN_POINT ( 'NONE',  ( 3.500000000000001332, 19.52072594216371115, -79.07139747004410424 ) ) ;
#35698=CARTESIAN_POINT ( 'NONE',  ( 3.310556943749999981, 15.58864905735836714, -73.34743913623280775 ) ) ;
#35702=CARTESIAN_POINT ( 'NONE',  ( 1.655278471874998436, 14.63297358603755249, -142.4307724695661364 ) ) ;
#35705=DIRECTION ( 'NONE',  ( 0.000000000000000000, 1.000000000000000000, 0.000000000000000000 ) ) ;
#35706=CARTESIAN_POINT ( 'NONE',  ( 2.340729813953370519E-16, 21.32270188528330479, -43.10160580289947063 ) ) ;
#35707=CARTESIAN_POINT ( 'NONE',  ( 1.655278471875001101, 20.36702641396249547, -105.1849391362327992 ) ) ;
#35708=ADVANCED_FACE ( 'NONE', ( #18323 ), #31295, .T. ) ;
#35709=CARTESIAN_POINT ( 'NONE',  ( -1.655278471875002211, 14.63297358603754006, -29.59743913623280775 ) ) ;
#35711=CARTESIAN_POINT ( 'NONE',  ( 3.500000000000001776, 19.52072594216371826, -108.3776474690881884 ) ) ;
#35713=CARTESIAN_POINT ( 'NONE',  ( -0.9378221735089310451, 14.00000000000002309, -118.7556390011600200 ) ) ;
#35714=CARTESIAN_POINT ( 'NONE',  ( 3.500000000000001776, 19.52072594216371115, -94.07139747004407582 ) ) ;
#35718=CARTESIAN_POINT ( 'NONE',  ( 3.500000000000000000, 15.47927405783632260, -60.54431413575483134 ) ) ;
#35721=CARTESIAN_POINT ( 'NONE',  ( 1.750000000000001110, 20.53108891324555074, -48.98806413671076854 ) ) ;
#35722=CARTESIAN_POINT ( 'NONE',  ( -1.749999999999999778, 20.53108891324556140, -132.1276474690881741 ) ) ;
#35723=CARTESIAN_POINT ( 'NONE',  ( -3.310556943750000425, 19.41135094264166128, -34.93493913623279923 ) ) ;
#35726=CARTESIAN_POINT ( 'NONE',  ( -0.9378221735089310451, 14.00000000000002309, -120.7556390011600485 ) ) ;
#35730=CARTESIAN_POINT ( 'NONE',  ( 1.655278471875001101, 20.36702641396249192, -84.09743913623279354 ) ) ;
#35731=CARTESIAN_POINT ( 'NONE',  ( 0.000000000000000000, 17.50000000000002487, -149.5231586289125687 ) ) ;
#35734=CARTESIAN_POINT ( 'NONE',  ( 1.750000000000001110, 20.53108891324555429, -87.29431413575483134 ) ) ;
#35735=AXIS2_PLACEMENT_3D ( 'NONE', #21519, #11517, #27494 ) ;
#35738=CARTESIAN_POINT ( 'NONE',  ( 3.310556943750001313, 19.41135094264166483, -89.18077246956613635 ) ) ;
#35742=ADVANCED_FACE ( 'NONE', ( #215 ), #35325, .T. ) ;
#35744=CARTESIAN_POINT ( 'NONE',  ( -3.500000000000000000, 19.52072594216371115, -84.73806413671076143 ) ) ;
#35748=CARTESIAN_POINT ( 'NONE',  ( -1.655278471874999990, 20.36702641396249902, -132.9307724695661364 ) ) ;
#35751=CARTESIAN_POINT ( 'NONE',  ( 1.655278471874998436, 14.63297358603754894, -120.5182724695661278 ) ) ;
#35752=CARTESIAN_POINT ( 'NONE',  ( -3.310556943750002645, 15.58864905735836714, -44.76827246956613493 ) ) ;
#35754=ADVANCED_FACE ( 'NONE', ( #12779 ), #41932, .T. ) ;
#35755=CARTESIAN_POINT ( 'NONE',  ( -3.500000000000000888, 19.52072594216372181, -129.7380641367107614 ) ) ;
#35758=CARTESIAN_POINT ( 'NONE',  ( 1.655278471875001101, 20.36702641396248836, -74.18493913623279923 ) ) ;
#35759=CARTESIAN_POINT ( 'NONE',  ( 3.500000000000000000, 15.47927405783632970, -121.5443141357548456 ) ) ;
#35760=CARTESIAN_POINT ( 'NONE',  ( 3.310556943749999981, 15.58864905735837070, -107.3474391362327935 ) ) ;
#35761=CARTESIAN_POINT ( 'NONE',  ( 0.9378221735089281585, 14.00000000000002132, -105.6663226036830139 ) ) ;
#35763=CARTESIAN_POINT ( 'NONE',  ( -1.750000000000002220, 14.46891108675448123, -74.79431413575484555 ) ) ;
#35764=DIRECTION ( 'NONE',  ( -0.000000000000000000, 1.259100132267607459E-16, -1.000000000000000000 ) ) ;
#35765=CARTESIAN_POINT ( 'NONE',  ( 3.310556943749999981, 15.58864905735836182, -38.34743913623280775 ) ) ;
#35766=CARTESIAN_POINT ( 'NONE',  ( 3.310556943750001313, 19.41135094264166483, -95.26827246956612782 ) ) ;
#35767=CARTESIAN_POINT ( 'NONE',  ( -1.749999999999999778, 20.53108891324555074, -66.82139747004409003 ) ) ;
#35769=CARTESIAN_POINT ( 'NONE',  ( 1.655278471875001101, 20.36702641396249547, -119.1849391362327992 ) ) ;
#35770=DIRECTION ( 'NONE',  ( -0.000000000000000000, 1.259100132267607459E-16, -1.000000000000000000 ) ) ;
#35775=CARTESIAN_POINT ( 'NONE',  ( -3.310556943750002201, 15.58864905735837425, -100.6807724695661364 ) ) ;
#35778=ORIENTED_EDGE ( 'NONE', *, *, #27855, .T. ) ;
#35780=CARTESIAN_POINT ( 'NONE',  ( -0.9378221735089310451, 14.00000000000002309, -126.7556390011600200 ) ) ;
#35781=CARTESIAN_POINT ( 'NONE',  ( 0.000000000000000000, 17.50000000000002487, -149.5231586289125687 ) ) ;
#35785=CARTESIAN_POINT ( 'NONE',  ( -3.310556943750000425, 19.41135094264166128, -30.84743913623280775 ) ) ;
#35792=ORIENTED_EDGE ( 'NONE', *, *, #28978, .F. ) ;
#35795=CYLINDRICAL_SURFACE ( 'NONE', #38779, 3.499999999999999556 ) ;
#35796=CARTESIAN_POINT ( 'NONE',  ( -3.500000000000000888, 19.52072594216371826, -117.7380641367107472 ) ) ;
#35798=CARTESIAN_POINT ( 'NONE',  ( -3.310556943750001313, 17.50000000000002487, -137.8516058028994564 ) ) ;
#35799=CARTESIAN_POINT ( 'NONE',  ( 1.749999999999998224, 14.46891108675447413, -33.62764746908818125 ) ) ;
#35801=CARTESIAN_POINT ( 'NONE',  ( 0.9378221735089281585, 14.00000000000000888, -37.36007260463890844 ) ) ;
#35803=CARTESIAN_POINT ( 'NONE',  ( 1.749999999999998224, 14.46891108675448834, -139.6276474690881741 ) ) ;
#35804=CARTESIAN_POINT ( 'NONE',  ( -1.655278471874999990, 20.36702641396249547, -122.9307724695661506 ) ) ;
#35807=CARTESIAN_POINT ( 'NONE',  ( -1.394453263437886604E-15, 14.00000000000001066, -38.40473080337743284 ) ) ;
#35808=CARTESIAN_POINT ( 'NONE',  ( 3.500000000000001776, 19.52072594216371115, -90.37764746908817415 ) ) ;
#35810=CARTESIAN_POINT ( 'NONE',  ( -0.9378221735089291577, 21.00000000000001066, -37.16632260368298546 ) ) ;
#35811=CARTESIAN_POINT ( 'NONE',  ( 3.310556943750001313, 19.41135094264166128, -56.18077246956613635 ) ) ;
#35812=CARTESIAN_POINT ( 'NONE',  ( -1.655278471874999990, 20.36702641396249547, -114.0182724695661278 ) ) ;
#35814=CARTESIAN_POINT ( 'NONE',  ( -3.500000000000002220, 15.47927405783632082, -32.57139747004410424 ) ) ;
#35817=ADVANCED_FACE ( 'NONE', ( #16195 ), #3411, .T. ) ;
#35818=CARTESIAN_POINT ( 'NONE',  ( -3.310556943750002201, 15.58864905735837780, -132.7682724695661420 ) ) ;
#35822=CARTESIAN_POINT ( 'NONE',  ( -3.310556943750001313, 17.50000000000001421, -70.85160580289947063 ) ) ;
#35824=CARTESIAN_POINT ( 'NONE',  ( -7.022189441860112050E-16, 13.67729811471671830, -65.51410580289946495 ) ) ;
#35826=CARTESIAN_POINT ( 'NONE',  ( -3.310556943750000425, 19.41135094264166838, -87.93493913623279923 ) ) ;
#35828=EDGE_CURVE ( 'NONE', #10062, #19734, #39134, .T. ) ;
#35830=CARTESIAN_POINT ( 'NONE',  ( 1.655278471874998436, 14.63297358603754006, -50.43077246956613635 ) ) ;
#35832=CARTESIAN_POINT ( 'NONE',  ( -7.022189441860112050E-16, 13.67729811471672541, -106.5141058028994792 ) ) ;
#35834=( BOUNDED_CURVE ( )  B_SPLINE_CURVE ( 2, ( #16942, #3136, #29910, #6537, #29067, #13123, #28338, #34722, #17577 ),
 .UNSPECIFIED., .F., .T. ) 
 B_SPLINE_CURVE_WITH_KNOTS ( ( 3, 2, 2, 2, 3 ),
 ( 0.1104166666666666630, 0.1111111111111111049, 0.1125000000000000028, 0.1138888888888888867, 0.1145833333333333426 ),
 .UNSPECIFIED. ) 
 CURVE ( )  GEOMETRIC_REPRESENTATION_ITEM ( )  RATIONAL_B_SPLINE_CURVE ( ( 0.9330127018922194093, 0.9330127018922194093, 1.000000000000000000, 0.8660254037844387076, 1.000000000000000000, 0.8660254037844387076, 1.000000000000000000, 0.9330127018922187432, 0.9330127018922194093 ) ) 
 REPRESENTATION_ITEM ( '' )  );
#35835=VERTEX_POINT ( 'NONE', #22977 ) ;
#35838=ORIENTED_EDGE ( 'NONE', *, *, #2482, .T. ) ;
#35840=CARTESIAN_POINT ( 'NONE',  ( 1.655278471875001101, 20.36702641396248836, -57.09743913623280065 ) ) ;
#35843=DIRECTION ( 'NONE',  ( -0.000000000000000000, 1.259100132267607459E-16, -1.000000000000000000 ) ) ;
#35849=CARTESIAN_POINT ( 'NONE',  ( -1.655278471875002211, 14.63297358603755249, -125.5974391362328078 ) ) ;
#35850=CARTESIAN_POINT ( 'NONE',  ( -1.394453263437886604E-15, 14.00000000000001066, -30.71098080242150630 ) ) ;
#35852=CARTESIAN_POINT ( 'NONE',  ( 2.340729813953370519E-16, 21.32270188528330479, -35.10160580289946353 ) ) ;
#35854=CARTESIAN_POINT ( 'NONE',  ( -3.310556943750002645, 15.58864905735837247, -89.76827246956612782 ) ) ;
#35855=CARTESIAN_POINT ( 'NONE',  ( 1.655278471875001101, 20.36702641396249902, -141.0974391362327935 ) ) ;
#35857=CARTESIAN_POINT ( 'NONE',  ( 0.9378221735089300459, 21.00000000000002132, -126.9493890021159359 ) ) ;
#35859=CARTESIAN_POINT ( 'NONE',  ( -3.310556943750000425, 19.41135094264167549, -130.9349391362327992 ) ) ;
#35861=CARTESIAN_POINT ( 'NONE',  ( -3.310556943750002645, 15.58864905735837247, -93.68077246956612214 ) ) ;
#35863=CYLINDRICAL_SURFACE ( 'NONE', #6233, 3.499999999999999556 ) ;
#35864=FACE_OUTER_BOUND ( 'NONE', #26601, .T. ) ;
#35865=CARTESIAN_POINT ( 'NONE',  ( -3.500000000000001332, 17.50000000000001421, -72.65473080337743284 ) ) ;
#35866=CARTESIAN_POINT ( 'NONE',  ( 3.310556943750001313, 17.50000000000001421, -61.35160580289945642 ) ) ;
#35870=CARTESIAN_POINT ( 'NONE',  ( 3.310556943750001313, 17.50000000000001776, -86.35160580289947063 ) ) ;
#35871=CARTESIAN_POINT ( 'NONE',  ( -1.750000000000002220, 14.46891108675448123, -77.48806413671076143 ) ) ;
#35874=CARTESIAN_POINT ( 'NONE',  ( -1.655278471874999990, 20.36702641396249547, -107.9307724695661506 ) ) ;
#35875=CARTESIAN_POINT ( 'NONE',  ( 1.655278471875001101, 20.36702641396249192, -83.09743913623279354 ) ) ;
#35878=CARTESIAN_POINT ( 'NONE',  ( 1.655278471874998436, 14.63297358603754716, -102.5182724695661278 ) ) ;
#35879=CARTESIAN_POINT ( 'NONE',  ( 1.750000000000001110, 20.53108891324555785, -102.9880641367107756 ) ) ;
#35882=LINE ( 'NONE', #26746, #24758 ) ;
#35883=CARTESIAN_POINT ( 'NONE',  ( 3.500000000000000000, 15.47927405783632437, -54.23806413671076854 ) ) ;
#35884=ADVANCED_FACE ( 'NONE', ( #25345 ), #19373, .T. ) ;
#35886=CARTESIAN_POINT ( 'NONE',  ( 2.340729813953370519E-16, 21.32270188528331190, -67.01410580289947916 ) ) ;
#35888=CARTESIAN_POINT ( 'NONE',  ( -3.310556943750000425, 19.41135094264166838, -120.8474391362327935 ) ) ;
#35889=CARTESIAN_POINT ( 'NONE',  ( 3.500000000000000000, 15.47927405783632615, -71.23806413671076143 ) ) ;
#35891=CARTESIAN_POINT ( 'NONE',  ( -1.750000000000002220, 14.46891108675448834, -125.4880641367107614 ) ) ;
#35892=VERTEX_POINT ( 'NONE', #16403 ) ;
#35893=CARTESIAN_POINT ( 'NONE',  ( 0.000000000000000000, 21.00000000000002487, -149.5231586289125687 ) ) ;
#35894=CARTESIAN_POINT ( 'NONE',  ( -0.9378221735089291577, 21.00000000000001776, -90.16632260368299967 ) ) ;
#35895=CARTESIAN_POINT ( 'NONE',  ( 2.340729813953370519E-16, 21.32270188528330834, -72.01410580289947916 ) ) ;
#35897=ORIENTED_EDGE ( 'NONE', *, *, #10529, .F. ) ;
#35899=CARTESIAN_POINT ( 'NONE',  ( -3.310556943750000425, 19.41135094264167549, -140.8474391362327935 ) ) ;
#35900=EDGE_CURVE ( 'NONE', #20991, #632, #4540, .T. ) ;
#35901=CARTESIAN_POINT ( 'NONE',  ( -1.394453263437886604E-15, 14.00000000000001066, -51.40473080337743284 ) ) ;
#35902=CARTESIAN_POINT ( 'NONE',  ( 1.750000000000001110, 20.53108891324554719, -40.98806413671076143 ) ) ;
#35903=CARTESIAN_POINT ( 'NONE',  ( 1.655278471874998436, 14.63297358603754006, -45.51827246956613493 ) ) ;
#35904=CARTESIAN_POINT ( 'NONE',  ( 3.310556943750001313, 19.41135094264166483, -101.2682724695661278 ) ) ;
#35905=( BOUNDED_CURVE ( )  B_SPLINE_CURVE ( 2, ( #37250, #18512, #9529, #24487, #12117, #19305, #24279, #37660, #14902 ),
 .UNSPECIFIED., .F., .F. ) 
 B_SPLINE_CURVE_WITH_KNOTS ( ( 3, 2, 2, 2, 3 ),
 ( 0.7895833333333333037, 0.7902777777777777457, 0.7916666666666666297, 0.7930555555555555136, 0.7937499999999999556 ),
 .UNSPECIFIED. ) 
 CURVE ( )  GEOMETRIC_REPRESENTATION_ITEM ( )  RATIONAL_B_SPLINE_CURVE ( ( 0.9330127018922194093, 0.9330127018922194093, 1.000000000000000000, 0.8660254037844387076, 1.000000000000000000, 0.8660254037844387076, 1.000000000000000000, 0.9330127018922194093, 0.9330127018922194093 ) ) 
 REPRESENTATION_ITEM ( '' )  );
#35907=CARTESIAN_POINT ( 'NONE',  ( 3.310556943750001313, 17.50000000000001066, -31.26410580289946850 ) ) ;
#35909=CARTESIAN_POINT ( 'NONE',  ( -1.750000000000002220, 14.46891108675448478, -103.7943141357548456 ) ) ;
#35911=FACE_OUTER_BOUND ( 'NONE', #33060, .T. ) ;
#35912=CARTESIAN_POINT ( 'NONE',  ( 2.474675557024783212E-16, 21.54145188432739744, -93.90473080337743284 ) ) ;
#35913=LINE ( 'NONE', #25939, #34959 ) ;
#35916=CARTESIAN_POINT ( 'NONE',  ( 3.500000000000000000, 15.47927405783632082, -52.54431413575484555 ) ) ;
#35919=CARTESIAN_POINT ( 'NONE',  ( 3.500000000000001332, 17.50000000000001066, -42.15473080337743284 ) ) ;
#35921=CARTESIAN_POINT ( 'NONE',  ( -1.655278471874999990, 20.36702641396248481, -26.01827246956613138 ) ) ;
#35923=CARTESIAN_POINT ( 'NONE',  ( 0.000000000000000000, 17.50000000000002487, -149.5231586289125687 ) ) ;
#35927=CARTESIAN_POINT ( 'NONE',  ( 3.500000000000000000, 15.47927405783632970, -102.2380641367107756 ) ) ;
#35930=CARTESIAN_POINT ( 'NONE',  ( -3.310556943750001313, 17.50000000000001776, -81.76410580289947916 ) ) ;
#35933=CARTESIAN_POINT ( 'NONE',  ( 4.648177544792955347E-16, 21.00000000000001066, -33.90473080337743284 ) ) ;
#35934=CARTESIAN_POINT ( 'NONE',  ( 1.749999999999998224, 14.46891108675448301, -108.3213974700441042 ) ) ;
#35937=CARTESIAN_POINT ( 'NONE',  ( 3.310556943750001313, 19.41135094264166483, -88.18077246956613635 ) ) ;
#35938=ORIENTED_EDGE ( 'NONE', *, *, #8226, .T. ) ;
#35944=CARTESIAN_POINT ( 'NONE',  ( -4.648177544792955347E-16, 21.00000000000002487, -143.2109808024214885 ) ) ;
#35945=VECTOR ( 'NONE', #15417, 1000.000000000000000 ) ;
#35946=CARTESIAN_POINT ( 'NONE',  ( 1.655278471874998436, 14.63297358603755072, -129.4307724695661364 ) ) ;
#35947=VERTEX_POINT ( 'NONE', #22145 ) ;
#35950=CARTESIAN_POINT ( 'NONE',  ( -3.310556943750001313, 17.50000000000002132, -118.8516058028994706 ) ) ;
#35951=ORIENTED_EDGE ( 'NONE', *, *, #1948, .T. ) ;
#35952=ORIENTED_EDGE ( 'NONE', *, *, #21794, .T. ) ;
#35953=CARTESIAN_POINT ( 'NONE',  ( 2.474675557024783212E-16, 21.54145188432740810, -130.9047308033774186 ) ) ;
#35954=( BOUNDED_CURVE ( )  B_SPLINE_CURVE ( 2, ( #41113, #11961, #38124, #37915, #5588, #31529, #2396, #30009, #38961 ),
 .UNSPECIFIED., .F., .F. ) 
 B_SPLINE_CURVE_WITH_KNOTS ( ( 3, 2, 2, 2, 3 ),
 ( 0.8645833333333333703, 0.8652777777777778123, 0.8666666666666666963, 0.8680555555555555802, 0.8687500000000000222 ),
 .UNSPECIFIED. ) 
 CURVE ( )  GEOMETRIC_REPRESENTATION_ITEM ( )  RATIONAL_B_SPLINE_CURVE ( ( 0.9330127018922194093, 0.9330127018922194093, 1.000000000000000000, 0.8660254037844387076, 1.000000000000000000, 0.8660254037844387076, 1.000000000000000000, 0.9330127018922194093, 0.9330127018922194093 ) ) 
 REPRESENTATION_ITEM ( '' )  );
#35955=CARTESIAN_POINT ( 'NONE',  ( 2.340729813953370519E-16, 21.32270188528330834, -70.10160580289945642 ) ) ;
#35956=CARTESIAN_POINT ( 'NONE',  ( 1.749999999999998224, 14.46891108675448478, -117.6276474690881741 ) ) ;
#35957=CARTESIAN_POINT ( 'NONE',  ( 3.310556943750001313, 17.50000000000002132, -103.2641058028994649 ) ) ;
#35958=ADVANCED_FACE ( 'NONE', ( #28724 ), #41718, .T. ) ;
#35959=CARTESIAN_POINT ( 'NONE',  ( 0.000000000000000000, 21.00000000000002487, -149.5231586289125687 ) ) ;
#35960=CARTESIAN_POINT ( 'NONE',  ( 1.749999999999998224, 14.46891108675448301, -105.6276474690881741 ) ) ;
#35962=CARTESIAN_POINT ( 'NONE',  ( -1.750000000000002220, 14.46891108675448123, -72.79431413575483134 ) ) ;
#35964=CARTESIAN_POINT ( 'NONE',  ( -3.500000000000000000, 19.52072594216370760, -51.04431413575484555 ) ) ;
#35965=CARTESIAN_POINT ( 'NONE',  ( -1.655278471875002211, 14.63297358603754006, -36.59743913623281486 ) ) ;
#35966=CARTESIAN_POINT ( 'NONE',  ( 2.340729813953370519E-16, 21.32270188528331190, -97.10160580289947063 ) ) ;
#35967=CARTESIAN_POINT ( 'NONE',  ( -3.500000000000002220, 15.47927405783632437, -64.57139747004410424 ) ) ;
#35968=CARTESIAN_POINT ( 'NONE',  ( -3.310556943750001313, 17.50000000000002132, -115.8516058028994706 ) ) ;
#35975=CARTESIAN_POINT ( 'NONE',  ( -1.655278471874999990, 20.36702641396249192, -98.93077246956613635 ) ) ;
#35979=CARTESIAN_POINT ( 'NONE',  ( -0.9378221735089291577, 21.00000000000001066, -29.16632260368298901 ) ) ;
#35980=EDGE_LOOP ( 'NONE', ( #5772, #40762, #40509, #28923 ) ) ;
#35984=CARTESIAN_POINT ( 'NONE',  ( 3.310556943750001313, 19.41135094264166128, -28.18077246956614346 ) ) ;
#35985=ORIENTED_EDGE ( 'NONE', *, *, #41992, .T. ) ;
#35987=CARTESIAN_POINT ( 'NONE',  ( -1.750000000000002220, 14.46891108675448834, -123.4880641367107614 ) ) ;
#35988=EDGE_CURVE ( 'NONE', #38180, #40349, #20576, .T. ) ;
#35991=CARTESIAN_POINT ( 'NONE',  ( -3.500000000000001332, 17.50000000000001421, -57.96098080242151696 ) ) ;
#35993=VECTOR ( 'NONE', #30492, 1000.000000000000000 ) ;
#35995=CARTESIAN_POINT ( 'NONE',  ( -1.394453263437886604E-15, 14.00000000000002132, -114.7109808024214885 ) ) ;
#35996=CARTESIAN_POINT ( 'NONE',  ( 0.9378221735089281585, 14.00000000000000888, -31.36007260463891200 ) ) ;
#35997=CARTESIAN_POINT ( 'NONE',  ( -1.749999999999999778, 20.53108891324555785, -120.8213974700441042 ) ) ;
#35998=CARTESIAN_POINT ( 'NONE',  ( 4.286263797015737581E-16, 14.00000000000002487, -149.5231586289125687 ) ) ;
#35999=CARTESIAN_POINT ( 'NONE',  ( 1.655278471875001101, 20.36702641396249902, -134.1849391362327992 ) ) ;
#36000=CARTESIAN_POINT ( 'NONE',  ( 3.500000000000001332, 17.50000000000001066, -26.46098080242151340 ) ) ;
#36004=CARTESIAN_POINT ( 'NONE',  ( 3.500000000000000000, 15.47927405783633326, -118.5443141357548313 ) ) ;
#36006=CARTESIAN_POINT ( 'NONE',  ( 3.500000000000001332, 17.50000000000002487, -138.4609808024214885 ) ) ;
#36007=CARTESIAN_POINT ( 'NONE',  ( -3.310556943750002645, 15.58864905735837780, -117.6807724695661364 ) ) ;
#36012=CARTESIAN_POINT ( 'NONE',  ( 3.500000000000000000, 15.47927405783632615, -90.54431413575484555 ) ) ;
#36013=CARTESIAN_POINT ( 'NONE',  ( -1.750000000000002220, 14.46891108675447590, -36.79431413575484555 ) ) ;
#36014=CARTESIAN_POINT ( 'NONE',  ( -3.310556943750000425, 19.41135094264166128, -51.84743913623280775 ) ) ;
#36016=CARTESIAN_POINT ( 'NONE',  ( 1.655278471874998436, 14.63297358603754894, -111.5182724695661420 ) ) ;
#36018=CARTESIAN_POINT ( 'NONE',  ( -3.500000000000001332, 17.50000000000001066, -33.65473080337742573 ) ) ;
#36021=CARTESIAN_POINT ( 'NONE',  ( 2.340729813953370519E-16, 21.32270188528332255, -133.1016058028994564 ) ) ;
#36023=CYLINDRICAL_SURFACE ( 'NONE', #8976, 3.499999999999999556 ) ;
#36026=CARTESIAN_POINT ( 'NONE',  ( 3.310556943749999981, 15.58864905735836537, -66.43493913623279923 ) ) ;
#36028=CARTESIAN_POINT ( 'NONE',  ( 1.655278471874998436, 14.63297358603754184, -67.43077246956613635 ) ) ;
#36029=ORIENTED_EDGE ( 'NONE', *, *, #11486, .F. ) ;
#36030=CARTESIAN_POINT ( 'NONE',  ( 1.655278471874998436, 14.63297358603754539, -84.51827246956612782 ) ) ;
#36032=DIRECTION ( 'NONE',  ( -0.000000000000000000, 1.259100132267607459E-16, -1.000000000000000000 ) ) ;
#36034=CARTESIAN_POINT ( 'NONE',  ( 1.655278471874998436, 14.63297358603754006, -42.43077246956614346 ) ) ;
#36036=CARTESIAN_POINT ( 'NONE',  ( 1.655278471875001101, 20.36702641396249547, -106.0974391362328078 ) ) ;
#36037=ORIENTED_EDGE ( 'NONE', *, *, #18935, .T. ) ;
#36039=ORIENTED_EDGE ( 'NONE', *, *, #21511, .F. ) ;
#36041=CARTESIAN_POINT ( 'NONE',  ( 3.310556943750001313, 19.41135094264166128, -60.18077246956613635 ) ) ;
#36043=EDGE_LOOP ( 'NONE', ( #17019, #18311, #31608, #15241 ) ) ;
#36044=CARTESIAN_POINT ( 'NONE',  ( 0.9378221735089300459, 21.00000000000001776, -76.25563900116002003 ) ) ;
#36045=EDGE_CURVE ( 'NONE', #5763, #12942, #40149, .T. ) ;
#36049=DIRECTION ( 'NONE',  ( -0.000000000000000000, 1.259100132267607459E-16, -1.000000000000000000 ) ) ;
#36052=CARTESIAN_POINT ( 'NONE',  ( -3.500000000000000888, 19.52072594216370405, -44.04431413575483845 ) ) ;
#36053=CARTESIAN_POINT ( 'NONE',  ( -7.022189441860112050E-16, 13.67729811471671653, -44.51410580289948626 ) ) ;
#36055=DIRECTION ( 'NONE',  ( -0.000000000000000000, 1.259100132267607459E-16, -1.000000000000000000 ) ) ;
#36058=CARTESIAN_POINT ( 'NONE',  ( -1.655278471875002211, 14.63297358603754006, -32.68493913623279923 ) ) ;
#36059=CARTESIAN_POINT ( 'NONE',  ( 4.648177544792955347E-16, 21.00000000000002132, -125.9047308033774186 ) ) ;
#36061=CARTESIAN_POINT ( 'NONE',  ( 3.310556943749999981, 15.58864905735836892, -81.43493913623278502 ) ) ;
#36062=CARTESIAN_POINT ( 'NONE',  ( 3.310556943750001313, 17.50000000000002487, -136.2641058028994792 ) ) ;
#36067=CARTESIAN_POINT ( 'NONE',  ( -3.310556943750000425, 19.41135094264167549, -129.9349391362327992 ) ) ;
#36068=CARTESIAN_POINT ( 'NONE',  ( 3.500000000000001332, 17.50000000000001421, -70.15473080337743284 ) ) ;
#36069=CARTESIAN_POINT ( 'NONE',  ( -7.022189441860112050E-16, 13.67729811471672363, -89.51410580289949337 ) ) ;
#36071=CARTESIAN_POINT ( 'NONE',  ( -1.749999999999999778, 20.53108891324555785, -126.1276474690881599 ) ) ;
#36072=CARTESIAN_POINT ( 'NONE',  ( 0.000000000000000000, 17.50000000000002487, -149.5231586289125687 ) ) ;
#36073=CARTESIAN_POINT ( 'NONE',  ( 3.500000000000001776, 19.52072594216371115, -75.07139747004410424 ) ) ;
#36074=CARTESIAN_POINT ( 'NONE',  ( -7.022189441860112050E-16, 13.67729811471672186, -61.60160580289946353 ) ) ;
#36078=CARTESIAN_POINT ( 'NONE',  ( 3.310556943750001313, 19.41135094264166483, -78.26827246956612782 ) ) ;
#36079=CARTESIAN_POINT ( 'NONE',  ( 0.000000000000000000, 21.00000000000002487, -149.5231586289125687 ) ) ;
#36081=CARTESIAN_POINT ( 'NONE',  ( -7.022189441860112050E-16, 13.67729811471672896, -110.5141058028994792 ) ) ;
#36082=CARTESIAN_POINT ( 'NONE',  ( -3.310556943750000425, 19.41135094264166483, -82.84743913623279354 ) ) ;
#36084=VERTEX_POINT ( 'NONE', #24210 ) ;
#36085=CARTESIAN_POINT ( 'NONE',  ( -1.655278471874999990, 20.36702641396249192, -101.0182724695661278 ) ) ;
#36086=CARTESIAN_POINT ( 'NONE',  ( -1.749999999999999778, 20.53108891324555785, -102.8213974700440900 ) ) ;
#36090=CARTESIAN_POINT ( 'NONE',  ( 0.9378221735089300459, 21.00000000000002132, -104.9493890021159501 ) ) ;
#36092=CARTESIAN_POINT ( 'NONE',  ( 3.310556943749999981, 15.58864905735836537, -60.34743913623281486 ) ) ;
#36094=CARTESIAN_POINT ( 'NONE',  ( -3.310556943750000425, 19.41135094264166838, -121.8474391362328078 ) ) ;
#36097=ORIENTED_EDGE ( 'NONE', *, *, #9355, .F. ) ;
#36099=CARTESIAN_POINT ( 'NONE',  ( 4.648177544792955347E-16, 21.00000000000001776, -99.21098080242150274 ) ) ;
#36100=LINE ( 'NONE', #29087, #36164 ) ;
#36101=CARTESIAN_POINT ( 'NONE',  ( -3.310556943750001313, 17.50000000000001421, -73.76410580289947916 ) ) ;
#36102=ORIENTED_EDGE ( 'NONE', *, *, #41015, .T. ) ;
#36103=ORIENTED_EDGE ( 'NONE', *, *, #22058, .T. ) ;
#36107=ADVANCED_FACE ( 'NONE', ( #1445 ), #10215, .T. ) ;
#36108=CARTESIAN_POINT ( 'NONE',  ( 1.655278471875001101, 20.36702641396249902, -142.0974391362327935 ) ) ;
#36109=CARTESIAN_POINT ( 'NONE',  ( -3.500000000000001332, 17.50000000000002132, -128.9609808024215170 ) ) ;
#36112=CARTESIAN_POINT ( 'NONE',  ( -1.655278471875002211, 14.63297358603754006, -39.68493913623280633 ) ) ;
#36114=CARTESIAN_POINT ( 'NONE',  ( -1.655278471875002211, 14.63297358603754894, -102.6849391362327992 ) ) ;
#36115=CARTESIAN_POINT ( 'NONE',  ( 2.340729813953370519E-16, 21.32270188528330479, -24.01410580289947916 ) ) ;
#36117=CARTESIAN_POINT ( 'NONE',  ( 3.500000000000000000, 15.47927405783632793, -102.5443141357548598 ) ) ;
#36119=CARTESIAN_POINT ( 'NONE',  ( 4.648177544792955347E-16, 21.00000000000002132, -119.2109808024215170 ) ) ;
#36120=CARTESIAN_POINT ( 'NONE',  ( -7.424026671074350129E-16, 13.45854811567263631, -91.40473080337744705 ) ) ;
#36124=CARTESIAN_POINT ( 'NONE',  ( -3.500000000000001332, 17.50000000000001421, -54.96098080242150985 ) ) ;
#36125=CARTESIAN_POINT ( 'NONE',  ( -1.394453263437886604E-15, 14.00000000000001776, -90.40473080337741862 ) ) ;
#36126=DIRECTION ( 'NONE',  ( 0.000000000000000000, 1.000000000000000000, 0.000000000000000000 ) ) ;
#36127=VECTOR ( 'NONE', #22655, 1000.000000000000000 ) ;
#36128=CARTESIAN_POINT ( 'NONE',  ( 1.750000000000001110, 20.53108891324554719, -41.98806413671076143 ) ) ;
#36129=CARTESIAN_POINT ( 'NONE',  ( 2.340729813953370519E-16, 21.32270188528330834, -28.10160580289947418 ) ) ;
#36131=CARTESIAN_POINT ( 'NONE',  ( 4.648177544792955347E-16, 21.00000000000001776, -74.90473080337743284 ) ) ;
#36132=CARTESIAN_POINT ( 'NONE',  ( -0.9378221735089310451, 14.00000000000001599, -60.44938900211594301 ) ) ;
#36136=CARTESIAN_POINT ( 'NONE',  ( -7.022189441860112050E-16, 13.67729811471672186, -79.51410580289946495 ) ) ;
#36139=CARTESIAN_POINT ( 'NONE',  ( -3.695301148110399846E-14, 21.00000000000002132, -124.2109808024214885 ) ) ;
#36140=CARTESIAN_POINT ( 'NONE',  ( -0.9378221735089291577, 21.00000000000001421, -54.86007260463890844 ) ) ;
#36144=CARTESIAN_POINT ( 'NONE',  ( -7.022189441860112050E-16, 13.67729811471672363, -91.51410580289947916 ) ) ;
#36149=( BOUNDED_CURVE ( )  B_SPLINE_CURVE ( 2, ( #2220, #15199, #8387, #21783, #22203, #34754, #21367, #5623, #28162 ),
 .UNSPECIFIED., .F., .T. ) 
 B_SPLINE_CURVE_WITH_KNOTS ( ( 3, 2, 2, 2, 3 ),
 ( 0.6520833333333333481, 0.6527777777777777901, 0.6541666666666666741, 0.6555555555555555580, 0.6562500000000000000 ),
 .UNSPECIFIED. ) 
 CURVE ( )  GEOMETRIC_REPRESENTATION_ITEM ( )  RATIONAL_B_SPLINE_CURVE ( ( 0.9330127018922194093, 0.9330127018922194093, 1.000000000000000000, 0.8660254037844387076, 1.000000000000000000, 0.8660254037844387076, 1.000000000000000000, 0.9330127018922194093, 0.9330127018922194093 ) ) 
 REPRESENTATION_ITEM ( '' )  );
#36152=CARTESIAN_POINT ( 'NONE',  ( 3.310556943750001313, 19.41135094264166838, -128.1807724695661364 ) ) ;
#36153=ORIENTED_EDGE ( 'NONE', *, *, #27764, .T. ) ;
#36154=CARTESIAN_POINT ( 'NONE',  ( -7.022189441860112050E-16, 13.67729811471671653, -51.60160580289946353 ) ) ;
#36156=CARTESIAN_POINT ( 'NONE',  ( -3.310556943750000425, 19.41135094264166838, -118.9349391362327992 ) ) ;
#36159=CARTESIAN_POINT ( 'NONE',  ( 1.749999999999998224, 14.46891108675448656, -124.3213974700440900 ) ) ;
#36161=CARTESIAN_POINT ( 'NONE',  ( 3.310556943750001313, 17.50000000000001421, -69.35160580289947063 ) ) ;
#36162=CARTESIAN_POINT ( 'NONE',  ( -1.749999999999999778, 20.53108891324555785, -120.1276474690881741 ) ) ;
#36163=CARTESIAN_POINT ( 'NONE',  ( -1.655278471875002211, 14.63297358603754894, -99.59743913623280775 ) ) ;
#36164=VECTOR ( 'NONE', #42086, 1000.000000000000000 ) ;
#36165=DIRECTION ( 'NONE',  ( -0.000000000000000000, 1.259100132267607459E-16, -1.000000000000000000 ) ) ;
#36167=AXIS2_PLACEMENT_3D ( 'NONE', #26285, #38830, #16296 ) ;
#36169=CARTESIAN_POINT ( 'NONE',  ( -7.424026671074350129E-16, 13.45854811567263454, -70.71098080242151696 ) ) ;
#36170=CYLINDRICAL_SURFACE ( 'NONE', #19641, 3.499999999999999556 ) ;
#36171=CARTESIAN_POINT ( 'NONE',  ( -3.310556943750000425, 19.41135094264165772, -37.84743913623281486 ) ) ;
#36172=CARTESIAN_POINT ( 'NONE',  ( 1.655278471875001101, 20.36702641396249192, -94.18493913623279923 ) ) ;
#36173=CARTESIAN_POINT ( 'NONE',  ( -1.749999999999999778, 20.53108891324555074, -56.82139747004409713 ) ) ;
#36175=CARTESIAN_POINT ( 'NONE',  ( -1.655278471875002211, 14.63297358603755072, -119.6849391362327992 ) ) ;
#36177=CARTESIAN_POINT ( 'NONE',  ( -1.749999999999999778, 20.53108891324555074, -61.12764746908818125 ) ) ;
#36180=CARTESIAN_POINT ( 'NONE',  ( 0.9378221735089281585, 14.00000000000001599, -79.66632260368298546 ) ) ;
#36182=CARTESIAN_POINT ( 'NONE',  ( -1.655278471874999990, 20.36702641396249192, -95.93077246956613635 ) ) ;
#36183=CARTESIAN_POINT ( 'NONE',  ( 0.9378221735089300459, 21.00000000000001066, -38.94938900211595723 ) ) ;
#36185=ORIENTED_EDGE ( 'NONE', *, *, #32136, .F. ) ;
#36186=CARTESIAN_POINT ( 'NONE',  ( -3.500000000000001332, 17.50000000000001066, -28.96098080242151696 ) ) ;
#36187=CARTESIAN_POINT ( 'NONE',  ( 0.9378221735089300459, 21.00000000000001776, -81.25563900116002003 ) ) ;
#36188=CARTESIAN_POINT ( 'NONE',  ( -3.500000000000000000, 19.52072594216371826, -105.7380641367107614 ) ) ;
#36194=CARTESIAN_POINT ( 'NONE',  ( -1.655278471875002211, 14.63297358603754006, -28.59743913623280420 ) ) ;
#36195=ORIENTED_EDGE ( 'NONE', *, *, #33490, .F. ) ;
#36196=CARTESIAN_POINT ( 'NONE',  ( -1.749999999999999778, 20.53108891324555785, -109.8213974700441042 ) ) ;
#36203=( BOUNDED_CURVE ( )  B_SPLINE_CURVE ( 2, ( #18149, #11344, #17941, #1777, #24132, #20922, #27313, #34313, #30919 ),
 .UNSPECIFIED., .F., .T. ) 
 B_SPLINE_CURVE_WITH_KNOTS ( ( 3, 2, 2, 2, 3 ),
 ( 0.2187500000000000000, 0.2194444444444444420, 0.2208333333333333259, 0.2222222222222222099, 0.2229166666666666796 ),
 .UNSPECIFIED. ) 
 CURVE ( )  GEOMETRIC_REPRESENTATION_ITEM ( )  RATIONAL_B_SPLINE_CURVE ( ( 0.9330127018922194093, 0.9330127018922194093, 1.000000000000000000, 0.8660254037844387076, 1.000000000000000000, 0.8660254037844387076, 1.000000000000000000, 0.9330127018922180770, 0.9330127018922194093 ) ) 
 REPRESENTATION_ITEM ( '' )  );
#36205=CARTESIAN_POINT ( 'NONE',  ( 3.310556943750001313, 17.50000000000002487, -141.2641058028994792 ) ) ;
#36207=LINE ( 'NONE', #7079, #30203 ) ;
#36208=CARTESIAN_POINT ( 'NONE',  ( 3.310556943750001313, 17.50000000000002487, -137.3516058028994564 ) ) ;
#36209=CARTESIAN_POINT ( 'NONE',  ( 1.749999999999998224, 14.46891108675447413, -30.62764746908817770 ) ) ;
#36214=CARTESIAN_POINT ( 'NONE',  ( 3.500000000000001776, 19.52072594216372181, -132.3776474690881741 ) ) ;
#36215=CARTESIAN_POINT ( 'NONE',  ( -3.310556943750000425, 19.41135094264166838, -119.8474391362328078 ) ) ;
#36218=EDGE_CURVE ( 'NONE', #31404, #37593, #41619, .T. ) ;
#36219=CARTESIAN_POINT ( 'NONE',  ( 4.648177544792955347E-16, 21.00000000000002132, -128.2109808024214885 ) ) ;
#36220=CARTESIAN_POINT ( 'NONE',  ( -3.500000000000000888, 19.52072594216371115, -85.04431413575483134 ) ) ;
#36221=CARTESIAN_POINT ( 'NONE',  ( -3.500000000000002220, 15.47927405783632437, -40.87764746908817415 ) ) ;
#36222=CARTESIAN_POINT ( 'NONE',  ( -3.310556943750000425, 19.41135094264166128, -52.84743913623281486 ) ) ;
#36223=CARTESIAN_POINT ( 'NONE',  ( 3.310556943749999981, 15.58864905735837247, -110.4349391362328134 ) ) ;
#36226=CARTESIAN_POINT ( 'NONE',  ( -7.424026671074350129E-16, 13.45854811567263098, -29.40473080337743639 ) ) ;
#36227=VECTOR ( 'NONE', #23216, 1000.000000000000000 ) ;
#36230=CARTESIAN_POINT ( 'NONE',  ( 2.340729813953370519E-16, 21.32270188528332255, -136.1016058028994564 ) ) ;
#36234=CARTESIAN_POINT ( 'NONE',  ( 3.310556943750001313, 17.50000000000001421, -64.35160580289945642 ) ) ;
#36236=CARTESIAN_POINT ( 'NONE',  ( 3.310556943750001313, 19.41135094264166128, -67.18077246956613635 ) ) ;
#36238=CARTESIAN_POINT ( 'NONE',  ( -3.310556943750001313, 17.50000000000001776, -83.85160580289947063 ) ) ;
#36241=DIRECTION ( 'NONE',  ( -0.000000000000000000, 1.259100132267607459E-16, -1.000000000000000000 ) ) ;
#36244=CARTESIAN_POINT ( 'NONE',  ( -1.655278471874999990, 20.36702641396248481, -45.93077246956614346 ) ) ;
#36246=CARTESIAN_POINT ( 'NONE',  ( 1.655278471874998436, 14.63297358603754716, -102.4307724695661364 ) ) ;
#36247=LINE ( 'NONE', #33057, #14876 ) ;
#36251=VERTEX_POINT ( 'NONE', #6086 ) ;
#36253=CARTESIAN_POINT ( 'NONE',  ( -3.310556943750002645, 15.58864905735836892, -54.68077246956613635 ) ) ;
#36257=CARTESIAN_POINT ( 'NONE',  ( 3.500000000000001332, 17.50000000000001776, -76.46098080242150274 ) ) ;
#36265=CARTESIAN_POINT ( 'NONE',  ( 1.749999999999998224, 14.46891108675447590, -41.62764746908817415 ) ) ;
#36266=CARTESIAN_POINT ( 'NONE',  ( 3.310556943750001313, 17.50000000000001066, -43.26410580289947916 ) ) ;
#36267=DIRECTION ( 'NONE',  ( -0.000000000000000000, 1.259100132267607459E-16, -1.000000000000000000 ) ) ;
#36272=CARTESIAN_POINT ( 'NONE',  ( 2.340729813953370519E-16, 21.32270188528330479, -29.10160580289947063 ) ) ;
#36273=CARTESIAN_POINT ( 'NONE',  ( 4.648177544792955347E-16, 21.00000000000001421, -49.21098080242150274 ) ) ;
#36274=CARTESIAN_POINT ( 'NONE',  ( -1.655278471875002211, 14.63297358603754716, -81.68493913623279923 ) ) ;
#36275=CARTESIAN_POINT ( 'NONE',  ( -1.655278471875002211, 14.63297358603755427, -136.5974391362328220 ) ) ;
#36279=CARTESIAN_POINT ( 'NONE',  ( -3.310556943750002645, 15.58864905735837780, -129.7682724695661420 ) ) ;
#36282=CARTESIAN_POINT ( 'NONE',  ( -3.310556943750000425, 19.41135094264166483, -83.84743913623280775 ) ) ;
#36283=DIRECTION ( 'NONE',  ( -0.000000000000000000, 1.259100132267607459E-16, -1.000000000000000000 ) ) ;
#36286=CARTESIAN_POINT ( 'NONE',  ( -1.749999999999999778, 20.53108891324555429, -77.82139747004410424 ) ) ;
#36287=CARTESIAN_POINT ( 'NONE',  ( 2.340729813953370519E-16, 21.32270188528331190, -58.10160580289947063 ) ) ;
#36290=CARTESIAN_POINT ( 'NONE',  ( -1.394453263437886604E-15, 14.00000000000001776, -90.71098080242150274 ) ) ;
#36291=CARTESIAN_POINT ( 'NONE',  ( -3.310556943750001313, 17.50000000000001776, -77.85160580289945642 ) ) ;
#36292=LINE ( 'NONE', #36079, #28226 ) ;
#36294=CARTESIAN_POINT ( 'NONE',  ( 1.655278471875001101, 20.36702641396249547, -111.0974391362328078 ) ) ;
#36295=CARTESIAN_POINT ( 'NONE',  ( -7.022189441860112050E-16, 13.67729811471672363, -82.51410580289946495 ) ) ;
#36297=VERTEX_POINT ( 'NONE', #28004 ) ;
#36298=CARTESIAN_POINT ( 'NONE',  ( 1.655278471875001101, 20.36702641396249192, -100.1849391362327992 ) ) ;
#36299=CARTESIAN_POINT ( 'NONE',  ( -3.500000000000000888, 19.52072594216371826, -104.7380641367107472 ) ) ;
#36300=AXIS2_PLACEMENT_3D ( 'NONE', #20817, #11640, #8454 ) ;
#36303=CARTESIAN_POINT ( 'NONE',  ( 1.749999999999998224, 14.46891108675447590, -44.32139747004409713 ) ) ;
#36306=CARTESIAN_POINT ( 'NONE',  ( 3.310556943749999981, 15.58864905735836537, -61.34743913623281486 ) ) ;
#36307=CARTESIAN_POINT ( 'NONE',  ( 4.648177544792955347E-16, 21.00000000000001421, -59.21098080242150274 ) ) ;
#36308=CARTESIAN_POINT ( 'NONE',  ( 2.340729813953370519E-16, 21.32270188528331900, -114.0141058028994792 ) ) ;
#36309=CARTESIAN_POINT ( 'NONE',  ( -3.500000000000001332, 17.50000000000002132, -117.9609808024215170 ) ) ;
#36315=CARTESIAN_POINT ( 'NONE',  ( 0.9378221735089281585, 14.00000000000002309, -131.3600726046389013 ) ) ;
#36317=CARTESIAN_POINT ( 'NONE',  ( -7.022189441860112050E-16, 13.67729811471672186, -75.51410580289946495 ) ) ;
#36319=EDGE_LOOP ( 'NONE', ( #15025, #1640, #12065, #41554 ) ) ;
#36322=ADVANCED_FACE ( 'NONE', ( #9285 ), #21834, .T. ) ;
#36325=CARTESIAN_POINT ( 'NONE',  ( 3.310556943750001313, 17.50000000000002487, -133.2641058028994507 ) ) ;
#36326=LINE ( 'NONE', #385, #10161 ) ;
#36329=CARTESIAN_POINT ( 'NONE',  ( -3.310556943750000425, 19.41135094264165772, -38.93493913623280633 ) ) ;
#36330=CARTESIAN_POINT ( 'NONE',  ( 3.310556943749999981, 15.58864905735837070, -98.43493913623279923 ) ) ;
#36332=( BOUNDED_CURVE ( )  B_SPLINE_CURVE ( 2, ( #4897, #31256, #18497, #18714, #1710, #25096, #11685, #41259, #12104 ),
 .UNSPECIFIED., .F., .F. ) 
 B_SPLINE_CURVE_WITH_KNOTS ( ( 3, 2, 2, 2, 3 ),
 ( 0.4812500000000000111, 0.4819444444444444531, 0.4833333333333333370, 0.4847222222222222210, 0.4854166666666666630 ),
 .UNSPECIFIED. ) 
 CURVE ( )  GEOMETRIC_REPRESENTATION_ITEM ( )  RATIONAL_B_SPLINE_CURVE ( ( 0.9330127018922194093, 0.9330127018922194093, 1.000000000000000000, 0.8660254037844387076, 1.000000000000000000, 0.8660254037844387076, 1.000000000000000000, 0.9330127018922194093, 0.9330127018922194093 ) ) 
 REPRESENTATION_ITEM ( '' )  );
#36333=VECTOR ( 'NONE', #25293, 1000.000000000000000 ) ;
#36334=( BOUNDED_CURVE ( )  B_SPLINE_CURVE ( 2, ( #24873, #8690, #2525, #21663, #35067, #5506, #12522, #8905, #18696 ),
 .UNSPECIFIED., .F., .T. ) 
 B_SPLINE_CURVE_WITH_KNOTS ( ( 3, 2, 2, 2, 3 ),
 ( 0.1270833333333333259, 0.1277777777777777679, 0.1291666666666666796, 0.1305555555555555636, 0.1312500000000000056 ),
 .UNSPECIFIED. ) 
 CURVE ( )  GEOMETRIC_REPRESENTATION_ITEM ( )  RATIONAL_B_SPLINE_CURVE ( ( 0.9330127018922194093, 0.9330127018922194093, 1.000000000000000000, 0.8660254037844387076, 1.000000000000000000, 0.8660254037844387076, 1.000000000000000000, 0.9330127018922194093, 0.9330127018922194093 ) ) 
 REPRESENTATION_ITEM ( '' )  );
#36335=CARTESIAN_POINT ( 'NONE',  ( 1.655278471874998436, 14.63297358603753651, -24.43077246956613990 ) ) ;
#36336=CARTESIAN_POINT ( 'NONE',  ( 2.474675557024783212E-16, 21.54145188432739744, -100.2109808024215170 ) ) ;
#36337=DIRECTION ( 'NONE',  ( 0.000000000000000000, 1.000000000000000000, 0.000000000000000000 ) ) ;
#36338=CARTESIAN_POINT ( 'NONE',  ( 3.500000000000000000, 15.47927405783633503, -142.2380641367107614 ) ) ;
#36339=CARTESIAN_POINT ( 'NONE',  ( -7.424026671074350129E-16, 13.45854811567263631, -90.40473080337743284 ) ) ;
#36343=CARTESIAN_POINT ( 'NONE',  ( 2.474675557024783212E-16, 21.54145188432739388, -55.21098080242150274 ) ) ;
#36344=CARTESIAN_POINT ( 'NONE',  ( -1.749999999999999778, 20.53108891324555429, -89.12764746908817415 ) ) ;
#36346=EDGE_CURVE ( 'NONE', #3024, #39330, #1564, .T. ) ;
#36348=CARTESIAN_POINT ( 'NONE',  ( -3.500000000000001332, 17.50000000000001066, -45.65473080337742573 ) ) ;
#36351=CARTESIAN_POINT ( 'NONE',  ( -3.310556943750002201, 15.58864905735836537, -27.76827246956613138 ) ) ;
#36356=CARTESIAN_POINT ( 'NONE',  ( -1.749999999999999778, 20.53108891324554719, -33.82139747004410424 ) ) ;
#36358=CARTESIAN_POINT ( 'NONE',  ( 3.310556943750001313, 19.41135094264166838, -76.18077246956615056 ) ) ;
#36359=CARTESIAN_POINT ( 'NONE',  ( -3.500000000000001332, 17.50000000000002487, -141.6547308033774186 ) ) ;
#36360=VERTEX_POINT ( 'NONE', #18436 ) ;
#36361=CARTESIAN_POINT ( 'NONE',  ( -3.500000000000000000, 19.52072594216371115, -98.04431413575484555 ) ) ;
#36362=CARTESIAN_POINT ( 'NONE',  ( -1.749999999999999778, 20.53108891324554719, -45.12764746908818125 ) ) ;
#36364=VERTEX_POINT ( 'NONE', #12257 ) ;
#36367=CARTESIAN_POINT ( 'NONE',  ( -1.655278471875002211, 14.63297358603754716, -90.59743913623280775 ) ) ;
#36368=ORIENTED_EDGE ( 'NONE', *, *, #1036, .T. ) ;
#36374=DIRECTION ( 'NONE',  ( -0.000000000000000000, 1.259100132267607459E-16, -1.000000000000000000 ) ) ;
#36375=CARTESIAN_POINT ( 'NONE',  ( 1.655278471874998436, 14.63297358603755072, -128.4307724695661364 ) ) ;
#36378=CARTESIAN_POINT ( 'NONE',  ( 3.310556943749999981, 15.58864905735836537, -54.43493913623280633 ) ) ;
#36379=CARTESIAN_POINT ( 'NONE',  ( -3.310556943750000425, 19.41135094264166838, -115.9349391362327850 ) ) ;
#36382=CARTESIAN_POINT ( 'NONE',  ( 3.500000000000000000, 15.47927405783633503, -123.2380641367107614 ) ) ;
#36383=CARTESIAN_POINT ( 'NONE',  ( 1.655278471874998436, 14.63297358603754006, -40.43077246956613635 ) ) ;
#36384=CARTESIAN_POINT ( 'NONE',  ( 3.310556943750001313, 17.50000000000001421, -70.35160580289947063 ) ) ;
#36385=CARTESIAN_POINT ( 'NONE',  ( 1.750000000000001110, 20.53108891324555785, -120.2943141357548313 ) ) ;
#36386=EDGE_CURVE ( 'NONE', #20433, #19472, #12988, .T. ) ;
#36387=CARTESIAN_POINT ( 'NONE',  ( -1.655278471874999990, 20.36702641396249192, -100.9307724695661364 ) ) ;
#36389=CYLINDRICAL_SURFACE ( 'NONE', #37478, 3.499999999999999556 ) ;
#36391=CARTESIAN_POINT ( 'NONE',  ( 1.749999999999998224, 14.46891108675447768, -67.62764746908817415 ) ) ;
#36392=CARTESIAN_POINT ( 'NONE',  ( -1.394453263437886604E-15, 14.00000000000001066, -31.40473080337742573 ) ) ;
#36393=CARTESIAN_POINT ( 'NONE',  ( 3.310556943750001313, 17.50000000000001066, -35.26410580289947205 ) ) ;
#36394=CARTESIAN_POINT ( 'NONE',  ( -1.655278471874999990, 20.36702641396249192, -97.01827246956612782 ) ) ;
#36395=CARTESIAN_POINT ( 'NONE',  ( -3.500000000000000888, 19.52072594216370760, -59.73806413671075433 ) ) ;
#36397=AXIS2_PLACEMENT_3D ( 'NONE', #5981, #38518, #38729 ) ;
#36398=CARTESIAN_POINT ( 'NONE',  ( -3.310556943750000425, 19.41135094264166838, -114.9349391362327850 ) ) ;
#36399=CARTESIAN_POINT ( 'NONE',  ( -3.310556943750001313, 17.50000000000001066, -41.85160580289947063 ) ) ;
#36405=CARTESIAN_POINT ( 'NONE',  ( -3.500000000000002220, 15.47927405783632082, -23.57139747004409003 ) ) ;
#36406=CARTESIAN_POINT ( 'NONE',  ( 3.310556943750001313, 19.41135094264166838, -94.18077246956613635 ) ) ;
#36407=CARTESIAN_POINT ( 'NONE',  ( -0.9378221735089291577, 21.00000000000002487, -135.8600726046389298 ) ) ;
#36409=ORIENTED_EDGE ( 'NONE', *, *, #5668, .T. ) ;
#36412=DIRECTION ( 'NONE',  ( -0.000000000000000000, 1.259100132267607459E-16, -1.000000000000000000 ) ) ;
#36414=APPLICATION_CONTEXT ( 'automotive_design' ) ;
#36418=CARTESIAN_POINT ( 'NONE',  ( -3.310556943750000425, 19.41135094264166128, -27.84743913623280065 ) ) ;
#36419=( BOUNDED_CURVE ( )  B_SPLINE_CURVE ( 2, ( #28422, #31407, #40989, #28216, #25039, #25461, #41204, #35226, #2483 ),
 .UNSPECIFIED., .F., .T. ) 
 B_SPLINE_CURVE_WITH_KNOTS ( ( 3, 2, 2, 2, 3 ),
 ( 0.1187500000000000083, 0.1194444444444444503, 0.1208333333333333343, 0.1222222222222222182, 0.1229166666666666741 ),
 .UNSPECIFIED. ) 
 CURVE ( )  GEOMETRIC_REPRESENTATION_ITEM ( )  RATIONAL_B_SPLINE_CURVE ( ( 0.9330127018922194093, 0.9330127018922200755, 1.000000000000000000, 0.8660254037844387076, 1.000000000000000000, 0.8660254037844387076, 1.000000000000000000, 0.9330127018922187432, 0.9330127018922194093 ) ) 
 REPRESENTATION_ITEM ( '' )  );
#36425=EDGE_LOOP ( 'NONE', ( #15454, #29450, #34780, #41938 ) ) ;
#36428=CARTESIAN_POINT ( 'NONE',  ( -1.655278471874999990, 20.36702641396249902, -141.9307724695661364 ) ) ;
#36430=CARTESIAN_POINT ( 'NONE',  ( 4.648177544792955347E-16, 21.00000000000002487, -136.2109808024215170 ) ) ;
#36431=CARTESIAN_POINT ( 'NONE',  ( -1.655278471875002211, 14.63297358603755249, -135.6849391362327992 ) ) ;
#36432=CARTESIAN_POINT ( 'NONE',  ( 3.500000000000001776, 19.52072594216370405, -30.37764746908817770 ) ) ;
#36434=CARTESIAN_POINT ( 'NONE',  ( -1.394453263437886604E-15, 14.00000000000001066, -44.40473080337743284 ) ) ;
#36435=CARTESIAN_POINT ( 'NONE',  ( 1.750000000000001110, 20.53108891324554719, -42.98806413671076143 ) ) ;
#36437=CARTESIAN_POINT ( 'NONE',  ( -3.500000000000001332, 17.50000000000002487, -135.9609808024214885 ) ) ;
#36439=CARTESIAN_POINT ( 'NONE',  ( 3.310556943750001313, 19.41135094264166838, -118.1807724695661364 ) ) ;
#36443=CARTESIAN_POINT ( 'NONE',  ( 1.750000000000001110, 20.53108891324555429, -84.29431413575483134 ) ) ;
#36444=CARTESIAN_POINT ( 'NONE',  ( -1.749999999999999778, 20.53108891324555429, -92.82139747004409003 ) ) ;
#36445=CARTESIAN_POINT ( 'NONE',  ( 3.310556943750001313, 19.41135094264166128, -54.18077246956613635 ) ) ;
#36446=CARTESIAN_POINT ( 'NONE',  ( -1.655278471874999990, 20.36702641396249547, -110.0182724695661420 ) ) ;
#36448=CARTESIAN_POINT ( 'NONE',  ( 2.474675557024783212E-16, 21.54145188432739033, -29.90473080337743994 ) ) ;
#36451=CARTESIAN_POINT ( 'NONE',  ( -3.310556943750001313, 17.50000000000002132, -127.8516058028994422 ) ) ;
#36455=CARTESIAN_POINT ( 'NONE',  ( -1.655278471875002211, 14.63297358603754361, -63.68493913623279923 ) ) ;
#36457=CARTESIAN_POINT ( 'NONE',  ( -3.310556943750001313, 17.50000000000001421, -61.76410580289947205 ) ) ;
#36459=CARTESIAN_POINT ( 'NONE',  ( -3.310556943750001313, 17.50000000000001776, -84.85160580289947063 ) ) ;
#36462=CARTESIAN_POINT ( 'NONE',  ( -1.749999999999999778, 20.53108891324554719, -40.12764746908817415 ) ) ;
#36464=CARTESIAN_POINT ( 'NONE',  ( -1.655278471875002211, 14.63297358603754184, -43.59743913623280775 ) ) ;
#36466=CARTESIAN_POINT ( 'NONE',  ( -1.655278471875002211, 14.63297358603754894, -102.5974391362328220 ) ) ;
#36467=CARTESIAN_POINT ( 'NONE',  ( 3.500000000000001332, 17.50000000000001421, -53.15473080337743284 ) ) ;
#36468=( BOUNDED_CURVE ( )  B_SPLINE_CURVE ( 2, ( #22293, #3560, #15714, #23132, #35696, #9542, #35485, #16348, #36099 ),
 .UNSPECIFIED., .F., .T. ) 
 B_SPLINE_CURVE_WITH_KNOTS ( ( 3, 2, 2, 2, 3 ),
 ( 0.3645833333333333148, 0.3652777777777777568, 0.3666666666666666408, 0.3680555555555555802, 0.3687500000000000222 ),
 .UNSPECIFIED. ) 
 CURVE ( )  GEOMETRIC_REPRESENTATION_ITEM ( )  RATIONAL_B_SPLINE_CURVE ( ( 0.9330127018922194093, 0.9330127018922194093, 1.000000000000000000, 0.8660254037844387076, 1.000000000000000000, 0.8660254037844387076, 1.000000000000000000, 0.9330127018922194093, 0.9330127018922194093 ) ) 
 REPRESENTATION_ITEM ( '' )  );
#36473=CARTESIAN_POINT ( 'NONE',  ( -3.310556943750000425, 19.41135094264166128, -52.84743913623281486 ) ) ;
#36474=EDGE_LOOP ( 'NONE', ( #39443, #11259, #9687, #22931 ) ) ;
#36475=ORIENTED_EDGE ( 'NONE', *, *, #29515, .F. ) ;
#36479=CARTESIAN_POINT ( 'NONE',  ( -1.394453263437886604E-15, 14.00000000000001776, -81.40473080337743284 ) ) ;
#36480=ORIENTED_EDGE ( 'NONE', *, *, #40548, .F. ) ;
#36482=CARTESIAN_POINT ( 'NONE',  ( 3.500000000000000000, 15.47927405783632082, -44.54431413575483845 ) ) ;
#36483=CARTESIAN_POINT ( 'NONE',  ( 1.655278471874998436, 14.63297358603754006, -43.43077246956614346 ) ) ;
#36484=CARTESIAN_POINT ( 'NONE',  ( 0.9378221735089630196, 14.00000000000003730, -108.6663226036829855 ) ) ;
#36486=CARTESIAN_POINT ( 'NONE',  ( 3.500000000000001332, 19.52072594216371115, -78.07139747004410424 ) ) ;
#36488=CARTESIAN_POINT ( 'NONE',  ( 1.655278471874998436, 14.63297358603753828, -27.51827246956613138 ) ) ;
#36489=CARTESIAN_POINT ( 'NONE',  ( -7.022189441860112050E-16, 13.67729811471671297, -24.60160580289946708 ) ) ;
#36490=CARTESIAN_POINT ( 'NONE',  ( -7.022189441860112050E-16, 13.67729811471672363, -83.60160580289947063 ) ) ;
#36491=CARTESIAN_POINT ( 'NONE',  ( -3.310556943750000425, 19.41135094264167549, -133.8474391362328220 ) ) ;
#36497=CARTESIAN_POINT ( 'NONE',  ( 1.655278471874998436, 14.63297358603755072, -126.5182724695661278 ) ) ;
#36498=CARTESIAN_POINT ( 'NONE',  ( -7.022189441860112050E-16, 13.67729811471672363, -85.51410580289946495 ) ) ;
#36500=CARTESIAN_POINT ( 'NONE',  ( 0.9378221735089300459, 21.00000000000001776, -75.25563900116003424 ) ) ;
#36501=DIRECTION ( 'NONE',  ( 0.000000000000000000, 1.000000000000000000, 0.000000000000000000 ) ) ;
#36502=CARTESIAN_POINT ( 'NONE',  ( -3.500000000000000888, 19.52072594216371115, -76.73806413671076143 ) ) ;
#36504=CARTESIAN_POINT ( 'NONE',  ( -3.310556943750000425, 19.41135094264166483, -58.93493913623279212 ) ) ;
#36507=CARTESIAN_POINT ( 'NONE',  ( 3.310556943749999981, 15.58864905735836714, -77.43493913623279923 ) ) ;
#36508=CARTESIAN_POINT ( 'NONE',  ( -7.022189441860112050E-16, 13.67729811471672896, -141.6016058028994564 ) ) ;
#36510=CARTESIAN_POINT ( 'NONE',  ( 1.655278471875001101, 20.36702641396249547, -109.0974391362328078 ) ) ;
#36511=CARTESIAN_POINT ( 'NONE',  ( 3.310556943750001313, 17.50000000000001776, -77.26410580289946495 ) ) ;
#36514=CARTESIAN_POINT ( 'NONE',  ( 3.310556943749999981, 15.58864905735837070, -99.43493913623281344 ) ) ;
#36515=CARTESIAN_POINT ( 'NONE',  ( -3.500000000000002220, 15.47927405783632970, -100.5713974700441042 ) ) ;
#36517=CARTESIAN_POINT ( 'NONE',  ( 3.500000000000001332, 17.50000000000001776, -88.15473080337743284 ) ) ;
#36520=CARTESIAN_POINT ( 'NONE',  ( 1.655278471874998436, 14.63297358603754184, -61.43077246956614346 ) ) ;
#36521=CARTESIAN_POINT ( 'NONE',  ( -0.9378221735089310451, 14.00000000000002309, -112.7556390011600342 ) ) ;
#36522=CARTESIAN_POINT ( 'NONE',  ( 3.310556943750001313, 19.41135094264166838, -116.1807724695661364 ) ) ;
#36523=CARTESIAN_POINT ( 'NONE',  ( -1.750000000000002220, 14.46891108675448656, -117.7943141357548313 ) ) ;
#36526=ORIENTED_EDGE ( 'NONE', *, *, #38659, .T. ) ;
#36528=LINE ( 'NONE', #13557, #1541 ) ;
#36530=CARTESIAN_POINT ( 'NONE',  ( -1.655278471875002211, 14.63297358603754539, -67.59743913623280775 ) ) ;
#36533=EDGE_CURVE ( 'NONE', #37791, #38180, #31983, .T. ) ;
#36536=EDGE_CURVE ( 'NONE', #40297, #22963, #12895, .T. ) ;
#36538=ORIENTED_EDGE ( 'NONE', *, *, #29817, .F. ) ;
#36539=CARTESIAN_POINT ( 'NONE',  ( 2.340729813953370519E-16, 21.32270188528332255, -136.0141058028994792 ) ) ;
#36541=CARTESIAN_POINT ( 'NONE',  ( -3.310556943750002645, 15.58864905735836714, -47.76827246956612782 ) ) ;
#36542=CARTESIAN_POINT ( 'NONE',  ( 4.648177544792955347E-16, 21.00000000000002132, -111.2109808024214885 ) ) ;
#36543=CARTESIAN_POINT ( 'NONE',  ( 1.655278471875001101, 20.36702641396248481, -39.18493913623280633 ) ) ;
#36544=CARTESIAN_POINT ( 'NONE',  ( 3.310556943750001313, 19.41135094264166483, -97.26827246956612782 ) ) ;
#36546=CARTESIAN_POINT ( 'NONE',  ( -3.310556943750000425, 19.41135094264165772, -23.84743913623281486 ) ) ;
#36547=LINE ( 'NONE', #30797, #16252 ) ;
#36548=CARTESIAN_POINT ( 'NONE',  ( -3.500000000000001332, 17.50000000000002132, -103.9609808024215027 ) ) ;
#36549=CARTESIAN_POINT ( 'NONE',  ( -1.394453263437886604E-15, 14.00000000000002132, -132.7109808024214885 ) ) ;
#36550=CARTESIAN_POINT ( 'NONE',  ( 0.000000000000000000, 17.50000000000002487, -149.5231586289125687 ) ) ;
#36551=CARTESIAN_POINT ( 'NONE',  ( -3.500000000000000888, 19.52072594216371115, -89.73806413671077564 ) ) ;
#36552=EDGE_CURVE ( 'NONE', #9807, #5083, #11611, .T. ) ;
#36555=EDGE_CURVE ( 'NONE', #17584, #17606, #40446, .T. ) ;
#36557=CARTESIAN_POINT ( 'NONE',  ( 0.000000000000000000, 17.50000000000002487, -149.5231586289125687 ) ) ;
#36558=CARTESIAN_POINT ( 'NONE',  ( -7.424026671074350129E-16, 13.45854811567263454, -55.71098080242150985 ) ) ;
#36559=CARTESIAN_POINT ( 'NONE',  ( -3.500000000000001332, 17.50000000000001421, -73.96098080242151696 ) ) ;
#36560=CARTESIAN_POINT ( 'NONE',  ( 1.743066579297357930E-14, 14.00000000000002132, -134.4047308033774186 ) ) ;
#36561=EDGE_LOOP ( 'NONE', ( #41930, #40282, #1845, #16600 ) ) ;
#36562=EDGE_CURVE ( 'NONE', #12468, #33623, #10330, .T. ) ;
#36563=CARTESIAN_POINT ( 'NONE',  ( 3.500000000000001332, 17.50000000000001066, -44.15473080337743994 ) ) ;
#36565=CARTESIAN_POINT ( 'NONE',  ( -3.310556943750002201, 15.58864905735836182, -24.76827246956612782 ) ) ;
#36566=FACE_OUTER_BOUND ( 'NONE', #2947, .T. ) ;
#36569=CARTESIAN_POINT ( 'NONE',  ( -0.9378221735089291577, 21.00000000000002132, -107.1663226036829855 ) ) ;
#36571=CARTESIAN_POINT ( 'NONE',  ( -3.310556943750002201, 15.58864905735837070, -74.68077246956613635 ) ) ;
#36573=ORIENTED_EDGE ( 'NONE', *, *, #9203, .F. ) ;
#36577=CARTESIAN_POINT ( 'NONE',  ( 2.340729813953370519E-16, 21.32270188528331190, -87.01410580289947916 ) ) ;
#36579=ORIENTED_EDGE ( 'NONE', *, *, #41296, .F. ) ;
#36582=CARTESIAN_POINT ( 'NONE',  ( -1.394453263437886604E-15, 14.00000000000001421, -61.40473080337742573 ) ) ;
#36583=VECTOR ( 'NONE', #32695, 1000.000000000000000 ) ;
#36584=( BOUNDED_CURVE ( )  B_SPLINE_CURVE ( 2, ( #38173, #12013, #25005, #31163, #24798, #25425, #41166, #5219, #8616 ),
 .UNSPECIFIED., .F., .F. ) 
 B_SPLINE_CURVE_WITH_KNOTS ( ( 3, 2, 2, 2, 3 ),
 ( 0.9479166666666666297, 0.9486111111111110716, 0.9499999999999999556, 0.9513888888888888395, 0.9520833333333332815 ),
 .UNSPECIFIED. ) 
 CURVE ( )  GEOMETRIC_REPRESENTATION_ITEM ( )  RATIONAL_B_SPLINE_CURVE ( ( 0.9330127018922194093, 0.9330127018922194093, 1.000000000000000000, 0.8660254037844387076, 1.000000000000000000, 0.8660254037844387076, 1.000000000000000000, 0.9330127018922194093, 0.9330127018922194093 ) ) 
 REPRESENTATION_ITEM ( '' )  );
#36585=ADVANCED_FACE ( 'NONE', ( #9712 ), #22673, .T. ) ;
#36586=CARTESIAN_POINT ( 'NONE',  ( -3.310556943750001313, 17.50000000000002132, -124.7641058028994649 ) ) ;
#36587=( BOUNDED_CURVE ( )  B_SPLINE_CURVE ( 2, ( #22370, #16212, #10404, #9406, #19186, #41952, #2814, #28543, #18771 ),
 .UNSPECIFIED., .F., .F. ) 
 B_SPLINE_CURVE_WITH_KNOTS ( ( 3, 2, 2, 2, 3 ),
 ( 0.5812500000000000444, 0.5819444444444444864, 0.5833333333333333703, 0.5847222222222222543, 0.5854166666666666963 ),
 .UNSPECIFIED. ) 
 CURVE ( )  GEOMETRIC_REPRESENTATION_ITEM ( )  RATIONAL_B_SPLINE_CURVE ( ( 0.9330127018922194093, 0.9330127018922194093, 1.000000000000000000, 0.8660254037844387076, 1.000000000000000000, 0.8660254037844387076, 1.000000000000000000, 0.9330127018922194093, 0.9330127018922194093 ) ) 
 REPRESENTATION_ITEM ( '' )  );
#36588=EDGE_CURVE ( 'NONE', #10316, #11709, #37952, .T. ) ;
#36591=CARTESIAN_POINT ( 'NONE',  ( 3.310556943749999981, 15.58864905735836182, -53.43493913623279923 ) ) ;
#36592=CARTESIAN_POINT ( 'NONE',  ( -3.310556943750001313, 17.50000000000002132, -112.8516058028994564 ) ) ;
#36593=ORIENTED_EDGE ( 'NONE', *, *, #28007, .T. ) ;
#36594=VERTEX_POINT ( 'NONE', #39670 ) ;
#36595=CARTESIAN_POINT ( 'NONE',  ( -1.749999999999999778, 20.53108891324555785, -124.8213974700440900 ) ) ;
#36596=CARTESIAN_POINT ( 'NONE',  ( 3.310556943749999981, 15.58864905735836182, -39.34743913623282197 ) ) ;
#36597=CARTESIAN_POINT ( 'NONE',  ( 1.655278471875001101, 20.36702641396248836, -66.18493913623279923 ) ) ;
#36598=CARTESIAN_POINT ( 'NONE',  ( -3.500000000000001332, 17.50000000000002132, -119.9609808024215170 ) ) ;
#36599=CARTESIAN_POINT ( 'NONE',  ( -1.655278471874999990, 20.36702641396249547, -102.9307724695661364 ) ) ;
#36600=ADVANCED_FACE ( 'NONE', ( #38253 ), #28672, .T. ) ;
#36605=CARTESIAN_POINT ( 'NONE',  ( -1.749999999999999778, 20.53108891324555074, -71.12764746908817415 ) ) ;
#36607=CARTESIAN_POINT ( 'NONE',  ( 3.310556943750001313, 17.50000000000001066, -37.26410580289947205 ) ) ;
#36608=CARTESIAN_POINT ( 'NONE',  ( -3.310556943750001313, 17.50000000000001776, -95.85160580289945642 ) ) ;
#36610=CARTESIAN_POINT ( 'NONE',  ( -1.749999999999999778, 20.53108891324555074, -57.82139747004409713 ) ) ;
#36612=CARTESIAN_POINT ( 'NONE',  ( -3.310556943750002201, 15.58864905735837780, -112.7682724695661278 ) ) ;
#36613=CARTESIAN_POINT ( 'NONE',  ( 2.340729813953370519E-16, 21.32270188528330834, -41.10160580289946353 ) ) ;
#36619=CARTESIAN_POINT ( 'NONE',  ( 1.749999999999998224, 14.46891108675447768, -61.62764746908818125 ) ) ;
#36620=CARTESIAN_POINT ( 'NONE',  ( 1.655278471874998436, 14.63297358603754539, -94.43077246956613635 ) ) ;
#36621=DIRECTION ( 'NONE',  ( -0.000000000000000000, -0.000000000000000000, -1.000000000000000000 ) ) ;
#36623=VECTOR ( 'NONE', #13773, 1000.000000000000000 ) ;
#36624=ORIENTED_EDGE ( 'NONE', *, *, #23407, .F. ) ;
#36627=CARTESIAN_POINT ( 'NONE',  ( 0.000000000000000000, 17.50000000000002487, -149.5231586289125687 ) ) ;
#36632=CARTESIAN_POINT ( 'NONE',  ( 1.655278471875001101, 20.36702641396248481, -31.09743913623280775 ) ) ;
#36638=ORIENTED_EDGE ( 'NONE', *, *, #12982, .T. ) ;
#36641=CARTESIAN_POINT ( 'NONE',  ( 0.9378221735089260491, 21.00000000000002842, -136.9493890021159928 ) ) ;
#36642=CARTESIAN_POINT ( 'NONE',  ( -0.9378221735089310451, 14.00000000000001599, -80.75563900116002003 ) ) ;
#36643=CARTESIAN_POINT ( 'NONE',  ( -1.750000000000002220, 14.46891108675448834, -135.7943141357548598 ) ) ;
#36644=CARTESIAN_POINT ( 'NONE',  ( 2.340729813953370519E-16, 21.32270188528331900, -129.1016058028994848 ) ) ;
#36645=CARTESIAN_POINT ( 'NONE',  ( 3.500000000000000000, 15.47927405783632082, -27.54431413575483489 ) ) ;
#36648=CARTESIAN_POINT ( 'NONE',  ( 4.648177544792955347E-16, 21.00000000000002132, -126.9047308033774186 ) ) ;
#36649=VECTOR ( 'NONE', #38504, 1000.000000000000000 ) ;
#36650=DIRECTION ( 'NONE',  ( 1.000000000000000000, 0.000000000000000000, 0.000000000000000000 ) ) ;
#36652=CARTESIAN_POINT ( 'NONE',  ( 1.749999999999998224, 14.46891108675448656, -135.6276474690881741 ) ) ;
#36653=CARTESIAN_POINT ( 'NONE',  ( 3.310556943750001313, 19.41135094264166838, -116.1807724695661364 ) ) ;
#36656=DIRECTION ( 'NONE',  ( 0.000000000000000000, 1.000000000000000000, 0.000000000000000000 ) ) ;
#36657=CARTESIAN_POINT ( 'NONE',  ( 3.500000000000001776, 19.52072594216371115, -83.37764746908818836 ) ) ;
#36659=CARTESIAN_POINT ( 'NONE',  ( 3.310556943749999981, 15.58864905735836182, -51.34743913623281486 ) ) ;
#36660=CARTESIAN_POINT ( 'NONE',  ( 3.310556943750001313, 19.41135094264166838, -111.2682724695661278 ) ) ;
#36661=CARTESIAN_POINT ( 'NONE',  ( -1.750000000000002220, 14.46891108675448301, -93.79431413575484555 ) ) ;
#36664=CARTESIAN_POINT ( 'NONE',  ( -3.310556943750002201, 15.58864905735837780, -127.7682724695661278 ) ) ;
#36667=CARTESIAN_POINT ( 'NONE',  ( 4.286263797015737581E-16, 14.00000000000002487, -149.5231586289125687 ) ) ;
#36668=( BOUNDED_CURVE ( )  B_SPLINE_CURVE ( 2, ( #2156, #11519, #5148, #41090, #31712, #21314, #14524, #12145, #21931 ),
 .UNSPECIFIED., .F., .T. ) 
 B_SPLINE_CURVE_WITH_KNOTS ( ( 3, 2, 2, 2, 3 ),
 ( 0.8729166666666666741, 0.8736111111111111160, 0.8750000000000000000, 0.8763888888888888840, 0.8770833333333333259 ),
 .UNSPECIFIED. ) 
 CURVE ( )  GEOMETRIC_REPRESENTATION_ITEM ( )  RATIONAL_B_SPLINE_CURVE ( ( 0.9330127018922194093, 0.9330127018922194093, 1.000000000000000000, 0.8660254037844387076, 1.000000000000000000, 0.8660254037844387076, 1.000000000000000000, 0.9330127018922194093, 0.9330127018922194093 ) ) 
 REPRESENTATION_ITEM ( '' )  );
#36669=CARTESIAN_POINT ( 'NONE',  ( -3.310556943750002645, 15.58864905735836892, -63.76827246956614204 ) ) ;
#36671=VERTEX_POINT ( 'NONE', #41243 ) ;
#36672=CARTESIAN_POINT ( 'NONE',  ( -3.310556943750001313, 17.50000000000001776, -78.85160580289945642 ) ) ;
#36676=CARTESIAN_POINT ( 'NONE',  ( -7.022189441860112050E-16, 13.67729811471671830, -45.51410580289946495 ) ) ;
#36677=CARTESIAN_POINT ( 'NONE',  ( 1.655278471875001101, 20.36702641396249547, -102.0974391362328220 ) ) ;
#36681=ORIENTED_EDGE ( 'NONE', *, *, #38846, .T. ) ;
#36684=CARTESIAN_POINT ( 'NONE',  ( -1.655278471875002211, 14.63297358603754184, -53.59743913623281486 ) ) ;
#36686=ORIENTED_EDGE ( 'NONE', *, *, #36045, .T. ) ;
#36687=ADVANCED_FACE ( 'NONE', ( #31658 ), #34434, .T. ) ;
#36688=CARTESIAN_POINT ( 'NONE',  ( 0.000000000000000000, 17.50000000000002487, -149.5231586289125687 ) ) ;
#36689=AXIS2_PLACEMENT_3D ( 'NONE', #25339, #22140, #28719 ) ;
#36694=CARTESIAN_POINT ( 'NONE',  ( -7.424026671074350129E-16, 13.45854811567263276, -42.71098080242150985 ) ) ;
#36695=CARTESIAN_POINT ( 'NONE',  ( 4.648177544792955347E-16, 21.00000000000001776, -96.90473080337741862 ) ) ;
#36696=CARTESIAN_POINT ( 'NONE',  ( 0.000000000000000000, 17.50000000000002487, -149.5231586289125687 ) ) ;
#36698=CARTESIAN_POINT ( 'NONE',  ( -1.655278471874999990, 20.36702641396248481, -29.01827246956613493 ) ) ;
#36699=CARTESIAN_POINT ( 'NONE',  ( -3.500000000000002220, 15.47927405783633326, -97.57139747004409003 ) ) ;
#36700=CARTESIAN_POINT ( 'NONE',  ( 3.310556943750001313, 19.41135094264166483, -81.26827246956612782 ) ) ;
#36701=CARTESIAN_POINT ( 'NONE',  ( -7.022189441860112050E-16, 13.67729811471672896, -136.5141058028994792 ) ) ;
#36705=CARTESIAN_POINT ( 'NONE',  ( -1.394453263437886604E-15, 14.00000000000000711, -24.40473080337742928 ) ) ;
#36707=CARTESIAN_POINT ( 'NONE',  ( -1.655278471874999990, 20.36702641396249547, -129.0182724695661136 ) ) ;
#36709=CARTESIAN_POINT ( 'NONE',  ( -7.022189441860112050E-16, 13.67729811471672363, -86.51410580289947916 ) ) ;
#36710=CYLINDRICAL_SURFACE ( 'NONE', #33511, 3.499999999999999556 ) ;
#36712=CARTESIAN_POINT ( 'NONE',  ( 3.500000000000001332, 19.52072594216370405, -25.07139747004409713 ) ) ;
#36713=CARTESIAN_POINT ( 'NONE',  ( 1.749999999999998224, 14.46891108675447946, -69.32139747004409003 ) ) ;
#36714=CARTESIAN_POINT ( 'NONE',  ( 1.655278471874998436, 14.63297358603754006, -53.51827246956612782 ) ) ;
#36717=CARTESIAN_POINT ( 'NONE',  ( 3.310556943749999981, 15.58864905735836714, -79.43493913623279923 ) ) ;
#36718=CARTESIAN_POINT ( 'NONE',  ( 1.655278471874998436, 14.63297358603755249, -139.5182724695661420 ) ) ;
#36720=CARTESIAN_POINT ( 'NONE',  ( -1.655278471874999990, 20.36702641396249547, -109.9307724695661506 ) ) ;
#36721=CARTESIAN_POINT ( 'NONE',  ( 2.340729813953370519E-16, 21.32270188528330834, -74.01410580289947916 ) ) ;
#36722=DIRECTION ( 'NONE',  ( -0.000000000000000000, 1.259100132267607459E-16, -1.000000000000000000 ) ) ;
#36724=( BOUNDED_CURVE ( )  B_SPLINE_CURVE ( 2, ( #17583, #2405, #26950, #36943, #10774, #7805, #1416, #14390, #27927 ),
 .UNSPECIFIED., .F., .T. ) 
 B_SPLINE_CURVE_WITH_KNOTS ( ( 3, 2, 2, 2, 3 ),
 ( 0.2270833333333333315, 0.2277777777777777735, 0.2291666666666666574, 0.2305555555555555691, 0.2312500000000000111 ),
 .UNSPECIFIED. ) 
 CURVE ( )  GEOMETRIC_REPRESENTATION_ITEM ( )  RATIONAL_B_SPLINE_CURVE ( ( 0.9330127018922194093, 0.9330127018922194093, 1.000000000000000000, 0.8660254037844387076, 1.000000000000000000, 0.8660254037844387076, 1.000000000000000000, 0.9330127018922194093, 0.9330127018922194093 ) ) 
 REPRESENTATION_ITEM ( '' )  );
#36726=CARTESIAN_POINT ( 'NONE',  ( -7.022189441860112050E-16, 13.67729811471672541, -97.60160580289945642 ) ) ;
#36727=CARTESIAN_POINT ( 'NONE',  ( -3.500000000000002220, 15.47927405783632970, -101.5713974700440900 ) ) ;
#36729=CARTESIAN_POINT ( 'NONE',  ( -1.749999999999999778, 20.53108891324554719, -33.12764746908818125 ) ) ;
#36730=CARTESIAN_POINT ( 'NONE',  ( -1.749999999999999778, 20.53108891324555074, -52.12764746908816704 ) ) ;
#36732=CARTESIAN_POINT ( 'NONE',  ( -3.310556943750000425, 19.41135094264166483, -61.84743913623281486 ) ) ;
#36734=CARTESIAN_POINT ( 'NONE',  ( -7.022189441860112050E-16, 13.67729811471672718, -117.5141058028994792 ) ) ;
#36737=EDGE_LOOP ( 'NONE', ( #41508, #33397, #12250, #6112 ) ) ;
#36742=CARTESIAN_POINT ( 'NONE',  ( -3.310556943750000425, 19.41135094264166128, -69.84743913623280775 ) ) ;
#36743=ORIENTED_EDGE ( 'NONE', *, *, #9774, .F. ) ;
#36744=ORIENTED_EDGE ( 'NONE', *, *, #31160, .T. ) ;
#36747=CARTESIAN_POINT ( 'NONE',  ( 3.500000000000001332, 19.52072594216371115, -83.37764746908818836 ) ) ;
#36751=EDGE_CURVE ( 'NONE', #30038, #3213, #36334, .T. ) ;
#36753=CARTESIAN_POINT ( 'NONE',  ( 3.310556943749999981, 15.58864905735837425, -134.3474391362328220 ) ) ;
#36756=CARTESIAN_POINT ( 'NONE',  ( 2.340729813953370519E-16, 21.32270188528330479, -45.10160580289947063 ) ) ;
#36758=CARTESIAN_POINT ( 'NONE',  ( 1.655278471874998436, 14.63297358603754006, -40.51827246956612782 ) ) ;
#36759=CARTESIAN_POINT ( 'NONE',  ( -1.655278471874999990, 20.36702641396249192, -99.01827246956612782 ) ) ;
#36761=CARTESIAN_POINT ( 'NONE',  ( 3.310556943749999981, 15.58864905735836004, -25.34743913623280420 ) ) ;
#36763=CARTESIAN_POINT ( 'NONE',  ( 3.500000000000001776, 19.52072594216371115, -100.3776474690881741 ) ) ;
#36766=CARTESIAN_POINT ( 'NONE',  ( -1.749999999999999778, 20.53108891324555429, -83.82139747004410424 ) ) ;
#36767=CARTESIAN_POINT ( 'NONE',  ( 1.655278471875001101, 20.36702641396248836, -70.18493913623279923 ) ) ;
#36772=CARTESIAN_POINT ( 'NONE',  ( 3.500000000000001332, 19.52072594216371826, -110.3776474690881741 ) ) ;
#36773=CARTESIAN_POINT ( 'NONE',  ( -3.500000000000002220, 15.47927405783632437, -55.87764746908817415 ) ) ;
#36774=AXIS2_PLACEMENT_3D ( 'NONE', #31747, #2618, #37513 ) ;
#36775=CYLINDRICAL_SURFACE ( 'NONE', #28395, 3.499999999999999556 ) ;
#36779=EDGE_CURVE ( 'NONE', #17107, #28825, #37709, .T. ) ;
#36780=CARTESIAN_POINT ( 'NONE',  ( 2.474675557024783212E-16, 21.54145188432739033, -42.90473080337743994 ) ) ;
#36782=CARTESIAN_POINT ( 'NONE',  ( -3.310556943750002201, 15.58864905735836537, -26.76827246956613493 ) ) ;
#36783=CARTESIAN_POINT ( 'NONE',  ( -1.394453263437886604E-15, 14.00000000000001776, -83.40473080337743284 ) ) ;
#36786=DIRECTION ( 'NONE',  ( -0.000000000000000000, 1.259100132267607459E-16, -1.000000000000000000 ) ) ;
#36788=CARTESIAN_POINT ( 'NONE',  ( 1.655278471874998436, 14.63297358603754361, -79.43077246956615056 ) ) ;
#36789=CARTESIAN_POINT ( 'NONE',  ( -1.750000000000002220, 14.46891108675448834, -133.7943141357548598 ) ) ;
#36793=CARTESIAN_POINT ( 'NONE',  ( 0.9378221735089300459, 21.00000000000001776, -89.94938900211595012 ) ) ;
#36796=CARTESIAN_POINT ( 'NONE',  ( 1.655278471874998436, 14.63297358603754539, -83.43077246956615056 ) ) ;
#36799=EDGE_LOOP ( 'NONE', ( #13404, #6816, #28518, #7275 ) ) ;
#36802=EDGE_CURVE ( 'NONE', #33769, #15570, #20314, .T. ) ;
#36806=CARTESIAN_POINT ( 'NONE',  ( -3.310556943750001313, 17.50000000000002132, -127.7641058028994792 ) ) ;
#36808=CARTESIAN_POINT ( 'NONE',  ( 3.310556943750001313, 17.50000000000001421, -55.35160580289947063 ) ) ;
#36809=CARTESIAN_POINT ( 'NONE',  ( 3.310556943750001313, 19.41135094264166838, -112.2682724695661420 ) ) ;
#36811=ORIENTED_EDGE ( 'NONE', *, *, #29239, .T. ) ;
#36812=CARTESIAN_POINT ( 'NONE',  ( 3.500000000000000000, 15.47927405783633503, -127.2380641367107756 ) ) ;
#36814=CARTESIAN_POINT ( 'NONE',  ( 1.655278471875001101, 20.36702641396248481, -38.09743913623281486 ) ) ;
#36815=CARTESIAN_POINT ( 'NONE',  ( -3.310556943750000425, 19.41135094264166128, -66.93493913623279923 ) ) ;
#36816=CARTESIAN_POINT ( 'NONE',  ( 3.500000000000000000, 15.47927405783632970, -119.5443141357548313 ) ) ;
#36817=CARTESIAN_POINT ( 'NONE',  ( 2.340729813953370519E-16, 21.32270188528331190, -95.01410580289946495 ) ) ;
#36818=DIRECTION ( 'NONE',  ( -0.000000000000000000, 1.259100132267607459E-16, -1.000000000000000000 ) ) ;
#36822=CARTESIAN_POINT ( 'NONE',  ( 1.750000000000001110, 20.53108891324555074, -72.29431413575483134 ) ) ;
#36823=CARTESIAN_POINT ( 'NONE',  ( 4.648177544792955347E-16, 21.00000000000001776, -100.2109808024215027 ) ) ;
#36824=CARTESIAN_POINT ( 'NONE',  ( -1.655278471874999990, 20.36702641396248481, -32.93077246956614346 ) ) ;
#36825=CARTESIAN_POINT ( 'NONE',  ( 1.655278471875001101, 20.36702641396249192, -92.18493913623279923 ) ) ;
#36826=CARTESIAN_POINT ( 'NONE',  ( -3.500000000000000888, 19.52072594216370760, -61.73806413671076143 ) ) ;
#36827=CARTESIAN_POINT ( 'NONE',  ( -1.750000000000002220, 14.46891108675449011, -137.7943141357548598 ) ) ;
#36828=CARTESIAN_POINT ( 'NONE',  ( -7.022189441860112050E-16, 13.67729811471672896, -112.6016058028994564 ) ) ;
#36829=CARTESIAN_POINT ( 'NONE',  ( -1.655278471875002211, 14.63297358603754184, -42.68493913623279212 ) ) ;
#36831=CARTESIAN_POINT ( 'NONE',  ( -1.749999999999999778, 20.53108891324555074, -62.82139747004410424 ) ) ;
#36836=CARTESIAN_POINT ( 'NONE',  ( -3.500000000000000000, 19.52072594216370405, -23.73806413671077209 ) ) ;
#36837=CARTESIAN_POINT ( 'NONE',  ( 3.310556943750001313, 17.50000000000001776, -91.26410580289947916 ) ) ;
#36839=VERTEX_POINT ( 'NONE', #39289 ) ;
#36840=CARTESIAN_POINT ( 'NONE',  ( 0.000000000000000000, 17.50000000000002487, -149.5231586289125687 ) ) ;
#36842=CARTESIAN_POINT ( 'NONE',  ( -3.500000000000002220, 15.47927405783632793, -78.87764746908817415 ) ) ;
#36846=CARTESIAN_POINT ( 'NONE',  ( 1.750000000000001110, 20.53108891324555074, -73.98806413671076143 ) ) ;
#36849=ORIENTED_EDGE ( 'NONE', *, *, #5392, .T. ) ;
#36850=CARTESIAN_POINT ( 'NONE',  ( 0.000000000000000000, 17.50000000000002487, -149.5231586289125687 ) ) ;
#36851=( BOUNDED_CURVE ( )  B_SPLINE_CURVE ( 2, ( #4568, #30727, #20742, #40086, #40300, #4982, #1174, #27546, #964 ),
 .UNSPECIFIED., .F., .F. ) 
 B_SPLINE_CURVE_WITH_KNOTS ( ( 3, 2, 2, 2, 3 ),
 ( 0.8270833333333332815, 0.8277777777777777235, 0.8291666666666667185, 0.8305555555555556024, 0.8312500000000000444 ),
 .UNSPECIFIED. ) 
 CURVE ( )  GEOMETRIC_REPRESENTATION_ITEM ( )  RATIONAL_B_SPLINE_CURVE ( ( 0.9330127018922194093, 0.9330127018922194093, 1.000000000000000000, 0.8660254037844387076, 1.000000000000000000, 0.8660254037844387076, 1.000000000000000000, 0.9330127018922194093, 0.9330127018922194093 ) ) 
 REPRESENTATION_ITEM ( '' )  );
#36857=CARTESIAN_POINT ( 'NONE',  ( -1.749999999999999778, 20.53108891324554719, -27.82139747004409713 ) ) ;
#36860=CARTESIAN_POINT ( 'NONE',  ( -3.310556943750002645, 15.58864905735837958, -141.6807724695661648 ) ) ;
#36862=CARTESIAN_POINT ( 'NONE',  ( 3.500000000000000000, 15.47927405783633326, -110.2380641367107614 ) ) ;
#36864=CARTESIAN_POINT ( 'NONE',  ( -3.500000000000000000, 19.52072594216371115, -75.04431413575485976 ) ) ;
#36865=CARTESIAN_POINT ( 'NONE',  ( -3.310556943750001313, 17.50000000000002487, -129.8516058028994564 ) ) ;
#36866=CARTESIAN_POINT ( 'NONE',  ( -1.750000000000002220, 14.46891108675447590, -26.79431413575483845 ) ) ;
#36868=CARTESIAN_POINT ( 'NONE',  ( -3.500000000000002220, 15.47927405783633503, -139.5713974700441042 ) ) ;
#36870=CARTESIAN_POINT ( 'NONE',  ( -1.750000000000002220, 14.46891108675448834, -135.7943141357548598 ) ) ;
#36871=CARTESIAN_POINT ( 'NONE',  ( -7.022189441860112050E-16, 13.67729811471672718, -115.5141058028994792 ) ) ;
#36873=DIRECTION ( 'NONE',  ( -0.000000000000000000, 1.259100132267607459E-16, -1.000000000000000000 ) ) ;
#36874=CARTESIAN_POINT ( 'NONE',  ( 2.474675557024783212E-16, 21.54145188432739744, -83.21098080242151696 ) ) ;
#36875=CARTESIAN_POINT ( 'NONE',  ( 4.648177544792955347E-16, 21.00000000000001421, -69.90473080337741862 ) ) ;
#36876=CARTESIAN_POINT ( 'NONE',  ( -3.310556943750001313, 17.50000000000001421, -54.76410580289947916 ) ) ;
#36877=CARTESIAN_POINT ( 'NONE',  ( 1.655278471875001101, 20.36702641396249547, -105.1849391362327992 ) ) ;
#36879=CYLINDRICAL_SURFACE ( 'NONE', #29361, 3.499999999999999556 ) ;
#36881=CARTESIAN_POINT ( 'NONE',  ( -3.310556943750002201, 15.58864905735837780, -128.7682724695661136 ) ) ;
#36885=CARTESIAN_POINT ( 'NONE',  ( 0.000000000000000000, 21.00000000000002487, -149.5231586289125687 ) ) ;
#36886=CARTESIAN_POINT ( 'NONE',  ( 3.310556943749999981, 15.58864905735836537, -63.43493913623279923 ) ) ;
#36887=ORIENTED_EDGE ( 'NONE', *, *, #9903, .F. ) ;
#36888=CARTESIAN_POINT ( 'NONE',  ( -3.310556943750002201, 15.58864905735837070, -80.76827246956612782 ) ) ;
#36889=ADVANCED_FACE ( 'NONE', ( #4207 ), #33339, .T. ) ;
#36892=ADVANCED_FACE ( 'NONE', ( #39935 ), #39725, .T. ) ;
#36895=CARTESIAN_POINT ( 'NONE',  ( 3.310556943750001313, 17.50000000000001066, -39.26410580289947916 ) ) ;
#36896=AXIS2_PLACEMENT_3D ( 'NONE', #41931, #6808, #6188 ) ;
#36897=CARTESIAN_POINT ( 'NONE',  ( 3.310556943750001313, 19.41135094264166838, -102.1807724695661364 ) ) ;
#36899=ORIENTED_EDGE ( 'NONE', *, *, #37381, .F. ) ;
#36901=VERTEX_POINT ( 'NONE', #20372 ) ;
#36903=EDGE_CURVE ( 'NONE', #27997, #31100, #23998, .T. ) ;
#36904=CARTESIAN_POINT ( 'NONE',  ( 1.655278471875001101, 20.36702641396248836, -51.09743913623280775 ) ) ;
#36906=VERTEX_POINT ( 'NONE', #33561 ) ;
#36910=CARTESIAN_POINT ( 'NONE',  ( 3.500000000000001332, 19.52072594216371826, -113.3776474690881741 ) ) ;
#36912=CARTESIAN_POINT ( 'NONE',  ( -3.500000000000001332, 17.50000000000001066, -43.96098080242151696 ) ) ;
#36913=CARTESIAN_POINT ( 'NONE',  ( -1.394453263437886604E-15, 14.00000000000001421, -68.40473080337741862 ) ) ;
#36914=CARTESIAN_POINT ( 'NONE',  ( 4.648177544792955347E-16, 21.00000000000002132, -110.9047308033774186 ) ) ;
#36916=CARTESIAN_POINT ( 'NONE',  ( -3.310556943750001313, 17.50000000000001066, -29.85160580289947063 ) ) ;
#36917=CARTESIAN_POINT ( 'NONE',  ( -3.500000000000002220, 15.47927405783633326, -106.5713974700441042 ) ) ;
#36918=AXIS2_PLACEMENT_3D ( 'NONE', #19448, #18818, #6051 ) ;
#36919=CARTESIAN_POINT ( 'NONE',  ( 3.310556943750001313, 17.50000000000001776, -81.35160580289945642 ) ) ;
#36920=CARTESIAN_POINT ( 'NONE',  ( -1.655278471874999990, 20.36702641396249902, -131.9307724695661364 ) ) ;
#36923=AXIS2_PLACEMENT_3D ( 'NONE', #26588, #29337, #9803 ) ;
#36924=CARTESIAN_POINT ( 'NONE',  ( -1.749999999999999778, 20.53108891324554719, -38.82139747004409713 ) ) ;
#36925=CARTESIAN_POINT ( 'NONE',  ( -1.655278471874999990, 20.36702641396249547, -127.0182724695661278 ) ) ;
#36926=CARTESIAN_POINT ( 'NONE',  ( 3.500000000000001332, 17.50000000000001066, -42.46098080242151696 ) ) ;
#36927=CARTESIAN_POINT ( 'NONE',  ( -3.310556943750002645, 15.58864905735837247, -84.68077246956613635 ) ) ;
#36930=CARTESIAN_POINT ( 'NONE',  ( 0.000000000000000000, 17.49999999999990052, 850.4768413710875166 ) ) ;
#36931=CARTESIAN_POINT ( 'NONE',  ( 3.500000000000001332, 17.50000000000001421, -67.15473080337743284 ) ) ;
#36933=CARTESIAN_POINT ( 'NONE',  ( 3.500000000000001332, 17.50000000000001421, -70.15473080337743284 ) ) ;
#36934=CARTESIAN_POINT ( 'NONE',  ( 1.655278471875001101, 20.36702641396248836, -54.18493913623280633 ) ) ;
#36936=CARTESIAN_POINT ( 'NONE',  ( -3.500000000000001332, 17.50000000000001421, -67.65473080337743284 ) ) ;
#36938=CARTESIAN_POINT ( 'NONE',  ( -3.310556943750002645, 15.58864905735837070, -80.76827246956612782 ) ) ;
#36939=CARTESIAN_POINT ( 'NONE',  ( 2.340729813953370519E-16, 21.32270188528332255, -139.1016058028994564 ) ) ;
#36941=CARTESIAN_POINT ( 'NONE',  ( 3.310556943750001313, 17.50000000000002132, -104.2641058028994649 ) ) ;
#36942=CARTESIAN_POINT ( 'NONE',  ( -1.655278471874999990, 20.36702641396248836, -73.93077246956613635 ) ) ;
#36943=CARTESIAN_POINT ( 'NONE',  ( -3.500000000000000000, 19.52072594216371826, -115.7380641367107614 ) ) ;
#36945=CARTESIAN_POINT ( 'NONE',  ( 1.655278471875001101, 20.36702641396249192, -99.18493913623279923 ) ) ;
#36946=CARTESIAN_POINT ( 'NONE',  ( 3.500000000000001776, 19.52072594216371115, -100.0713974700440900 ) ) ;
#36948=CARTESIAN_POINT ( 'NONE',  ( -3.500000000000001332, 17.50000000000001776, -85.65473080337743284 ) ) ;
#36949=CARTESIAN_POINT ( 'NONE',  ( -1.394453263437886604E-15, 14.00000000000001066, -51.71098080242150274 ) ) ;
#36950=CARTESIAN_POINT ( 'NONE',  ( -1.394453263437886604E-15, 14.00000000000002132, -113.4047308033774186 ) ) ;
#36951=CARTESIAN_POINT ( 'NONE',  ( -3.310556943750001313, 17.50000000000001421, -58.76410580289947916 ) ) ;
#36953=CARTESIAN_POINT ( 'NONE',  ( -1.750000000000002220, 14.46891108675448123, -68.48806413671077564 ) ) ;
#36954=CARTESIAN_POINT ( 'NONE',  ( 1.655278471875001101, 20.36702641396249547, -114.0974391362327935 ) ) ;
#36957=ORIENTED_EDGE ( 'NONE', *, *, #41264, .T. ) ;
#36961=CARTESIAN_POINT ( 'NONE',  ( 4.648177544792955347E-16, 21.00000000000002487, -130.9047308033774186 ) ) ;
#36962=CARTESIAN_POINT ( 'NONE',  ( 3.500000000000001332, 17.50000000000001066, -33.46098080242150274 ) ) ;
#36964=CARTESIAN_POINT ( 'NONE',  ( -1.655278471875002211, 14.63297358603754539, -70.59743913623280775 ) ) ;
#36967=ORIENTED_EDGE ( 'NONE', *, *, #15459, .F. ) ;
#36968=CARTESIAN_POINT ( 'NONE',  ( 4.648177544792955347E-16, 21.00000000000002487, -131.2109808024214885 ) ) ;
#36969=CARTESIAN_POINT ( 'NONE',  ( 1.750000000000001110, 20.53108891324555785, -111.9880641367107614 ) ) ;
#36972=VECTOR ( 'NONE', #38228, 1000.000000000000000 ) ;
#36973=ORIENTED_EDGE ( 'NONE', *, *, #37893, .T. ) ;
#36975=CARTESIAN_POINT ( 'NONE',  ( 3.310556943750001313, 17.50000000000002487, -134.2641058028994507 ) ) ;
#36976=CARTESIAN_POINT ( 'NONE',  ( -3.500000000000002220, 15.47927405783632793, -74.57139747004410424 ) ) ;
#36977=CARTESIAN_POINT ( 'NONE',  ( 2.340729813953370519E-16, 21.32270188528330834, -47.10160580289945642 ) ) ;
#36979=CARTESIAN_POINT ( 'NONE',  ( -3.310556943750001313, 17.50000000000001066, -32.85160580289946353 ) ) ;
#36980=CARTESIAN_POINT ( 'NONE',  ( -1.655278471875002211, 14.63297358603754894, -100.6849391362327992 ) ) ;
#36981=EDGE_CURVE ( 'NONE', #39088, #31100, #27402, .T. ) ;
#36983=CARTESIAN_POINT ( 'NONE',  ( 1.655278471875001101, 20.36702641396248481, -24.09743913623281486 ) ) ;
#36984=LINE ( 'NONE', #13796, #11466 ) ;
#36985=CARTESIAN_POINT ( 'NONE',  ( -3.500000000000002220, 15.47927405783632970, -95.87764746908815994 ) ) ;
#36986=CARTESIAN_POINT ( 'NONE',  ( 3.500000000000001332, 17.50000000000002487, -132.4609808024214885 ) ) ;
#36987=CARTESIAN_POINT ( 'NONE',  ( -0.9378221735089291577, 21.00000000000001421, -61.86007260463890134 ) ) ;
#36988=CARTESIAN_POINT ( 'NONE',  ( -7.424026671074350129E-16, 13.45854811567263631, -87.40473080337743284 ) ) ;
#36989=CARTESIAN_POINT ( 'NONE',  ( -1.655278471874999990, 20.36702641396248836, -72.01827246956612782 ) ) ;
#36991=CARTESIAN_POINT ( 'NONE',  ( -0.9378221735089310451, 14.00000000000002309, -111.4493890021159501 ) ) ;
#36993=CARTESIAN_POINT ( 'NONE',  ( -1.394453263437886604E-15, 14.00000000000002132, -119.7109808024215170 ) ) ;
#36994=CARTESIAN_POINT ( 'NONE',  ( 2.474675557024783212E-16, 21.54145188432739388, -48.21098080242150274 ) ) ;
#36995=CARTESIAN_POINT ( 'NONE',  ( 4.286263797015737581E-16, 14.00000000000002487, -149.5231586289125687 ) ) ;
#36996=CARTESIAN_POINT ( 'NONE',  ( 7.367361408496833051E-14, 14.00000000000001776, -95.71098080242150274 ) ) ;
#36997=ORIENTED_EDGE ( 'NONE', *, *, #33525, .T. ) ;
#36998=CARTESIAN_POINT ( 'NONE',  ( 3.500000000000001776, 19.52072594216371826, -113.0713974700440900 ) ) ;
#37001=CARTESIAN_POINT ( 'NONE',  ( -3.310556943750001313, 17.50000000000001066, -23.85160580289946708 ) ) ;
#37006=CARTESIAN_POINT ( 'NONE',  ( -3.310556943750001313, 17.50000000000001776, -76.76410580289946495 ) ) ;
#37007=CARTESIAN_POINT ( 'NONE',  ( 3.500000000000001332, 19.52072594216371826, -116.0713974700440900 ) ) ;
#37008=CARTESIAN_POINT ( 'NONE',  ( 1.749999999999998224, 14.46891108675448656, -127.3213974700440900 ) ) ;
#37009=CARTESIAN_POINT ( 'NONE',  ( -1.394453263437886604E-15, 14.00000000000001421, -75.40473080337740441 ) ) ;
#37010=EDGE_LOOP ( 'NONE', ( #4563, #37201, #13781, #17028 ) ) ;
#37012=CARTESIAN_POINT ( 'NONE',  ( 3.310556943749999981, 15.58864905735836892, -83.34743913623279354 ) ) ;
#37013=ORIENTED_EDGE ( 'NONE', *, *, #31226, .T. ) ;
#37014=EDGE_LOOP ( 'NONE', ( #14178, #34800, #31280, #38829 ) ) ;
#37020=EDGE_CURVE ( 'NONE', #19667, #5882, #26032, .T. ) ;
#37021=AXIS2_PLACEMENT_3D ( 'NONE', #33520, #13956, #3953 ) ;
#37022=DIRECTION ( 'NONE',  ( -0.000000000000000000, 1.259100132267607459E-16, -1.000000000000000000 ) ) ;
#37023=CARTESIAN_POINT ( 'NONE',  ( -3.310556943750002645, 15.58864905735836714, -53.76827246956612782 ) ) ;
#37024=CARTESIAN_POINT ( 'NONE',  ( 1.655278471875001101, 20.36702641396249547, -114.1849391362327850 ) ) ;
#37026=CARTESIAN_POINT ( 'NONE',  ( -3.500000000000002220, 15.47927405783633503, -124.5713974700440900 ) ) ;
#37027=CARTESIAN_POINT ( 'NONE',  ( 3.310556943750001313, 17.50000000000001066, -40.26410580289947916 ) ) ;
#37028=CARTESIAN_POINT ( 'NONE',  ( 3.310556943750001313, 19.41135094264166128, -65.26827246956614204 ) ) ;
#37029=CARTESIAN_POINT ( 'NONE',  ( 3.500000000000001776, 19.52072594216371826, -113.3776474690881741 ) ) ;
#37030=CARTESIAN_POINT ( 'NONE',  ( -3.310556943750002645, 15.58864905735837425, -98.68077246956613635 ) ) ;
#37032=CARTESIAN_POINT ( 'NONE',  ( 0.000000000000000000, 17.50000000000002487, -149.5231586289125687 ) ) ;
#37035=CARTESIAN_POINT ( 'NONE',  ( 3.500000000000001332, 17.50000000000001421, -70.46098080242151696 ) ) ;
#37037=CARTESIAN_POINT ( 'NONE',  ( -1.655278471874999990, 20.36702641396248481, -29.93077246956614346 ) ) ;
#37038=CARTESIAN_POINT ( 'NONE',  ( 3.310556943750001313, 17.50000000000001776, -92.35160580289947063 ) ) ;
#37039=CARTESIAN_POINT ( 'NONE',  ( 3.500000000000001776, 19.52072594216370760, -61.07139747004409713 ) ) ;
#37040=CARTESIAN_POINT ( 'NONE',  ( 4.648177544792955347E-16, 21.00000000000001421, -55.90473080337743284 ) ) ;
#37041=CARTESIAN_POINT ( 'NONE',  ( 3.310556943749999981, 15.58864905735837247, -114.4349391362327850 ) ) ;
#37042=CARTESIAN_POINT ( 'NONE',  ( -1.655278471874999990, 20.36702641396248481, -37.01827246956612782 ) ) ;
#37048=CARTESIAN_POINT ( 'NONE',  ( 4.648177544792955347E-16, 21.00000000000001066, -23.90473080337742928 ) ) ;
#37050=CARTESIAN_POINT ( 'NONE',  ( -3.310556943750002201, 15.58864905735837425, -95.68077246956615056 ) ) ;
#37051=( BOUNDED_CURVE ( )  B_SPLINE_CURVE ( 2, ( #254, #465, #32785, #36188, #898, #32382, #39593, #9854, #22810 ),
 .UNSPECIFIED., .F., .T. ) 
 B_SPLINE_CURVE_WITH_KNOTS ( ( 3, 2, 2, 2, 3 ),
 ( 0.3104166666666666741, 0.3111111111111111160, 0.3125000000000000000, 0.3138888888888888840, 0.3145833333333333259 ),
 .UNSPECIFIED. ) 
 CURVE ( )  GEOMETRIC_REPRESENTATION_ITEM ( )  RATIONAL_B_SPLINE_CURVE ( ( 0.9330127018922194093, 0.9330127018922194093, 1.000000000000000000, 0.8660254037844387076, 1.000000000000000000, 0.8660254037844387076, 1.000000000000000000, 0.9330127018922194093, 0.9330127018922194093 ) ) 
 REPRESENTATION_ITEM ( '' )  );
#37052=CARTESIAN_POINT ( 'NONE',  ( -1.750000000000002220, 14.46891108675448834, -135.4880641367107614 ) ) ;
#37062=ORIENTED_EDGE ( 'NONE', *, *, #38722, .F. ) ;
#37065=EDGE_LOOP ( 'NONE', ( #22092, #26766, #7600, #30972 ) ) ;
#37066=CARTESIAN_POINT ( 'NONE',  ( 3.500000000000001332, 17.50000000000002132, -118.1547308033774328 ) ) ;
#37072=DIRECTION ( 'NONE',  ( -0.000000000000000000, 1.259100132267607459E-16, -1.000000000000000000 ) ) ;
#37074=ADVANCED_FACE ( 'NONE', ( #8644 ), #37995, .T. ) ;
#37075=CARTESIAN_POINT ( 'NONE',  ( -1.655278471874999990, 20.36702641396249902, -139.9307724695661364 ) ) ;
#37076=CARTESIAN_POINT ( 'NONE',  ( 4.648177544792955347E-16, 21.00000000000001421, -68.21098080242148853 ) ) ;
#37077=CARTESIAN_POINT ( 'NONE',  ( 3.500000000000001332, 19.52072594216371115, -101.3776474690881741 ) ) ;
#37078=CARTESIAN_POINT ( 'NONE',  ( 3.310556943749999981, 15.58864905735837425, -131.4349391362327992 ) ) ;
#37079=CARTESIAN_POINT ( 'NONE',  ( 3.310556943750001313, 17.50000000000001421, -57.35160580289947063 ) ) ;
#37080=VERTEX_POINT ( 'NONE', #37578 ) ;
#37082=CARTESIAN_POINT ( 'NONE',  ( 3.500000000000001776, 19.52072594216372181, -139.0713974700441042 ) ) ;
#37085=CARTESIAN_POINT ( 'NONE',  ( -3.500000000000002220, 15.47927405783633503, -126.8776474690881741 ) ) ;
#37086=CARTESIAN_POINT ( 'NONE',  ( -1.655278471874999990, 20.36702641396249547, -111.9307724695661506 ) ) ;
#37088=CARTESIAN_POINT ( 'NONE',  ( 0.9378221735089367073, 14.00000000000002487, -128.6663226036829428 ) ) ;
#37089=CARTESIAN_POINT ( 'NONE',  ( -3.500000000000001332, 17.50000000000001776, -85.96098080242151696 ) ) ;
#37090=CARTESIAN_POINT ( 'NONE',  ( 0.000000000000000000, 21.00000000000002487, -149.5231586289125687 ) ) ;
#37091=CARTESIAN_POINT ( 'NONE',  ( 1.655278471874998436, 14.63297358603754006, -50.43077246956613635 ) ) ;
#37092=CARTESIAN_POINT ( 'NONE',  ( 3.310556943749999981, 15.58864905735837070, -107.4349391362327992 ) ) ;
#37093=CARTESIAN_POINT ( 'NONE',  ( -3.500000000000001332, 17.50000000000001776, -93.96098080242151696 ) ) ;
#37094=CARTESIAN_POINT ( 'NONE',  ( -1.749999999999999778, 20.53108891324555429, -80.12764746908817415 ) ) ;
#37097=CARTESIAN_POINT ( 'NONE',  ( -3.310556943750001313, 17.50000000000002132, -126.8516058028994422 ) ) ;
#37102=CARTESIAN_POINT ( 'NONE',  ( 2.340729813953370519E-16, 21.32270188528330834, -60.10160580289947063 ) ) ;
#37105=( BOUNDED_CURVE ( )  B_SPLINE_CURVE ( 2, ( #33603, #4462, #30610, #18056, #20412, #37007, #24240, #31030, #27010 ),
 .UNSPECIFIED., .F., .T. ) 
 B_SPLINE_CURVE_WITH_KNOTS ( ( 3, 2, 2, 2, 3 ),
 ( 0.2229166666666666796, 0.2236111111111111216, 0.2250000000000000056, 0.2263888888888888895, 0.2270833333333333315 ),
 .UNSPECIFIED. ) 
 CURVE ( )  GEOMETRIC_REPRESENTATION_ITEM ( )  RATIONAL_B_SPLINE_CURVE ( ( 0.9330127018922194093, 0.9330127018922207416, 1.000000000000000000, 0.8660254037844387076, 1.000000000000000000, 0.8660254037844387076, 1.000000000000000000, 0.9330127018922194093, 0.9330127018922194093 ) ) 
 REPRESENTATION_ITEM ( '' )  );
#37106=CARTESIAN_POINT ( 'NONE',  ( 3.310556943750001313, 17.50000000000001776, -79.35160580289945642 ) ) ;
#37107=EDGE_CURVE ( 'NONE', #16494, #30409, #39072, .T. ) ;
#37112=CARTESIAN_POINT ( 'NONE',  ( -3.310556943750002201, 15.58864905735836714, -41.68077246956614346 ) ) ;
#37113=CARTESIAN_POINT ( 'NONE',  ( 3.310556943749999981, 15.58864905735837070, -99.34743913623280775 ) ) ;
#37114=CARTESIAN_POINT ( 'NONE',  ( -1.394453263437886604E-15, 14.00000000000001421, -59.71098080242150274 ) ) ;
#37117=ORIENTED_EDGE ( 'NONE', *, *, #28049, .T. ) ;
#37119=CARTESIAN_POINT ( 'NONE',  ( -3.310556943750002645, 15.58864905735836714, -51.68077246956613635 ) ) ;
#37120=ORIENTED_EDGE ( 'NONE', *, *, #21452, .F. ) ;
#37123=CARTESIAN_POINT ( 'NONE',  ( 3.500000000000000000, 15.47927405783633503, -125.2380641367107614 ) ) ;
#37125=CARTESIAN_POINT ( 'NONE',  ( 3.500000000000000000, 15.47927405783633326, -113.5443141357548456 ) ) ;
#37128=CARTESIAN_POINT ( 'NONE',  ( -1.749999999999999778, 20.53108891324554719, -40.12764746908817415 ) ) ;
#37130=EDGE_CURVE ( 'NONE', #14304, #39088, #40766, .T. ) ;
#37132=CARTESIAN_POINT ( 'NONE',  ( 2.340729813953370519E-16, 21.32270188528330479, -32.10160580289945642 ) ) ;
#37133=EDGE_CURVE ( 'NONE', #18319, #5191, #40980, .T. ) ;
#37135=CARTESIAN_POINT ( 'NONE',  ( -7.022189441860112050E-16, 13.67729811471672718, -129.5141058028994507 ) ) ;
#37138=CARTESIAN_POINT ( 'NONE',  ( -3.500000000000000000, 19.52072594216371115, -75.73806413671076143 ) ) ;
#37139=CARTESIAN_POINT ( 'NONE',  ( -3.310556943750001313, 17.50000000000002132, -123.8516058028994564 ) ) ;
#37141=CARTESIAN_POINT ( 'NONE',  ( 3.310556943750001313, 19.41135094264166483, -88.18077246956613635 ) ) ;
#37142=CARTESIAN_POINT ( 'NONE',  ( 4.648177544792955347E-16, 21.00000000000001066, -45.90473080337741862 ) ) ;
#37143=CARTESIAN_POINT ( 'NONE',  ( 3.500000000000001332, 19.52072594216370760, -65.07139747004410424 ) ) ;
#37144=CARTESIAN_POINT ( 'NONE',  ( -3.310556943750001313, 17.50000000000002487, -142.8516058028994564 ) ) ;
#37145=CARTESIAN_POINT ( 'NONE',  ( 1.750000000000001110, 20.53108891324555074, -68.98806413671077564 ) ) ;
#37147=CARTESIAN_POINT ( 'NONE',  ( 1.655278471874998436, 14.63297358603754184, -56.51827246956612782 ) ) ;
#37149=CARTESIAN_POINT ( 'NONE',  ( 0.9378221735089260491, 21.00000000000002842, -137.2556390011600627 ) ) ;
#37150=CARTESIAN_POINT ( 'NONE',  ( -1.394453263437886604E-15, 14.00000000000001776, -98.71098080242150274 ) ) ;
#37151=CARTESIAN_POINT ( 'NONE',  ( -3.310556943750002645, 15.58864905735837070, -74.76827246956612782 ) ) ;
#37152=CARTESIAN_POINT ( 'NONE',  ( -3.310556943750002645, 15.58864905735837958, -139.7682724695661420 ) ) ;
#37154=CARTESIAN_POINT ( 'NONE',  ( -1.655278471875002211, 14.63297358603754894, -102.5974391362328220 ) ) ;
#37155=CARTESIAN_POINT ( 'NONE',  ( -3.310556943750001313, 17.50000000000001776, -74.76410580289947916 ) ) ;
#37156=ORIENTED_EDGE ( 'NONE', *, *, #41556, .T. ) ;
#37157=CARTESIAN_POINT ( 'NONE',  ( 1.655278471874998436, 14.63297358603754539, -94.51827246956612782 ) ) ;
#37159=CARTESIAN_POINT ( 'NONE',  ( 4.648177544792955347E-16, 21.00000000000001776, -81.90473080337743284 ) ) ;
#37160=CARTESIAN_POINT ( 'NONE',  ( -1.394453263437886604E-15, 14.00000000000001776, -103.7109808024215027 ) ) ;
#37161=CARTESIAN_POINT ( 'NONE',  ( -3.310556943750000425, 19.41135094264166483, -56.84743913623280065 ) ) ;
#37162=CARTESIAN_POINT ( 'NONE',  ( -3.500000000000001332, 17.50000000000002132, -124.9609808024215027 ) ) ;
#37163=CARTESIAN_POINT ( 'NONE',  ( 3.310556943749999981, 15.58864905735837247, -116.3474391362327935 ) ) ;
#37164=DIRECTION ( 'NONE',  ( -0.000000000000000000, 1.259100132267607459E-16, -1.000000000000000000 ) ) ;
#37169=CARTESIAN_POINT ( 'NONE',  ( -1.749999999999999778, 20.53108891324555785, -110.1276474690881741 ) ) ;
#37170=CARTESIAN_POINT ( 'NONE',  ( -3.310556943750002645, 15.58864905735837070, -69.68077246956613635 ) ) ;
#37178=CARTESIAN_POINT ( 'NONE',  ( -0.9378221735089303790, 14.00000000000002487, -142.7556390011600342 ) ) ;
#37179=CARTESIAN_POINT ( 'NONE',  ( 2.340729813953370519E-16, 21.32270188528332255, -138.0141058028994792 ) ) ;
#37180=CARTESIAN_POINT ( 'NONE',  ( -1.750000000000002220, 14.46891108675448123, -74.48806413671076143 ) ) ;
#37181=CARTESIAN_POINT ( 'NONE',  ( 3.310556943750001313, 17.50000000000001066, -46.35160580289945642 ) ) ;
#37182=CARTESIAN_POINT ( 'NONE',  ( 3.310556943749999981, 15.58864905735836182, -32.43493913623279923 ) ) ;
#37183=CARTESIAN_POINT ( 'NONE',  ( 3.310556943750001313, 19.41135094264166483, -98.26827246956612782 ) ) ;
#37185=CARTESIAN_POINT ( 'NONE',  ( 3.310556943750001313, 19.41135094264167549, -136.2682724695661136 ) ) ;
#37187=CARTESIAN_POINT ( 'NONE',  ( 2.474675557024783212E-16, 21.54145188432739744, -98.21098080242150274 ) ) ;
#37188=CARTESIAN_POINT ( 'NONE',  ( 1.749999999999998224, 14.46891108675448656, -132.6276474690881741 ) ) ;
#37190=CARTESIAN_POINT ( 'NONE',  ( 3.500000000000001776, 19.52072594216371115, -86.07139747004409003 ) ) ;
#37191=ADVANCED_FACE ( 'NONE', ( #39035 ), #32446, .T. ) ;
#37192=CARTESIAN_POINT ( 'NONE',  ( 2.340729813953370519E-16, 21.32270188528331190, -71.10160580289947063 ) ) ;
#37194=CARTESIAN_POINT ( 'NONE',  ( 1.749999999999998224, 14.46891108675448123, -84.32139747004409003 ) ) ;
#37196=CARTESIAN_POINT ( 'NONE',  ( 4.286263797015737581E-16, 14.00000000000002487, -149.5231586289125687 ) ) ;
#37197=CARTESIAN_POINT ( 'NONE',  ( 1.750000000000001110, 20.53108891324555074, -48.29431413575484555 ) ) ;
#37198=CARTESIAN_POINT ( 'NONE',  ( 1.655278471875001101, 20.36702641396249547, -119.0974391362328078 ) ) ;
#37199=DIRECTION ( 'NONE',  ( -0.000000000000000000, 1.259100132267607459E-16, -1.000000000000000000 ) ) ;
#37201=ORIENTED_EDGE ( 'NONE', *, *, #32578, .T. ) ;
#37202=CARTESIAN_POINT ( 'NONE',  ( 3.500000000000000000, 15.47927405783632970, -116.2380641367107614 ) ) ;
#37204=CYLINDRICAL_SURFACE ( 'NONE', #11122, 3.499999999999999556 ) ;
#37205=CARTESIAN_POINT ( 'NONE',  ( 4.286263797015737581E-16, 14.00000000000002487, -149.5231586289125687 ) ) ;
#37208=CARTESIAN_POINT ( 'NONE',  ( 2.340729813953370519E-16, 21.32270188528331190, -70.01410580289947916 ) ) ;
#37209=CARTESIAN_POINT ( 'NONE',  ( -3.500000000000000000, 19.52072594216371826, -134.0443141357548598 ) ) ;
#37210=CARTESIAN_POINT ( 'NONE',  ( -1.750000000000002220, 14.46891108675447768, -44.79431413575483845 ) ) ;
#37212=CARTESIAN_POINT ( 'NONE',  ( -0.9378221735089291577, 21.00000000000001421, -64.16632260368298546 ) ) ;
#37213=CARTESIAN_POINT ( 'NONE',  ( -1.655278471874999990, 20.36702641396249192, -85.93077246956613635 ) ) ;
#37214=ORIENTED_EDGE ( 'NONE', *, *, #6867, .T. ) ;
#37215=VERTEX_POINT ( 'NONE', #39234 ) ;
#37216=( BOUNDED_CURVE ( )  B_SPLINE_CURVE ( 2, ( #14607, #1216, #11207, #24597, #34373, #14812, #4405, #5231, #23982 ),
 .UNSPECIFIED., .F., .F. ) 
 B_SPLINE_CURVE_WITH_KNOTS ( ( 3, 2, 2, 2, 3 ),
 ( 0.9729166666666666519, 0.9736111111111110938, 0.9749999999999999778, 0.9763888888888888618, 0.9770833333333333037 ),
 .UNSPECIFIED. ) 
 CURVE ( )  GEOMETRIC_REPRESENTATION_ITEM ( )  RATIONAL_B_SPLINE_CURVE ( ( 0.9330127018922194093, 0.9330127018922194093, 1.000000000000000000, 0.8660254037844387076, 1.000000000000000000, 0.8660254037844387076, 1.000000000000000000, 0.9330127018922194093, 0.9330127018922194093 ) ) 
 REPRESENTATION_ITEM ( '' )  );
#37219=CARTESIAN_POINT ( 'NONE',  ( 0.000000000000000000, 21.00000000000002487, -149.5231586289125687 ) ) ;
#37220=( BOUNDED_CURVE ( )  B_SPLINE_CURVE ( 2, ( #11915, #8314, #17689, #4914, #8106, #24281, #15121, #37868, #18302 ),
 .UNSPECIFIED., .F., .T. ) 
 B_SPLINE_CURVE_WITH_KNOTS ( ( 3, 2, 2, 2, 3 ),
 ( 0.2145833333333333481, 0.2152777777777777901, 0.2166666666666666741, 0.2180555555555555580, 0.2187500000000000000 ),
 .UNSPECIFIED. ) 
 CURVE ( )  GEOMETRIC_REPRESENTATION_ITEM ( )  RATIONAL_B_SPLINE_CURVE ( ( 0.9330127018922194093, 0.9330127018922207416, 1.000000000000000000, 0.8660254037844387076, 1.000000000000000000, 0.8660254037844387076, 1.000000000000000000, 0.9330127018922194093, 0.9330127018922194093 ) ) 
 REPRESENTATION_ITEM ( '' )  );
#37222=CARTESIAN_POINT ( 'NONE',  ( -0.9378221735089291577, 21.00000000000002132, -126.8600726046389155 ) ) ;
#37223=CARTESIAN_POINT ( 'NONE',  ( 3.310556943750001313, 19.41135094264165772, -46.26827246956613493 ) ) ;
#37224=CARTESIAN_POINT ( 'NONE',  ( -1.655278471875002211, 14.63297358603755072, -115.6849391362327850 ) ) ;
#37225=VERTEX_POINT ( 'NONE', #15887 ) ;
#37226=CARTESIAN_POINT ( 'NONE',  ( -1.749999999999999778, 20.53108891324555785, -121.8213974700441042 ) ) ;
#37227=CARTESIAN_POINT ( 'NONE',  ( 3.310556943749999981, 15.58864905735836182, -38.34743913623280775 ) ) ;
#37228=CARTESIAN_POINT ( 'NONE',  ( -3.310556943750000425, 19.41135094264166128, -63.93493913623280633 ) ) ;
#37229=CARTESIAN_POINT ( 'NONE',  ( -3.500000000000000888, 19.52072594216371826, -111.0443141357548456 ) ) ;
#37231=CARTESIAN_POINT ( 'NONE',  ( 1.655278471874998436, 14.63297358603754716, -97.43077246956613635 ) ) ;
#37234=CARTESIAN_POINT ( 'NONE',  ( -3.500000000000002220, 15.47927405783632082, -25.87764746908817060 ) ) ;
#37237=CARTESIAN_POINT ( 'NONE',  ( 2.474675557024783212E-16, 21.54145188432739388, -65.21098080242150274 ) ) ;
#37239=CARTESIAN_POINT ( 'NONE',  ( -7.022189441860112050E-16, 13.67729811471671475, -34.51410580289947205 ) ) ;
#37240=CARTESIAN_POINT ( 'NONE',  ( -3.310556943750001313, 17.50000000000001776, -91.85160580289947063 ) ) ;
#37241=CARTESIAN_POINT ( 'NONE',  ( -3.500000000000002220, 15.47927405783632437, -56.57139747004409713 ) ) ;
#37242=CARTESIAN_POINT ( 'NONE',  ( -1.749999999999999778, 20.53108891324556140, -138.1276474690881741 ) ) ;
#37243=CARTESIAN_POINT ( 'NONE',  ( 3.310556943749999981, 15.58864905735837247, -111.4349391362327992 ) ) ;
#37244=CARTESIAN_POINT ( 'NONE',  ( 3.310556943749999981, 15.58864905735836182, -35.43493913623279923 ) ) ;
#37246=CARTESIAN_POINT ( 'NONE',  ( 3.500000000000000000, 15.47927405783632437, -66.23806413671076143 ) ) ;
#37250=CARTESIAN_POINT ( 'NONE',  ( -1.394453263437886604E-15, 14.00000000000001066, -48.71098080242150985 ) ) ;
#37251=CARTESIAN_POINT ( 'NONE',  ( 3.310556943750001313, 17.50000000000001776, -92.26410580289947916 ) ) ;
#37252=CYLINDRICAL_SURFACE ( 'NONE', #28058, 3.499999999999999556 ) ;
#37258=CARTESIAN_POINT ( 'NONE',  ( 0.000000000000000000, 21.00000000000002487, -149.5231586289125687 ) ) ;
#37259=ORIENTED_EDGE ( 'NONE', *, *, #21246, .F. ) ;
#37263=ORIENTED_EDGE ( 'NONE', *, *, #38433, .F. ) ;
#37271=ORIENTED_EDGE ( 'NONE', *, *, #6803, .F. ) ;
#37272=CARTESIAN_POINT ( 'NONE',  ( -1.750000000000002220, 14.46891108675447768, -53.79431413575484555 ) ) ;
#37274=CARTESIAN_POINT ( 'NONE',  ( -3.310556943750001313, 17.50000000000002487, -134.7641058028994507 ) ) ;
#37275=CARTESIAN_POINT ( 'NONE',  ( -0.9378221735089291577, 21.00000000000002487, -132.8600726046389013 ) ) ;
#37276=CARTESIAN_POINT ( 'NONE',  ( 4.648177544792955347E-16, 21.00000000000001776, -76.90473080337740441 ) ) ;
#37277=CARTESIAN_POINT ( 'NONE',  ( 3.310556943749999981, 15.58864905735837425, -130.4349391362327992 ) ) ;
#37278=CARTESIAN_POINT ( 'NONE',  ( -3.310556943750000425, 19.41135094264166128, -53.93493913623280633 ) ) ;
#37279=ORIENTED_EDGE ( 'NONE', *, *, #34964, .T. ) ;
#37282=CARTESIAN_POINT ( 'NONE',  ( -1.749999999999999778, 20.53108891324556140, -138.8213974700441042 ) ) ;
#37284=CARTESIAN_POINT ( 'NONE',  ( -7.424026671074350129E-16, 13.45854811567264164, -126.7109808024215027 ) ) ;
#37285=CARTESIAN_POINT ( 'NONE',  ( 3.310556943749999981, 15.58864905735837247, -115.3474391362327935 ) ) ;
#37287=( BOUNDED_CURVE ( )  B_SPLINE_CURVE ( 2, ( #13293, #4351, #33709, #14971, #27938, #11360, #2201, #37314, #31132 ),
 .UNSPECIFIED., .F., .F. ) 
 B_SPLINE_CURVE_WITH_KNOTS ( ( 3, 2, 2, 2, 3 ),
 ( 0.4104166666666666519, 0.4111111111111110938, 0.4124999999999999778, 0.4138888888888888618, 0.4145833333333333592 ),
 .UNSPECIFIED. ) 
 CURVE ( )  GEOMETRIC_REPRESENTATION_ITEM ( )  RATIONAL_B_SPLINE_CURVE ( ( 0.9330127018922194093, 0.9330127018922194093, 1.000000000000000000, 0.8660254037844387076, 1.000000000000000000, 0.8660254037844387076, 1.000000000000000000, 0.9330127018922167448, 0.9330127018922194093 ) ) 
 REPRESENTATION_ITEM ( '' )  );
#37289=CARTESIAN_POINT ( 'NONE',  ( -3.500000000000000888, 19.52072594216371115, -80.04431413575484555 ) ) ;
#37290=AXIS2_PLACEMENT_3D ( 'NONE', #473, #7068, #13445 ) ;
#37291=LINE ( 'NONE', #8145, #6978 ) ;
#37292=CARTESIAN_POINT ( 'NONE',  ( -3.310556943750000425, 19.41135094264166128, -48.84743913623280775 ) ) ;
#37293=CARTESIAN_POINT ( 'NONE',  ( -1.655278471875002211, 14.63297358603754894, -105.6849391362327992 ) ) ;
#37294=LINE ( 'NONE', #11539, #19367 ) ;
#37295=CARTESIAN_POINT ( 'NONE',  ( -1.394453263437886604E-15, 14.00000000000001066, -35.40473080337743284 ) ) ;
#37297=CARTESIAN_POINT ( 'NONE',  ( 2.340729813953370519E-16, 21.32270188528332255, -131.1016058028994564 ) ) ;
#37300=CARTESIAN_POINT ( 'NONE',  ( 3.500000000000001332, 19.52072594216371826, -143.0713974700441042 ) ) ;
#37301=LINE ( 'NONE', #30066, #23098 ) ;
#37302=CARTESIAN_POINT ( 'NONE',  ( 2.340729813953370519E-16, 21.32270188528330834, -59.10160580289947063 ) ) ;
#37303=EDGE_CURVE ( 'NONE', #21810, #42029, #1321, .T. ) ;
#37305=CARTESIAN_POINT ( 'NONE',  ( 3.310556943749999981, 15.58864905735836892, -81.43493913623281344 ) ) ;
#37306=EDGE_CURVE ( 'NONE', #34834, #3024, #42070, .T. ) ;
#37307=CARTESIAN_POINT ( 'NONE',  ( 0.9378221735089300459, 21.00000000000001066, -45.25563900116003424 ) ) ;
#37308=CARTESIAN_POINT ( 'NONE',  ( 1.749999999999998224, 14.46891108675447946, -77.32139747004410424 ) ) ;
#37311=CARTESIAN_POINT ( 'NONE',  ( -1.394453263437886604E-15, 14.00000000000001421, -74.40473080337743284 ) ) ;
#37313=CARTESIAN_POINT ( 'NONE',  ( -3.310556943750000425, 19.41135094264166128, -40.84743913623280775 ) ) ;
#37314=CARTESIAN_POINT ( 'NONE',  ( -0.9378221735088960731, 14.00000000000000000, -93.44938900211595012 ) ) ;
#37316=ORIENTED_EDGE ( 'NONE', *, *, #12203, .F. ) ;
#37318=CARTESIAN_POINT ( 'NONE',  ( 1.655278471875001101, 20.36702641396248836, -47.09743913623280775 ) ) ;
#37319=VERTEX_POINT ( 'NONE', #25868 ) ;
#37322=CARTESIAN_POINT ( 'NONE',  ( -3.500000000000000000, 19.52072594216371115, -98.73806413671077564 ) ) ;
#37326=CARTESIAN_POINT ( 'NONE',  ( 0.9378221735089281585, 14.00000000000001066, -43.66632260368299256 ) ) ;
#37327=CARTESIAN_POINT ( 'NONE',  ( 1.750000000000001110, 20.53108891324554719, -37.29431413575484555 ) ) ;
#37328=DIRECTION ( 'NONE',  ( -0.000000000000000000, 1.259100132267607459E-16, -1.000000000000000000 ) ) ;
#37329=DIRECTION ( 'NONE',  ( 0.000000000000000000, 1.000000000000000000, 0.000000000000000000 ) ) ;
#37333=CARTESIAN_POINT ( 'NONE',  ( 3.310556943750001313, 17.50000000000001066, -26.35160580289947063 ) ) ;
#37334=CARTESIAN_POINT ( 'NONE',  ( 1.749999999999998224, 14.46891108675448478, -122.3213974700441042 ) ) ;
#37335=CARTESIAN_POINT ( 'NONE',  ( -1.655278471875002211, 14.63297358603755249, -128.5974391362328220 ) ) ;
#37338=CARTESIAN_POINT ( 'NONE',  ( -1.394453263437886604E-15, 14.00000000000001066, -45.40473080337742573 ) ) ;
#37339=( BOUNDED_CURVE ( )  B_SPLINE_CURVE ( 2, ( #17253, #8294, #34242, #24065, #7679, #20858, #14887, #20439, #14480 ),
 .UNSPECIFIED., .F., .F. ) 
 B_SPLINE_CURVE_WITH_KNOTS ( ( 3, 2, 2, 2, 3 ),
 ( 0.7937499999999999556, 0.7944444444444443976, 0.7958333333333332815, 0.7972222222222222765, 0.7979166666666667185 ),
 .UNSPECIFIED. ) 
 CURVE ( )  GEOMETRIC_REPRESENTATION_ITEM ( )  RATIONAL_B_SPLINE_CURVE ( ( 0.9330127018922194093, 0.9330127018922194093, 1.000000000000000000, 0.8660254037844387076, 1.000000000000000000, 0.8660254037844387076, 1.000000000000000000, 0.9330127018922194093, 0.9330127018922194093 ) ) 
 REPRESENTATION_ITEM ( '' )  );
#37340=CARTESIAN_POINT ( 'NONE',  ( 3.310556943749999981, 15.58864905735837247, -122.4349391362327992 ) ) ;
#37341=CARTESIAN_POINT ( 'NONE',  ( -0.9378221735089310451, 14.00000000000001599, -55.44938900211595723 ) ) ;
#37342=CARTESIAN_POINT ( 'NONE',  ( -7.424026671074350129E-16, 13.45854811567263098, -35.40473080337743284 ) ) ;
#37344=CARTESIAN_POINT ( 'NONE',  ( -3.310556943750000425, 19.41135094264167549, -141.9349391362327992 ) ) ;
#37345=CARTESIAN_POINT ( 'NONE',  ( 2.474675557024783212E-16, 21.54145188432739388, -70.90473080337743284 ) ) ;
#37346=CARTESIAN_POINT ( 'NONE',  ( 3.310556943750001313, 17.50000000000001421, -54.35160580289946353 ) ) ;
#37349=CARTESIAN_POINT ( 'NONE',  ( 3.310556943749999981, 15.58864905735836714, -74.43493913623279923 ) ) ;
#37351=CARTESIAN_POINT ( 'NONE',  ( 1.655278471874998436, 14.63297358603754716, -101.4307724695661364 ) ) ;
#37352=CARTESIAN_POINT ( 'NONE',  ( -1.655278471874999990, 20.36702641396249192, -75.93077246956613635 ) ) ;
#37354=CARTESIAN_POINT ( 'NONE',  ( -3.310556943750000425, 19.41135094264166838, -93.93493913623279923 ) ) ;
#37358=CARTESIAN_POINT ( 'NONE',  ( 4.648177544792955347E-16, 21.00000000000001066, -33.90473080337743284 ) ) ;
#37359=CARTESIAN_POINT ( 'NONE',  ( -3.310556943750001313, 17.50000000000001421, -57.76410580289947916 ) ) ;
#37361=CARTESIAN_POINT ( 'NONE',  ( 1.655278471874998436, 14.63297358603754716, -108.4307724695661506 ) ) ;
#37365=ADVANCED_FACE ( 'NONE', ( #13093 ), #19677, .T. ) ;
#37369=CARTESIAN_POINT ( 'NONE',  ( -3.310556943750001313, 17.50000000000001421, -68.76410580289947916 ) ) ;
#37370=EDGE_LOOP ( 'NONE', ( #32953, #34496, #7820, #31512 ) ) ;
#37371=ORIENTED_EDGE ( 'NONE', *, *, #12478, .F. ) ;
#37372=DIRECTION ( 'NONE',  ( -0.000000000000000000, 1.259100132267607459E-16, -1.000000000000000000 ) ) ;
#37373=CARTESIAN_POINT ( 'NONE',  ( 0.9378221735089300459, 21.00000000000002132, -111.9493890021159501 ) ) ;
#37376=ORIENTED_EDGE ( 'NONE', *, *, #26123, .F. ) ;
#37378=CARTESIAN_POINT ( 'NONE',  ( -1.655278471874999990, 20.36702641396249902, -132.9307724695661364 ) ) ;
#37379=AXIS2_PLACEMENT_3D ( 'NONE', #16075, #23055, #29643 ) ;
#37380=CARTESIAN_POINT ( 'NONE',  ( -3.500000000000000000, 19.52072594216371115, -74.73806413671076143 ) ) ;
#37381=EDGE_CURVE ( 'NONE', #19458, #13615, #177, .T. ) ;
#37382=CARTESIAN_POINT ( 'NONE',  ( -3.310556943750000425, 19.41135094264165772, -39.93493913623280633 ) ) ;
#37383=CARTESIAN_POINT ( 'NONE',  ( 1.655278471875001101, 20.36702641396248481, -32.18493913623279923 ) ) ;
#37384=CARTESIAN_POINT ( 'NONE',  ( 3.310556943750001313, 17.50000000000001776, -92.35160580289947063 ) ) ;
#37385=CARTESIAN_POINT ( 'NONE',  ( 1.749999999999998224, 14.46891108675447413, -26.32139747004409713 ) ) ;
#37387=VECTOR ( 'NONE', #37997, 1000.000000000000000 ) ;
#37388=CARTESIAN_POINT ( 'NONE',  ( 3.310556943749999981, 15.58864905735837780, -140.4349391362327992 ) ) ;
#37390=CARTESIAN_POINT ( 'NONE',  ( 3.500000000000000000, 15.47927405783632793, -95.54431413575484555 ) ) ;
#37394=CARTESIAN_POINT ( 'NONE',  ( 3.500000000000001776, 19.52072594216371115, -87.07139747004410424 ) ) ;
#37395=CARTESIAN_POINT ( 'NONE',  ( -1.655278471875002211, 14.63297358603754539, -71.68493913623278502 ) ) ;
#37397=CARTESIAN_POINT ( 'NONE',  ( 3.500000000000001332, 17.50000000000001776, -84.15473080337743284 ) ) ;
#37400=CARTESIAN_POINT ( 'NONE',  ( 1.749999999999998224, 14.46891108675447590, -48.62764746908818125 ) ) ;
#37401=CARTESIAN_POINT ( 'NONE',  ( -1.655278471874999990, 20.36702641396249547, -119.9307724695661364 ) ) ;
#37403=CARTESIAN_POINT ( 'NONE',  ( -1.749999999999999778, 20.53108891324554719, -35.12764746908818125 ) ) ;
#37404=VERTEX_POINT ( 'NONE', #23941 ) ;
#37405=CARTESIAN_POINT ( 'NONE',  ( 2.474675557024783212E-16, 21.54145188432740099, -115.9047308033774328 ) ) ;
#37407=CARTESIAN_POINT ( 'NONE',  ( -3.500000000000001332, 17.50000000000001776, -83.65473080337743284 ) ) ;
#37408=DIRECTION ( 'NONE',  ( -0.000000000000000000, 1.259100132267607459E-16, -1.000000000000000000 ) ) ;
#37411=CARTESIAN_POINT ( 'NONE',  ( -3.310556943750000425, 19.41135094264166483, -73.84743913623280775 ) ) ;
#37412=CARTESIAN_POINT ( 'NONE',  ( -3.500000000000002220, 15.47927405783633326, -96.87764746908817415 ) ) ;
#37413=CONICAL_SURFACE ( 'NONE', #10224, 577.3502691896253509, 0.5235987755982987046 ) ;
#37416=EDGE_CURVE ( 'NONE', #4203, #11365, #8890, .T. ) ;
#37417=LINE ( 'NONE', #11457, #11725 ) ;
#37418=CARTESIAN_POINT ( 'NONE',  ( 3.500000000000001332, 19.52072594216370405, -25.37764746908817415 ) ) ;
#37419=CARTESIAN_POINT ( 'NONE',  ( 1.655278471875001101, 20.36702641396249192, -86.09743913623279354 ) ) ;
#37421=VERTEX_POINT ( 'NONE', #20528 ) ;
#37427=ORIENTED_EDGE ( 'NONE', *, *, #30611, .T. ) ;
#37429=CARTESIAN_POINT ( 'NONE',  ( -3.310556943750000425, 19.41135094264166128, -49.93493913623279923 ) ) ;
#37430=CARTESIAN_POINT ( 'NONE',  ( -7.022189441860112050E-16, 13.67729811471672541, -106.6016058028994564 ) ) ;
#37434=CARTESIAN_POINT ( 'NONE',  ( -3.310556943750002645, 15.58864905735836537, -33.68077246956615056 ) ) ;
#37435=CARTESIAN_POINT ( 'NONE',  ( -3.310556943750001313, 17.50000000000001421, -64.85160580289945642 ) ) ;
#37436=CARTESIAN_POINT ( 'NONE',  ( -1.749999999999999778, 20.53108891324555785, -113.1276474690881741 ) ) ;
#37438=CARTESIAN_POINT ( 'NONE',  ( -1.655278471874999990, 20.36702641396249192, -98.93077246956613635 ) ) ;
#37440=CARTESIAN_POINT ( 'NONE',  ( 0.9378221735089281585, 14.00000000000001066, -52.36007260463890844 ) ) ;
#37443=CARTESIAN_POINT ( 'NONE',  ( -3.500000000000002220, 15.47927405783632437, -63.87764746908818125 ) ) ;
#37444=CARTESIAN_POINT ( 'NONE',  ( -1.394453263437886604E-15, 14.00000000000001066, -43.71098080242150985 ) ) ;
#37445=CARTESIAN_POINT ( 'NONE',  ( -3.310556943750001313, 17.50000000000001066, -32.76410580289947205 ) ) ;
#37446=CARTESIAN_POINT ( 'NONE',  ( -3.310556943750000425, 19.41135094264166483, -91.93493913623278502 ) ) ;
#37447=CARTESIAN_POINT ( 'NONE',  ( -3.500000000000002220, 15.47927405783632260, -51.57139747004408292 ) ) ;
#37448=CARTESIAN_POINT ( 'NONE',  ( -8.715332896486792803E-15, 21.00000000000002842, -138.2109808024214601 ) ) ;
#37449=CARTESIAN_POINT ( 'NONE',  ( -7.022189441860112050E-16, 13.67729811471672896, -109.6016058028994564 ) ) ;
#37450=CARTESIAN_POINT ( 'NONE',  ( 3.310556943749999981, 15.58864905735836182, -37.43493913623280633 ) ) ;
#37452=CARTESIAN_POINT ( 'NONE',  ( -1.394453263437886604E-15, 14.00000000000001066, -53.71098080242150985 ) ) ;
#37458=CARTESIAN_POINT ( 'NONE',  ( 3.310556943750001313, 17.50000000000001776, -86.26410580289947916 ) ) ;
#37463=CARTESIAN_POINT ( 'NONE',  ( 4.648177544792955347E-16, 21.00000000000001066, -27.21098080242150985 ) ) ;
#37464=( BOUNDED_CURVE ( )  B_SPLINE_CURVE ( 2, ( #7200, #14008, #10806, #23790, #6568, #32504, #26141, #19742, #32710 ),
 .UNSPECIFIED., .F., .F. ) 
 B_SPLINE_CURVE_WITH_KNOTS ( ( 3, 2, 2, 2, 3 ),
 ( 0.07291666666666667129, 0.07361111111111111327, 0.07499999999999999722, 0.07638888888888889506, 0.07708333333333333703 ),
 .UNSPECIFIED. ) 
 CURVE ( )  GEOMETRIC_REPRESENTATION_ITEM ( )  RATIONAL_B_SPLINE_CURVE ( ( 0.9330127018922194093, 0.9330127018922200755, 1.000000000000000000, 0.8660254037844387076, 1.000000000000000000, 0.8660254037844387076, 1.000000000000000000, 0.9330127018922194093, 0.9330127018922194093 ) ) 
 REPRESENTATION_ITEM ( '' )  );
#37470=CARTESIAN_POINT ( 'NONE',  ( 3.500000000000001332, 19.52072594216371115, -82.07139747004410424 ) ) ;
#37472=CARTESIAN_POINT ( 'NONE',  ( 4.286263797015737581E-16, 14.00000000000002487, -149.5231586289125687 ) ) ;
#37477=CARTESIAN_POINT ( 'NONE',  ( 3.500000000000001332, 19.52072594216371826, -135.0713974700441042 ) ) ;
#37478=AXIS2_PLACEMENT_3D ( 'NONE', #23423, #4054, #17039 ) ;
#37480=CARTESIAN_POINT ( 'NONE',  ( -3.310556943750000425, 19.41135094264167549, -138.8474391362327935 ) ) ;
#37481=CARTESIAN_POINT ( 'NONE',  ( 4.648177544792955347E-16, 21.00000000000001066, -40.90473080337742573 ) ) ;
#37483=CARTESIAN_POINT ( 'NONE',  ( -3.310556943750000425, 19.41135094264166838, -127.9349391362327850 ) ) ;
#37484=CARTESIAN_POINT ( 'NONE',  ( -3.310556943750000425, 19.41135094264166128, -56.93493913623279212 ) ) ;
#37485=ORIENTED_EDGE ( 'NONE', *, *, #29986, .F. ) ;
#37487=CARTESIAN_POINT ( 'NONE',  ( 2.474675557024783212E-16, 21.54145188432740810, -136.9047308033774186 ) ) ;
#37489=CARTESIAN_POINT ( 'NONE',  ( 3.500000000000001776, 19.52072594216371826, -129.3776474690881741 ) ) ;
#37490=CARTESIAN_POINT ( 'NONE',  ( 1.655278471875001101, 20.36702641396249547, -112.0974391362328078 ) ) ;
#37494=CARTESIAN_POINT ( 'NONE',  ( -1.749999999999999778, 20.53108891324555429, -82.12764746908818836 ) ) ;
#37496=CARTESIAN_POINT ( 'NONE',  ( 3.310556943750001313, 17.50000000000001421, -48.26410580289947205 ) ) ;
#37497=CARTESIAN_POINT ( 'NONE',  ( 3.310556943750001313, 17.50000000000002132, -104.3516058028994564 ) ) ;
#37498=CARTESIAN_POINT ( 'NONE',  ( -3.500000000000000000, 19.52072594216371826, -130.7380641367107614 ) ) ;
#37500=CARTESIAN_POINT ( 'NONE',  ( 1.655278471875001101, 20.36702641396249547, -121.1849391362327992 ) ) ;
#37503=CARTESIAN_POINT ( 'NONE',  ( 3.500000000000000000, 15.47927405783632793, -83.23806413671076143 ) ) ;
#37504=CARTESIAN_POINT ( 'NONE',  ( 1.749999999999998224, 14.46891108675448656, -130.3213974700441042 ) ) ;
#37505=CARTESIAN_POINT ( 'NONE',  ( 3.310556943750001313, 17.50000000000001421, -57.35160580289947063 ) ) ;
#37508=CARTESIAN_POINT ( 'NONE',  ( -1.655278471874999990, 20.36702641396249192, -82.01827246956614204 ) ) ;
#37513=DIRECTION ( 'NONE',  ( 0.000000000000000000, 1.000000000000000000, 0.000000000000000000 ) ) ;
#37515=CARTESIAN_POINT ( 'NONE',  ( 3.310556943750001313, 17.50000000000001066, -38.26410580289947916 ) ) ;
#37516=LINE ( 'NONE', #33907, #42064 ) ;
#37518=ORIENTED_EDGE ( 'NONE', *, *, #18320, .F. ) ;
#37521=CARTESIAN_POINT ( 'NONE',  ( 3.310556943750001313, 19.41135094264165772, -45.18077246956613635 ) ) ;
#37522=ORIENTED_EDGE ( 'NONE', *, *, #5292, .T. ) ;
#37523=ORIENTED_EDGE ( 'NONE', *, *, #22812, .F. ) ;
#37526=CARTESIAN_POINT ( 'NONE',  ( -3.500000000000002220, 15.47927405783633326, -104.5713974700440900 ) ) ;
#37528=CARTESIAN_POINT ( 'NONE',  ( -3.500000000000000888, 19.52072594216370405, -41.04431413575483845 ) ) ;
#37529=( BOUNDED_CURVE ( )  B_SPLINE_CURVE ( 2, ( #4029, #36140, #17232, #1275, #20416, #10636, #33606, #17646, #13823 ),
 .UNSPECIFIED., .F., .T. ) 
 B_SPLINE_CURVE_WITH_KNOTS ( ( 3, 2, 2, 2, 3 ),
 ( 0.7354166666666667185, 0.7361111111111111605, 0.7375000000000000444, 0.7388888888888889284, 0.7395833333333333703 ),
 .UNSPECIFIED. ) 
 CURVE ( )  GEOMETRIC_REPRESENTATION_ITEM ( )  RATIONAL_B_SPLINE_CURVE ( ( 0.9330127018922194093, 0.9330127018922194093, 1.000000000000000000, 0.8660254037844387076, 1.000000000000000000, 0.8660254037844387076, 1.000000000000000000, 0.9330127018922194093, 0.9330127018922194093 ) ) 
 REPRESENTATION_ITEM ( '' )  );
#37530=CARTESIAN_POINT ( 'NONE',  ( 0.000000000000000000, 21.00000000000002487, -149.5231586289125687 ) ) ;
#37532=CARTESIAN_POINT ( 'NONE',  ( -3.500000000000001332, 17.50000000000001776, -76.96098080242150274 ) ) ;
#37535=CARTESIAN_POINT ( 'NONE',  ( 3.310556943750001313, 17.50000000000001066, -24.35160580289946708 ) ) ;
#37537=CARTESIAN_POINT ( 'NONE',  ( 2.340729813953370519E-16, 21.32270188528331900, -129.0141058028994507 ) ) ;
#37540=CARTESIAN_POINT ( 'NONE',  ( 0.000000000000000000, 17.50000000000002487, -149.5231586289125687 ) ) ;
#37541=CARTESIAN_POINT ( 'NONE',  ( 1.655278471874998436, 14.63297358603754894, -121.5182724695661278 ) ) ;
#37543=CARTESIAN_POINT ( 'NONE',  ( 3.500000000000001332, 17.50000000000001066, -36.15473080337743284 ) ) ;
#37544=AXIS2_PLACEMENT_3D ( 'NONE', #27253, #7471, #40215 ) ;
#37545=CARTESIAN_POINT ( 'NONE',  ( -1.750000000000002220, 14.46891108675447768, -49.48806413671076854 ) ) ;
#37547=CARTESIAN_POINT ( 'NONE',  ( -3.310556943750000425, 19.41135094264167549, -136.9349391362327992 ) ) ;
#37548=CARTESIAN_POINT ( 'NONE',  ( -3.500000000000002220, 15.47927405783632615, -67.57139747004409003 ) ) ;
#37551=CARTESIAN_POINT ( 'NONE',  ( 1.655278471874998436, 14.63297358603754006, -52.51827246956612782 ) ) ;
#37553=CARTESIAN_POINT ( 'NONE',  ( -0.9378221735089291577, 21.00000000000001421, -73.16632260368299967 ) ) ;
#37554=VECTOR ( 'NONE', #26436, 1000.000000000000000 ) ;
#37555=CARTESIAN_POINT ( 'NONE',  ( -1.655278471874999990, 20.36702641396248836, -73.01827246956612782 ) ) ;
#37557=CARTESIAN_POINT ( 'NONE',  ( -3.310556943750001313, 17.50000000000002132, -104.7641058028994649 ) ) ;
#37558=CARTESIAN_POINT ( 'NONE',  ( -7.022189441860112050E-16, 13.67729811471672186, -71.51410580289947916 ) ) ;
#37560=CARTESIAN_POINT ( 'NONE',  ( -7.022189441860112050E-16, 13.67729811471672541, -95.60160580289945642 ) ) ;
#37563=CARTESIAN_POINT ( 'NONE',  ( 0.9378221735089300459, 21.00000000000002132, -117.2556390011600200 ) ) ;
#37564=CARTESIAN_POINT ( 'NONE',  ( 1.655278471875001101, 20.36702641396248836, -56.09743913623280065 ) ) ;
#37565=EDGE_CURVE ( 'NONE', #14314, #6275, #40931, .T. ) ;
#37566=CARTESIAN_POINT ( 'NONE',  ( -1.750000000000002220, 14.46891108675447413, -24.48806413671077209 ) ) ;
#37567=CARTESIAN_POINT ( 'NONE',  ( 1.655278471874998436, 14.63297358603754894, -109.4307724695661506 ) ) ;
#37568=EDGE_CURVE ( 'NONE', #9218, #12140, #13237, .T. ) ;
#37569=VERTEX_POINT ( 'NONE', #14570 ) ;
#37574=CARTESIAN_POINT ( 'NONE',  ( -3.310556943750001313, 17.50000000000001421, -64.76410580289946495 ) ) ;
#37576=EDGE_LOOP ( 'NONE', ( #1120, #40642, #25126, #7661 ) ) ;
#37578=CARTESIAN_POINT ( 'NONE',  ( -1.394453263437886604E-15, 14.00000000000001421, -69.71098080242150274 ) ) ;
#37585=CARTESIAN_POINT ( 'NONE',  ( -3.310556943750001313, 17.50000000000002487, -130.7641058028994507 ) ) ;
#37586=CARTESIAN_POINT ( 'NONE',  ( -1.749999999999999778, 20.53108891324555785, -116.1276474690881741 ) ) ;
#37587=( BOUNDED_CURVE ( )  B_SPLINE_CURVE ( 2, ( #37651, #24690, #11090, #4903, #1305, #24074, #40219, #14894, #21074 ),
 .UNSPECIFIED., .F., .F. ) 
 B_SPLINE_CURVE_WITH_KNOTS ( ( 3, 2, 2, 2, 3 ),
 ( 0.4229166666666666630, 0.4236111111111111049, 0.4249999999999999889, 0.4263888888888888729, 0.4270833333333333148 ),
 .UNSPECIFIED. ) 
 CURVE ( )  GEOMETRIC_REPRESENTATION_ITEM ( )  RATIONAL_B_SPLINE_CURVE ( ( 0.9330127018922194093, 0.9330127018922194093, 1.000000000000000000, 0.8660254037844387076, 1.000000000000000000, 0.8660254037844387076, 1.000000000000000000, 0.9330127018922194093, 0.9330127018922194093 ) ) 
 REPRESENTATION_ITEM ( '' )  );
#37588=EDGE_CURVE ( 'NONE', #22244, #8756, #4296, .T. ) ;
#37589=CARTESIAN_POINT ( 'NONE',  ( -7.022189441860112050E-16, 13.67729811471671475, -37.60160580289947063 ) ) ;
#37590=CARTESIAN_POINT ( 'NONE',  ( -3.310556943750001313, 17.50000000000001066, -30.85160580289945997 ) ) ;
#37591=CARTESIAN_POINT ( 'NONE',  ( 1.655278471874998436, 14.63297358603754716, -95.51827246956612782 ) ) ;
#37592=CARTESIAN_POINT ( 'NONE',  ( -1.750000000000002220, 14.46891108675447590, -26.48806413671075788 ) ) ;
#37593=VERTEX_POINT ( 'NONE', #7267 ) ;
#37595=CARTESIAN_POINT ( 'NONE',  ( 2.340729813953370519E-16, 21.32270188528332255, -138.1016058028994564 ) ) ;
#37596=CARTESIAN_POINT ( 'NONE',  ( 3.405278471875001323, 17.50000000000002487, -143.4062933026604583 ) ) ;
#37597=CARTESIAN_POINT ( 'NONE',  ( 1.750000000000001110, 20.53108891324555429, -98.29431413575484555 ) ) ;
#37598=CARTESIAN_POINT ( 'NONE',  ( 3.310556943750001313, 19.41135094264166128, -57.18077246956614346 ) ) ;
#37599=CARTESIAN_POINT ( 'NONE',  ( -1.394453263437886604E-15, 14.00000000000001421, -64.71098080242150274 ) ) ;
#37600=CARTESIAN_POINT ( 'NONE',  ( 3.500000000000000000, 15.47927405783632615, -87.23806413671076143 ) ) ;
#37601=CARTESIAN_POINT ( 'NONE',  ( 3.310556943749999981, 15.58864905735836714, -72.43493913623278502 ) ) ;
#37604=CARTESIAN_POINT ( 'NONE',  ( 4.648177544792955347E-16, 21.00000000000001421, -48.21098080242150274 ) ) ;
#37605=CARTESIAN_POINT ( 'NONE',  ( -3.500000000000001332, 17.50000000000001421, -48.96098080242150274 ) ) ;
#37606=CARTESIAN_POINT ( 'NONE',  ( 3.310556943750001313, 17.50000000000002132, -122.2641058028994792 ) ) ;
#37609=VERTEX_POINT ( 'NONE', #26622 ) ;
#37610=CARTESIAN_POINT ( 'NONE',  ( -1.750000000000002220, 14.46891108675448656, -112.4880641367107614 ) ) ;
#37613=CARTESIAN_POINT ( 'NONE',  ( 3.500000000000001332, 19.52072594216370405, -37.37764746908816704 ) ) ;
#37616=CARTESIAN_POINT ( 'NONE',  ( 3.310556943749999981, 15.58864905735836714, -73.34743913623280775 ) ) ;
#37617=EDGE_CURVE ( 'NONE', #3213, #8887, #31730, .T. ) ;
#37621=EDGE_LOOP ( 'NONE', ( #39541, #17959, #21303, #2353 ) ) ;
#37623=CARTESIAN_POINT ( 'NONE',  ( 4.648177544792955347E-16, 21.00000000000001066, -34.90473080337743284 ) ) ;
#37624=CARTESIAN_POINT ( 'NONE',  ( 3.500000000000001332, 17.50000000000001776, -88.46098080242151696 ) ) ;
#37625=CARTESIAN_POINT ( 'NONE',  ( 3.310556943750001313, 19.41135094264166483, -78.18077246956613635 ) ) ;
#37632=VERTEX_POINT ( 'NONE', #666 ) ;
#37633=DIRECTION ( 'NONE',  ( 0.000000000000000000, -1.259100132267607459E-16, 1.000000000000000000 ) ) ;
#37634=CARTESIAN_POINT ( 'NONE',  ( 2.340729813953370519E-16, 21.32270188528330834, -50.10160580289946353 ) ) ;
#37635=CARTESIAN_POINT ( 'NONE',  ( 1.655278471874998436, 14.63297358603754894, -110.5182724695661420 ) ) ;
#37636=ORIENTED_EDGE ( 'NONE', *, *, #24318, .F. ) ;
#37638=CARTESIAN_POINT ( 'NONE',  ( -1.655278471874999990, 20.36702641396248481, -36.93077246956613635 ) ) ;
#37639=CARTESIAN_POINT ( 'NONE',  ( -3.310556943750000425, 19.41135094264166128, -61.93493913623280633 ) ) ;
#37640=CARTESIAN_POINT ( 'NONE',  ( 1.750000000000001110, 20.53108891324555785, -114.2943141357548313 ) ) ;
#37643=CARTESIAN_POINT ( 'NONE',  ( -3.310556943750002645, 15.58864905735837425, -95.68077246956615056 ) ) ;
#37647=CARTESIAN_POINT ( 'NONE',  ( 3.500000000000001332, 17.50000000000001421, -65.46098080242150274 ) ) ;
#37649=CARTESIAN_POINT ( 'NONE',  ( -3.310556943750000425, 19.41135094264165772, -32.84743913623280775 ) ) ;
#37650=CARTESIAN_POINT ( 'NONE',  ( -3.500000000000002220, 15.47927405783632260, -53.57139747004409713 ) ) ;
#37651=CARTESIAN_POINT ( 'NONE',  ( -1.394453263437886604E-15, 14.00000000000001776, -92.71098080242150274 ) ) ;
#37652=CARTESIAN_POINT ( 'NONE',  ( -7.022189441860112050E-16, 13.67729811471672541, -107.6016058028994564 ) ) ;
#37653=CARTESIAN_POINT ( 'NONE',  ( -3.310556943750000425, 19.41135094264166128, -39.93493913623280633 ) ) ;
#37655=CARTESIAN_POINT ( 'NONE',  ( 1.749999999999998224, 14.46891108675448656, -135.6276474690881741 ) ) ;
#37660=CARTESIAN_POINT ( 'NONE',  ( 0.9378221735089300459, 21.00000000000001421, -48.25563900116002714 ) ) ;
#37662=CARTESIAN_POINT ( 'NONE',  ( 1.655278471874998436, 14.63297358603754539, -85.43077246956613635 ) ) ;
#37667=CARTESIAN_POINT ( 'NONE',  ( -1.394453263437886604E-15, 14.00000000000001066, -50.40473080337741862 ) ) ;
#37668=VERTEX_POINT ( 'NONE', #17266 ) ;
#37674=CARTESIAN_POINT ( 'NONE',  ( -1.749999999999999778, 20.53108891324555429, -78.82139747004410424 ) ) ;
#37675=ORIENTED_EDGE ( 'NONE', *, *, #28767, .T. ) ;
#37679=CARTESIAN_POINT ( 'NONE',  ( 4.648177544792955347E-16, 21.00000000000001776, -90.21098080242150274 ) ) ;
#37684=CARTESIAN_POINT ( 'NONE',  ( 1.750000000000001110, 20.53108891324556140, -139.9880641367107614 ) ) ;
#37685=CARTESIAN_POINT ( 'NONE',  ( 1.655278471875001101, 20.36702641396249902, -137.0974391362328220 ) ) ;
#37686=CARTESIAN_POINT ( 'NONE',  ( 3.500000000000001332, 19.52072594216371826, -104.0713974700440900 ) ) ;
#37689=CARTESIAN_POINT ( 'NONE',  ( -3.500000000000000000, 19.52072594216370760, -63.73806413671076143 ) ) ;
#37690=CARTESIAN_POINT ( 'NONE',  ( -1.655278471874999990, 20.36702641396249547, -124.0182724695661278 ) ) ;
#37691=CARTESIAN_POINT ( 'NONE',  ( 2.340729813953370519E-16, 21.32270188528330834, -57.10160580289947063 ) ) ;
#37692=ORIENTED_EDGE ( 'NONE', *, *, #35227, .T. ) ;
#37694=CARTESIAN_POINT ( 'NONE',  ( -3.500000000000002220, 15.47927405783633503, -138.5713974700441042 ) ) ;
#37696=SHAPE_REPRESENTATION_RELATIONSHIP ( 'NONE' , 'NONE' ,  #38314, #25429 ) ;
#37698=CARTESIAN_POINT ( 'NONE',  ( 3.310556943749999981, 15.58864905735836714, -78.43493913623278502 ) ) ;
#37699=CARTESIAN_POINT ( 'NONE',  ( 1.750000000000001110, 20.53108891324555785, -126.2943141357548456 ) ) ;
#37700=CARTESIAN_POINT ( 'NONE',  ( 3.310556943750001313, 17.50000000000002132, -113.2641058028994792 ) ) ;
#37704=CARTESIAN_POINT ( 'NONE',  ( 1.750000000000001110, 20.53108891324555429, -82.29431413575483134 ) ) ;
#37707=CARTESIAN_POINT ( 'NONE',  ( 3.310556943749999981, 15.58864905735836182, -46.34743913623280775 ) ) ;
#37708=CARTESIAN_POINT ( 'NONE',  ( 3.310556943750001313, 17.50000000000002132, -106.3516058028994564 ) ) ;
#37709=( BOUNDED_CURVE ( )  B_SPLINE_CURVE ( 2, ( #5927, #31448, #25505, #28465, #18900, #9333, #15303, #6135, #25078 ),
 .UNSPECIFIED., .F., .T. ) 
 B_SPLINE_CURVE_WITH_KNOTS ( ( 3, 2, 2, 2, 3 ),
 ( 0.7854166666666666519, 0.7861111111111110938, 0.7874999999999999778, 0.7888888888888888618, 0.7895833333333333037 ),
 .UNSPECIFIED. ) 
 CURVE ( )  GEOMETRIC_REPRESENTATION_ITEM ( )  RATIONAL_B_SPLINE_CURVE ( ( 0.9330127018922194093, 0.9330127018922194093, 1.000000000000000000, 0.8660254037844387076, 1.000000000000000000, 0.8660254037844387076, 1.000000000000000000, 0.9330127018922194093, 0.9330127018922194093 ) ) 
 REPRESENTATION_ITEM ( '' )  );
#37710=CARTESIAN_POINT ( 'NONE',  ( -1.394453263437886604E-15, 14.00000000000002132, -130.4047308033774186 ) ) ;
#37711=CARTESIAN_POINT ( 'NONE',  ( -1.394453263437886604E-15, 14.00000000000001066, -42.40473080337742573 ) ) ;
#37713=CARTESIAN_POINT ( 'NONE',  ( -7.022189441860112050E-16, 13.67729811471672896, -120.6016058028994564 ) ) ;
#37714=EDGE_CURVE ( 'NONE', #27788, #18643, #14359, .T. ) ;
#37717=CARTESIAN_POINT ( 'NONE',  ( 4.648177544792955347E-16, 21.00000000000001776, -82.90473080337743284 ) ) ;
#37718=CARTESIAN_POINT ( 'NONE',  ( 0.9378221735089281585, 14.00000000000002309, -130.3600726046389013 ) ) ;
#37719=CARTESIAN_POINT ( 'NONE',  ( 0.000000000000000000, 21.00000000000002487, -149.5231586289125687 ) ) ;
#37720=CARTESIAN_POINT ( 'NONE',  ( -7.022189441860112050E-16, 13.67729811471671830, -57.60160580289946353 ) ) ;
#37722=CARTESIAN_POINT ( 'NONE',  ( -7.022189441860112050E-16, 13.67729811471672186, -72.60160580289947063 ) ) ;
#37723=CYLINDRICAL_SURFACE ( 'NONE', #27185, 3.499999999999999556 ) ;
#37724=DIRECTION ( 'NONE',  ( -0.000000000000000000, 1.259100132267607459E-16, -1.000000000000000000 ) ) ;
#37725=CARTESIAN_POINT ( 'NONE',  ( 4.648177544792955347E-16, 21.00000000000001776, -80.90473080337743284 ) ) ;
#37728=CARTESIAN_POINT ( 'NONE',  ( 3.310556943749999981, 15.58864905735836182, -42.34743913623280775 ) ) ;
#37731=ORIENTED_EDGE ( 'NONE', *, *, #7671, .T. ) ;
#37733=CARTESIAN_POINT ( 'NONE',  ( -3.310556943750002645, 15.58864905735836714, -48.68077246956615056 ) ) ;
#37734=ORIENTED_EDGE ( 'NONE', *, *, #6921, .F. ) ;
#37736=DIRECTION ( 'NONE',  ( 0.000000000000000000, 1.000000000000000000, 0.000000000000000000 ) ) ;
#37737=DIRECTION ( 'NONE',  ( 0.000000000000000000, 1.000000000000000000, 0.000000000000000000 ) ) ;
#37740=CARTESIAN_POINT ( 'NONE',  ( 0.9378221735089300459, 21.00000000000002132, -112.9493890021159643 ) ) ;
#37741=CARTESIAN_POINT ( 'NONE',  ( 0.9378221735089300459, 21.00000000000001776, -89.25563900116003424 ) ) ;
#37742=CARTESIAN_POINT ( 'NONE',  ( -3.500000000000001332, 17.50000000000001066, -37.96098080242150985 ) ) ;
#37744=CARTESIAN_POINT ( 'NONE',  ( -1.749999999999999778, 20.53108891324555429, -77.12764746908817415 ) ) ;
#37747=CARTESIAN_POINT ( 'NONE',  ( 1.655278471874998436, 14.63297358603753828, -26.51827246956613138 ) ) ;
#37749=CARTESIAN_POINT ( 'NONE',  ( -1.655278471875002211, 14.63297358603755249, -126.5974391362328078 ) ) ;
#37750=VECTOR ( 'NONE', #38547, 1000.000000000000000 ) ;
#37754=CARTESIAN_POINT ( 'NONE',  ( 3.500000000000001332, 17.50000000000001776, -94.15473080337744705 ) ) ;
#37755=CARTESIAN_POINT ( 'NONE',  ( 3.310556943750001313, 19.41135094264166838, -120.2682724695661278 ) ) ;
#37757=CARTESIAN_POINT ( 'NONE',  ( 2.474675557024783212E-16, 21.54145188432739033, -38.90473080337743994 ) ) ;
#37760=CARTESIAN_POINT ( 'NONE',  ( 1.655278471875001101, 20.36702641396249902, -140.1849391362327708 ) ) ;
#37762=CARTESIAN_POINT ( 'NONE',  ( -1.655278471874999990, 20.36702641396248836, -50.01827246956614204 ) ) ;
#37765=CARTESIAN_POINT ( 'NONE',  ( 3.310556943750001313, 17.50000000000001776, -75.35160580289947063 ) ) ;
#37767=CARTESIAN_POINT ( 'NONE',  ( -1.655278471875002211, 14.63297358603754894, -103.5974391362328220 ) ) ;
#37768=CARTESIAN_POINT ( 'NONE',  ( 1.655278471874998436, 14.63297358603754361, -72.43077246956613635 ) ) ;
#37770=CARTESIAN_POINT ( 'NONE',  ( 1.655278471874998436, 14.63297358603754539, -92.51827246956611361 ) ) ;
#37772=CARTESIAN_POINT ( 'NONE',  ( 3.500000000000001332, 17.50000000000001421, -49.46098080242150274 ) ) ;
#37775=CARTESIAN_POINT ( 'NONE',  ( 3.310556943749999981, 15.58864905735836537, -58.34743913623280065 ) ) ;
#37776=CARTESIAN_POINT ( 'NONE',  ( 7.785697387528201340E-15, 14.00000000000002487, -137.4047308033774470 ) ) ;
#37777=CARTESIAN_POINT ( 'NONE',  ( 3.310556943750001313, 19.41135094264166838, -113.1807724695661221 ) ) ;
#37778=ORIENTED_EDGE ( 'NONE', *, *, #11191, .F. ) ;
#37779=ORIENTED_EDGE ( 'NONE', *, *, #9811, .F. ) ;
#37781=EDGE_LOOP ( 'NONE', ( #20795, #8113, #26963, #28920 ) ) ;
#37783=CARTESIAN_POINT ( 'NONE',  ( -3.310556943750002645, 15.58864905735836892, -64.68077246956615056 ) ) ;
#37784=( BOUNDED_CURVE ( )  B_SPLINE_CURVE ( 2, ( #2975, #39775, #25316, #41911, #38915, #15537, #41692, #22533, #32110 ),
 .UNSPECIFIED., .F., .T. ) 
 B_SPLINE_CURVE_WITH_KNOTS ( ( 3, 2, 2, 2, 3 ),
 ( 0.7729166666666666963, 0.7736111111111111382, 0.7750000000000000222, 0.7763888888888889062, 0.7770833333333333481 ),
 .UNSPECIFIED. ) 
 CURVE ( )  GEOMETRIC_REPRESENTATION_ITEM ( )  RATIONAL_B_SPLINE_CURVE ( ( 0.9330127018922194093, 0.9330127018922194093, 1.000000000000000000, 0.8660254037844387076, 1.000000000000000000, 0.8660254037844387076, 1.000000000000000000, 0.9330127018922194093, 0.9330127018922194093 ) ) 
 REPRESENTATION_ITEM ( '' )  );
#37787=CARTESIAN_POINT ( 'NONE',  ( 0.9378221735089281585, 14.00000000000000888, -30.66632260368298901 ) ) ;
#37790=DIRECTION ( 'NONE',  ( -0.000000000000000000, 1.259100132267607459E-16, -1.000000000000000000 ) ) ;
#37791=VERTEX_POINT ( 'NONE', #31267 ) ;
#37792=CARTESIAN_POINT ( 'NONE',  ( -3.500000000000000000, 19.52072594216370760, -55.04431413575484555 ) ) ;
#37793=CARTESIAN_POINT ( 'NONE',  ( -1.655278471875002211, 14.63297358603755249, -128.5974391362328220 ) ) ;
#37794=CARTESIAN_POINT ( 'NONE',  ( -7.460324959392693302E-14, 21.00000000000002132, -103.2109808024215027 ) ) ;
#37795=CARTESIAN_POINT ( 'NONE',  ( 3.310556943749999981, 15.58864905735836182, -40.43493913623280633 ) ) ;
#37796=CARTESIAN_POINT ( 'NONE',  ( -1.655278471874999990, 20.36702641396248481, -32.01827246956613493 ) ) ;
#37797=CARTESIAN_POINT ( 'NONE',  ( -1.655278471874999990, 20.36702641396249192, -95.01827246956612782 ) ) ;
#37798=CARTESIAN_POINT ( 'NONE',  ( 1.749999999999998224, 14.46891108675447235, -24.32139747004409713 ) ) ;
#37800=EDGE_CURVE ( 'NONE', #6800, #21422, #17597, .T. ) ;
#37802=CARTESIAN_POINT ( 'NONE',  ( 2.340729813953370519E-16, 21.32270188528332255, -140.1016058028994564 ) ) ;
#37803=LINE ( 'NONE', #37596, #16642 ) ;
#37804=CARTESIAN_POINT ( 'NONE',  ( 3.500000000000001332, 17.50000000000001776, -87.15473080337743284 ) ) ;
#37805=CARTESIAN_POINT ( 'NONE',  ( -7.022189441860112050E-16, 13.67729811471671830, -57.51410580289947916 ) ) ;
#37806=CARTESIAN_POINT ( 'NONE',  ( -1.394453263437886604E-15, 14.00000000000002132, -132.4047308033774186 ) ) ;
#37807=CARTESIAN_POINT ( 'NONE',  ( 1.749999999999998224, 14.46891108675448123, -81.32139747004410424 ) ) ;
#37808=CARTESIAN_POINT ( 'NONE',  ( -1.655278471875002211, 14.63297358603754361, -62.68493913623279923 ) ) ;
#37811=CARTESIAN_POINT ( 'NONE',  ( -3.500000000000000000, 19.52072594216371115, -91.04431413575484555 ) ) ;
#37813=CARTESIAN_POINT ( 'NONE',  ( -3.310556943750000425, 19.41135094264166838, -119.8474391362328078 ) ) ;
#37816=ORIENTED_EDGE ( 'NONE', *, *, #25079, .T. ) ;
#37817=CARTESIAN_POINT ( 'NONE',  ( 3.500000000000001332, 17.50000000000002132, -114.1547308033774328 ) ) ;
#37818=CARTESIAN_POINT ( 'NONE',  ( 4.648177544792955347E-16, 21.00000000000001776, -100.2109808024215027 ) ) ;
#37819=CARTESIAN_POINT ( 'NONE',  ( -3.500000000000001332, 17.50000000000001776, -82.65473080337743284 ) ) ;
#37820=LINE ( 'NONE', #37205, #24453 ) ;
#37821=CARTESIAN_POINT ( 'NONE',  ( -1.394453263437886604E-15, 14.00000000000002132, -120.7109808024215170 ) ) ;
#37823=CARTESIAN_POINT ( 'NONE',  ( -1.655278471875002211, 14.63297358603754539, -69.59743913623280775 ) ) ;
#37825=EDGE_CURVE ( 'NONE', #12038, #22032, #18702, .T. ) ;
#37826=CARTESIAN_POINT ( 'NONE',  ( 1.749999999999998224, 14.46891108675447946, -69.62764746908817415 ) ) ;
#37828=VERTEX_POINT ( 'NONE', #30440 ) ;
#37829=CARTESIAN_POINT ( 'NONE',  ( 3.310556943749999981, 15.58864905735836004, -25.34743913623280065 ) ) ;
#37831=CARTESIAN_POINT ( 'NONE',  ( 1.655278471874998436, 14.63297358603754361, -80.43077246956615056 ) ) ;
#37834=( BOUNDED_CURVE ( )  B_SPLINE_CURVE ( 2, ( #25575, #35135, #19390, #32362, #29153, #13012, #16420, #25992, #6826 ),
 .UNSPECIFIED., .F., .T. ) 
 B_SPLINE_CURVE_WITH_KNOTS ( ( 3, 2, 2, 2, 3 ),
 ( 0.1395833333333333370, 0.1402777777777777790, 0.1416666666666666630, 0.1430555555555555469, 0.1437499999999999889 ),
 .UNSPECIFIED. ) 
 CURVE ( )  GEOMETRIC_REPRESENTATION_ITEM ( )  RATIONAL_B_SPLINE_CURVE ( ( 0.9330127018922194093, 0.9330127018922194093, 1.000000000000000000, 0.8660254037844387076, 1.000000000000000000, 0.8660254037844387076, 1.000000000000000000, 0.9330127018922194093, 0.9330127018922194093 ) ) 
 REPRESENTATION_ITEM ( '' )  );
#37837=CARTESIAN_POINT ( 'NONE',  ( 4.648177544792955347E-16, 21.00000000000001421, -70.90473080337743284 ) ) ;
#37838=VERTEX_POINT ( 'NONE', #24078 ) ;
#37840=CARTESIAN_POINT ( 'NONE',  ( 3.310556943750001313, 19.41135094264166128, -48.26827246956613493 ) ) ;
#37841=CARTESIAN_POINT ( 'NONE',  ( 3.310556943749999981, 15.58864905735837247, -111.4349391362327850 ) ) ;
#37844=ADVANCED_FACE ( 'NONE', ( #1723 ), #7904, .T. ) ;
#37846=CARTESIAN_POINT ( 'NONE',  ( -1.655278471875002211, 14.63297358603754006, -36.59743913623281486 ) ) ;
#37847=CARTESIAN_POINT ( 'NONE',  ( 3.310556943749999981, 15.58864905735836537, -62.43493913623279923 ) ) ;
#37848=CARTESIAN_POINT ( 'NONE',  ( -3.500000000000000888, 19.52072594216371826, -115.0443141357548313 ) ) ;
#37850=CARTESIAN_POINT ( 'NONE',  ( -7.022189441860112050E-16, 13.67729811471672363, -90.51410580289946495 ) ) ;
#37852=CARTESIAN_POINT ( 'NONE',  ( 0.000000000000000000, 21.00000000000002487, -149.5231586289125687 ) ) ;
#37854=CARTESIAN_POINT ( 'NONE',  ( 3.500000000000001776, 19.52072594216370760, -66.37764746908817415 ) ) ;
#37855=CARTESIAN_POINT ( 'NONE',  ( -1.749999999999999778, 20.53108891324555074, -72.12764746908817415 ) ) ;
#37856=CARTESIAN_POINT ( 'NONE',  ( 3.310556943750001313, 19.41135094264165772, -25.18077246956613635 ) ) ;
#37857=CARTESIAN_POINT ( 'NONE',  ( 3.500000000000000000, 15.47927405783632260, -56.23806413671076143 ) ) ;
#37858=CARTESIAN_POINT ( 'NONE',  ( 3.500000000000000000, 15.47927405783632615, -77.54431413575484555 ) ) ;
#37859=CARTESIAN_POINT ( 'NONE',  ( -1.655278471874999990, 20.36702641396249547, -105.0182724695661278 ) ) ;
#37860=CARTESIAN_POINT ( 'NONE',  ( -3.310556943750000425, 19.41135094264166128, -37.93493913623280633 ) ) ;
#37862=CARTESIAN_POINT ( 'NONE',  ( 3.500000000000000000, 15.47927405783633503, -135.5443141357548598 ) ) ;
#37865=CARTESIAN_POINT ( 'NONE',  ( -1.750000000000002220, 14.46891108675447768, -49.79431413575484555 ) ) ;
#37867=CARTESIAN_POINT ( 'NONE',  ( -1.655278471875002211, 14.63297358603754716, -88.59743913623280775 ) ) ;
#37868=CARTESIAN_POINT ( 'NONE',  ( 0.9378221735089300459, 21.00000000000002132, -116.9493890021159501 ) ) ;
#37870=ORIENTED_EDGE ( 'NONE', *, *, #7387, .F. ) ;
#37872=CARTESIAN_POINT ( 'NONE',  ( -1.394453263437886604E-15, 14.00000000000002132, -109.7109808024215170 ) ) ;
#37876=CARTESIAN_POINT ( 'NONE',  ( 3.310556943750001313, 17.50000000000001776, -95.26410580289946495 ) ) ;
#37878=EDGE_LOOP ( 'NONE', ( #22243, #28357, #25707 ) ) ;
#37888=CARTESIAN_POINT ( 'NONE',  ( 3.500000000000001332, 19.52072594216371115, -91.07139747004409003 ) ) ;
#37890=CARTESIAN_POINT ( 'NONE',  ( 1.655278471875001101, 20.36702641396249902, -136.0974391362328220 ) ) ;
#37893=EDGE_CURVE ( 'NONE', #11163, #12311, #26288, .T. ) ;
#37894=CARTESIAN_POINT ( 'NONE',  ( -1.750000000000002220, 14.46891108675447946, -63.48806413671076143 ) ) ;
#37895=CARTESIAN_POINT ( 'NONE',  ( 3.310556943750001313, 19.41135094264166838, -123.2682724695661278 ) ) ;
#37896=CARTESIAN_POINT ( 'NONE',  ( 3.310556943750001313, 19.41135094264166128, -56.26827246956613493 ) ) ;
#37900=CARTESIAN_POINT ( 'NONE',  ( -1.749999999999999778, 20.53108891324556140, -133.8213974700441042 ) ) ;
#37903=EDGE_CURVE ( 'NONE', #4923, #33342, #31893, .T. ) ;
#37905=CARTESIAN_POINT ( 'NONE',  ( -3.310556943750002645, 15.58864905735837070, -74.76827246956612782 ) ) ;
#37906=CARTESIAN_POINT ( 'NONE',  ( 3.500000000000001332, 17.50000000000002132, -128.4609808024215170 ) ) ;
#37907=CARTESIAN_POINT ( 'NONE',  ( 3.310556943749999981, 15.58864905735837247, -113.3474391362328220 ) ) ;
#37910=CARTESIAN_POINT ( 'NONE',  ( -3.500000000000001332, 17.50000000000001776, -81.96098080242150274 ) ) ;
#37911=CARTESIAN_POINT ( 'NONE',  ( 4.648177544792955347E-16, 21.00000000000001421, -69.21098080242148853 ) ) ;
#37912=CARTESIAN_POINT ( 'NONE',  ( -3.310556943750001313, 17.50000000000001066, -45.76410580289946495 ) ) ;
#37913=CARTESIAN_POINT ( 'NONE',  ( 3.310556943750001313, 19.41135094264166483, -99.26827246956612782 ) ) ;
#37914=CARTESIAN_POINT ( 'NONE',  ( 4.648177544792955347E-16, 21.00000000000002487, -130.9047308033774186 ) ) ;
#37915=CARTESIAN_POINT ( 'NONE',  ( 3.500000000000000000, 15.47927405783632082, -39.54431413575484555 ) ) ;
#37917=CARTESIAN_POINT ( 'NONE',  ( 2.340729813953370519E-16, 21.32270188528331900, -124.1016058028994564 ) ) ;
#37921=DIRECTION ( 'NONE',  ( -0.000000000000000000, 1.259100132267607459E-16, -1.000000000000000000 ) ) ;
#37923=CARTESIAN_POINT ( 'NONE',  ( -1.394453263437886604E-15, 14.00000000000001421, -54.40473080337742573 ) ) ;
#37926=CARTESIAN_POINT ( 'NONE',  ( 1.655278471874998436, 14.63297358603754361, -73.51827246956612782 ) ) ;
#37927=CARTESIAN_POINT ( 'NONE',  ( -1.394453263437886604E-15, 14.00000000000001066, -47.40473080337742573 ) ) ;
#37928=CARTESIAN_POINT ( 'NONE',  ( -1.394453263437886604E-15, 14.00000000000001776, -102.4047308033774186 ) ) ;
#37933=CARTESIAN_POINT ( 'NONE',  ( -1.655278471874999990, 20.36702641396248481, -36.93077246956613635 ) ) ;
#37939=CARTESIAN_POINT ( 'NONE',  ( -1.655278471874999990, 20.36702641396248836, -46.93077246956614346 ) ) ;
#37947=CYLINDRICAL_SURFACE ( 'NONE', #15286, 3.499999999999999556 ) ;
#37948=CARTESIAN_POINT ( 'NONE',  ( -7.424026671074350129E-16, 13.45854811567263098, -36.71098080242150985 ) ) ;
#37949=CARTESIAN_POINT ( 'NONE',  ( 3.500000000000001332, 17.50000000000001776, -86.46098080242151696 ) ) ;
#37951=( BOUNDED_CURVE ( )  B_SPLINE_CURVE ( 2, ( #25758, #29343, #22768, #19159, #32129, #6604, #18950, #19569, #2995 ),
 .UNSPECIFIED., .F., .T. ) 
 B_SPLINE_CURVE_WITH_KNOTS ( ( 3, 2, 2, 2, 3 ),
 ( 0.6395833333333332815, 0.6402777777777777235, 0.6416666666666667185, 0.6430555555555556024, 0.6437500000000000444 ),
 .UNSPECIFIED. ) 
 CURVE ( )  GEOMETRIC_REPRESENTATION_ITEM ( )  RATIONAL_B_SPLINE_CURVE ( ( 0.9330127018922194093, 0.9330127018922194093, 1.000000000000000000, 0.8660254037844387076, 1.000000000000000000, 0.8660254037844387076, 1.000000000000000000, 0.9330127018922194093, 0.9330127018922194093 ) ) 
 REPRESENTATION_ITEM ( '' )  );
#37952=( BOUNDED_CURVE ( )  B_SPLINE_CURVE ( 2, ( #23522, #36484, #20318, #33285, #13727, #4150, #755, #17134, #26707 ),
 .UNSPECIFIED., .F., .T. ) 
 B_SPLINE_CURVE_WITH_KNOTS ( ( 3, 2, 2, 2, 3 ),
 ( 0.2895833333333333592, 0.2902777777777778012, 0.2916666666666666852, 0.2930555555555555691, 0.2937500000000000111 ),
 .UNSPECIFIED. ) 
 CURVE ( )  GEOMETRIC_REPRESENTATION_ITEM ( )  RATIONAL_B_SPLINE_CURVE ( ( 0.9330127018922194093, 0.9330127018922220739, 1.000000000000000000, 0.8660254037844387076, 1.000000000000000000, 0.8660254037844387076, 1.000000000000000000, 0.9330127018922194093, 0.9330127018922194093 ) ) 
 REPRESENTATION_ITEM ( '' )  );
#37953=CARTESIAN_POINT ( 'NONE',  ( 4.648177544792955347E-16, 21.00000000000001776, -96.21098080242150274 ) ) ;
#37955=CARTESIAN_POINT ( 'NONE',  ( 2.340729813953370519E-16, 21.32270188528330479, -26.10160580289947063 ) ) ;
#37956=CARTESIAN_POINT ( 'NONE',  ( 0.000000000000000000, 21.00000000000002487, -149.5231586289125687 ) ) ;
#37957=CARTESIAN_POINT ( 'NONE',  ( -7.022189441860112050E-16, 13.67729811471672718, -127.5141058028994649 ) ) ;
#37960=CARTESIAN_POINT ( 'NONE',  ( -0.9378221735089291577, 21.00000000000001776, -76.86007260463890134 ) ) ;
#37961=CARTESIAN_POINT ( 'NONE',  ( -3.310556943750002645, 15.58864905735837780, -120.7682724695661420 ) ) ;
#37962=CARTESIAN_POINT ( 'NONE',  ( 1.743066579297357930E-14, 14.00000000000002132, -134.4047308033774186 ) ) ;
#37963=CARTESIAN_POINT ( 'NONE',  ( -1.750000000000002220, 14.46891108675447590, -36.48806413671076854 ) ) ;
#37966=CARTESIAN_POINT ( 'NONE',  ( 2.340729813953370519E-16, 21.32270188528332255, -140.1016058028994564 ) ) ;
#37967=DIRECTION ( 'NONE',  ( -0.000000000000000000, 1.259100132267607459E-16, -1.000000000000000000 ) ) ;
#37968=CARTESIAN_POINT ( 'NONE',  ( -1.655278471874999990, 20.36702641396248836, -51.01827246956612782 ) ) ;
#37971=CARTESIAN_POINT ( 'NONE',  ( 3.310556943749999981, 15.58864905735836714, -73.43493913623279923 ) ) ;
#37973=CARTESIAN_POINT ( 'NONE',  ( -3.310556943750001313, 17.50000000000001776, -98.76410580289947916 ) ) ;
#37974=CARTESIAN_POINT ( 'NONE',  ( 3.310556943750001313, 17.50000000000001421, -71.26410580289947916 ) ) ;
#37976=CARTESIAN_POINT ( 'NONE',  ( -1.655278471875002211, 14.63297358603754716, -91.68493913623279923 ) ) ;
#37978=CARTESIAN_POINT ( 'NONE',  ( 0.9378221735089281585, 14.00000000000001066, -49.66632260368299256 ) ) ;
#37979=CARTESIAN_POINT ( 'NONE',  ( -3.500000000000002220, 15.47927405783632970, -84.87764746908817415 ) ) ;
#37981=CARTESIAN_POINT ( 'NONE',  ( -1.655278471874999990, 20.36702641396248836, -54.93077246956613635 ) ) ;
#37983=CARTESIAN_POINT ( 'NONE',  ( 1.655278471875001101, 20.36702641396249547, -112.0974391362328078 ) ) ;
#37985=ORIENTED_EDGE ( 'NONE', *, *, #23614, .T. ) ;
#37987=VERTEX_POINT ( 'NONE', #25108 ) ;
#37989=CARTESIAN_POINT ( 'NONE',  ( -1.655278471875002211, 14.63297358603754361, -64.59743913623280775 ) ) ;
#37995=CYLINDRICAL_SURFACE ( 'NONE', #26934, 3.499999999999999556 ) ;
#37997=DIRECTION ( 'NONE',  ( -0.000000000000000000, 1.259100132267607459E-16, -1.000000000000000000 ) ) ;
#37999=ORIENTED_EDGE ( 'NONE', *, *, #13119, .F. ) ;
#38001=CARTESIAN_POINT ( 'NONE',  ( -3.310556943750002201, 15.58864905735837780, -130.6807724695661364 ) ) ;
#38003=CARTESIAN_POINT ( 'NONE',  ( -3.310556943750002645, 15.58864905735836537, -38.76827246956612782 ) ) ;
#38004=CARTESIAN_POINT ( 'NONE',  ( 3.310556943749999981, 15.58864905735836004, -25.43493913623279212 ) ) ;
#38005=CARTESIAN_POINT ( 'NONE',  ( -1.655278471875002211, 14.63297358603754716, -94.68493913623279923 ) ) ;
#38006=CARTESIAN_POINT ( 'NONE',  ( 2.340729813953370519E-16, 21.32270188528332255, -143.0141058028994792 ) ) ;
#38009=CARTESIAN_POINT ( 'NONE',  ( 1.655278471874998436, 14.63297358603755249, -137.5182724695661420 ) ) ;
#38012=FACE_OUTER_BOUND ( 'NONE', #7, .T. ) ;
#38013=CARTESIAN_POINT ( 'NONE',  ( -1.749999999999999778, 20.53108891324555429, -80.82139747004410424 ) ) ;
#38014=CARTESIAN_POINT ( 'NONE',  ( 2.340729813953370519E-16, 21.32270188528331190, -65.10160580289945642 ) ) ;
#38017=CYLINDRICAL_SURFACE ( 'NONE', #29506, 3.499999999999999556 ) ;
#38020=CARTESIAN_POINT ( 'NONE',  ( 3.310556943749999981, 15.58864905735837247, -120.3474391362328078 ) ) ;
#38021=LINE ( 'NONE', #19090, #19676 ) ;
#38023=ORIENTED_EDGE ( 'NONE', *, *, #17100, .T. ) ;
#38025=CARTESIAN_POINT ( 'NONE',  ( 2.474675557024783212E-16, 21.54145188432740099, -108.9047308033774328 ) ) ;
#38027=( LENGTH_UNIT ( ) NAMED_UNIT ( * ) SI_UNIT ( .MILLI., .METRE. ) );
#38029=CARTESIAN_POINT ( 'NONE',  ( 3.500000000000001332, 19.52072594216370760, -59.07139747004410424 ) ) ;
#38031=CARTESIAN_POINT ( 'NONE',  ( 1.655278471874998436, 14.63297358603754361, -71.43077246956613635 ) ) ;
#38032=( BOUNDED_CURVE ( )  B_SPLINE_CURVE ( 2, ( #22788, #35761, #35960, #6823, #19796, #3633, #16620, #29580, #444 ),
 .UNSPECIFIED., .F., .T. ) 
 B_SPLINE_CURVE_WITH_KNOTS ( ( 3, 2, 2, 2, 3 ),
 ( 0.3145833333333333259, 0.3152777777777777679, 0.3166666666666666519, 0.3180555555555555358, 0.3187499999999999778 ),
 .UNSPECIFIED. ) 
 CURVE ( )  GEOMETRIC_REPRESENTATION_ITEM ( )  RATIONAL_B_SPLINE_CURVE ( ( 0.9330127018922194093, 0.9330127018922194093, 1.000000000000000000, 0.8660254037844387076, 1.000000000000000000, 0.8660254037844387076, 1.000000000000000000, 0.9330127018922194093, 0.9330127018922194093 ) ) 
 REPRESENTATION_ITEM ( '' )  );
#38033=CARTESIAN_POINT ( 'NONE',  ( 0.000000000000000000, 17.50000000000002487, -149.5231586289125687 ) ) ;
#38034=DIRECTION ( 'NONE',  ( -0.000000000000000000, 1.259100132267607459E-16, -1.000000000000000000 ) ) ;
#38037=CARTESIAN_POINT ( 'NONE',  ( -7.022189441860112050E-16, 13.67729811471671297, -24.51410580289947561 ) ) ;
#38038=DIRECTION ( 'NONE',  ( 0.000000000000000000, 1.000000000000000000, 0.000000000000000000 ) ) ;
#38039=CARTESIAN_POINT ( 'NONE',  ( -3.310556943750001313, 17.50000000000001776, -77.76410580289946495 ) ) ;
#38045=CARTESIAN_POINT ( 'NONE',  ( 1.743066579297357930E-14, 14.00000000000002132, -129.4047308033774186 ) ) ;
#38047=CARTESIAN_POINT ( 'NONE',  ( -3.500000000000000000, 19.52072594216371826, -113.7380641367107472 ) ) ;
#38048=CARTESIAN_POINT ( 'NONE',  ( 3.310556943749999981, 15.58864905735836182, -50.43493913623279923 ) ) ;
#38049=CARTESIAN_POINT ( 'NONE',  ( -3.310556943750000425, 19.41135094264166838, -110.9349391362327850 ) ) ;
#38051=ADVANCED_FACE ( 'NONE', ( #13176 ), #33370, .T. ) ;
#38052=ADVANCED_FACE ( 'NONE', ( #39966 ), #26162, .T. ) ;
#38053=CARTESIAN_POINT ( 'NONE',  ( -3.310556943750001313, 17.50000000000001066, -36.76410580289947205 ) ) ;
#38054=CARTESIAN_POINT ( 'NONE',  ( 3.310556943750001313, 17.50000000000001421, -61.35160580289945642 ) ) ;
#38055=CARTESIAN_POINT ( 'NONE',  ( 2.474675557024783212E-16, 21.54145188432740099, -106.2109808024214885 ) ) ;
#38057=CARTESIAN_POINT ( 'NONE',  ( 1.655278471875001101, 20.36702641396249192, -90.09743913623280775 ) ) ;
#38058=CARTESIAN_POINT ( 'NONE',  ( 3.500000000000000000, 15.47927405783632793, -98.23806413671076143 ) ) ;
#38060=DIRECTION ( 'NONE',  ( -0.000000000000000000, 1.259100132267607459E-16, -1.000000000000000000 ) ) ;
#38062=CARTESIAN_POINT ( 'NONE',  ( 2.474675557024783212E-16, 21.54145188432739388, -62.21098080242150274 ) ) ;
#38065=CARTESIAN_POINT ( 'NONE',  ( -3.310556943750000425, 19.41135094264165772, -24.84743913623281841 ) ) ;
#38066=CARTESIAN_POINT ( 'NONE',  ( -3.500000000000001332, 17.50000000000001066, -46.65473080337742573 ) ) ;
#38069=CARTESIAN_POINT ( 'NONE',  ( -1.655278471875002211, 14.63297358603754894, -106.6849391362327992 ) ) ;
#38070=CARTESIAN_POINT ( 'NONE',  ( 2.340729813953370519E-16, 21.32270188528330834, -34.10160580289946353 ) ) ;
#38076=CARTESIAN_POINT ( 'NONE',  ( 3.310556943750001313, 17.50000000000001776, -87.26410580289947916 ) ) ;
#38077=CARTESIAN_POINT ( 'NONE',  ( -3.500000000000000000, 19.52072594216370405, -24.04431413575484910 ) ) ;
#38080=( BOUNDED_CURVE ( )  B_SPLINE_CURVE ( 2, ( #18597, #40716, #41149, #24987, #37949, #8810, #21782, #24358, #4989 ),
 .UNSPECIFIED., .F., .T. ) 
 B_SPLINE_CURVE_WITH_KNOTS ( ( 3, 2, 2, 2, 3 ),
 ( 0.4729166666666666519, 0.4736111111111110938, 0.4749999999999999778, 0.4763888888888888618, 0.4770833333333333592 ),
 .UNSPECIFIED. ) 
 CURVE ( )  GEOMETRIC_REPRESENTATION_ITEM ( )  RATIONAL_B_SPLINE_CURVE ( ( 0.9330127018922194093, 0.9330127018922194093, 1.000000000000000000, 0.8660254037844387076, 1.000000000000000000, 0.8660254037844387076, 1.000000000000000000, 0.9330127018922167448, 0.9330127018922194093 ) ) 
 REPRESENTATION_ITEM ( '' )  );
#38085=EDGE_CURVE ( 'NONE', #24436, #40707, #2675, .T. ) ;
#38087=CARTESIAN_POINT ( 'NONE',  ( 1.655278471874998436, 14.63297358603754716, -95.43077246956613635 ) ) ;
#38089=VERTEX_POINT ( 'NONE', #13592 ) ;
#38090=DIRECTION ( 'NONE',  ( -0.000000000000000000, 1.259100132267607459E-16, -1.000000000000000000 ) ) ;
#38091=VERTEX_POINT ( 'NONE', #39114 ) ;
#38099=VECTOR ( 'NONE', #33107, 1000.000000000000000 ) ;
#38100=CARTESIAN_POINT ( 'NONE',  ( 3.500000000000001332, 17.50000000000002132, -109.1547308033774186 ) ) ;
#38101=LINE ( 'NONE', #8958, #29587 ) ;
#38102=CARTESIAN_POINT ( 'NONE',  ( 3.310556943750001313, 17.50000000000002487, -137.2641058028994792 ) ) ;
#38103=CARTESIAN_POINT ( 'NONE',  ( 3.500000000000001332, 19.52072594216371826, -133.3776474690881741 ) ) ;
#38104=EDGE_LOOP ( 'NONE', ( #36899, #34384, #27011, #14355 ) ) ;
#38105=CARTESIAN_POINT ( 'NONE',  ( 0.9378221735089300459, 21.00000000000001421, -72.94938900211596433 ) ) ;
#38106=CARTESIAN_POINT ( 'NONE',  ( 1.655278471875001101, 20.36702641396249547, -127.1849391362327992 ) ) ;
#38107=CARTESIAN_POINT ( 'NONE',  ( -7.022189441860112050E-16, 13.67729811471671653, -48.60160580289946353 ) ) ;
#38108=ORIENTED_EDGE ( 'NONE', *, *, #34340, .F. ) ;
#38110=CARTESIAN_POINT ( 'NONE',  ( 1.750000000000001110, 20.53108891324556140, -134.9880641367107614 ) ) ;
#38113=CARTESIAN_POINT ( 'NONE',  ( -3.310556943750000425, 19.41135094264166483, -76.93493913623278502 ) ) ;
#38114=CARTESIAN_POINT ( 'NONE',  ( -1.750000000000002220, 14.46891108675448834, -125.7943141357548456 ) ) ;
#38115=CARTESIAN_POINT ( 'NONE',  ( -3.310556943750002645, 15.58864905735837425, -107.6807724695661506 ) ) ;
#38119=CARTESIAN_POINT ( 'NONE',  ( 3.500000000000000000, 15.47927405783632615, -81.54431413575484555 ) ) ;
#38121=CARTESIAN_POINT ( 'NONE',  ( 2.340729813953370519E-16, 21.32270188528330479, -45.01410580289947916 ) ) ;
#38122=CARTESIAN_POINT ( 'NONE',  ( -3.310556943750002645, 15.58864905735837425, -98.76827246956612782 ) ) ;
#38124=CARTESIAN_POINT ( 'NONE',  ( 1.749999999999998224, 14.46891108675447413, -39.62764746908817415 ) ) ;
#38125=ADVANCED_FACE ( 'NONE', ( #36566 ), #26576, .T. ) ;
#38126=ORIENTED_EDGE ( 'NONE', *, *, #6889, .T. ) ;
#38127=CARTESIAN_POINT ( 'NONE',  ( 3.310556943749999981, 15.58864905735837247, -122.4349391362327992 ) ) ;
#38132=FACE_OUTER_BOUND ( 'NONE', #11615, .T. ) ;
#38134=EDGE_LOOP ( 'NONE', ( #24703, #12131, #3773, #15243 ) ) ;
#38135=CARTESIAN_POINT ( 'NONE',  ( -7.022189441860112050E-16, 13.67729811471672186, -74.60160580289947063 ) ) ;
#38137=CARTESIAN_POINT ( 'NONE',  ( -3.500000000000000000, 19.52072594216371826, -139.7380641367107614 ) ) ;
#38140=CARTESIAN_POINT ( 'NONE',  ( -3.310556943750000425, 19.41135094264166128, -34.84743913623280775 ) ) ;
#38141=EDGE_CURVE ( 'NONE', #12883, #36360, #23569, .T. ) ;
#38148=CARTESIAN_POINT ( 'NONE',  ( -7.022189441860112050E-16, 13.67729811471671653, -48.51410580289947205 ) ) ;
#38149=ORIENTED_EDGE ( 'NONE', *, *, #12685, .T. ) ;
#38155=CARTESIAN_POINT ( 'NONE',  ( 0.000000000000000000, 17.50000000000002487, -149.5231586289125687 ) ) ;
#38156=CARTESIAN_POINT ( 'NONE',  ( 3.500000000000000000, 15.47927405783632082, -33.54431413575484555 ) ) ;
#38157=CARTESIAN_POINT ( 'NONE',  ( 1.749999999999998224, 14.46891108675447413, -35.62764746908816704 ) ) ;
#38158=CYLINDRICAL_SURFACE ( 'NONE', #31874, 3.499999999999999556 ) ;
#38159=CARTESIAN_POINT ( 'NONE',  ( 0.000000000000000000, 17.50000000000002487, -149.5231586289125687 ) ) ;
#38161=CARTESIAN_POINT ( 'NONE',  ( -1.749999999999999778, 20.53108891324556140, -142.1276474690881741 ) ) ;
#38162=CARTESIAN_POINT ( 'NONE',  ( -1.655278471874999990, 20.36702641396249547, -123.9307724695661364 ) ) ;
#38166=EDGE_CURVE ( 'NONE', #4518, #5180, #38569, .T. ) ;
#38167=CARTESIAN_POINT ( 'NONE',  ( 3.310556943749999981, 15.58864905735837247, -119.4349391362327992 ) ) ;
#38168=CARTESIAN_POINT ( 'NONE',  ( 0.9378221735089300459, 21.00000000000002487, -133.9493890021159359 ) ) ;
#38169=CARTESIAN_POINT ( 'NONE',  ( 1.750000000000001110, 20.53108891324554719, -38.98806413671076854 ) ) ;
#38171=CARTESIAN_POINT ( 'NONE',  ( 3.310556943750001313, 17.50000000000002487, -137.3516058028994564 ) ) ;
#38173=CARTESIAN_POINT ( 'NONE',  ( -1.394453263437886604E-15, 14.00000000000001066, -29.71098080242150985 ) ) ;
#38174=CARTESIAN_POINT ( 'NONE',  ( 3.310556943749999981, 15.58864905735836182, -46.43493913623279212 ) ) ;
#38176=CARTESIAN_POINT ( 'NONE',  ( -1.394453263437886604E-15, 14.00000000000001776, -104.7109808024215027 ) ) ;
#38177=CARTESIAN_POINT ( 'NONE',  ( 3.310556943749999981, 15.58864905735836714, -71.43493913623278502 ) ) ;
#38179=CARTESIAN_POINT ( 'NONE',  ( 1.655278471874998436, 14.63297358603754361, -68.43077246956613635 ) ) ;
#38180=VERTEX_POINT ( 'NONE', #14860 ) ;
#38181=CARTESIAN_POINT ( 'NONE',  ( -3.310556943750002201, 15.58864905735837247, -93.76827246956612782 ) ) ;
#38187=CARTESIAN_POINT ( 'NONE',  ( 1.749999999999998224, 14.46891108675448656, -131.6276474690881741 ) ) ;
#38188=CARTESIAN_POINT ( 'NONE',  ( -7.022189441860112050E-16, 13.67729811471671830, -49.51410580289947205 ) ) ;
#38189=FACE_OUTER_BOUND ( 'NONE', #10945, .T. ) ;
#38190=CARTESIAN_POINT ( 'NONE',  ( 1.655278471874998436, 14.63297358603754894, -110.4307724695661506 ) ) ;
#38191=CARTESIAN_POINT ( 'NONE',  ( -1.750000000000002220, 14.46891108675448478, -101.4880641367107756 ) ) ;
#38197=CARTESIAN_POINT ( 'NONE',  ( -3.310556943750000425, 19.41135094264166128, -64.84743913623280775 ) ) ;
#38200=( BOUNDED_CURVE ( )  B_SPLINE_CURVE ( 2, ( #4023, #36569, #7434, #17006, #1060, #23820, #7226, #14035, #39969 ),
 .UNSPECIFIED., .F., .F. ) 
 B_SPLINE_CURVE_WITH_KNOTS ( ( 3, 2, 2, 2, 3 ),
 ( 0.3020833333333333148, 0.3027777777777777568, 0.3041666666666666408, 0.3055555555555555802, 0.3062500000000000222 ),
 .UNSPECIFIED. ) 
 CURVE ( )  GEOMETRIC_REPRESENTATION_ITEM ( )  RATIONAL_B_SPLINE_CURVE ( ( 0.9330127018922194093, 0.9330127018922194093, 1.000000000000000000, 0.8660254037844387076, 1.000000000000000000, 0.8660254037844387076, 1.000000000000000000, 0.9330127018922194093, 0.9330127018922194093 ) ) 
 REPRESENTATION_ITEM ( '' )  );
#38205=ORIENTED_EDGE ( 'NONE', *, *, #30838, .F. ) ;
#38207=CARTESIAN_POINT ( 'NONE',  ( -1.655278471874999990, 20.36702641396249902, -131.9307724695661364 ) ) ;
#38210=CARTESIAN_POINT ( 'NONE',  ( -3.310556943750001313, 17.50000000000001066, -39.85160580289947063 ) ) ;
#38211=ADVANCED_FACE ( 'NONE', ( #30815 ), #40800, .T. ) ;
#38212=CARTESIAN_POINT ( 'NONE',  ( 3.310556943749999981, 15.58864905735836182, -27.43493913623279212 ) ) ;
#38214=CARTESIAN_POINT ( 'NONE',  ( -3.310556943750002645, 15.58864905735837247, -93.76827246956612782 ) ) ;
#38215=CARTESIAN_POINT ( 'NONE',  ( -3.310556943750001313, 17.50000000000002487, -142.7641058028994792 ) ) ;
#38217=AXIS2_PLACEMENT_3D ( 'NONE', #36688, #17340, #14142 ) ;
#38219=CARTESIAN_POINT ( 'NONE',  ( -7.022189441860112050E-16, 13.67729811471672718, -132.6016058028994564 ) ) ;
#38221=CARTESIAN_POINT ( 'NONE',  ( 0.9378221735089300459, 21.00000000000001066, -27.94938900211595012 ) ) ;
#38222=CARTESIAN_POINT ( 'NONE',  ( -0.9378221735089291577, 21.00000000000002132, -123.1663226036829855 ) ) ;
#38224=CARTESIAN_POINT ( 'NONE',  ( 1.750000000000001110, 20.53108891324555429, -80.98806413671076143 ) ) ;
#38225=CARTESIAN_POINT ( 'NONE',  ( 1.655278471874998436, 14.63297358603754184, -63.51827246956613493 ) ) ;
#38228=DIRECTION ( 'NONE',  ( -0.000000000000000000, 1.259100132267607459E-16, -1.000000000000000000 ) ) ;
#38229=CARTESIAN_POINT ( 'NONE',  ( 2.340729813953370519E-16, 21.32270188528331190, -88.10160580289947063 ) ) ;
#38230=CARTESIAN_POINT ( 'NONE',  ( -1.750000000000002220, 14.46891108675447768, -47.79431413575484555 ) ) ;
#38232=CARTESIAN_POINT ( 'NONE',  ( -1.655278471875002211, 14.63297358603755072, -114.5974391362327935 ) ) ;
#38233=DIRECTION ( 'NONE',  ( -0.000000000000000000, 1.259100132267607459E-16, -1.000000000000000000 ) ) ;
#38235=ORIENTED_EDGE ( 'NONE', *, *, #30462, .T. ) ;
#38236=CARTESIAN_POINT ( 'NONE',  ( 3.500000000000000000, 15.47927405783632793, -106.2380641367107756 ) ) ;
#38238=CARTESIAN_POINT ( 'NONE',  ( 4.648177544792955347E-16, 21.00000000000001776, -82.90473080337743284 ) ) ;
#38241=CARTESIAN_POINT ( 'NONE',  ( -3.500000000000000000, 19.52072594216370405, -32.73806413671076143 ) ) ;
#38243=CARTESIAN_POINT ( 'NONE',  ( -1.655278471875002211, 14.63297358603754539, -67.59743913623280775 ) ) ;
#38246=ORIENTED_EDGE ( 'NONE', *, *, #41458, .F. ) ;
#38247=CARTESIAN_POINT ( 'NONE',  ( -1.655278471874999990, 20.36702641396248481, -25.93077246956613990 ) ) ;
#38248=AXIS2_PLACEMENT_3D ( 'NONE', #27658, #4494, #30436 ) ;
#38249=CARTESIAN_POINT ( 'NONE',  ( -1.394453263437886604E-15, 14.00000000000002132, -125.4047308033774186 ) ) ;
#38250=CARTESIAN_POINT ( 'NONE',  ( 2.340729813953370519E-16, 21.32270188528331190, -77.01410580289946495 ) ) ;
#38253=FACE_OUTER_BOUND ( 'NONE', #41450, .T. ) ;
#38257=CARTESIAN_POINT ( 'NONE',  ( -7.022189441860112050E-16, 13.67729811471671653, -45.60160580289945642 ) ) ;
#38258=CARTESIAN_POINT ( 'NONE',  ( 1.655278471875001101, 20.36702641396249547, -107.1849391362327992 ) ) ;
#38259=EDGE_LOOP ( 'NONE', ( #22550, #40852, #24975, #8124 ) ) ;
#38260=CARTESIAN_POINT ( 'NONE',  ( -3.310556943750001313, 17.50000000000001066, -28.76410580289948271 ) ) ;
#38261=CARTESIAN_POINT ( 'NONE',  ( 3.310556943750001313, 17.50000000000001421, -59.35160580289947063 ) ) ;
#38262=CARTESIAN_POINT ( 'NONE',  ( 1.749999999999998224, 14.46891108675448301, -107.6276474690881741 ) ) ;
#38264=CARTESIAN_POINT ( 'NONE',  ( -7.424026671074350129E-16, 13.45854811567263809, -96.40473080337741862 ) ) ;
#38266=( BOUNDED_CURVE ( )  B_SPLINE_CURVE ( 2, ( #16936, #10761, #4168, #13747, #29904, #26727, #23541, #36500, #7362 ),
 .UNSPECIFIED., .F., .F. ) 
 B_SPLINE_CURVE_WITH_KNOTS ( ( 3, 2, 2, 2, 3 ),
 ( 0.5645833333333333259, 0.5652777777777777679, 0.5666666666666666519, 0.5680555555555555358, 0.5687499999999999778 ),
 .UNSPECIFIED. ) 
 CURVE ( )  GEOMETRIC_REPRESENTATION_ITEM ( )  RATIONAL_B_SPLINE_CURVE ( ( 0.9330127018922194093, 0.9330127018922194093, 1.000000000000000000, 0.8660254037844387076, 1.000000000000000000, 0.8660254037844387076, 1.000000000000000000, 0.9330127018922194093, 0.9330127018922194093 ) ) 
 REPRESENTATION_ITEM ( '' )  );
#38269=CARTESIAN_POINT ( 'NONE',  ( -3.500000000000001332, 17.50000000000001421, -58.96098080242151696 ) ) ;
#38270=CARTESIAN_POINT ( 'NONE',  ( 3.310556943749999981, 15.58864905735836182, -26.34743913623280065 ) ) ;
#38271=CARTESIAN_POINT ( 'NONE',  ( -1.750000000000002220, 14.46891108675447768, -49.48806413671076854 ) ) ;
#38273=AXIS2_PLACEMENT_3D ( 'NONE', #3110, #6510, #26077 ) ;
#38274=CARTESIAN_POINT ( 'NONE',  ( -7.022189441860112050E-16, 13.67729811471672541, -101.6016058028994706 ) ) ;
#38275=CARTESIAN_POINT ( 'NONE',  ( 3.310556943750001313, 17.50000000000001066, -34.35160580289946353 ) ) ;
#38282=CARTESIAN_POINT ( 'NONE',  ( -1.655278471874999990, 20.36702641396249192, -88.93077246956613635 ) ) ;
#38284=CARTESIAN_POINT ( 'NONE',  ( 3.500000000000000000, 15.47927405783631727, -23.23806413671077209 ) ) ;
#38285=ORIENTED_EDGE ( 'NONE', *, *, #3658, .F. ) ;
#38286=CARTESIAN_POINT ( 'NONE',  ( 0.9378221735089300459, 21.00000000000002132, -109.2556390011600342 ) ) ;
#38290=CARTESIAN_POINT ( 'NONE',  ( 1.655278471874998436, 14.63297358603754716, -97.43077246956613635 ) ) ;
#38292=VERTEX_POINT ( 'NONE', #31025 ) ;
#38293=CARTESIAN_POINT ( 'NONE',  ( 0.9378221735089300459, 21.00000000000002132, -120.9493890021159643 ) ) ;
#38294=EDGE_LOOP ( 'NONE', ( #31381, #17652, #4981, #20308 ) ) ;
#38295=CARTESIAN_POINT ( 'NONE',  ( 3.500000000000001332, 19.52072594216371826, -139.3776474690881741 ) ) ;
#38296=EDGE_CURVE ( 'NONE', #37791, #26292, #38948, .T. ) ;
#38303=CARTESIAN_POINT ( 'NONE',  ( -1.394453263437886604E-15, 14.00000000000002132, -132.7109808024214885 ) ) ;
#38305=CARTESIAN_POINT ( 'NONE',  ( 1.655278471875001101, 20.36702641396249902, -131.0974391362328220 ) ) ;
#38306=AXIS2_PLACEMENT_3D ( 'NONE', #10780, #14395, #33957 ) ;
#38309=CARTESIAN_POINT ( 'NONE',  ( -1.749999999999999778, 20.53108891324554719, -31.82139747004410069 ) ) ;
#38310=CARTESIAN_POINT ( 'NONE',  ( 3.310556943750001313, 19.41135094264166838, -127.2682724695661136 ) ) ;
#38311=CARTESIAN_POINT ( 'NONE',  ( 1.655278471875001101, 20.36702641396248836, -52.18493913623279923 ) ) ;
#38312=VERTEX_POINT ( 'NONE', #1677 ) ;
#38313=CARTESIAN_POINT ( 'NONE',  ( 3.500000000000001332, 17.50000000000002487, -135.1547308033774186 ) ) ;
#38314=SHAPE_REPRESENTATION ( 'Tension Adjustment Lead Screw Shaft', ( #40442 ), #34335 ) ;
#38316=CARTESIAN_POINT ( 'NONE',  ( 1.655278471875001101, 20.36702641396249192, -77.18493913623279923 ) ) ;
#38317=CARTESIAN_POINT ( 'NONE',  ( -1.750000000000002220, 14.46891108675448656, -122.7943141357548456 ) ) ;
#38318=CARTESIAN_POINT ( 'NONE',  ( -1.655278471874999990, 20.36702641396249547, -105.9307724695661364 ) ) ;
#38319=ADVANCED_FACE ( 'NONE', ( #40178 ), #37204, .T. ) ;
#38320=DIRECTION ( 'NONE',  ( 0.000000000000000000, 1.000000000000000000, 0.000000000000000000 ) ) ;
#38323=CARTESIAN_POINT ( 'NONE',  ( -1.749999999999999778, 20.53108891324555429, -76.12764746908817415 ) ) ;
#38324=CARTESIAN_POINT ( 'NONE',  ( -1.394453263437886604E-15, 14.00000000000001421, -61.71098080242150985 ) ) ;
#38325=CARTESIAN_POINT ( 'NONE',  ( 2.340729813953370519E-16, 21.32270188528330479, -43.01410580289948626 ) ) ;
#38327=EDGE_CURVE ( 'NONE', #32026, #18625, #6768, .T. ) ;
#38328=CARTESIAN_POINT ( 'NONE',  ( -3.310556943750000425, 19.41135094264166483, -101.9349391362327992 ) ) ;
#38329=CARTESIAN_POINT ( 'NONE',  ( -0.9378221735089291577, 21.00000000000002132, -114.1663226036829997 ) ) ;
#38331=CARTESIAN_POINT ( 'NONE',  ( 3.500000000000001332, 17.50000000000001421, -62.15473080337742573 ) ) ;
#38334=CARTESIAN_POINT ( 'NONE',  ( 1.655278471875001101, 20.36702641396249547, -124.1849391362327992 ) ) ;
#38335=CARTESIAN_POINT ( 'NONE',  ( -1.394453263437886604E-15, 14.00000000000001776, -91.71098080242150274 ) ) ;
#38338=CARTESIAN_POINT ( 'NONE',  ( -1.394453263437886604E-15, 14.00000000000001421, -76.71098080242148853 ) ) ;
#38339=CARTESIAN_POINT ( 'NONE',  ( 4.648177544792955347E-16, 21.00000000000001421, -60.21098080242150274 ) ) ;
#38340=CARTESIAN_POINT ( 'NONE',  ( -3.500000000000002220, 15.47927405783632437, -52.57139747004409003 ) ) ;
#38343=CARTESIAN_POINT ( 'NONE',  ( -3.310556943750002201, 15.58864905735837070, -75.76827246956612782 ) ) ;
#38344=CARTESIAN_POINT ( 'NONE',  ( 0.9378221735089281585, 14.00000000000001066, -40.66632260368298546 ) ) ;
#38346=CARTESIAN_POINT ( 'NONE',  ( -1.394453263437886604E-15, 14.00000000000001421, -73.40473080337743284 ) ) ;
#38350=CARTESIAN_POINT ( 'NONE',  ( 2.340729813953370519E-16, 21.32270188528330834, -32.01410580289947205 ) ) ;
#38357=CARTESIAN_POINT ( 'NONE',  ( 0.000000000000000000, 21.00000000000002487, -143.4609808024215170 ) ) ;
#38362=VECTOR ( 'NONE', #7576, 1000.000000000000000 ) ;
#38363=CARTESIAN_POINT ( 'NONE',  ( 3.500000000000000000, 15.47927405783632970, -118.2380641367107472 ) ) ;
#38365=CARTESIAN_POINT ( 'NONE',  ( -3.500000000000001332, 17.50000000000001066, -35.96098080242150985 ) ) ;
#38367=CARTESIAN_POINT ( 'NONE',  ( 0.000000000000000000, 17.50000000000002487, -149.5231586289125687 ) ) ;
#38370=CARTESIAN_POINT ( 'NONE',  ( -3.500000000000001332, 17.50000000000001421, -65.65473080337743284 ) ) ;
#38372=CARTESIAN_POINT ( 'NONE',  ( 3.500000000000001776, 19.52072594216372181, -138.3776474690881741 ) ) ;
#38374=CARTESIAN_POINT ( 'NONE',  ( -3.310556943750000425, 19.41135094264166838, -121.8474391362328078 ) ) ;
#38377=EDGE_CURVE ( 'NONE', #1224, #11775, #14661, .T. ) ;
#38378=EDGE_CURVE ( 'NONE', #9702, #34168, #816, .T. ) ;
#38379=CARTESIAN_POINT ( 'NONE',  ( 1.750000000000001110, 20.53108891324555429, -93.98806413671076143 ) ) ;
#38380=CARTESIAN_POINT ( 'NONE',  ( 3.500000000000000000, 15.47927405783632615, -88.54431413575483134 ) ) ;
#38381=EDGE_CURVE ( 'NONE', #29607, #3989, #12736, .T. ) ;
#38382=CARTESIAN_POINT ( 'NONE',  ( 3.310556943749999981, 15.58864905735837247, -115.4349391362327850 ) ) ;
#38384=CARTESIAN_POINT ( 'NONE',  ( 3.500000000000000000, 15.47927405783632082, -34.23806413671076854 ) ) ;
#38385=CARTESIAN_POINT ( 'NONE',  ( -3.695301148110399846E-14, 21.00000000000002132, -124.9047308033774186 ) ) ;
#38387=CARTESIAN_POINT ( 'NONE',  ( 1.655278471875001101, 20.36702641396249902, -139.1849391362327708 ) ) ;
#38390=CARTESIAN_POINT ( 'NONE',  ( 2.340729813953370519E-16, 21.32270188528331190, -47.10160580289945642 ) ) ;
#38393=CARTESIAN_POINT ( 'NONE',  ( 1.655278471875001101, 20.36702641396248836, -71.18493913623278502 ) ) ;
#38395=CARTESIAN_POINT ( 'NONE',  ( -1.655278471874999990, 20.36702641396248836, -71.93077246956613635 ) ) ;
#38396=ORIENTED_EDGE ( 'NONE', *, *, #18387, .T. ) ;
#38397=CARTESIAN_POINT ( 'NONE',  ( 3.310556943749999981, 15.58864905735836892, -91.43493913623279923 ) ) ;
#38401=CARTESIAN_POINT ( 'NONE',  ( 1.655278471874998436, 14.63297358603754006, -49.43077246956615056 ) ) ;
#38402=( BOUNDED_CURVE ( )  B_SPLINE_CURVE ( 2, ( #15502, #40448, #23665, #41235, #30662, #17278, #30243, #11304, #24286 ),
 .UNSPECIFIED., .F., .T. ) 
 B_SPLINE_CURVE_WITH_KNOTS ( ( 3, 2, 2, 2, 3 ),
 ( 0.8062500000000000222, 0.8069444444444444642, 0.8083333333333333481, 0.8097222222222222321, 0.8104166666666666741 ),
 .UNSPECIFIED. ) 
 CURVE ( )  GEOMETRIC_REPRESENTATION_ITEM ( )  RATIONAL_B_SPLINE_CURVE ( ( 0.9330127018922194093, 0.9330127018922194093, 1.000000000000000000, 0.8660254037844387076, 1.000000000000000000, 0.8660254037844387076, 1.000000000000000000, 0.9330127018922194093, 0.9330127018922194093 ) ) 
 REPRESENTATION_ITEM ( '' )  );
#38404=CARTESIAN_POINT ( 'NONE',  ( -3.310556943750000425, 19.41135094264166838, -103.8474391362328220 ) ) ;
#38407=ORIENTED_EDGE ( 'NONE', *, *, #23796, .F. ) ;
#38411=CARTESIAN_POINT ( 'NONE',  ( -7.022189441860112050E-16, 13.67729811471671830, -61.51410580289946495 ) ) ;
#38413=ORIENTED_EDGE ( 'NONE', *, *, #14532, .F. ) ;
#38416=CARTESIAN_POINT ( 'NONE',  ( -0.9378221735089308231, 21.00000000000002487, -142.8600726046389298 ) ) ;
#38418=CARTESIAN_POINT ( 'NONE',  ( 1.045839947578414805E-15, 14.00000000000002665, -141.4047308033774186 ) ) ;
#38419=EDGE_CURVE ( 'NONE', #17551, #23461, #18205, .T. ) ;
#38423=CARTESIAN_POINT ( 'NONE',  ( 3.310556943750001313, 19.41135094264166838, -125.1807724695661364 ) ) ;
#38426=CARTESIAN_POINT ( 'NONE',  ( -1.655278471875002211, 14.63297358603754006, -36.68493913623279923 ) ) ;
#38427=CARTESIAN_POINT ( 'NONE',  ( -1.655278471875002211, 14.63297358603754006, -29.68493913623279568 ) ) ;
#38428=EDGE_CURVE ( 'NONE', #5239, #19673, #25065, .T. ) ;
#38429=CARTESIAN_POINT ( 'NONE',  ( 1.655278471874998436, 14.63297358603754539, -88.51827246956612782 ) ) ;
#38430=CARTESIAN_POINT ( 'NONE',  ( -3.310556943750002645, 15.58864905735837958, -137.6807724695661364 ) ) ;
#38433=EDGE_CURVE ( 'NONE', #23444, #19172, #12071, .T. ) ;
#38434=CARTESIAN_POINT ( 'NONE',  ( -1.655278471875002211, 14.63297358603755249, -133.6849391362327992 ) ) ;
#38435=AXIS2_PLACEMENT_3D ( 'NONE', #32345, #2791, #9385 ) ;
#38436=CARTESIAN_POINT ( 'NONE',  ( 1.749999999999998224, 14.46891108675447946, -70.32139747004409003 ) ) ;
#38437=CARTESIAN_POINT ( 'NONE',  ( 4.648177544792955347E-16, 21.00000000000001066, -27.90473080337742928 ) ) ;
#38438=CYLINDRICAL_SURFACE ( 'NONE', #29996, 3.499999999999999556 ) ;
#38439=CARTESIAN_POINT ( 'NONE',  ( 1.749999999999998224, 14.46891108675448301, -95.32139747004409003 ) ) ;
#38440=CARTESIAN_POINT ( 'NONE',  ( 1.750000000000001110, 20.53108891324555429, -82.98806413671074722 ) ) ;
#38441=CARTESIAN_POINT ( 'NONE',  ( 3.310556943750001313, 17.50000000000001421, -62.35160580289945642 ) ) ;
#38444=CARTESIAN_POINT ( 'NONE',  ( 4.648177544792955347E-16, 21.00000000000001421, -47.21098080242149564 ) ) ;
#38445=CARTESIAN_POINT ( 'NONE',  ( -1.655278471875002211, 14.63297358603754716, -87.68493913623279923 ) ) ;
#38446=CARTESIAN_POINT ( 'NONE',  ( -3.500000000000001332, 17.50000000000002132, -116.6547308033774328 ) ) ;
#38447=CARTESIAN_POINT ( 'NONE',  ( 1.655278471874998436, 14.63297358603754894, -114.4307724695661364 ) ) ;
#38448=CARTESIAN_POINT ( 'NONE',  ( 3.500000000000001332, 17.50000000000001066, -34.46098080242150985 ) ) ;
#38449=CARTESIAN_POINT ( 'NONE',  ( -1.394453263437886604E-15, 14.00000000000001421, -62.40473080337742573 ) ) ;
#38451=CARTESIAN_POINT ( 'NONE',  ( 2.474675557024783212E-16, 21.54145188432740099, -110.9047308033774328 ) ) ;
#38452=LINE ( 'NONE', #41649, #871 ) ;
#38455=CARTESIAN_POINT ( 'NONE',  ( -1.394453263437886604E-15, 14.00000000000001421, -64.40473080337743284 ) ) ;
#38457=CARTESIAN_POINT ( 'NONE',  ( -1.655278471874999990, 20.36702641396248836, -65.93077246956613635 ) ) ;
#38459=CARTESIAN_POINT ( 'NONE',  ( -7.022189441860112050E-16, 13.67729811471672718, -120.5141058028994649 ) ) ;
#38463=MANIFOLD_SOLID_BREP ( 'Thread2', #24028 ) ;
#38466=CARTESIAN_POINT ( 'NONE',  ( -3.500000000000002220, 15.47927405783633326, -104.8776474690881741 ) ) ;
#38467=CARTESIAN_POINT ( 'NONE',  ( 1.655278471875001101, 20.36702641396249192, -78.09743913623280775 ) ) ;
#38468=VERTEX_POINT ( 'NONE', #9100 ) ;
#38472=CARTESIAN_POINT ( 'NONE',  ( -7.022189441860112050E-16, 13.67729811471673074, -138.5141058028994792 ) ) ;
#38475=CARTESIAN_POINT ( 'NONE',  ( -3.310556943750001313, 17.50000000000001066, -44.85160580289947063 ) ) ;
#38477=CARTESIAN_POINT ( 'NONE',  ( 2.340729813953370519E-16, 21.32270188528331900, -102.1016058028994564 ) ) ;
#38478=EDGE_LOOP ( 'NONE', ( #376, #25658, #41225, #8746 ) ) ;
#38479=CARTESIAN_POINT ( 'NONE',  ( 1.655278471875001101, 20.36702641396248481, -29.09743913623280420 ) ) ;
#38480=CARTESIAN_POINT ( 'NONE',  ( 1.655278471875001101, 20.36702641396248836, -59.18493913623279212 ) ) ;
#38481=CARTESIAN_POINT ( 'NONE',  ( 3.500000000000000000, 15.47927405783632793, -105.5443141357548456 ) ) ;
#38484=CARTESIAN_POINT ( 'NONE',  ( 3.500000000000001332, 17.50000000000001776, -95.15473080337743284 ) ) ;
#38488=CARTESIAN_POINT ( 'NONE',  ( 1.749999999999998224, 14.46891108675447768, -56.62764746908817415 ) ) ;
#38490=CARTESIAN_POINT ( 'NONE',  ( 1.655278471875001101, 20.36702641396248481, -27.09743913623280420 ) ) ;
#38491=CARTESIAN_POINT ( 'NONE',  ( 2.474675557024783212E-16, 21.54145188432739388, -47.90473080337741862 ) ) ;
#38493=CARTESIAN_POINT ( 'NONE',  ( -3.310556943750001313, 17.50000000000001066, -31.85160580289945997 ) ) ;
#38496=CARTESIAN_POINT ( 'NONE',  ( -1.750000000000002220, 14.46891108675449011, -141.7943141357548313 ) ) ;
#38500=CARTESIAN_POINT ( 'NONE',  ( -3.310556943750000425, 19.41135094264166838, -84.84743913623279354 ) ) ;
#38501=DIRECTION ( 'NONE',  ( -0.000000000000000000, 1.259100132267607459E-16, -1.000000000000000000 ) ) ;
#38504=DIRECTION ( 'NONE',  ( -0.000000000000000000, 1.259100132267607459E-16, -1.000000000000000000 ) ) ;
#38507=CARTESIAN_POINT ( 'NONE',  ( -3.310556943750002645, 15.58864905735837247, -94.68077246956613635 ) ) ;
#38510=CARTESIAN_POINT ( 'NONE',  ( -1.394453263437886604E-15, 14.00000000000001421, -78.40473080337741862 ) ) ;
#38511=ORIENTED_EDGE ( 'NONE', *, *, #23407, .T. ) ;
#38513=DIRECTION ( 'NONE',  ( -0.000000000000000000, 1.259100132267607459E-16, -1.000000000000000000 ) ) ;
#38517=CARTESIAN_POINT ( 'NONE',  ( 4.648177544792955347E-16, 21.00000000000001776, -88.90473080337740441 ) ) ;
#38518=DIRECTION ( 'NONE',  ( -0.000000000000000000, 1.259100132267607459E-16, -1.000000000000000000 ) ) ;
#38519=CARTESIAN_POINT ( 'NONE',  ( -3.310556943750001313, 17.50000000000002487, -130.7641058028994507 ) ) ;
#38521=ORIENTED_EDGE ( 'NONE', *, *, #16777, .F. ) ;
#38522=CARTESIAN_POINT ( 'NONE',  ( -3.500000000000000000, 19.52072594216371826, -141.0443141357548313 ) ) ;
#38524=CARTESIAN_POINT ( 'NONE',  ( -1.655278471874999990, 20.36702641396249547, -126.0182724695661278 ) ) ;
#38525=CARTESIAN_POINT ( 'NONE',  ( 2.340729813953370519E-16, 21.32270188528330834, -52.10160580289946353 ) ) ;
#38526=ORIENTED_EDGE ( 'NONE', *, *, #10392, .F. ) ;
#38527=CARTESIAN_POINT ( 'NONE',  ( -7.424026671074350129E-16, 13.45854811567264164, -131.4047308033774186 ) ) ;
#38530=CARTESIAN_POINT ( 'NONE',  ( 3.310556943749999981, 15.58864905735836714, -76.43493913623278502 ) ) ;
#38531=CARTESIAN_POINT ( 'NONE',  ( -3.500000000000002220, 15.47927405783633503, -122.8776474690881741 ) ) ;
#38532=CARTESIAN_POINT ( 'NONE',  ( 1.655278471874998436, 14.63297358603754716, -108.4307724695661506 ) ) ;
#38533=CARTESIAN_POINT ( 'NONE',  ( -1.750000000000002220, 14.46891108675448478, -107.4880641367107614 ) ) ;
#38536=CARTESIAN_POINT ( 'NONE',  ( 3.500000000000001332, 17.50000000000001421, -73.46098080242151696 ) ) ;
#38537=CARTESIAN_POINT ( 'NONE',  ( -3.310556943750002645, 15.58864905735836714, -42.68077246956614346 ) ) ;
#38538=CARTESIAN_POINT ( 'NONE',  ( -3.310556943750002645, 15.58864905735837425, -101.7682724695661278 ) ) ;
#38539=CARTESIAN_POINT ( 'NONE',  ( 4.648177544792955347E-16, 21.00000000000001421, -67.90473080337741862 ) ) ;
#38540=CARTESIAN_POINT ( 'NONE',  ( 3.500000000000000000, 15.47927405783632260, -66.23806413671077564 ) ) ;
#38542=VERTEX_POINT ( 'NONE', #9316 ) ;
#38543=CARTESIAN_POINT ( 'NONE',  ( 3.310556943750001313, 19.41135094264166838, -115.2682724695661278 ) ) ;
#38544=CARTESIAN_POINT ( 'NONE',  ( -3.500000000000001332, 17.50000000000002487, -136.6547308033774186 ) ) ;
#38547=DIRECTION ( 'NONE',  ( -0.000000000000000000, 1.259100132267607459E-16, -1.000000000000000000 ) ) ;
#38552=CARTESIAN_POINT ( 'NONE',  ( 1.655278471874998436, 14.63297358603754361, -76.51827246956612782 ) ) ;
#38553=CARTESIAN_POINT ( 'NONE',  ( 0.9378221735089281585, 14.00000000000001066, -48.36007260463891555 ) ) ;
#38554=CARTESIAN_POINT ( 'NONE',  ( 0.9378221735089281585, 14.00000000000001066, -45.36007260463890134 ) ) ;
#38558=CARTESIAN_POINT ( 'NONE',  ( 2.340729813953370519E-16, 21.32270188528330834, -36.01410580289947205 ) ) ;
#38561=ORIENTED_EDGE ( 'NONE', *, *, #25232, .T. ) ;
#38564=EDGE_CURVE ( 'NONE', #17584, #4518, #35882, .T. ) ;
#38567=CARTESIAN_POINT ( 'NONE',  ( -3.500000000000002220, 15.47927405783632970, -85.87764746908817415 ) ) ;
#38569=( BOUNDED_CURVE ( )  B_SPLINE_CURVE ( 2, ( #409, #13385, #33155, #10196, #16794, #29755, #17003, #33596, #27828 ),
 .UNSPECIFIED., .F., .T. ) 
 B_SPLINE_CURVE_WITH_KNOTS ( ( 3, 2, 2, 2, 3 ),
 ( 0.8604166666666667185, 0.8611111111111111605, 0.8625000000000000444, 0.8638888888888889284, 0.8645833333333333703 ),
 .UNSPECIFIED. ) 
 CURVE ( )  GEOMETRIC_REPRESENTATION_ITEM ( )  RATIONAL_B_SPLINE_CURVE ( ( 0.9330127018922194093, 0.9330127018922194093, 1.000000000000000000, 0.8660254037844387076, 1.000000000000000000, 0.8660254037844387076, 1.000000000000000000, 0.9330127018922194093, 0.9330127018922194093 ) ) 
 REPRESENTATION_ITEM ( '' )  );
#38570=CARTESIAN_POINT ( 'NONE',  ( 3.369928719974892676E-15, 14.00000000000002309, -140.7109808024215170 ) ) ;
#38571=CARTESIAN_POINT ( 'NONE',  ( -3.500000000000002220, 15.47927405783633503, -121.5713974700441042 ) ) ;
#38573=CARTESIAN_POINT ( 'NONE',  ( 1.749999999999998224, 14.46891108675447413, -35.62764746908816704 ) ) ;
#38575=CARTESIAN_POINT ( 'NONE',  ( -1.394453263437886604E-15, 14.00000000000001066, -40.71098080242150274 ) ) ;
#38576=CARTESIAN_POINT ( 'NONE',  ( 3.500000000000001332, 19.52072594216371826, -142.3776474690881741 ) ) ;
#38578=CARTESIAN_POINT ( 'NONE',  ( 3.500000000000000000, 15.47927405783633503, -141.5443141357548313 ) ) ;
#38579=CARTESIAN_POINT ( 'NONE',  ( 0.9378221735089281585, 14.00000000000002132, -120.6663226036829855 ) ) ;
#38580=CARTESIAN_POINT ( 'NONE',  ( 2.340729813953370519E-16, 21.32270188528331900, -124.0141058028994792 ) ) ;
#38583=EDGE_CURVE ( 'NONE', #41433, #11548, #11370, .T. ) ;
#38585=CARTESIAN_POINT ( 'NONE',  ( -3.500000000000001332, 17.50000000000001776, -92.96098080242151696 ) ) ;
#38587=CARTESIAN_POINT ( 'NONE',  ( 2.340729813953370519E-16, 21.32270188528330834, -61.01410580289946495 ) ) ;
#38588=CARTESIAN_POINT ( 'NONE',  ( 3.310556943750001313, 19.41135094264166838, -117.2682724695661278 ) ) ;
#38590=CARTESIAN_POINT ( 'NONE',  ( -3.500000000000002220, 15.47927405783633503, -121.8776474690881884 ) ) ;
#38591=CARTESIAN_POINT ( 'NONE',  ( 1.750000000000001110, 20.53108891324554719, -34.98806413671076854 ) ) ;
#38592=CARTESIAN_POINT ( 'NONE',  ( 0.000000000000000000, 17.50000000000002487, -149.5231586289125687 ) ) ;
#38594=CARTESIAN_POINT ( 'NONE',  ( 1.655278471875001101, 20.36702641396249902, -132.1849391362327992 ) ) ;
#38596=CARTESIAN_POINT ( 'NONE',  ( 1.750000000000001110, 20.53108891324556140, -137.9880641367107614 ) ) ;
#38597=CARTESIAN_POINT ( 'NONE',  ( -1.655278471874999990, 20.36702641396248481, -43.01827246956613493 ) ) ;
#38599=DIRECTION ( 'NONE',  ( -0.000000000000000000, 1.259100132267607459E-16, -1.000000000000000000 ) ) ;
#38600=CARTESIAN_POINT ( 'NONE',  ( -1.655278471874999990, 20.36702641396248836, -69.01827246956612782 ) ) ;
#38602=CARTESIAN_POINT ( 'NONE',  ( -3.310556943750000425, 19.41135094264166128, -63.84743913623280775 ) ) ;
#38603=ORIENTED_EDGE ( 'NONE', *, *, #33220, .T. ) ;
#38604=CARTESIAN_POINT ( 'NONE',  ( -7.022189441860112050E-16, 13.67729811471672363, -89.60160580289947063 ) ) ;
#38608=CARTESIAN_POINT ( 'NONE',  ( -3.500000000000000000, 19.52072594216370760, -70.04431413575484555 ) ) ;
#38609=CARTESIAN_POINT ( 'NONE',  ( -7.022189441860112050E-16, 13.67729811471671830, -50.51410580289947205 ) ) ;
#38612=CARTESIAN_POINT ( 'NONE',  ( 3.310556943750001313, 19.41135094264166838, -107.1807724695661364 ) ) ;
#38613=ORIENTED_EDGE ( 'NONE', *, *, #7441, .F. ) ;
#38614=SHAPE_DEFINITION_REPRESENTATION ( #14294, #38314 ) ;
#38616=ORIENTED_EDGE ( 'NONE', *, *, #25346, .F. ) ;
#38618=CARTESIAN_POINT ( 'NONE',  ( 1.655278471875001101, 20.36702641396248836, -60.09743913623280775 ) ) ;
#38620=VERTEX_POINT ( 'NONE', #39273 ) ;
#38624=EDGE_CURVE ( 'NONE', #4881, #9822, #35591, .T. ) ;
#38629=CARTESIAN_POINT ( 'NONE',  ( 2.340729813953370519E-16, 21.32270188528331900, -126.0141058028994792 ) ) ;
#38632=CARTESIAN_POINT ( 'NONE',  ( 3.310556943749999981, 15.58864905735836182, -37.43493913623280633 ) ) ;
#38633=CARTESIAN_POINT ( 'NONE',  ( -1.655278471875002211, 14.63297358603754006, -28.68493913623279568 ) ) ;
#38634=CARTESIAN_POINT ( 'NONE',  ( 3.310556943750001313, 17.50000000000001776, -89.35160580289947063 ) ) ;
#38635=CARTESIAN_POINT ( 'NONE',  ( -3.310556943750001313, 17.50000000000002487, -138.7641058028994792 ) ) ;
#38637=CARTESIAN_POINT ( 'NONE',  ( 1.750000000000001110, 20.53108891324555785, -126.9880641367107614 ) ) ;
#38639=CARTESIAN_POINT ( 'NONE',  ( 2.340729813953370519E-16, 21.32270188528332255, -134.1016058028994564 ) ) ;
#38642=CARTESIAN_POINT ( 'NONE',  ( -1.750000000000002220, 14.46891108675448834, -125.7943141357548456 ) ) ;
#38644=CARTESIAN_POINT ( 'NONE',  ( -3.500000000000000888, 19.52072594216371115, -81.73806413671076143 ) ) ;
#38645=CARTESIAN_POINT ( 'NONE',  ( 3.310556943749999981, 15.58864905735836537, -65.43493913623279923 ) ) ;
#38646=( BOUNDED_CURVE ( )  B_SPLINE_CURVE ( 2, ( #3038, #12818, #9421, #12399, #5601, #28349, #16031, #15600, #8790 ),
 .UNSPECIFIED., .F., .T. ) 
 B_SPLINE_CURVE_WITH_KNOTS ( ( 3, 2, 2, 2, 3 ),
 ( 0.8562499999999999556, 0.8569444444444443976, 0.8583333333333332815, 0.8597222222222222765, 0.8604166666666667185 ),
 .UNSPECIFIED. ) 
 CURVE ( )  GEOMETRIC_REPRESENTATION_ITEM ( )  RATIONAL_B_SPLINE_CURVE ( ( 0.9330127018922194093, 0.9330127018922194093, 1.000000000000000000, 0.8660254037844387076, 1.000000000000000000, 0.8660254037844387076, 1.000000000000000000, 0.9330127018922194093, 0.9330127018922194093 ) ) 
 REPRESENTATION_ITEM ( '' )  );
#38650=CARTESIAN_POINT ( 'NONE',  ( 3.310556943749999981, 15.58864905735836892, -83.43493913623279923 ) ) ;
#38651=DIRECTION ( 'NONE',  ( 0.000000000000000000, 1.000000000000000000, 0.000000000000000000 ) ) ;
#38653=CARTESIAN_POINT ( 'NONE',  ( 3.310556943750001313, 17.50000000000002132, -116.2641058028994792 ) ) ;
#38656=ORIENTED_EDGE ( 'NONE', *, *, #11116, .T. ) ;
#38657=CARTESIAN_POINT ( 'NONE',  ( -1.749999999999999778, 20.53108891324555785, -109.8213974700441042 ) ) ;
#38659=EDGE_CURVE ( 'NONE', #6853, #4034, #13851, .T. ) ;
#38661=CARTESIAN_POINT ( 'NONE',  ( 4.286263797015737581E-16, 14.00000000000002487, -149.5231586289125687 ) ) ;
#38665=CARTESIAN_POINT ( 'NONE',  ( 1.655278471875001101, 20.36702641396248836, -67.09743913623280775 ) ) ;
#38667=CARTESIAN_POINT ( 'NONE',  ( 1.655278471875001101, 20.36702641396249547, -119.0974391362328078 ) ) ;
#38672=CARTESIAN_POINT ( 'NONE',  ( 3.310556943749999981, 15.58864905735836714, -72.34743913623279354 ) ) ;
#38676=EDGE_CURVE ( 'NONE', #7219, #31508, #15229, .T. ) ;
#38677=CARTESIAN_POINT ( 'NONE',  ( 3.310556943749999981, 15.58864905735837780, -142.3474391362327935 ) ) ;
#38679=VECTOR ( 'NONE', #11874, 1000.000000000000000 ) ;
#38680=CARTESIAN_POINT ( 'NONE',  ( -0.9378221735089291577, 21.00000000000002132, -113.8600726046389155 ) ) ;
#38681=CARTESIAN_POINT ( 'NONE',  ( -7.022189441860112050E-16, 13.67729811471671653, -41.60160580289947063 ) ) ;
#38682=CARTESIAN_POINT ( 'NONE',  ( 2.340729813953370519E-16, 21.32270188528331900, -106.1016058028994564 ) ) ;
#38685=CARTESIAN_POINT ( 'NONE',  ( 2.340729813953370519E-16, 21.32270188528330479, -31.01410580289947205 ) ) ;
#38686=CARTESIAN_POINT ( 'NONE',  ( 4.648177544792955347E-16, 21.00000000000002132, -112.2109808024214743 ) ) ;
#38687=CARTESIAN_POINT ( 'NONE',  ( -1.750000000000002220, 14.46891108675448656, -109.7943141357548456 ) ) ;
#38690=CARTESIAN_POINT ( 'NONE',  ( -3.500000000000001332, 17.50000000000001776, -94.65473080337743284 ) ) ;
#38691=CARTESIAN_POINT ( 'NONE',  ( -1.750000000000002220, 14.46891108675448478, -108.4880641367107614 ) ) ;
#38695=CARTESIAN_POINT ( 'NONE',  ( 3.500000000000000000, 15.47927405783632260, -56.54431413575483134 ) ) ;
#38697=CARTESIAN_POINT ( 'NONE',  ( 1.655278471874998436, 14.63297358603753651, -25.43077246956613990 ) ) ;
#38699=CARTESIAN_POINT ( 'NONE',  ( -1.749999999999999778, 20.53108891324555074, -47.82139747004410424 ) ) ;
#38701=ADVANCED_FACE ( 'NONE', ( #32899 ), #13134, .T. ) ;
#38702=CARTESIAN_POINT ( 'NONE',  ( 3.310556943750001313, 19.41135094264166128, -31.26827246956613493 ) ) ;
#38707=CARTESIAN_POINT ( 'NONE',  ( -1.394453263437886604E-15, 14.00000000000002132, -123.4047308033774044 ) ) ;
#38709=CARTESIAN_POINT ( 'NONE',  ( 3.310556943750001313, 19.41135094264166838, -83.18077246956613635 ) ) ;
#38714=EDGE_LOOP ( 'NONE', ( #12349, #34122, #21712, #25655 ) ) ;
#38716=EDGE_CURVE ( 'NONE', #37828, #1932, #8383, .T. ) ;
#38718=CARTESIAN_POINT ( 'NONE',  ( -3.310556943750000425, 19.41135094264166483, -92.84743913623280775 ) ) ;
#38719=ORIENTED_EDGE ( 'NONE', *, *, #4871, .F. ) ;
#38721=ORIENTED_EDGE ( 'NONE', *, *, #18982, .F. ) ;
#38722=EDGE_CURVE ( 'NONE', #745, #17696, #10876, .T. ) ;
#38727=ORIENTED_EDGE ( 'NONE', *, *, #38419, .F. ) ;
#38728=CARTESIAN_POINT ( 'NONE',  ( -1.394453263437886604E-15, 14.00000000000002132, -111.4047308033774186 ) ) ;
#38729=DIRECTION ( 'NONE',  ( 0.000000000000000000, 1.000000000000000000, 0.000000000000000000 ) ) ;
#38730=CARTESIAN_POINT ( 'NONE',  ( -1.655278471875002211, 14.63297358603755249, -130.5974391362328220 ) ) ;
#38732=CARTESIAN_POINT ( 'NONE',  ( -1.394453263437886604E-15, 14.00000000000001421, -73.40473080337743284 ) ) ;
#38733=CARTESIAN_POINT ( 'NONE',  ( -3.310556943750002645, 15.58864905735837780, -119.7682724695661278 ) ) ;
#38734=CARTESIAN_POINT ( 'NONE',  ( -7.022189441860112050E-16, 13.67729811471671653, -50.60160580289946353 ) ) ;
#38736=CARTESIAN_POINT ( 'NONE',  ( 2.474675557024783212E-16, 21.54145188432740810, -129.9047308033774186 ) ) ;
#38738=CARTESIAN_POINT ( 'NONE',  ( -1.655278471875002211, 14.63297358603754539, -71.68493913623278502 ) ) ;
#38739=CARTESIAN_POINT ( 'NONE',  ( 1.750000000000001110, 20.53108891324555785, -125.2943141357548456 ) ) ;
#38740=ADVANCED_FACE ( 'NONE', ( #27371 ), #4815, .T. ) ;
#38741=CARTESIAN_POINT ( 'NONE',  ( -7.022189441860112050E-16, 13.67729811471672541, -106.5141058028994792 ) ) ;
#38742=CARTESIAN_POINT ( 'NONE',  ( 1.655278471874998436, 14.63297358603753651, -23.51827246956612782 ) ) ;
#38745=CARTESIAN_POINT ( 'NONE',  ( -3.500000000000002220, 15.47927405783632615, -75.87764746908818836 ) ) ;
#38747=CARTESIAN_POINT ( 'NONE',  ( 1.655278471874998436, 14.63297358603754006, -41.43077246956614346 ) ) ;
#38749=CARTESIAN_POINT ( 'NONE',  ( 1.655278471875001101, 20.36702641396249192, -101.1849391362327992 ) ) ;
#38751=CARTESIAN_POINT ( 'NONE',  ( 3.500000000000001776, 19.52072594216370760, -66.07139747004409003 ) ) ;
#38754=CARTESIAN_POINT ( 'NONE',  ( -7.022189441860112050E-16, 13.67729811471672896, -118.6016058028994706 ) ) ;
#38755=CARTESIAN_POINT ( 'NONE',  ( -0.9378221735089268263, 14.00000000000002309, -136.4493890021159643 ) ) ;
#38760=CARTESIAN_POINT ( 'NONE',  ( 3.310556943750001313, 17.50000000000001776, -97.26410580289947916 ) ) ;
#38763=ORIENTED_EDGE ( 'NONE', *, *, #33934, .T. ) ;
#38764=CARTESIAN_POINT ( 'NONE',  ( 0.9378221735089324884, 14.00000000000002665, -136.6663226036829997 ) ) ;
#38765=CARTESIAN_POINT ( 'NONE',  ( -1.394453263437886604E-15, 14.00000000000001066, -48.40473080337742573 ) ) ;
#38769=EDGE_CURVE ( 'NONE', #18226, #33342, #28744, .T. ) ;
#38771=CARTESIAN_POINT ( 'NONE',  ( -1.655278471875002211, 14.63297358603754006, -34.59743913623280775 ) ) ;
#38775=EDGE_LOOP ( 'NONE', ( #13495, #12732, #31488, #38149 ) ) ;
#38777=ORIENTED_EDGE ( 'NONE', *, *, #2022, .T. ) ;
#38779=AXIS2_PLACEMENT_3D ( 'NONE', #19008, #6657, #26236 ) ;
#38781=CARTESIAN_POINT ( 'NONE',  ( 1.749999999999998224, 14.46891108675447413, -31.32139747004410069 ) ) ;
#38782=CARTESIAN_POINT ( 'NONE',  ( 1.749999999999998224, 14.46891108675448478, -117.3213974700440900 ) ) ;
#38783=CARTESIAN_POINT ( 'NONE',  ( -1.750000000000002220, 14.46891108675447590, -33.79431413575484555 ) ) ;
#38784=CARTESIAN_POINT ( 'NONE',  ( 3.310556943750001313, 19.41135094264167549, -137.2682724695661420 ) ) ;
#38785=CARTESIAN_POINT ( 'NONE',  ( 3.500000000000001332, 17.50000000000001066, -31.46098080242150274 ) ) ;
#38787=CARTESIAN_POINT ( 'NONE',  ( -3.500000000000000000, 19.52072594216370405, -44.73806413671076143 ) ) ;
#38789=CARTESIAN_POINT ( 'NONE',  ( 4.648177544792955347E-16, 21.00000000000001421, -65.90473080337741862 ) ) ;
#38791=CARTESIAN_POINT ( 'NONE',  ( -3.500000000000000888, 19.52072594216372181, -141.0443141357548313 ) ) ;
#38792=CARTESIAN_POINT ( 'NONE',  ( -3.500000000000000000, 19.52072594216370760, -53.04431413575484555 ) ) ;
#38793=CARTESIAN_POINT ( 'NONE',  ( 1.655278471875001101, 20.36702641396249547, -125.0974391362328078 ) ) ;
#38796=CARTESIAN_POINT ( 'NONE',  ( -1.749999999999999778, 20.53108891324555429, -82.12764746908818836 ) ) ;
#38797=CARTESIAN_POINT ( 'NONE',  ( -1.749999999999999778, 20.53108891324555429, -90.12764746908817415 ) ) ;
#38799=CARTESIAN_POINT ( 'NONE',  ( 3.310556943749999981, 15.58864905735836537, -56.34743913623280065 ) ) ;
#38800=CARTESIAN_POINT ( 'NONE',  ( -3.310556943750000425, 19.41135094264166838, -119.9349391362327850 ) ) ;
#38802=CARTESIAN_POINT ( 'NONE',  ( -3.500000000000001332, 17.50000000000001066, -31.65473080337742573 ) ) ;
#38803=FACE_OUTER_BOUND ( 'NONE', #1525, .T. ) ;
#38805=CARTESIAN_POINT ( 'NONE',  ( 1.655278471875001101, 20.36702641396249902, -135.1849391362327992 ) ) ;
#38807=CARTESIAN_POINT ( 'NONE',  ( 0.000000000000000000, 17.50000000000002487, -143.4609808024215170 ) ) ;
#38808=CARTESIAN_POINT ( 'NONE',  ( 2.340729813953370519E-16, 21.32270188528330834, -43.10160580289947063 ) ) ;
#38809=DIRECTION ( 'NONE',  ( -0.000000000000000000, 1.259100132267607459E-16, -1.000000000000000000 ) ) ;
#38810=CARTESIAN_POINT ( 'NONE',  ( -3.310556943750001313, 17.50000000000001421, -66.85160580289947063 ) ) ;
#38811=CARTESIAN_POINT ( 'NONE',  ( -3.310556943750002645, 15.58864905735836892, -64.68077246956615056 ) ) ;
#38812=ORIENTED_EDGE ( 'NONE', *, *, #21423, .F. ) ;
#38813=AXIS2_PLACEMENT_3D ( 'NONE', #11582, #5211, #21792 ) ;
#38814=CARTESIAN_POINT ( 'NONE',  ( -7.022189441860112050E-16, 13.67729811471672363, -84.60160580289947063 ) ) ;
#38816=CARTESIAN_POINT ( 'NONE',  ( 4.648177544792955347E-16, 21.00000000000002132, -116.2109808024215027 ) ) ;
#38817=CARTESIAN_POINT ( 'NONE',  ( -0.9378221735089310451, 14.00000000000001066, -39.75563900116003424 ) ) ;
#38819=CARTESIAN_POINT ( 'NONE',  ( -3.310556943750000425, 19.41135094264166483, -47.84743913623280775 ) ) ;
#38821=CARTESIAN_POINT ( 'NONE',  ( -3.310556943750002645, 15.58864905735837425, -103.6807724695661506 ) ) ;
#38822=( BOUNDED_CURVE ( )  B_SPLINE_CURVE ( 2, ( #3062, #25407, #12841, #25825, #13050, #6464, #19842, #19432, #32809 ),
 .UNSPECIFIED., .F., .F. ) 
 B_SPLINE_CURVE_WITH_KNOTS ( ( 3, 2, 2, 2, 3 ),
 ( 0.8479166666666666519, 0.8486111111111110938, 0.8499999999999999778, 0.8513888888888888618, 0.8520833333333333037 ),
 .UNSPECIFIED. ) 
 CURVE ( )  GEOMETRIC_REPRESENTATION_ITEM ( )  RATIONAL_B_SPLINE_CURVE ( ( 0.9330127018922194093, 0.9330127018922194093, 1.000000000000000000, 0.8660254037844387076, 1.000000000000000000, 0.8660254037844387076, 1.000000000000000000, 0.9330127018922194093, 0.9330127018922194093 ) ) 
 REPRESENTATION_ITEM ( '' )  );
#38827=CARTESIAN_POINT ( 'NONE',  ( 3.310556943750001313, 17.50000000000001421, -58.26410580289947916 ) ) ;
#38828=VERTEX_POINT ( 'NONE', #39918 ) ;
#38829=ORIENTED_EDGE ( 'NONE', *, *, #33970, .T. ) ;
#38830=DIRECTION ( 'NONE',  ( 0.000000000000000000, -1.000000000000000000, 0.000000000000000000 ) ) ;
#38832=EDGE_CURVE ( 'NONE', #24647, #8593, #1422, .T. ) ;
#38834=CARTESIAN_POINT ( 'NONE',  ( 0.9378221735089300459, 21.00000000000002132, -114.2556390011600200 ) ) ;
#38836=DIRECTION ( 'NONE',  ( -0.000000000000000000, 1.259100132267607459E-16, -1.000000000000000000 ) ) ;
#38837=CARTESIAN_POINT ( 'NONE',  ( -3.310556943750000425, 19.41135094264166838, -126.8474391362328078 ) ) ;
#38840=CARTESIAN_POINT ( 'NONE',  ( -1.655278471874999990, 20.36702641396248481, -34.01827246956613493 ) ) ;
#38841=CARTESIAN_POINT ( 'NONE',  ( -3.310556943750001313, 17.50000000000001066, -29.85160580289947063 ) ) ;
#38842=CARTESIAN_POINT ( 'NONE',  ( -1.655278471874999990, 20.36702641396249192, -86.01827246956612782 ) ) ;
#38843=CARTESIAN_POINT ( 'NONE',  ( 1.655278471875001101, 20.36702641396249902, -140.0974391362327935 ) ) ;
#38845=CARTESIAN_POINT ( 'NONE',  ( 3.500000000000001332, 19.52072594216370760, -49.07139747004410424 ) ) ;
#38846=EDGE_CURVE ( 'NONE', #25228, #41613, #18208, .T. ) ;
#38848=CARTESIAN_POINT ( 'NONE',  ( -3.310556943750000425, 19.41135094264167549, -133.9349391362327992 ) ) ;
#38849=FACE_OUTER_BOUND ( 'NONE', #15249, .T. ) ;
#38850=CARTESIAN_POINT ( 'NONE',  ( -1.655278471874999990, 20.36702641396249192, -91.93077246956613635 ) ) ;
#38852=CARTESIAN_POINT ( 'NONE',  ( -1.750000000000002220, 14.46891108675448123, -75.79431413575484555 ) ) ;
#38853=CARTESIAN_POINT ( 'NONE',  ( 3.500000000000001332, 17.50000000000002132, -111.4609808024215027 ) ) ;
#38854=CARTESIAN_POINT ( 'NONE',  ( 3.500000000000001776, 19.52072594216370760, -73.07139747004410424 ) ) ;
#38855=EDGE_CURVE ( 'NONE', #6382, #24201, #37216, .T. ) ;
#38856=CARTESIAN_POINT ( 'NONE',  ( -3.310556943750002201, 15.58864905735836892, -56.76827246956612782 ) ) ;
#38858=CARTESIAN_POINT ( 'NONE',  ( -1.394453263437886604E-15, 14.00000000000002132, -118.4047308033774328 ) ) ;
#38861=CARTESIAN_POINT ( 'NONE',  ( 1.655278471875001101, 20.36702641396249192, -84.18493913623278502 ) ) ;
#38862=CARTESIAN_POINT ( 'NONE',  ( -0.9378221735089310451, 14.00000000000001599, -59.75563900116002003 ) ) ;
#38863=CARTESIAN_POINT ( 'NONE',  ( -3.310556943750002201, 15.58864905735837780, -113.6807724695661364 ) ) ;
#38864=CARTESIAN_POINT ( 'NONE',  ( -7.022189441860112050E-16, 13.67729811471672363, -83.51410580289947916 ) ) ;
#38866=EDGE_LOOP ( 'NONE', ( #30617, #15587, #36037, #38126 ) ) ;
#38867=EDGE_CURVE ( 'NONE', #2948, #19887, #22542, .T. ) ;
#38868=CARTESIAN_POINT ( 'NONE',  ( -1.750000000000002220, 14.46891108675448478, -106.4880641367107614 ) ) ;
#38870=CARTESIAN_POINT ( 'NONE',  ( -0.9378221735089310451, 14.00000000000002132, -94.44938900211595012 ) ) ;
#38871=CARTESIAN_POINT ( 'NONE',  ( 0.9378221735089281585, 14.00000000000001776, -88.36007260463890134 ) ) ;
#38873=CARTESIAN_POINT ( 'NONE',  ( 0.9378221735089300459, 21.00000000000001421, -58.94938900211595012 ) ) ;
#38875=CARTESIAN_POINT ( 'NONE',  ( 1.655278471875001101, 20.36702641396248836, -64.09743913623280775 ) ) ;
#38877=CARTESIAN_POINT ( 'NONE',  ( 3.310556943750001313, 17.50000000000002132, -120.2641058028994792 ) ) ;
#38880=ORIENTED_EDGE ( 'NONE', *, *, #22150, .F. ) ;
#38883=CARTESIAN_POINT ( 'NONE',  ( 3.310556943750001313, 19.41135094264166128, -73.18077246956615056 ) ) ;
#38884=ORIENTED_EDGE ( 'NONE', *, *, #34755, .T. ) ;
#38885=EDGE_LOOP ( 'NONE', ( #39912, #28502, #27101, #26488 ) ) ;
#38890=CARTESIAN_POINT ( 'NONE',  ( -7.022189441860112050E-16, 13.67729811471673074, -141.5141058028994792 ) ) ;
#38891=CARTESIAN_POINT ( 'NONE',  ( 4.648177544792955347E-16, 21.00000000000001066, -45.90473080337741862 ) ) ;
#38892=CARTESIAN_POINT ( 'NONE',  ( 0.000000000000000000, 17.50000000000002487, -149.5231586289125687 ) ) ;
#38893=CARTESIAN_POINT ( 'NONE',  ( 3.310556943750001313, 19.41135094264165772, -45.26827246956613493 ) ) ;
#38894=CARTESIAN_POINT ( 'NONE',  ( 1.655278471874998436, 14.63297358603754716, -101.5182724695661278 ) ) ;
#38895=( BOUNDED_CURVE ( )  B_SPLINE_CURVE ( 2, ( #26327, #4965, #4189, #30712, #10581, #794, #23559, #13345, #20149 ),
 .UNSPECIFIED., .F., .T. ) 
 B_SPLINE_CURVE_WITH_KNOTS ( ( 3, 2, 2, 2, 3 ),
 ( 0.7062500000000000444, 0.7069444444444444864, 0.7083333333333333703, 0.7097222222222222543, 0.7104166666666666963 ),
 .UNSPECIFIED. ) 
 CURVE ( )  GEOMETRIC_REPRESENTATION_ITEM ( )  RATIONAL_B_SPLINE_CURVE ( ( 0.9330127018922194093, 0.9330127018922194093, 1.000000000000000000, 0.8660254037844387076, 1.000000000000000000, 0.8660254037844387076, 1.000000000000000000, 0.9330127018922194093, 0.9330127018922194093 ) ) 
 REPRESENTATION_ITEM ( '' )  );
#38896=CARTESIAN_POINT ( 'NONE',  ( -7.022189441860112050E-16, 13.67729811471671475, -31.51410580289946850 ) ) ;
#38898=CARTESIAN_POINT ( 'NONE',  ( 2.474675557024783212E-16, 21.54145188432740099, -109.2109808024215027 ) ) ;
#38900=CARTESIAN_POINT ( 'NONE',  ( -1.394453263437886604E-15, 14.00000000000001421, -62.71098080242150274 ) ) ;
#38901=CARTESIAN_POINT ( 'NONE',  ( 3.500000000000000000, 15.47927405783632615, -94.23806413671077564 ) ) ;
#38906=CARTESIAN_POINT ( 'NONE',  ( 3.500000000000000000, 15.47927405783632260, -58.54431413575483845 ) ) ;
#38907=CARTESIAN_POINT ( 'NONE',  ( -0.9378221735089291577, 21.00000000000001066, -30.86007260463891200 ) ) ;
#38908=DIRECTION ( 'NONE',  ( -0.000000000000000000, 1.259100132267607459E-16, -1.000000000000000000 ) ) ;
#38909=EDGE_CURVE ( 'NONE', #10596, #5345, #24188, .T. ) ;
#38910=CARTESIAN_POINT ( 'NONE',  ( -3.500000000000002220, 15.47927405783632260, -47.57139747004409713 ) ) ;
#38911=CARTESIAN_POINT ( 'NONE',  ( 3.500000000000001332, 19.52072594216371826, -106.3776474690881741 ) ) ;
#38912=CARTESIAN_POINT ( 'NONE',  ( -7.022189441860112050E-16, 13.67729811471671653, -32.60160580289946353 ) ) ;
#38915=CARTESIAN_POINT ( 'NONE',  ( 3.500000000000001332, 17.50000000000001421, -50.15473080337742573 ) ) ;
#38918=CARTESIAN_POINT ( 'NONE',  ( 0.000000000000000000, 21.00000000000002487, -149.5231586289125687 ) ) ;
#38920=CARTESIAN_POINT ( 'NONE',  ( 3.310556943750001313, 17.50000000000001776, -81.26410580289947916 ) ) ;
#38923=ORIENTED_EDGE ( 'NONE', *, *, #11895, .F. ) ;
#38924=CARTESIAN_POINT ( 'NONE',  ( -1.394453263437886604E-15, 14.00000000000002132, -123.7109808024214885 ) ) ;
#38925=ORIENTED_EDGE ( 'NONE', *, *, #21454, .T. ) ;
#38927=CYLINDRICAL_SURFACE ( 'NONE', #36923, 3.499999999999999556 ) ;
#38928=CARTESIAN_POINT ( 'NONE',  ( 1.655278471874998436, 14.63297358603754539, -92.43077246956613635 ) ) ;
#38930=CYLINDRICAL_SURFACE ( 'NONE', #4653, 3.499999999999999556 ) ;
#38933=CARTESIAN_POINT ( 'NONE',  ( -3.500000000000002220, 15.47927405783632970, -84.57139747004409003 ) ) ;
#38935=CARTESIAN_POINT ( 'NONE',  ( -1.750000000000002220, 14.46891108675448301, -88.48806413671076143 ) ) ;
#38938=CARTESIAN_POINT ( 'NONE',  ( 3.310556943749999981, 15.58864905735837425, -130.3474391362328220 ) ) ;
#38941=CARTESIAN_POINT ( 'NONE',  ( 3.500000000000000000, 15.47927405783633503, -139.2380641367107614 ) ) ;
#38942=CARTESIAN_POINT ( 'NONE',  ( -7.022189441860112050E-16, 13.67729811471672718, -120.6016058028994564 ) ) ;
#38943=CARTESIAN_POINT ( 'NONE',  ( -3.310556943750000425, 19.41135094264166128, -52.93493913623280633 ) ) ;
#38946=CARTESIAN_POINT ( 'NONE',  ( 3.500000000000001776, 19.52072594216371826, -129.0713974700440758 ) ) ;
#38947=( BOUNDED_CURVE ( )  B_SPLINE_CURVE ( 2, ( #24962, #41960, #28964, #2821, #41120, #19194, #31328, #12808, #28551 ),
 .UNSPECIFIED., .F., .T. ) 
 B_SPLINE_CURVE_WITH_KNOTS ( ( 3, 2, 2, 2, 3 ),
 ( 0.9229166666666667185, 0.9236111111111111605, 0.9250000000000000444, 0.9263888888888889284, 0.9270833333333333703 ),
 .UNSPECIFIED. ) 
 CURVE ( )  GEOMETRIC_REPRESENTATION_ITEM ( )  RATIONAL_B_SPLINE_CURVE ( ( 0.9330127018922194093, 0.9330127018922194093, 1.000000000000000000, 0.8660254037844387076, 1.000000000000000000, 0.8660254037844387076, 1.000000000000000000, 0.9330127018922194093, 0.9330127018922194093 ) ) 
 REPRESENTATION_ITEM ( '' )  );
#38948=CIRCLE ( 'NONE', #948, 3.499999999999999556 ) ;
#38949=CARTESIAN_POINT ( 'NONE',  ( 3.310556943749999981, 15.58864905735836714, -72.43493913623278502 ) ) ;
#38950=CARTESIAN_POINT ( 'NONE',  ( -1.750000000000002220, 14.46891108675448656, -121.7943141357548456 ) ) ;
#38951=CARTESIAN_POINT ( 'NONE',  ( -1.655278471874999990, 20.36702641396249547, -104.9307724695661364 ) ) ;
#38953=CARTESIAN_POINT ( 'NONE',  ( -3.500000000000000000, 19.52072594216371826, -107.7380641367107756 ) ) ;
#38956=CARTESIAN_POINT ( 'NONE',  ( -3.500000000000000888, 19.52072594216371115, -77.04431413575484555 ) ) ;
#38957=CYLINDRICAL_SURFACE ( 'NONE', #39564, 3.499999999999999556 ) ;
#38958=CARTESIAN_POINT ( 'NONE',  ( -3.310556943750000425, 19.41135094264165772, -42.84743913623280065 ) ) ;
#38959=CARTESIAN_POINT ( 'NONE',  ( 1.655278471874998436, 14.63297358603754539, -93.51827246956612782 ) ) ;
#38960=CARTESIAN_POINT ( 'NONE',  ( 1.750000000000001110, 20.53108891324555074, -66.98806413671076143 ) ) ;
#38961=CARTESIAN_POINT ( 'NONE',  ( 4.648177544792955347E-16, 21.00000000000001066, -39.21098080242150985 ) ) ;
#38962=CARTESIAN_POINT ( 'NONE',  ( 3.310556943749999981, 15.58864905735837247, -116.4349391362327850 ) ) ;
#38968=CARTESIAN_POINT ( 'NONE',  ( 1.655278471874998436, 14.63297358603754716, -100.4307724695661364 ) ) ;
#38971=EDGE_LOOP ( 'NONE', ( #39025, #18543, #23509, #16095 ) ) ;
#38972=CARTESIAN_POINT ( 'NONE',  ( -3.500000000000002220, 15.47927405783632082, -28.87764746908817770 ) ) ;
#38973=CARTESIAN_POINT ( 'NONE',  ( -1.750000000000002220, 14.46891108675448656, -118.4880641367107614 ) ) ;
#38974=AXIS2_PLACEMENT_3D ( 'NONE', #27209, #23812, #40173 ) ;
#38975=CARTESIAN_POINT ( 'NONE',  ( 0.9378221735089300459, 21.00000000000002132, -122.9493890021159359 ) ) ;
#38979=CARTESIAN_POINT ( 'NONE',  ( 1.655278471874998436, 14.63297358603753828, -27.43077246956614346 ) ) ;
#38985=ORIENTED_EDGE ( 'NONE', *, *, #3592, .F. ) ;
#38987=CARTESIAN_POINT ( 'NONE',  ( 3.500000000000001332, 19.52072594216371115, -90.37764746908817415 ) ) ;
#38988=CARTESIAN_POINT ( 'NONE',  ( 1.750000000000001110, 20.53108891324554719, -30.98806413671076498 ) ) ;
#38989=CARTESIAN_POINT ( 'NONE',  ( 2.474675557024783212E-16, 21.54145188432740099, -120.9047308033774328 ) ) ;
#38991=CARTESIAN_POINT ( 'NONE',  ( 3.310556943750001313, 17.50000000000002487, -133.3516058028994564 ) ) ;
#38992=CARTESIAN_POINT ( 'NONE',  ( -1.750000000000002220, 14.46891108675447590, -31.79431413575484200 ) ) ;
#38993=CARTESIAN_POINT ( 'NONE',  ( -0.9378221735089310451, 14.00000000000001599, -65.75563900116003424 ) ) ;
#38994=LINE ( 'NONE', #29192, #4747 ) ;
#38997=CARTESIAN_POINT ( 'NONE',  ( -7.424026671074350129E-16, 13.45854811567264164, -140.7109808024214885 ) ) ;
#38998=CARTESIAN_POINT ( 'NONE',  ( 2.340729813953370519E-16, 21.32270188528331900, -121.0141058028994792 ) ) ;
#38999=ADVANCED_FACE ( 'NONE', ( #31175 ), #15232, .T. ) ;
#39002=CYLINDRICAL_SURFACE ( 'NONE', #25924, 3.499999999999999556 ) ;
#39003=CARTESIAN_POINT ( 'NONE',  ( 3.500000000000001776, 19.52072594216371115, -91.37764746908817415 ) ) ;
#39004=CARTESIAN_POINT ( 'NONE',  ( -1.394453263437886604E-15, 14.00000000000001066, -33.40473080337742573 ) ) ;
#39005=CARTESIAN_POINT ( 'NONE',  ( -1.655278471874999990, 20.36702641396248836, -56.93077246956614346 ) ) ;
#39006=CARTESIAN_POINT ( 'NONE',  ( -3.310556943750002645, 15.58864905735837780, -109.7682724695661278 ) ) ;
#39007=CARTESIAN_POINT ( 'NONE',  ( -1.394453263437886604E-15, 14.00000000000002132, -121.7109808024215170 ) ) ;
#39008=CARTESIAN_POINT ( 'NONE',  ( -1.750000000000002220, 14.46891108675447590, -34.48806413671076854 ) ) ;
#39009=CARTESIAN_POINT ( 'NONE',  ( -1.750000000000002220, 14.46891108675448656, -121.4880641367107614 ) ) ;
#39011=CARTESIAN_POINT ( 'NONE',  ( -1.655278471874999990, 20.36702641396249902, -134.0182724695661420 ) ) ;
#39014=CARTESIAN_POINT ( 'NONE',  ( 1.655278471874998436, 14.63297358603754361, -71.51827246956612782 ) ) ;
#39016=ORIENTED_EDGE ( 'NONE', *, *, #24827, .F. ) ;
#39017=CARTESIAN_POINT ( 'NONE',  ( -7.022189441860112050E-16, 13.67729811471672363, -87.60160580289947063 ) ) ;
#39021=CARTESIAN_POINT ( 'NONE',  ( 3.310556943750001313, 17.50000000000001421, -51.26410580289947205 ) ) ;
#39023=CARTESIAN_POINT ( 'NONE',  ( 2.340729813953370519E-16, 21.32270188528331900, -103.0141058028994792 ) ) ;
#39025=ORIENTED_EDGE ( 'NONE', *, *, #7083, .F. ) ;
#39030=CARTESIAN_POINT ( 'NONE',  ( -1.655278471875002211, 14.63297358603754361, -59.59743913623280775 ) ) ;
#39031=VERTEX_POINT ( 'NONE', #34575 ) ;
#39033=DIRECTION ( 'NONE',  ( 0.000000000000000000, 1.000000000000000000, 0.000000000000000000 ) ) ;
#39034=VECTOR ( 'NONE', #21784, 1000.000000000000000 ) ;
#39035=FACE_OUTER_BOUND ( 'NONE', #25230, .T. ) ;
#39041=CARTESIAN_POINT ( 'NONE',  ( 3.310556943749999981, 15.58864905735837425, -124.3474391362328078 ) ) ;
#39042=EDGE_CURVE ( 'NONE', #14962, #9702, #6066, .T. ) ;
#39043=LINE ( 'NONE', #35439, #28472 ) ;
#39045=CARTESIAN_POINT ( 'NONE',  ( -3.310556943750001313, 17.50000000000001066, -32.85160580289946353 ) ) ;
#39046=CARTESIAN_POINT ( 'NONE',  ( 1.655278471874998436, 14.63297358603753651, -24.51827246956613138 ) ) ;
#39047=CARTESIAN_POINT ( 'NONE',  ( -3.310556943750002645, 15.58864905735837247, -86.76827246956612782 ) ) ;
#39048=CARTESIAN_POINT ( 'NONE',  ( 1.655278471875001101, 20.36702641396249902, -137.0974391362328220 ) ) ;
#39053=CARTESIAN_POINT ( 'NONE',  ( -1.655278471874999990, 20.36702641396249902, -131.0182724695661136 ) ) ;
#39055=CARTESIAN_POINT ( 'NONE',  ( -1.655278471875002211, 14.63297358603754716, -90.59743913623280775 ) ) ;
#39056=CARTESIAN_POINT ( 'NONE',  ( 7.367361408496833051E-14, 14.00000000000001776, -95.71098080242150274 ) ) ;
#39057=LINE ( 'NONE', #9941, #32036 ) ;
#39058=CARTESIAN_POINT ( 'NONE',  ( 4.648177544792955347E-16, 21.00000000000002487, -131.9047308033774186 ) ) ;
#39059=CARTESIAN_POINT ( 'NONE',  ( -7.424026671074350129E-16, 13.45854811567263454, -76.40473080337743284 ) ) ;
#39060=CARTESIAN_POINT ( 'NONE',  ( -3.310556943750001313, 17.50000000000001421, -58.85160580289947063 ) ) ;
#39064=CARTESIAN_POINT ( 'NONE',  ( 1.655278471874998436, 14.63297358603754539, -85.51827246956612782 ) ) ;
#39065=CARTESIAN_POINT ( 'NONE',  ( -1.655278471875002211, 14.63297358603755072, -112.5974391362328078 ) ) ;
#39066=CARTESIAN_POINT ( 'NONE',  ( -1.655278471875002211, 14.63297358603754539, -79.59743913623280775 ) ) ;
#39069=ORIENTED_EDGE ( 'NONE', *, *, #14997, .F. ) ;
#39070=CARTESIAN_POINT ( 'NONE',  ( 3.310556943750001313, 17.50000000000002132, -103.3516058028994564 ) ) ;
#39071=CARTESIAN_POINT ( 'NONE',  ( -3.500000000000000888, 19.52072594216371115, -101.7380641367107756 ) ) ;
#39072=( BOUNDED_CURVE ( )  B_SPLINE_CURVE ( 2, ( #1848, #38416, #9280, #34387, #34803, #15251, #18646, #31192, #27795 ),
 .UNSPECIFIED., .F., .T. ) 
 B_SPLINE_CURVE_WITH_KNOTS ( ( 3, 2, 2, 2, 3 ),
 ( 0.002083333333333334605, 0.002777777777777777884, 0.004166666666666666609, 0.005555555555555555768, 0.006250000000000000347 ),
 .UNSPECIFIED. ) 
 CURVE ( )  GEOMETRIC_REPRESENTATION_ITEM ( )  RATIONAL_B_SPLINE_CURVE ( ( 0.9330127018922192983, 0.9330127018922194093, 1.000000000000000000, 0.8660254037844387076, 1.000000000000000000, 0.8660254037844387076, 1.000000000000000000, 0.9330127018922192983, 0.9330127018922194093 ) ) 
 REPRESENTATION_ITEM ( '' )  );
#39079=CARTESIAN_POINT ( 'NONE',  ( 3.310556943750001313, 19.41135094264166483, -66.18077246956613635 ) ) ;
#39081=CARTESIAN_POINT ( 'NONE',  ( 2.340729813953370519E-16, 21.32270188528331900, -121.0141058028994792 ) ) ;
#39082=CARTESIAN_POINT ( 'NONE',  ( 3.500000000000001332, 17.50000000000001421, -71.15473080337743284 ) ) ;
#39083=CARTESIAN_POINT ( 'NONE',  ( -1.394453263437886604E-15, 14.00000000000002132, -125.4047308033774186 ) ) ;
#39085=CARTESIAN_POINT ( 'NONE',  ( -1.750000000000002220, 14.46891108675448478, -103.7943141357548456 ) ) ;
#39087=CARTESIAN_POINT ( 'NONE',  ( 1.655278471875001101, 20.36702641396248836, -73.09743913623280775 ) ) ;
#39088=VERTEX_POINT ( 'NONE', #12454 ) ;
#39089=ORIENTED_EDGE ( 'NONE', *, *, #38381, .T. ) ;
#39092=CARTESIAN_POINT ( 'NONE',  ( -3.310556943750002201, 15.58864905735837958, -140.6807724695661364 ) ) ;
#39094=CARTESIAN_POINT ( 'NONE',  ( -3.310556943750002645, 15.58864905735836714, -42.76827246956613493 ) ) ;
#39095=CARTESIAN_POINT ( 'NONE',  ( 3.310556943750001313, 19.41135094264166838, -105.2682724695661278 ) ) ;
#39096=CARTESIAN_POINT ( 'NONE',  ( 1.655278471875001101, 20.36702641396248481, -27.09743913623280420 ) ) ;
#39098=CARTESIAN_POINT ( 'NONE',  ( 3.500000000000000000, 15.47927405783632793, -103.5443141357548456 ) ) ;
#39101=CARTESIAN_POINT ( 'NONE',  ( 1.750000000000001110, 20.53108891324555429, -88.98806413671076143 ) ) ;
#39102=CARTESIAN_POINT ( 'NONE',  ( -3.500000000000000000, 19.52072594216371115, -78.04431413575485976 ) ) ;
#39104=ADVANCED_FACE ( 'NONE', ( #2879 ), #15871, .T. ) ;
#39106=CARTESIAN_POINT ( 'NONE',  ( 2.474675557024783212E-16, 21.54145188432739388, -51.21098080242150274 ) ) ;
#39108=CARTESIAN_POINT ( 'NONE',  ( 4.648177544792955347E-16, 21.00000000000001066, -36.21098080242150985 ) ) ;
#39110=CARTESIAN_POINT ( 'NONE',  ( -7.424026671074350129E-16, 13.45854811567263276, -41.40473080337743284 ) ) ;
#39112=CARTESIAN_POINT ( 'NONE',  ( -7.022189441860112050E-16, 13.67729811471671653, -27.60160580289947063 ) ) ;
#39114=CARTESIAN_POINT ( 'NONE',  ( 4.648177544792955347E-16, 21.00000000000001776, -99.21098080242150274 ) ) ;
#39115=CARTESIAN_POINT ( 'NONE',  ( 4.648177544792955347E-16, 21.00000000000001066, -37.21098080242150985 ) ) ;
#39119=CARTESIAN_POINT ( 'NONE',  ( 1.655278471874998436, 14.63297358603754539, -82.43077246956615056 ) ) ;
#39121=EDGE_LOOP ( 'NONE', ( #31924, #19681, #18261, #35540 ) ) ;
#39123=CARTESIAN_POINT ( 'NONE',  ( 0.9378221735089281585, 14.00000000000001776, -87.66632260368299967 ) ) ;
#39126=CARTESIAN_POINT ( 'NONE',  ( 1.655278471874998436, 14.63297358603754539, -88.43077246956613635 ) ) ;
#39132=( BOUNDED_CURVE ( )  B_SPLINE_CURVE ( 2, ( #29116, #19553, #12759, #22325, #6376, #5953, #38496, #25532, #19142 ),
 .UNSPECIFIED., .F., .F. ) 
 B_SPLINE_CURVE_WITH_KNOTS ( ( 3, 2, 2, 2, 3 ),
 ( 0.01041666666666666782, 0.01111111111111111154, 0.01250000000000000069, 0.01388888888888888812, 0.01458333333333333356 ),
 .UNSPECIFIED. ) 
 CURVE ( )  GEOMETRIC_REPRESENTATION_ITEM ( )  RATIONAL_B_SPLINE_CURVE ( ( 0.9330127018922192983, 0.9330127018922194093, 1.000000000000000000, 0.8660254037844387076, 1.000000000000000000, 0.8660254037844387076, 1.000000000000000000, 0.9330127018922191873, 0.9330127018922192983 ) ) 
 REPRESENTATION_ITEM ( '' )  );
#39134=LINE ( 'NONE', #15993, #14674 ) ;
#39135=ADVANCED_FACE ( 'NONE', ( #18834 ), #31794, .T. ) ;
#39136=CARTESIAN_POINT ( 'NONE',  ( -1.655278471875002211, 14.63297358603755249, -133.5974391362328220 ) ) ;
#39138=EDGE_LOOP ( 'NONE', ( #28304, #19790, #35952, #27876 ) ) ;
#39140=CARTESIAN_POINT ( 'NONE',  ( 2.340729813953370519E-16, 21.32270188528331900, -121.1016058028994706 ) ) ;
#39141=VERTEX_POINT ( 'NONE', #2250 ) ;
#39143=CARTESIAN_POINT ( 'NONE',  ( 3.500000000000000000, 15.47927405783633503, -131.2380641367107614 ) ) ;
#39144=CARTESIAN_POINT ( 'NONE',  ( -3.310556943750000425, 19.41135094264166128, -70.93493913623278502 ) ) ;
#39145=CARTESIAN_POINT ( 'NONE',  ( -3.500000000000000888, 19.52072594216371826, -118.0443141357548313 ) ) ;
#39146=CARTESIAN_POINT ( 'NONE',  ( 2.340729813953370519E-16, 21.32270188528331900, -104.0141058028994649 ) ) ;
#39150=CARTESIAN_POINT ( 'NONE',  ( -1.750000000000002220, 14.46891108675448123, -77.79431413575484555 ) ) ;
#39152=CARTESIAN_POINT ( 'NONE',  ( 3.310556943750001313, 19.41135094264165772, -38.18077246956614346 ) ) ;
#39153=CARTESIAN_POINT ( 'NONE',  ( -3.310556943750000425, 19.41135094264166483, -96.93493913623281344 ) ) ;
#39154=CARTESIAN_POINT ( 'NONE',  ( -3.500000000000000888, 19.52072594216370760, -66.73806413671076143 ) ) ;
#39156=CARTESIAN_POINT ( 'NONE',  ( -1.655278471874999990, 20.36702641396249547, -119.0182724695661278 ) ) ;
#39157=CARTESIAN_POINT ( 'NONE',  ( -3.500000000000000000, 19.52072594216370760, -62.73806413671076143 ) ) ;
#39162=CARTESIAN_POINT ( 'NONE',  ( 1.655278471874998436, 14.63297358603754716, -96.43077246956613635 ) ) ;
#39163=CARTESIAN_POINT ( 'NONE',  ( 3.500000000000001332, 17.50000000000001421, -62.46098080242150274 ) ) ;
#39165=EDGE_LOOP ( 'NONE', ( #36480, #22088, #93, #35150 ) ) ;
#39166=CARTESIAN_POINT ( 'NONE',  ( 4.648177544792955347E-16, 21.00000000000001066, -26.90473080337742928 ) ) ;
#39167=EDGE_CURVE ( 'NONE', #19669, #25746, #6524, .T. ) ;
#39168=CARTESIAN_POINT ( 'NONE',  ( 4.648177544792955347E-16, 21.00000000000001421, -47.90473080337742573 ) ) ;
#39169=CARTESIAN_POINT ( 'NONE',  ( 4.648177544792955347E-16, 21.00000000000001066, -30.21098080242151340 ) ) ;
#39170=EDGE_LOOP ( 'NONE', ( #41789, #41709, #24398, #2729 ) ) ;
#39175=CARTESIAN_POINT ( 'NONE',  ( 3.310556943749999981, 15.58864905735836182, -31.34743913623280775 ) ) ;
#39176=VERTEX_POINT ( 'NONE', #97 ) ;
#39177=CARTESIAN_POINT ( 'NONE',  ( -1.394453263437886604E-15, 14.00000000000002132, -109.4047308033774186 ) ) ;
#39182=VERTEX_POINT ( 'NONE', #3918 ) ;
#39184=( BOUNDED_CURVE ( )  B_SPLINE_CURVE ( 2, ( #33149, #33363, #30388, #10824, #36559, #4231, #39752, #7217, #26995 ),
 .UNSPECIFIED., .F., .T. ) 
 B_SPLINE_CURVE_WITH_KNOTS ( ( 3, 2, 2, 2, 3 ),
 ( 0.5770833333333332815, 0.5777777777777777235, 0.5791666666666667185, 0.5805555555555556024, 0.5812500000000000444 ),
 .UNSPECIFIED. ) 
 CURVE ( )  GEOMETRIC_REPRESENTATION_ITEM ( )  RATIONAL_B_SPLINE_CURVE ( ( 0.9330127018922194093, 0.9330127018922194093, 1.000000000000000000, 0.8660254037844387076, 1.000000000000000000, 0.8660254037844387076, 1.000000000000000000, 0.9330127018922194093, 0.9330127018922194093 ) ) 
 REPRESENTATION_ITEM ( '' )  );
#39185=CARTESIAN_POINT ( 'NONE',  ( -1.750000000000002220, 14.46891108675448301, -85.79431413575483134 ) ) ;
#39186=EDGE_CURVE ( 'NONE', #32852, #23778, #12484, .T. ) ;
#39187=CARTESIAN_POINT ( 'NONE',  ( -1.750000000000002220, 14.46891108675448656, -119.4880641367107614 ) ) ;
#39188=CARTESIAN_POINT ( 'NONE',  ( -1.750000000000002220, 14.46891108675448656, -118.4880641367107614 ) ) ;
#39189=CARTESIAN_POINT ( 'NONE',  ( -1.394453263437886604E-15, 14.00000000000001421, -59.40473080337742573 ) ) ;
#39190=CARTESIAN_POINT ( 'NONE',  ( 1.655278471875001101, 20.36702641396249902, -136.1849391362327992 ) ) ;
#39191=CARTESIAN_POINT ( 'NONE',  ( -3.500000000000000888, 19.52072594216370405, -26.04431413575483489 ) ) ;
#39195=CARTESIAN_POINT ( 'NONE',  ( -1.750000000000002220, 14.46891108675449011, -139.7943141357548313 ) ) ;
#39196=CARTESIAN_POINT ( 'NONE',  ( -1.655278471875002211, 14.63297358603755072, -120.5974391362328078 ) ) ;
#39199=DIRECTION ( 'NONE',  ( 0.000000000000000000, 1.000000000000000000, 0.000000000000000000 ) ) ;
#39200=CARTESIAN_POINT ( 'NONE',  ( -1.750000000000002220, 14.46891108675448301, -89.79431413575483134 ) ) ;
#39202=CARTESIAN_POINT ( 'NONE',  ( -3.310556943750001313, 17.50000000000001421, -55.76410580289947916 ) ) ;
#39203=CARTESIAN_POINT ( 'NONE',  ( -3.310556943750001313, 17.50000000000002132, -112.8516058028994564 ) ) ;
#39205=CARTESIAN_POINT ( 'NONE',  ( 1.749999999999998224, 14.46891108675447413, -32.32139747004410424 ) ) ;
#39208=CARTESIAN_POINT ( 'NONE',  ( 3.310556943749999981, 15.58864905735837425, -133.4349391362327992 ) ) ;
#39210=CARTESIAN_POINT ( 'NONE',  ( 4.648177544792955347E-16, 21.00000000000001066, -31.21098080242150630 ) ) ;
#39212=CARTESIAN_POINT ( 'NONE',  ( -3.310556943750001313, 17.50000000000001421, -61.85160580289945642 ) ) ;
#39214=CARTESIAN_POINT ( 'NONE',  ( 1.655278471874998436, 14.63297358603754184, -62.43077246956614346 ) ) ;
#39215=ORIENTED_EDGE ( 'NONE', *, *, #8589, .F. ) ;
#39216=CARTESIAN_POINT ( 'NONE',  ( -3.310556943750001313, 17.50000000000001776, -85.85160580289947063 ) ) ;
#39217=EDGE_CURVE ( 'NONE', #11828, #644, #26062, .T. ) ;
#39220=CARTESIAN_POINT ( 'NONE',  ( -3.310556943750001313, 17.50000000000001066, -43.76410580289947916 ) ) ;
#39222=CARTESIAN_POINT ( 'NONE',  ( 3.310556943750001313, 19.41135094264166838, -108.1807724695661506 ) ) ;
#39223=CARTESIAN_POINT ( 'NONE',  ( -1.394453263437886604E-15, 14.00000000000001066, -42.40473080337742573 ) ) ;
#39230=CARTESIAN_POINT ( 'NONE',  ( 1.655278471874998436, 14.63297358603754184, -58.43077246956614346 ) ) ;
#39231=ORIENTED_EDGE ( 'NONE', *, *, #3512, .T. ) ;
#39232=EDGE_LOOP ( 'NONE', ( #39385, #22278, #6848, #4301 ) ) ;
#39234=CARTESIAN_POINT ( 'NONE',  ( 4.648177544792955347E-16, 21.00000000000001776, -91.21098080242150274 ) ) ;
#39237=CARTESIAN_POINT ( 'NONE',  ( 1.749999999999998224, 14.46891108675448478, -114.6276474690881741 ) ) ;
#39239=CARTESIAN_POINT ( 'NONE',  ( -0.9378221735089291577, 21.00000000000001066, -39.16632260368298546 ) ) ;
#39240=CARTESIAN_POINT ( 'NONE',  ( -1.655278471874999990, 20.36702641396249547, -123.9307724695661364 ) ) ;
#39243=CARTESIAN_POINT ( 'NONE',  ( -3.310556943750002645, 15.58864905735836537, -32.76827246956613493 ) ) ;
#39244=CARTESIAN_POINT ( 'NONE',  ( 3.310556943749999981, 15.58864905735836004, -23.43493913623280633 ) ) ;
#39245=CARTESIAN_POINT ( 'NONE',  ( -1.655278471874999990, 20.36702641396249192, -88.01827246956612782 ) ) ;
#39246=CARTESIAN_POINT ( 'NONE',  ( -1.655278471875002211, 14.63297358603755427, -141.5974391362327935 ) ) ;
#39248=CARTESIAN_POINT ( 'NONE',  ( 4.648177544792955347E-16, 21.00000000000002132, -126.9047308033774186 ) ) ;
#39249=CARTESIAN_POINT ( 'NONE',  ( -1.750000000000002220, 14.46891108675447946, -66.79431413575484555 ) ) ;
#39250=CARTESIAN_POINT ( 'NONE',  ( -1.655278471875002211, 14.63297358603755249, -125.6849391362327992 ) ) ;
#39251=DIRECTION ( 'NONE',  ( -0.000000000000000000, 1.259100132267607459E-16, -1.000000000000000000 ) ) ;
#39252=CARTESIAN_POINT ( 'NONE',  ( 2.340729813953370519E-16, 21.32270188528331190, -91.01410580289947916 ) ) ;
#39254=CARTESIAN_POINT ( 'NONE',  ( -3.500000000000002220, 15.47927405783632970, -92.87764746908815994 ) ) ;
#39256=ADVANCED_FACE ( 'NONE', ( #25853 ), #23064, .T. ) ;
#39257=CARTESIAN_POINT ( 'NONE',  ( -3.500000000000000888, 19.52072594216371115, -74.73806413671076143 ) ) ;
#39258=CARTESIAN_POINT ( 'NONE',  ( -3.310556943750002201, 15.58864905735836892, -57.76827246956613493 ) ) ;
#39260=CYLINDRICAL_SURFACE ( 'NONE', #19038, 3.499999999999999556 ) ;
#39261=CARTESIAN_POINT ( 'NONE',  ( -1.394453263437886604E-15, 14.00000000000001776, -100.7109808024215027 ) ) ;
#39262=CARTESIAN_POINT ( 'NONE',  ( 3.310556943749999981, 15.58864905735836892, -84.43493913623278502 ) ) ;
#39263=CARTESIAN_POINT ( 'NONE',  ( -1.749999999999999778, 20.53108891324555429, -77.82139747004410424 ) ) ;
#39265=CARTESIAN_POINT ( 'NONE',  ( -7.022189441860112050E-16, 13.67729811471672896, -111.5141058028994507 ) ) ;
#39266=CARTESIAN_POINT ( 'NONE',  ( 3.310556943750001313, 17.50000000000001776, -79.26410580289946495 ) ) ;
#39269=CARTESIAN_POINT ( 'NONE',  ( -3.310556943750001313, 17.50000000000001776, -101.8516058028994706 ) ) ;
#39270=CARTESIAN_POINT ( 'NONE',  ( -1.749999999999999778, 20.53108891324555785, -104.8213974700441042 ) ) ;
#39273=CARTESIAN_POINT ( 'NONE',  ( -1.394453263437886604E-15, 14.00000000000001066, -34.40473080337743284 ) ) ;
#39276=CARTESIAN_POINT ( 'NONE',  ( -3.310556943750002201, 15.58864905735836892, -61.68077246956614346 ) ) ;
#39277=CARTESIAN_POINT ( 'NONE',  ( -1.655278471875002211, 14.63297358603755072, -122.5974391362328078 ) ) ;
#39278=CARTESIAN_POINT ( 'NONE',  ( -1.394453263437886604E-15, 14.00000000000001776, -99.71098080242150274 ) ) ;
#39284=CARTESIAN_POINT ( 'NONE',  ( 0.9378221735089367073, 14.00000000000002487, -128.3600726046389013 ) ) ;
#39285=ADVANCED_FACE ( 'NONE', ( #13487 ), #13706, .T. ) ;
#39286=CARTESIAN_POINT ( 'NONE',  ( 1.655278471874998436, 14.63297358603754361, -71.43077246956613635 ) ) ;
#39287=VERTEX_POINT ( 'NONE', #35629 ) ;
#39289=CARTESIAN_POINT ( 'NONE',  ( 4.648177544792955347E-16, 21.00000000000001421, -54.90473080337742573 ) ) ;
#39291=CARTESIAN_POINT ( 'NONE',  ( 3.310556943749999981, 15.58864905735837780, -139.3474391362327935 ) ) ;
#39292=CARTESIAN_POINT ( 'NONE',  ( 1.743066579297357930E-14, 14.00000000000002132, -128.7109808024214885 ) ) ;
#39295=CARTESIAN_POINT ( 'NONE',  ( -1.655278471875002211, 14.63297358603754006, -37.68493913623280633 ) ) ;
#39296=CARTESIAN_POINT ( 'NONE',  ( -7.022189441860112050E-16, 13.67729811471672541, -105.6016058028994422 ) ) ;
#39298=( BOUNDED_CURVE ( )  B_SPLINE_CURVE ( 2, ( #29631, #39407, #38796, #3069, #16261, #42000, #9669, #6471, #19849 ),
 .UNSPECIFIED., .F., .F. ) 
 B_SPLINE_CURVE_WITH_KNOTS ( ( 3, 2, 2, 2, 3 ),
 ( 0.5104166666666666297, 0.5111111111111110716, 0.5124999999999999556, 0.5138888888888888395, 0.5145833333333332815 ),
 .UNSPECIFIED. ) 
 CURVE ( )  GEOMETRIC_REPRESENTATION_ITEM ( )  RATIONAL_B_SPLINE_CURVE ( ( 0.9330127018922194093, 0.9330127018922194093, 1.000000000000000000, 0.8660254037844387076, 1.000000000000000000, 0.8660254037844387076, 1.000000000000000000, 0.9330127018922194093, 0.9330127018922194093 ) ) 
 REPRESENTATION_ITEM ( '' )  );
#39299=( BOUNDED_CURVE ( )  B_SPLINE_CURVE ( 2, ( #40383, #24020, #10822, #7854, #23807, #36772, #27616, #34202, #7634 ),
 .UNSPECIFIED., .F., .T. ) 
 B_SPLINE_CURVE_WITH_KNOTS ( ( 3, 2, 2, 2, 3 ),
 ( 0.2729166666666666963, 0.2736111111111111382, 0.2750000000000000222, 0.2763888888888889062, 0.2770833333333333481 ),
 .UNSPECIFIED. ) 
 CURVE ( )  GEOMETRIC_REPRESENTATION_ITEM ( )  RATIONAL_B_SPLINE_CURVE ( ( 0.9330127018922194093, 0.9330127018922220739, 1.000000000000000000, 0.8660254037844387076, 1.000000000000000000, 0.8660254037844387076, 1.000000000000000000, 0.9330127018922194093, 0.9330127018922194093 ) ) 
 REPRESENTATION_ITEM ( '' )  );
#39300=CARTESIAN_POINT ( 'NONE',  ( 3.310556943750001313, 19.41135094264165772, -25.18077246956613635 ) ) ;
#39302=CARTESIAN_POINT ( 'NONE',  ( -3.500000000000000888, 19.52072594216371115, -101.0443141357548456 ) ) ;
#39304=DIRECTION ( 'NONE',  ( -0.000000000000000000, 1.259100132267607459E-16, -1.000000000000000000 ) ) ;
#39305=CARTESIAN_POINT ( 'NONE',  ( 3.500000000000000000, 15.47927405783632615, -90.23806413671076143 ) ) ;
#39309=CARTESIAN_POINT ( 'NONE',  ( 3.500000000000001332, 17.50000000000001421, -54.46098080242150985 ) ) ;
#39311=CARTESIAN_POINT ( 'NONE',  ( -3.310556943750001313, 17.50000000000001066, -23.76410580289947561 ) ) ;
#39312=CARTESIAN_POINT ( 'NONE',  ( -1.749999999999999778, 20.53108891324554719, -40.82139747004409713 ) ) ;
#39314=CARTESIAN_POINT ( 'NONE',  ( -1.655278471875002211, 14.63297358603754006, -29.68493913623279568 ) ) ;
#39316=DIRECTION ( 'NONE',  ( -0.000000000000000000, 1.259100132267607459E-16, -1.000000000000000000 ) ) ;
#39317=CARTESIAN_POINT ( 'NONE',  ( -1.750000000000002220, 14.46891108675447946, -60.48806413671076143 ) ) ;
#39319=CARTESIAN_POINT ( 'NONE',  ( 1.750000000000001110, 20.53108891324554719, -35.98806413671076854 ) ) ;
#39322=CARTESIAN_POINT ( 'NONE',  ( -3.310556943750000425, 19.41135094264166838, -82.84743913623279354 ) ) ;
#39327=ORIENTED_EDGE ( 'NONE', *, *, #3457, .T. ) ;
#39329=CARTESIAN_POINT ( 'NONE',  ( 3.310556943750001313, 17.50000000000001776, -90.26410580289947916 ) ) ;
#39330=VERTEX_POINT ( 'NONE', #26684 ) ;
#39334=CYLINDRICAL_SURFACE ( 'NONE', #36896, 3.499999999999999556 ) ;
#39338=CARTESIAN_POINT ( 'NONE',  ( -3.310556943750002645, 15.58864905735837780, -125.6807724695661506 ) ) ;
#39339=ORIENTED_EDGE ( 'NONE', *, *, #41031, .F. ) ;
#39341=CARTESIAN_POINT ( 'NONE',  ( 2.340729813953370519E-16, 21.32270188528330834, -55.10160580289946353 ) ) ;
#39342=CARTESIAN_POINT ( 'NONE',  ( 3.310556943749999981, 15.58864905735837247, -122.4349391362327992 ) ) ;
#39344=ORIENTED_EDGE ( 'NONE', *, *, #35227, .F. ) ;
#39345=CARTESIAN_POINT ( 'NONE',  ( -3.500000000000002220, 15.47927405783633503, -130.5713974700441042 ) ) ;
#39346=CARTESIAN_POINT ( 'NONE',  ( 1.655278471874998436, 14.63297358603754361, -69.51827246956612782 ) ) ;
#39347=CARTESIAN_POINT ( 'NONE',  ( -1.749999999999999778, 20.53108891324555785, -116.1276474690881741 ) ) ;
#39348=CARTESIAN_POINT ( 'NONE',  ( -1.655278471875002211, 14.63297358603754894, -100.5974391362328078 ) ) ;
#39352=CARTESIAN_POINT ( 'NONE',  ( -3.500000000000002220, 15.47927405783632615, -68.87764746908817415 ) ) ;
#39355=CARTESIAN_POINT ( 'NONE',  ( 3.310556943750001313, 19.41135094264165772, -36.18077246956613635 ) ) ;
#39356=CARTESIAN_POINT ( 'NONE',  ( 1.655278471874998436, 14.63297358603754539, -94.51827246956612782 ) ) ;
#39357=CARTESIAN_POINT ( 'NONE',  ( 1.750000000000001110, 20.53108891324555074, -61.98806413671076143 ) ) ;
#39360=CARTESIAN_POINT ( 'NONE',  ( -3.310556943750001313, 17.50000000000002132, -119.8516058028994706 ) ) ;
#39361=EDGE_CURVE ( 'NONE', #13986, #18793, #15724, .T. ) ;
#39369=CARTESIAN_POINT ( 'NONE',  ( -3.310556943750001313, 17.50000000000001776, -95.76410580289946495 ) ) ;
#39373=EDGE_LOOP ( 'NONE', ( #521, #37214, #28463, #15542 ) ) ;
#39374=CARTESIAN_POINT ( 'NONE',  ( 1.749999999999998224, 14.46891108675448834, -136.6276474690881741 ) ) ;
#39375=AXIS2_PLACEMENT_3D ( 'NONE', #11648, #20827, #5065 ) ;
#39378=CARTESIAN_POINT ( 'NONE',  ( -0.9378221735089310451, 14.00000000000001599, -70.75563900116003424 ) ) ;
#39380=CARTESIAN_POINT ( 'NONE',  ( -0.9378221735089221633, 14.00000000000001599, -134.7556390011600342 ) ) ;
#39383=CARTESIAN_POINT ( 'NONE',  ( -1.655278471875002211, 14.63297358603754006, -31.59743913623280775 ) ) ;
#39384=( BOUNDED_CURVE ( )  B_SPLINE_CURVE ( 2, ( #27186, #5042, #14418, #37380, #33568, #36976, #37180, #4212, #8237 ),
 .UNSPECIFIED., .F., .T. ) 
 B_SPLINE_CURVE_WITH_KNOTS ( ( 3, 2, 2, 2, 3 ),
 ( 0.5687499999999999778, 0.5694444444444444198, 0.5708333333333333037, 0.5722222222222221877, 0.5729166666666666297 ),
 .UNSPECIFIED. ) 
 CURVE ( )  GEOMETRIC_REPRESENTATION_ITEM ( )  RATIONAL_B_SPLINE_CURVE ( ( 0.9330127018922194093, 0.9330127018922194093, 1.000000000000000000, 0.8660254037844387076, 1.000000000000000000, 0.8660254037844387076, 1.000000000000000000, 0.9330127018922194093, 0.9330127018922194093 ) ) 
 REPRESENTATION_ITEM ( '' )  );
#39385=ORIENTED_EDGE ( 'NONE', *, *, #24556, .F. ) ;
#39390=AXIS2_PLACEMENT_3D ( 'NONE', #1203, #1618, #4392 ) ;
#39393=CARTESIAN_POINT ( 'NONE',  ( 3.500000000000001332, 17.50000000000001066, -31.15473080337742573 ) ) ;
#39394=CARTESIAN_POINT ( 'NONE',  ( 4.648177544792955347E-16, 21.00000000000001776, -81.21098080242150274 ) ) ;
#39395=DIRECTION ( 'NONE',  ( -0.000000000000000000, 1.259100132267607459E-16, -1.000000000000000000 ) ) ;
#39396=CARTESIAN_POINT ( 'NONE',  ( 3.310556943750001313, 17.50000000000002487, -136.3516058028994564 ) ) ;
#39397=CARTESIAN_POINT ( 'NONE',  ( 3.500000000000001332, 17.50000000000001066, -25.46098080242151340 ) ) ;
#39399=CARTESIAN_POINT ( 'NONE',  ( 4.286263797015737581E-16, 14.00000000000002487, -149.5231586289125687 ) ) ;
#39402=CARTESIAN_POINT ( 'NONE',  ( -7.424026671074350129E-16, 13.45854811567264164, -133.7109808024214885 ) ) ;
#39403=ADVANCED_FACE ( 'NONE', ( #39862 ), #26896, .T. ) ;
#39404=CARTESIAN_POINT ( 'NONE',  ( 3.310556943750001313, 17.50000000000002132, -117.2641058028994792 ) ) ;
#39407=CARTESIAN_POINT ( 'NONE',  ( -0.9378221735089291577, 21.00000000000001776, -82.16632260368298546 ) ) ;
#39408=CARTESIAN_POINT ( 'NONE',  ( -7.424026671074350129E-16, 13.45854811567263631, -85.71098080242151696 ) ) ;
#39409=CYLINDRICAL_SURFACE ( 'NONE', #15821, 3.499999999999999556 ) ;
#39410=CARTESIAN_POINT ( 'NONE',  ( 2.340729813953370519E-16, 21.32270188528330834, -53.01410580289947916 ) ) ;
#39411=CARTESIAN_POINT ( 'NONE',  ( -3.310556943750001313, 17.50000000000002132, -110.8516058028994564 ) ) ;
#39413=CARTESIAN_POINT ( 'NONE',  ( -7.424026671074350129E-16, 13.45854811567263098, -27.40473080337743639 ) ) ;
#39414=DIRECTION ( 'NONE',  ( -0.000000000000000000, 1.259100132267607459E-16, -1.000000000000000000 ) ) ;
#39416=CARTESIAN_POINT ( 'NONE',  ( -3.310556943750000425, 19.41135094264167549, -131.9349391362327992 ) ) ;
#39418=CARTESIAN_POINT ( 'NONE',  ( -3.500000000000001332, 17.50000000000001066, -29.65473080337743994 ) ) ;
#39420=EDGE_CURVE ( 'NONE', #4823, #33117, #41005, .T. ) ;
#39421=CARTESIAN_POINT ( 'NONE',  ( 3.310556943749999981, 15.58864905735836537, -61.43493913623279212 ) ) ;
#39424=CARTESIAN_POINT ( 'NONE',  ( 1.655278471875001101, 20.36702641396248836, -67.09743913623280775 ) ) ;
#39426=CARTESIAN_POINT ( 'NONE',  ( 1.655278471875001101, 20.36702641396249192, -86.18493913623278502 ) ) ;
#39427=EDGE_CURVE ( 'NONE', #13398, #5083, #22271, .T. ) ;
#39429=DIRECTION ( 'NONE',  ( -0.000000000000000000, 1.259100132267607459E-16, -1.000000000000000000 ) ) ;
#39431=CARTESIAN_POINT ( 'NONE',  ( -7.022189441860112050E-16, 13.67729811471671830, -47.51410580289947205 ) ) ;
#39433=CARTESIAN_POINT ( 'NONE',  ( 2.340729813953370519E-16, 21.32270188528331190, -98.01410580289947916 ) ) ;
#39435=( BOUNDED_CURVE ( )  B_SPLINE_CURVE ( 2, ( #25571, #13008, #6620, #38953, #3222, #18968, #38533, #12376, #8974 ),
 .UNSPECIFIED., .F., .T. ) 
 B_SPLINE_CURVE_WITH_KNOTS ( ( 3, 2, 2, 2, 3 ),
 ( 0.2937500000000000111, 0.2944444444444444531, 0.2958333333333333370, 0.2972222222222222210, 0.2979166666666666630 ),
 .UNSPECIFIED. ) 
 CURVE ( )  GEOMETRIC_REPRESENTATION_ITEM ( )  RATIONAL_B_SPLINE_CURVE ( ( 0.9330127018922194093, 0.9330127018922194093, 1.000000000000000000, 0.8660254037844387076, 1.000000000000000000, 0.8660254037844387076, 1.000000000000000000, 0.9330127018922194093, 0.9330127018922194093 ) ) 
 REPRESENTATION_ITEM ( '' )  );
#39436=VECTOR ( 'NONE', #19622, 1000.000000000000000 ) ;
#39440=ORIENTED_EDGE ( 'NONE', *, *, #26123, .T. ) ;
#39442=CARTESIAN_POINT ( 'NONE',  ( -1.655278471874999990, 20.36702641396248836, -56.93077246956614346 ) ) ;
#39443=ORIENTED_EDGE ( 'NONE', *, *, #2536, .F. ) ;
#39444=ORIENTED_EDGE ( 'NONE', *, *, #38378, .F. ) ;
#39446=CARTESIAN_POINT ( 'NONE',  ( 1.750000000000001110, 20.53108891324554719, -31.29431413575484200 ) ) ;
#39449=CARTESIAN_POINT ( 'NONE',  ( 0.9378221735089281585, 14.00000000000001066, -47.36007260463890844 ) ) ;
#39452=CARTESIAN_POINT ( 'NONE',  ( -7.424026671074350129E-16, 13.45854811567263276, -43.71098080242151696 ) ) ;
#39453=CARTESIAN_POINT ( 'NONE',  ( 3.310556943750001313, 19.41135094264165772, -43.18077246956614346 ) ) ;
#39454=CARTESIAN_POINT ( 'NONE',  ( -1.750000000000002220, 14.46891108675447590, -38.79431413575484555 ) ) ;
#39455=CARTESIAN_POINT ( 'NONE',  ( 0.9378221735089281585, 14.00000000000002132, -97.36007260463890134 ) ) ;
#39456=CARTESIAN_POINT ( 'NONE',  ( -3.500000000000002220, 15.47927405783633503, -117.5713974700440900 ) ) ;
#39457=ADVANCED_FACE ( 'NONE', ( #18875 ), #38017, .T. ) ;
#39459=CARTESIAN_POINT ( 'NONE',  ( -1.655278471874999990, 20.36702641396248481, -32.01827246956613493 ) ) ;
#39461=CARTESIAN_POINT ( 'NONE',  ( 3.310556943750001313, 17.50000000000001066, -24.35160580289946708 ) ) ;
#39462=CARTESIAN_POINT ( 'NONE',  ( 3.310556943750001313, 19.41135094264166483, -82.26827246956614204 ) ) ;
#39463=CARTESIAN_POINT ( 'NONE',  ( 3.310556943749999981, 15.58864905735837425, -136.3474391362328220 ) ) ;
#39465=CARTESIAN_POINT ( 'NONE',  ( 3.500000000000001332, 17.50000000000001421, -49.15473080337742573 ) ) ;
#39466=CARTESIAN_POINT ( 'NONE',  ( -1.394453263437886604E-15, 14.00000000000002132, -114.4047308033774186 ) ) ;
#39468=CARTESIAN_POINT ( 'NONE',  ( -7.022189441860112050E-16, 13.67729811471672718, -130.6016058028994280 ) ) ;
#39469=CARTESIAN_POINT ( 'NONE',  ( -1.394453263437886604E-15, 14.00000000000001421, -68.71098080242148853 ) ) ;
#39470=CARTESIAN_POINT ( 'NONE',  ( -1.655278471874999990, 20.36702641396249192, -83.93077246956615056 ) ) ;
#39472=CARTESIAN_POINT ( 'NONE',  ( 0.000000000000000000, 21.00000000000002487, -149.5231586289125687 ) ) ;
#39474=CARTESIAN_POINT ( 'NONE',  ( -3.500000000000001332, 17.50000000000001776, -74.65473080337743284 ) ) ;
#39475=EDGE_CURVE ( 'NONE', #21407, #3780, #31487, .T. ) ;
#39476=CARTESIAN_POINT ( 'NONE',  ( -3.310556943750002201, 15.58864905735836892, -58.76827246956613493 ) ) ;
#39480=CARTESIAN_POINT ( 'NONE',  ( -7.022189441860112050E-16, 13.67729811471672186, -80.60160580289947063 ) ) ;
#39481=CARTESIAN_POINT ( 'NONE',  ( -0.9378221735089310451, 14.00000000000001599, -77.44938900211595012 ) ) ;
#39483=CARTESIAN_POINT ( 'NONE',  ( -1.655278471875002211, 14.63297358603755072, -110.5974391362328078 ) ) ;
#39484=CARTESIAN_POINT ( 'NONE',  ( 3.310556943750001313, 17.50000000000001776, -80.26410580289946495 ) ) ;
#39485=CARTESIAN_POINT ( 'NONE',  ( 3.500000000000001332, 17.50000000000001421, -57.15473080337743284 ) ) ;
#39486=ORIENTED_EDGE ( 'NONE', *, *, #9774, .T. ) ;
#39487=CARTESIAN_POINT ( 'NONE',  ( -1.655278471875002211, 14.63297358603754894, -99.68493913623279923 ) ) ;
#39488=CARTESIAN_POINT ( 'NONE',  ( -3.500000000000002220, 15.47927405783632970, -102.5713974700440900 ) ) ;
#39491=CARTESIAN_POINT ( 'NONE',  ( -3.500000000000000000, 19.52072594216371115, -95.73806413671074722 ) ) ;
#39492=CARTESIAN_POINT ( 'NONE',  ( 3.500000000000001332, 17.50000000000001421, -54.15473080337743284 ) ) ;
#39493=CARTESIAN_POINT ( 'NONE',  ( 4.648177544792955347E-16, 21.00000000000001776, -90.90473080337741862 ) ) ;
#39494=CARTESIAN_POINT ( 'NONE',  ( 3.310556943750001313, 19.41135094264166483, -60.18077246956614346 ) ) ;
#39496=CARTESIAN_POINT ( 'NONE',  ( 1.655278471874998436, 14.63297358603754894, -118.4307724695661364 ) ) ;
#39502=CARTESIAN_POINT ( 'NONE',  ( 3.500000000000001332, 19.52072594216371826, -131.0713974700441042 ) ) ;
#39503=CARTESIAN_POINT ( 'NONE',  ( 4.648177544792955347E-16, 21.00000000000001776, -90.21098080242150274 ) ) ;
#39504=CARTESIAN_POINT ( 'NONE',  ( 3.310556943750001313, 19.41135094264166128, -72.18077246956613635 ) ) ;
#39511=CARTESIAN_POINT ( 'NONE',  ( 1.655278471874998436, 14.63297358603755249, -136.4307724695661364 ) ) ;
#39513=CARTESIAN_POINT ( 'NONE',  ( 3.310556943749999981, 15.58864905735836182, -40.43493913623280633 ) ) ;
#39514=CARTESIAN_POINT ( 'NONE',  ( -3.310556943750000425, 19.41135094264166483, -98.93493913623279923 ) ) ;
#39516=CARTESIAN_POINT ( 'NONE',  ( 3.310556943750001313, 17.50000000000001066, -24.26410580289947561 ) ) ;
#39517=CARTESIAN_POINT ( 'NONE',  ( -3.500000000000000000, 19.52072594216371826, -112.0443141357548456 ) ) ;
#39518=CARTESIAN_POINT ( 'NONE',  ( -1.749999999999999778, 20.53108891324555785, -103.1276474690881741 ) ) ;
#39520=CARTESIAN_POINT ( 'NONE',  ( 4.648177544792955347E-16, 21.00000000000001066, -24.90473080337743284 ) ) ;
#39521=CARTESIAN_POINT ( 'NONE',  ( -7.424026671074350129E-16, 13.45854811567263631, -93.40473080337743284 ) ) ;
#39523=ADVANCED_FACE ( 'NONE', ( #25261 ), #41428, .T. ) ;
#39524=DIRECTION ( 'NONE',  ( -0.000000000000000000, 1.259100132267607459E-16, -1.000000000000000000 ) ) ;
#39527=CARTESIAN_POINT ( 'NONE',  ( -1.394453263437886604E-15, 14.00000000000001421, -68.40473080337741862 ) ) ;
#39528=CARTESIAN_POINT ( 'NONE',  ( 3.500000000000001332, 17.50000000000001421, -55.46098080242150985 ) ) ;
#39529=CARTESIAN_POINT ( 'NONE',  ( 4.648177544792955347E-16, 21.00000000000001776, -89.21098080242148853 ) ) ;
#39530=CYLINDRICAL_SURFACE ( 'NONE', #14950, 3.499999999999999556 ) ;
#39531=ORIENTED_EDGE ( 'NONE', *, *, #30589, .F. ) ;
#39532=CARTESIAN_POINT ( 'NONE',  ( 1.749999999999998224, 14.46891108675447590, -43.32139747004409713 ) ) ;
#39533=CARTESIAN_POINT ( 'NONE',  ( 4.648177544792955347E-16, 21.00000000000002132, -106.2109808024215027 ) ) ;
#39534=CARTESIAN_POINT ( 'NONE',  ( 3.310556943750001313, 17.50000000000001066, -26.35160580289947063 ) ) ;
#39537=CARTESIAN_POINT ( 'NONE',  ( 0.9378221735089300459, 21.00000000000002132, -119.9493890021159643 ) ) ;
#39539=CARTESIAN_POINT ( 'NONE',  ( -7.022189441860112050E-16, 13.67729811471672186, -76.51410580289946495 ) ) ;
#39541=ORIENTED_EDGE ( 'NONE', *, *, #474, .F. ) ;
#39542=FACE_OUTER_BOUND ( 'NONE', #32860, .T. ) ;
#39543=CARTESIAN_POINT ( 'NONE',  ( 4.648177544792955347E-16, 21.00000000000001066, -45.21098080242150985 ) ) ;
#39547=CARTESIAN_POINT ( 'NONE',  ( -3.310556943750000425, 19.41135094264166483, -87.84743913623279354 ) ) ;
#39554=( BOUNDED_CURVE ( )  B_SPLINE_CURVE ( 2, ( #38517, #26184, #9599, #22557, #25762, #3409, #38935, #6398, #16402 ),
 .UNSPECIFIED., .F., .F. ) 
 B_SPLINE_CURVE_WITH_KNOTS ( ( 3, 2, 2, 2, 3 ),
 ( 0.4520833333333333370, 0.4527777777777777790, 0.4541666666666666630, 0.4555555555555555469, 0.4562499999999999889 ),
 .UNSPECIFIED. ) 
 CURVE ( )  GEOMETRIC_REPRESENTATION_ITEM ( )  RATIONAL_B_SPLINE_CURVE ( ( 0.9330127018922194093, 0.9330127018922194093, 1.000000000000000000, 0.8660254037844387076, 1.000000000000000000, 0.8660254037844387076, 1.000000000000000000, 0.9330127018922194093, 0.9330127018922194093 ) ) 
 REPRESENTATION_ITEM ( '' )  );
#39555=CARTESIAN_POINT ( 'NONE',  ( 3.310556943749999981, 15.58864905735837425, -124.3474391362328078 ) ) ;
#39556=EDGE_LOOP ( 'NONE', ( #5288, #20164, #29826, #9699 ) ) ;
#39558=CARTESIAN_POINT ( 'NONE',  ( -3.310556943750001313, 17.50000000000001421, -52.85160580289946353 ) ) ;
#39559=CARTESIAN_POINT ( 'NONE',  ( 3.310556943750001313, 19.41135094264166838, -118.2682724695661278 ) ) ;
#39562=CARTESIAN_POINT ( 'NONE',  ( -3.500000000000001332, 17.50000000000002132, -126.6547308033774186 ) ) ;
#39563=CARTESIAN_POINT ( 'NONE',  ( 2.340729813953370519E-16, 21.32270188528330479, -40.01410580289947916 ) ) ;
#39564=AXIS2_PLACEMENT_3D ( 'NONE', #9833, #35764, #6625 ) ;
#39565=CARTESIAN_POINT ( 'NONE',  ( -1.655278471875002211, 14.63297358603754539, -72.68493913623279923 ) ) ;
#39566=CARTESIAN_POINT ( 'NONE',  ( 3.500000000000001776, 19.52072594216371826, -118.3776474690881741 ) ) ;
#39568=CARTESIAN_POINT ( 'NONE',  ( -1.655278471874999990, 20.36702641396249192, -101.9307724695661364 ) ) ;
#39574=CARTESIAN_POINT ( 'NONE',  ( -7.424026671074350129E-16, 13.45854811567263454, -69.71098080242151696 ) ) ;
#39575=CARTESIAN_POINT ( 'NONE',  ( -1.394453263437886604E-15, 14.00000000000001776, -91.40473080337741862 ) ) ;
#39576=CARTESIAN_POINT ( 'NONE',  ( 1.655278471874998436, 14.63297358603753828, -35.43077246956613635 ) ) ;
#39577=CARTESIAN_POINT ( 'NONE',  ( -1.655278471875002211, 14.63297358603754894, -97.68493913623279923 ) ) ;
#39578=CARTESIAN_POINT ( 'NONE',  ( 3.500000000000000000, 15.47927405783632260, -60.23806413671076143 ) ) ;
#39579=CARTESIAN_POINT ( 'NONE',  ( -7.022189441860112050E-16, 13.67729811471672896, -113.6016058028994564 ) ) ;
#39580=CARTESIAN_POINT ( 'NONE',  ( 3.310556943749999981, 15.58864905735836182, -42.43493913623279212 ) ) ;
#39582=CARTESIAN_POINT ( 'NONE',  ( -3.500000000000002220, 15.47927405783632615, -60.87764746908818125 ) ) ;
#39587=CARTESIAN_POINT ( 'NONE',  ( -1.655278471875002211, 14.63297358603754716, -90.59743913623280775 ) ) ;
#39588=CARTESIAN_POINT ( 'NONE',  ( -3.500000000000000000, 19.52072594216370405, -36.73806413671076854 ) ) ;
#39590=ORIENTED_EDGE ( 'NONE', *, *, #22574, .T. ) ;
#39591=DIRECTION ( 'NONE',  ( -0.000000000000000000, 1.259100132267607459E-16, -1.000000000000000000 ) ) ;
#39593=CARTESIAN_POINT ( 'NONE',  ( -1.750000000000002220, 14.46891108675448478, -105.4880641367107614 ) ) ;
#39598=CARTESIAN_POINT ( 'NONE',  ( 3.310556943749999981, 15.58864905735836182, -27.34743913623280420 ) ) ;
#39605=VECTOR ( 'NONE', #37072, 1000.000000000000000 ) ;
#39607=CARTESIAN_POINT ( 'NONE',  ( 3.500000000000000000, 15.47927405783633503, -135.2380641367107614 ) ) ;
#39609=CARTESIAN_POINT ( 'NONE',  ( -3.310556943750000425, 19.41135094264167549, -142.8474391362327935 ) ) ;
#39610=CARTESIAN_POINT ( 'NONE',  ( 1.749999999999998224, 14.46891108675447946, -68.62764746908817415 ) ) ;
#39611=CARTESIAN_POINT ( 'NONE',  ( -0.9378221735089221633, 14.00000000000001599, -135.7556390011600058 ) ) ;
#39612=CARTESIAN_POINT ( 'NONE',  ( -3.310556943750002645, 15.58864905735837958, -136.7682724695661420 ) ) ;
#39613=CARTESIAN_POINT ( 'NONE',  ( 3.500000000000001332, 17.50000000000001066, -30.46098080242151696 ) ) ;
#39614=EDGE_CURVE ( 'NONE', #25349, #21640, #2291, .T. ) ;
#39616=CARTESIAN_POINT ( 'NONE',  ( -3.500000000000002220, 15.47927405783632437, -44.57139747004409713 ) ) ;
#39617=EDGE_CURVE ( 'NONE', #5189, #33816, #5157, .T. ) ;
#39619=CARTESIAN_POINT ( 'NONE',  ( 3.500000000000001776, 19.52072594216372181, -135.3776474690881741 ) ) ;
#39620=CARTESIAN_POINT ( 'NONE',  ( -3.310556943750002645, 15.58864905735837780, -116.6807724695661506 ) ) ;
#39624=CARTESIAN_POINT ( 'NONE',  ( 3.500000000000001776, 19.52072594216371115, -84.37764746908818836 ) ) ;
#39626=CARTESIAN_POINT ( 'NONE',  ( -1.655278471874999990, 20.36702641396248836, -55.93077246956613635 ) ) ;
#39627=CARTESIAN_POINT ( 'NONE',  ( 2.340729813953370519E-16, 21.32270188528331900, -110.1016058028994706 ) ) ;
#39629=CARTESIAN_POINT ( 'NONE',  ( 3.500000000000001332, 17.50000000000001066, -27.15473080337743639 ) ) ;
#39633=CARTESIAN_POINT ( 'NONE',  ( 3.310556943750001313, 19.41135094264166838, -128.2682724695661136 ) ) ;
#39636=( BOUNDED_CURVE ( )  B_SPLINE_CURVE ( 2, ( #40785, #28433, #11848, #24847, #37804, #5689, #41214, #8659, #18664 ),
 .UNSPECIFIED., .F., .F. ) 
 B_SPLINE_CURVE_WITH_KNOTS ( ( 3, 2, 2, 2, 3 ),
 ( 0.4645833333333333481, 0.4652777777777777901, 0.4666666666666666741, 0.4680555555555555580, 0.4687500000000000000 ),
 .UNSPECIFIED. ) 
 CURVE ( )  GEOMETRIC_REPRESENTATION_ITEM ( )  RATIONAL_B_SPLINE_CURVE ( ( 0.9330127018922194093, 0.9330127018922194093, 1.000000000000000000, 0.8660254037844387076, 1.000000000000000000, 0.8660254037844387076, 1.000000000000000000, 0.9330127018922194093, 0.9330127018922194093 ) ) 
 REPRESENTATION_ITEM ( '' )  );
#39637=CARTESIAN_POINT ( 'NONE',  ( -1.655278471874999990, 20.36702641396248836, -66.01827246956612782 ) ) ;
#39638=EDGE_CURVE ( 'NONE', #37215, #1748, #21182, .T. ) ;
#39640=CARTESIAN_POINT ( 'NONE',  ( -1.655278471874999990, 20.36702641396248836, -61.93077246956614346 ) ) ;
#39641=ORIENTED_EDGE ( 'NONE', *, *, #29097, .T. ) ;
#39642=CARTESIAN_POINT ( 'NONE',  ( -7.022189441860112050E-16, 13.67729811471672363, -85.60160580289947063 ) ) ;
#39644=VECTOR ( 'NONE', #5454, 1000.000000000000000 ) ;
#39649=CARTESIAN_POINT ( 'NONE',  ( 3.310556943750001313, 17.50000000000001066, -43.26410580289947916 ) ) ;
#39651=CARTESIAN_POINT ( 'NONE',  ( 3.310556943750001313, 19.41135094264166483, -101.1807724695661364 ) ) ;
#39652=CARTESIAN_POINT ( 'NONE',  ( 3.500000000000000000, 15.47927405783632082, -53.23806413671076854 ) ) ;
#39653=ORIENTED_EDGE ( 'NONE', *, *, #17754, .F. ) ;
#39657=CARTESIAN_POINT ( 'NONE',  ( 1.655278471874998436, 14.63297358603754006, -53.43077246956613635 ) ) ;
#39659=ORIENTED_EDGE ( 'NONE', *, *, #436, .F. ) ;
#39667=CARTESIAN_POINT ( 'NONE',  ( 3.500000000000001776, 19.52072594216370405, -46.37764746908818125 ) ) ;
#39668=CARTESIAN_POINT ( 'NONE',  ( -7.022189441860112050E-16, 13.67729811471671653, -43.51410580289947916 ) ) ;
#39670=CARTESIAN_POINT ( 'NONE',  ( 4.648177544792955347E-16, 21.00000000000002132, -114.2109808024214885 ) ) ;
#39672=CYLINDRICAL_SURFACE ( 'NONE', #32957, 3.499999999999999556 ) ;
#39673=FACE_OUTER_BOUND ( 'NONE', #36561, .T. ) ;
#39675=VECTOR ( 'NONE', #11449, 1000.000000000000000 ) ;
#39677=CARTESIAN_POINT ( 'NONE',  ( -3.310556943750000425, 19.41135094264165772, -27.93493913623279568 ) ) ;
#39678=CARTESIAN_POINT ( 'NONE',  ( -3.310556943750001313, 17.50000000000001066, -24.85160580289946708 ) ) ;
#39679=CARTESIAN_POINT ( 'NONE',  ( -7.022189441860112050E-16, 13.67729811471672363, -81.60160580289947063 ) ) ;
#39680=CARTESIAN_POINT ( 'NONE',  ( -3.310556943750001313, 17.50000000000002487, -134.7641058028994507 ) ) ;
#39683=CARTESIAN_POINT ( 'NONE',  ( -0.9378221735089310451, 14.00000000000001066, -38.44938900211595723 ) ) ;
#39684=CARTESIAN_POINT ( 'NONE',  ( 4.648177544792955347E-16, 21.00000000000001776, -85.21098080242151696 ) ) ;
#39685=CARTESIAN_POINT ( 'NONE',  ( -1.655278471874999990, 20.36702641396249547, -128.0182724695661136 ) ) ;
#39686=CARTESIAN_POINT ( 'NONE',  ( 1.749999999999998224, 14.46891108675448834, -141.3213974700441042 ) ) ;
#39687=CARTESIAN_POINT ( 'NONE',  ( -7.022189441860112050E-16, 13.67729811471672363, -88.51410580289947916 ) ) ;
#39690=CARTESIAN_POINT ( 'NONE',  ( -7.424026671074350129E-16, 13.45854811567263454, -75.40473080337741862 ) ) ;
#39691=CARTESIAN_POINT ( 'NONE',  ( 1.655278471875001101, 20.36702641396248836, -57.18493913623279212 ) ) ;
#39695=CARTESIAN_POINT ( 'NONE',  ( -7.022189441860112050E-16, 13.67729811471672186, -77.60160580289947063 ) ) ;
#39696=CARTESIAN_POINT ( 'NONE',  ( 3.310556943749999981, 15.58864905735837780, -138.4349391362327708 ) ) ;
#39698=CARTESIAN_POINT ( 'NONE',  ( -1.655278471875002211, 14.63297358603755072, -109.5974391362328078 ) ) ;
#39699=CARTESIAN_POINT ( 'NONE',  ( -3.310556943750002645, 15.58864905735837247, -82.68077246956613635 ) ) ;
#39700=ORIENTED_EDGE ( 'NONE', *, *, #30839, .T. ) ;
#39701=( BOUNDED_CURVE ( )  B_SPLINE_CURVE ( 2, ( #38449, #19091, #8670, #18676, #21857, #28238, #41224, #9095, #35045 ),
 .UNSPECIFIED., .F., .T. ) 
 B_SPLINE_CURVE_WITH_KNOTS ( ( 3, 2, 2, 2, 3 ),
 ( 0.6729166666666667185, 0.6736111111111111605, 0.6750000000000000444, 0.6763888888888889284, 0.6770833333333333703 ),
 .UNSPECIFIED. ) 
 CURVE ( )  GEOMETRIC_REPRESENTATION_ITEM ( )  RATIONAL_B_SPLINE_CURVE ( ( 0.9330127018922194093, 0.9330127018922194093, 1.000000000000000000, 0.8660254037844387076, 1.000000000000000000, 0.8660254037844387076, 1.000000000000000000, 0.9330127018922194093, 0.9330127018922194093 ) ) 
 REPRESENTATION_ITEM ( '' )  );
#39702=CARTESIAN_POINT ( 'NONE',  ( 3.310556943750001313, 19.41135094264166838, -101.2682724695661278 ) ) ;
#39703=CARTESIAN_POINT ( 'NONE',  ( 3.500000000000000000, 15.47927405783632793, -102.2380641367107756 ) ) ;
#39704=VECTOR ( 'NONE', #31011, 1000.000000000000000 ) ;
#39706=CARTESIAN_POINT ( 'NONE',  ( -0.9378221735089291577, 21.00000000000001776, -94.86007260463890134 ) ) ;
#39707=CARTESIAN_POINT ( 'NONE',  ( -1.750000000000002220, 14.46891108675447590, -37.79431413575484555 ) ) ;
#39709=CARTESIAN_POINT ( 'NONE',  ( 0.000000000000000000, 21.00000000000002487, -149.5231586289125687 ) ) ;
#39710=CARTESIAN_POINT ( 'NONE',  ( -3.310556943750001313, 17.50000000000001421, -61.76410580289947205 ) ) ;
#39711=CARTESIAN_POINT ( 'NONE',  ( -1.394453263437886604E-15, 14.00000000000002132, -124.7109808024214885 ) ) ;
#39712=CARTESIAN_POINT ( 'NONE',  ( -3.310556943750000425, 19.41135094264166838, -117.8474391362327935 ) ) ;
#39713=CARTESIAN_POINT ( 'NONE',  ( 0.000000000000000000, 21.00000000000002487, -149.5231586289125687 ) ) ;
#39717=VERTEX_POINT ( 'NONE', #16326 ) ;
#39718=VECTOR ( 'NONE', #26864, 1000.000000000000000 ) ;
#39721=CARTESIAN_POINT ( 'NONE',  ( -3.500000000000001332, 17.50000000000001776, -89.96098080242151696 ) ) ;
#39722=CARTESIAN_POINT ( 'NONE',  ( 1.655278471875001101, 20.36702641396248836, -66.09743913623280775 ) ) ;
#39723=EDGE_LOOP ( 'NONE', ( #4769, #20735, #36997, #10267 ) ) ;
#39725=CYLINDRICAL_SURFACE ( 'NONE', #19460, 3.499999999999999556 ) ;
#39727=EDGE_CURVE ( 'NONE', #35272, #4881, #32677, .T. ) ;
#39728=VERTEX_POINT ( 'NONE', #39261 ) ;
#39729=CARTESIAN_POINT ( 'NONE',  ( -3.310556943750002201, 15.58864905735837780, -135.6807724695661364 ) ) ;
#39733=CARTESIAN_POINT ( 'NONE',  ( -3.310556943750000425, 19.41135094264165772, -43.93493913623279212 ) ) ;
#39734=CARTESIAN_POINT ( 'NONE',  ( -1.394453263437886604E-15, 14.00000000000001066, -41.40473080337741862 ) ) ;
#39735=CARTESIAN_POINT ( 'NONE',  ( 2.340729813953370519E-16, 21.32270188528330479, -40.10160580289946353 ) ) ;
#39736=CARTESIAN_POINT ( 'NONE',  ( 3.310556943750001313, 19.41135094264166483, -96.26827246956612782 ) ) ;
#39740=CARTESIAN_POINT ( 'NONE',  ( -3.310556943750002645, 15.58864905735836182, -24.68077246956613990 ) ) ;
#39741=AXIS2_PLACEMENT_3D ( 'NONE', #12650, #13273, #35613 ) ;
#39742=CARTESIAN_POINT ( 'NONE',  ( 4.648177544792955347E-16, 21.00000000000002132, -121.2109808024215170 ) ) ;
#39743=CARTESIAN_POINT ( 'NONE',  ( 1.750000000000001110, 20.53108891324555785, -103.2943141357548456 ) ) ;
#39744=CARTESIAN_POINT ( 'NONE',  ( -1.749999999999999778, 20.53108891324555074, -73.82139747004410424 ) ) ;
#39746=CARTESIAN_POINT ( 'NONE',  ( -3.500000000000002220, 15.47927405783632793, -92.57139747004409003 ) ) ;
#39750=CARTESIAN_POINT ( 'NONE',  ( -1.394453263437886604E-15, 14.00000000000001066, -50.71098080242150274 ) ) ;
#39751=CARTESIAN_POINT ( 'NONE',  ( -1.750000000000002220, 14.46891108675447768, -53.79431413575484555 ) ) ;
#39752=CARTESIAN_POINT ( 'NONE',  ( -1.750000000000002220, 14.46891108675448123, -73.79431413575483134 ) ) ;
#39753=CARTESIAN_POINT ( 'NONE',  ( 0.000000000000000000, 17.50000000000002487, -149.5231586289125687 ) ) ;
#39754=ORIENTED_EDGE ( 'NONE', *, *, #28524, .T. ) ;
#39755=CARTESIAN_POINT ( 'NONE',  ( -3.500000000000000888, 19.52072594216370405, -45.73806413671076854 ) ) ;
#39757=CARTESIAN_POINT ( 'NONE',  ( 3.310556943750001313, 19.41135094264166128, -28.26827246956613138 ) ) ;
#39758=CARTESIAN_POINT ( 'NONE',  ( 3.500000000000001332, 19.52072594216371115, -75.07139747004410424 ) ) ;
#39759=CARTESIAN_POINT ( 'NONE',  ( 4.648177544792955347E-16, 21.00000000000001421, -64.21098080242150274 ) ) ;
#39761=FACE_OUTER_BOUND ( 'NONE', #14729, .T. ) ;
#39763=CARTESIAN_POINT ( 'NONE',  ( -1.655278471875002211, 14.63297358603754539, -75.59743913623280775 ) ) ;
#39765=ORIENTED_EDGE ( 'NONE', *, *, #3592, .T. ) ;
#39766=CYLINDRICAL_SURFACE ( 'NONE', #41069, 3.499999999999999556 ) ;
#39767=LINE ( 'NONE', #10422, #29837 ) ;
#39769=ORIENTED_EDGE ( 'NONE', *, *, #15576, .F. ) ;
#39771=CARTESIAN_POINT ( 'NONE',  ( -3.310556943750002645, 15.58864905735837247, -82.68077246956613635 ) ) ;
#39772=( BOUNDED_CURVE ( )  B_SPLINE_CURVE ( 2, ( #31208, #15477, #31008, #41213, #41632, #12056, #5688, #18663, #22061 ),
 .UNSPECIFIED., .F., .T. ) 
 B_SPLINE_CURVE_WITH_KNOTS ( ( 3, 2, 2, 2, 3 ),
 ( 0.4937500000000000222, 0.4944444444444444642, 0.4958333333333333481, 0.4972222222222222321, 0.4979166666666666741 ),
 .UNSPECIFIED. ) 
 CURVE ( )  GEOMETRIC_REPRESENTATION_ITEM ( )  RATIONAL_B_SPLINE_CURVE ( ( 0.9330127018922194093, 0.9330127018922194093, 1.000000000000000000, 0.8660254037844387076, 1.000000000000000000, 0.8660254037844387076, 1.000000000000000000, 0.9330127018922194093, 0.9330127018922194093 ) ) 
 REPRESENTATION_ITEM ( '' )  );
#39775=CARTESIAN_POINT ( 'NONE',  ( 0.9378221735089281585, 14.00000000000001066, -50.36007260463890844 ) ) ;
#39779=CARTESIAN_POINT ( 'NONE',  ( -3.500000000000000000, 19.52072594216370760, -59.04431413575484555 ) ) ;
#39780=CARTESIAN_POINT ( 'NONE',  ( -1.655278471875002211, 14.63297358603755249, -125.5974391362328078 ) ) ;
#39783=CARTESIAN_POINT ( 'NONE',  ( -1.655278471875002211, 14.63297358603754361, -56.68493913623279212 ) ) ;
#39785=CARTESIAN_POINT ( 'NONE',  ( 2.340729813953370519E-16, 21.32270188528331900, -113.1016058028994706 ) ) ;
#39788=CARTESIAN_POINT ( 'NONE',  ( 2.474675557024783212E-16, 21.54145188432740099, -127.9047308033774470 ) ) ;
#39789=CARTESIAN_POINT ( 'NONE',  ( 3.310556943750001313, 19.41135094264165772, -42.18077246956614346 ) ) ;
#39790=CARTESIAN_POINT ( 'NONE',  ( 1.655278471874998436, 14.63297358603754184, -64.51827246956614204 ) ) ;
#39791=CARTESIAN_POINT ( 'NONE',  ( 2.474675557024783212E-16, 21.54145188432740099, -115.2109808024215027 ) ) ;
#39792=CARTESIAN_POINT ( 'NONE',  ( 3.310556943749999981, 15.58864905735837070, -102.3474391362328078 ) ) ;
#39793=CARTESIAN_POINT ( 'NONE',  ( 3.500000000000001332, 17.50000000000001421, -60.15473080337743994 ) ) ;
#39795=CARTESIAN_POINT ( 'NONE',  ( -0.9378221735089291577, 21.00000000000001421, -70.86007260463892976 ) ) ;
#39797=CARTESIAN_POINT ( 'NONE',  ( 3.500000000000000000, 15.47927405783632437, -68.54431413575484555 ) ) ;
#39798=CARTESIAN_POINT ( 'NONE',  ( 1.749999999999998224, 14.46891108675448478, -122.6276474690881741 ) ) ;
#39799=CARTESIAN_POINT ( 'NONE',  ( 2.340729813953370519E-16, 21.32270188528330479, -36.01410580289947205 ) ) ;
#39800=CARTESIAN_POINT ( 'NONE',  ( -1.655278471874999990, 20.36702641396249192, -94.01827246956612782 ) ) ;
#39801=CARTESIAN_POINT ( 'NONE',  ( -3.500000000000002220, 15.47927405783632437, -58.57139747004409713 ) ) ;
#39803=VECTOR ( 'NONE', #29564, 1000.000000000000000 ) ;
#39804=CARTESIAN_POINT ( 'NONE',  ( 3.310556943750001313, 17.50000000000002132, -112.3516058028994564 ) ) ;
#39805=CARTESIAN_POINT ( 'NONE',  ( -1.655278471874999990, 20.36702641396248481, -42.01827246956612782 ) ) ;
#39807=CARTESIAN_POINT ( 'NONE',  ( 1.750000000000001110, 20.53108891324555785, -127.2943141357548456 ) ) ;
#39811=CARTESIAN_POINT ( 'NONE',  ( 4.648177544792955347E-16, 21.00000000000002132, -107.2109808024215027 ) ) ;
#39812=CARTESIAN_POINT ( 'NONE',  ( -3.310556943750002201, 15.58864905735837247, -92.68077246956613635 ) ) ;
#39813=CARTESIAN_POINT ( 'NONE',  ( 4.648177544792955347E-16, 21.00000000000001066, -36.90473080337743284 ) ) ;
#39815=ORIENTED_EDGE ( 'NONE', *, *, #35023, .T. ) ;
#39816=CARTESIAN_POINT ( 'NONE',  ( 3.500000000000000000, 15.47927405783632437, -57.54431413575483134 ) ) ;
#39818=DIRECTION ( 'NONE',  ( 0.000000000000000000, 1.000000000000000000, 0.000000000000000000 ) ) ;
#39822=CARTESIAN_POINT ( 'NONE',  ( -3.310556943750000425, 19.41135094264166128, -29.84743913623280775 ) ) ;
#39823=ORIENTED_EDGE ( 'NONE', *, *, #20326, .F. ) ;
#39830=VERTEX_POINT ( 'NONE', #19921 ) ;
#39831=DIRECTION ( 'NONE',  ( -0.000000000000000000, 1.259100132267607459E-16, -1.000000000000000000 ) ) ;
#39833=CARTESIAN_POINT ( 'NONE',  ( 1.750000000000001110, 20.53108891324556140, -136.9880641367107614 ) ) ;
#39835=CARTESIAN_POINT ( 'NONE',  ( -1.394453263437886604E-15, 14.00000000000001421, -78.71098080242148853 ) ) ;
#39837=CARTESIAN_POINT ( 'NONE',  ( -3.310556943750002645, 15.58864905735837780, -131.7682724695661136 ) ) ;
#39838=CARTESIAN_POINT ( 'NONE',  ( -3.500000000000002220, 15.47927405783632082, -28.87764746908817770 ) ) ;
#39840=CARTESIAN_POINT ( 'NONE',  ( -3.500000000000000888, 19.52072594216372181, -142.7380641367107330 ) ) ;
#39842=CARTESIAN_POINT ( 'NONE',  ( 1.749999999999998224, 14.46891108675448656, -132.6276474690881741 ) ) ;
#39843=CARTESIAN_POINT ( 'NONE',  ( 3.310556943749999981, 15.58864905735837247, -116.3474391362327935 ) ) ;
#39846=CARTESIAN_POINT ( 'NONE',  ( 3.500000000000000000, 15.47927405783632615, -83.54431413575483134 ) ) ;
#39847=CARTESIAN_POINT ( 'NONE',  ( -3.500000000000001332, 17.50000000000001776, -92.65473080337743284 ) ) ;
#39848=CARTESIAN_POINT ( 'NONE',  ( -1.655278471874999990, 20.36702641396248836, -53.93077246956613635 ) ) ;
#39849=CARTESIAN_POINT ( 'NONE',  ( -3.310556943750000425, 19.41135094264166838, -110.9349391362327850 ) ) ;
#39851=CARTESIAN_POINT ( 'NONE',  ( 3.500000000000001776, 19.52072594216370405, -28.07139747004409713 ) ) ;
#39853=CARTESIAN_POINT ( 'NONE',  ( -3.310556943750000425, 19.41135094264167549, -130.9349391362327992 ) ) ;
#39856=DIRECTION ( 'NONE',  ( -0.000000000000000000, 1.259100132267607459E-16, -1.000000000000000000 ) ) ;
#39857=CARTESIAN_POINT ( 'NONE',  ( -3.310556943750001313, 17.50000000000001421, -65.85160580289945642 ) ) ;
#39860=CARTESIAN_POINT ( 'NONE',  ( -7.022189441860112050E-16, 13.67729811471672363, -81.60160580289944221 ) ) ;
#39862=FACE_OUTER_BOUND ( 'NONE', #39165, .T. ) ;
#39864=CARTESIAN_POINT ( 'NONE',  ( 2.340729813953370519E-16, 21.32270188528331190, -47.01410580289947205 ) ) ;
#39865=EDGE_CURVE ( 'NONE', #23575, #25161, #19295, .T. ) ;
#39867=CARTESIAN_POINT ( 'NONE',  ( -3.310556943750002645, 15.58864905735837425, -99.68077246956613635 ) ) ;
#39868=CARTESIAN_POINT ( 'NONE',  ( 1.750000000000001110, 20.53108891324554719, -41.98806413671076143 ) ) ;
#39873=CARTESIAN_POINT ( 'NONE',  ( 1.655278471875001101, 20.36702641396248836, -52.09743913623281486 ) ) ;
#39876=FACE_OUTER_BOUND ( 'NONE', #38478, .T. ) ;
#39882=CARTESIAN_POINT ( 'NONE',  ( 1.750000000000001110, 20.53108891324554719, -46.29431413575483845 ) ) ;
#39883=CARTESIAN_POINT ( 'NONE',  ( 0.000000000000000000, 17.50000000000002487, -149.5231586289125687 ) ) ;
#39885=CARTESIAN_POINT ( 'NONE',  ( 1.749999999999998224, 14.46891108675447946, -78.32139747004410424 ) ) ;
#39886=EDGE_CURVE ( 'NONE', #34688, #14781, #35834, .T. ) ;
#39888=CARTESIAN_POINT ( 'NONE',  ( -3.310556943750001313, 17.50000000000001066, -28.85160580289947063 ) ) ;
#39890=CARTESIAN_POINT ( 'NONE',  ( -3.310556943750002645, 15.58864905735837247, -84.76827246956612782 ) ) ;
#39891=CARTESIAN_POINT ( 'NONE',  ( 3.310556943750001313, 19.41135094264167549, -134.1807724695661364 ) ) ;
#39895=CARTESIAN_POINT ( 'NONE',  ( 1.655278471874998436, 14.63297358603755072, -127.5182724695661278 ) ) ;
#39897=CARTESIAN_POINT ( 'NONE',  ( -3.310556943750000425, 19.41135094264166483, -88.84743913623279354 ) ) ;
#39898=CARTESIAN_POINT ( 'NONE',  ( 4.286263797015737581E-16, 14.00000000000002487, -149.5231586289125687 ) ) ;
#39899=CARTESIAN_POINT ( 'NONE',  ( -1.394453263437886604E-15, 14.00000000000001066, -30.40473080337742928 ) ) ;
#39900=CARTESIAN_POINT ( 'NONE',  ( 3.500000000000001332, 17.50000000000001066, -25.15473080337743284 ) ) ;
#39901=CARTESIAN_POINT ( 'NONE',  ( 3.500000000000001776, 19.52072594216370760, -71.07139747004409003 ) ) ;
#39902=CARTESIAN_POINT ( 'NONE',  ( -3.310556943750000425, 19.41135094264166483, -51.93493913623279923 ) ) ;
#39907=CARTESIAN_POINT ( 'NONE',  ( -1.655278471875002211, 14.63297358603754716, -82.68493913623278502 ) ) ;
#39908=CARTESIAN_POINT ( 'NONE',  ( -1.655278471875002211, 14.63297358603755427, -141.6849391362327708 ) ) ;
#39910=CARTESIAN_POINT ( 'NONE',  ( -1.655278471875002211, 14.63297358603754894, -107.5974391362328078 ) ) ;
#39911=CARTESIAN_POINT ( 'NONE',  ( 1.655278471875001101, 20.36702641396249192, -75.09743913623280775 ) ) ;
#39912=ORIENTED_EDGE ( 'NONE', *, *, #27718, .F. ) ;
#39914=CARTESIAN_POINT ( 'NONE',  ( -3.310556943750002201, 15.58864905735837425, -97.76827246956612782 ) ) ;
#39915=CARTESIAN_POINT ( 'NONE',  ( -3.500000000000002220, 15.47927405783632970, -103.5713974700441042 ) ) ;
#39917=CARTESIAN_POINT ( 'NONE',  ( -1.394453263437886604E-15, 14.00000000000001776, -91.71098080242150274 ) ) ;
#39918=CARTESIAN_POINT ( 'NONE',  ( 4.648177544792955347E-16, 21.00000000000002132, -113.2109808024214885 ) ) ;
#39920=CARTESIAN_POINT ( 'NONE',  ( 3.310556943749999981, 15.58864905735836537, -59.34743913623281486 ) ) ;
#39921=CARTESIAN_POINT ( 'NONE',  ( -1.749999999999999778, 20.53108891324555074, -68.82139747004409003 ) ) ;
#39922=CARTESIAN_POINT ( 'NONE',  ( -3.310556943750002645, 15.58864905735837780, -117.6807724695661364 ) ) ;
#39923=CARTESIAN_POINT ( 'NONE',  ( -3.500000000000000000, 19.52072594216371826, -118.0443141357548313 ) ) ;
#39926=ORIENTED_EDGE ( 'NONE', *, *, #4867, .T. ) ;
#39931=CARTESIAN_POINT ( 'NONE',  ( -3.310556943750001313, 17.50000000000001421, -69.76410580289947916 ) ) ;
#39932=VERTEX_POINT ( 'NONE', #34514 ) ;
#39933=VERTEX_POINT ( 'NONE', #33531 ) ;
#39934=CARTESIAN_POINT ( 'NONE',  ( -1.394453263437886604E-15, 14.00000000000001776, -86.71098080242151696 ) ) ;
#39935=FACE_OUTER_BOUND ( 'NONE', #10947, .T. ) ;
#39938=ORIENTED_EDGE ( 'NONE', *, *, #31503, .T. ) ;
#39939=CARTESIAN_POINT ( 'NONE',  ( -3.310556943750001313, 17.50000000000002487, -134.7641058028994507 ) ) ;
#39941=( BOUNDED_CURVE ( )  B_SPLINE_CURVE ( 2, ( #12366, #25350, #38309, #9174, #22149, #33393, #16814, #7667, #33620 ),
 .UNSPECIFIED., .F., .T. ) 
 B_SPLINE_CURVE_WITH_KNOTS ( ( 3, 2, 2, 2, 3 ),
 ( 0.9270833333333333703, 0.9277777777777778123, 0.9291666666666666963, 0.9305555555555555802, 0.9312500000000000222 ),
 .UNSPECIFIED. ) 
 CURVE ( )  GEOMETRIC_REPRESENTATION_ITEM ( )  RATIONAL_B_SPLINE_CURVE ( ( 0.9330127018922194093, 0.9330127018922194093, 1.000000000000000000, 0.8660254037844387076, 1.000000000000000000, 0.8660254037844387076, 1.000000000000000000, 0.9330127018922194093, 0.9330127018922194093 ) ) 
 REPRESENTATION_ITEM ( '' )  );
#39942=CARTESIAN_POINT ( 'NONE',  ( -3.310556943750001313, 17.50000000000001421, -47.85160580289946353 ) ) ;
#39943=CARTESIAN_POINT ( 'NONE',  ( 1.655278471875001101, 20.36702641396248481, -37.18493913623280633 ) ) ;
#39944=CARTESIAN_POINT ( 'NONE',  ( 3.310556943750001313, 17.50000000000001776, -99.35160580289947063 ) ) ;
#39946=CARTESIAN_POINT ( 'NONE',  ( -3.310556943750002645, 15.58864905735837958, -142.7682724695661420 ) ) ;
#39948=CARTESIAN_POINT ( 'NONE',  ( 1.749999999999998224, 14.46891108675448301, -102.6276474690881741 ) ) ;
#39949=LINE ( 'NONE', #26987, #2153 ) ;
#39950=EDGE_CURVE ( 'NONE', #18214, #13874, #40193, .T. ) ;
#39951=LINE ( 'NONE', #20602, #39704 ) ;
#39952=CARTESIAN_POINT ( 'NONE',  ( 3.500000000000000000, 15.47927405783632615, -89.23806413671076143 ) ) ;
#39953=CARTESIAN_POINT ( 'NONE',  ( -3.310556943750001313, 17.50000000000001421, -69.85160580289947063 ) ) ;
#39958=CARTESIAN_POINT ( 'NONE',  ( -3.500000000000000888, 19.52072594216370760, -53.04431413575485266 ) ) ;
#39959=CARTESIAN_POINT ( 'NONE',  ( -1.394453263437886604E-15, 14.00000000000001066, -30.40473080337742928 ) ) ;
#39960=CARTESIAN_POINT ( 'NONE',  ( -3.500000000000002220, 15.47927405783632793, -79.57139747004410424 ) ) ;
#39963=CARTESIAN_POINT ( 'NONE',  ( -1.749999999999999778, 20.53108891324554719, -45.82139747004410424 ) ) ;
#39965=CARTESIAN_POINT ( 'NONE',  ( 3.310556943750001313, 17.50000000000001066, -28.35160580289947063 ) ) ;
#39966=FACE_OUTER_BOUND ( 'NONE', #23193, .T. ) ;
#39967=CARTESIAN_POINT ( 'NONE',  ( -3.500000000000000000, 19.52072594216371115, -90.73806413671074722 ) ) ;
#39969=CARTESIAN_POINT ( 'NONE',  ( -1.394453263437886604E-15, 14.00000000000001776, -106.7109808024215027 ) ) ;
#39971=CARTESIAN_POINT ( 'NONE',  ( 3.310556943750001313, 17.50000000000001776, -77.26410580289946495 ) ) ;
#39972=EDGE_CURVE ( 'NONE', #38091, #14972, #41564, .T. ) ;
#39977=CARTESIAN_POINT ( 'NONE',  ( 3.500000000000000000, 15.47927405783632793, -90.23806413671076143 ) ) ;
#39978=VERTEX_POINT ( 'NONE', #35564 ) ;
#39979=CARTESIAN_POINT ( 'NONE',  ( -1.394453263437886604E-15, 14.00000000000002132, -120.4047308033774328 ) ) ;
#39980=CARTESIAN_POINT ( 'NONE',  ( 1.655278471875001101, 20.36702641396249192, -83.09743913623279354 ) ) ;
#39986=CARTESIAN_POINT ( 'NONE',  ( 3.310556943749999981, 15.58864905735837425, -126.3474391362328078 ) ) ;
#39987=ORIENTED_EDGE ( 'NONE', *, *, #436, .T. ) ;
#39989=CARTESIAN_POINT ( 'NONE',  ( -3.310556943750000425, 19.41135094264166128, -54.93493913623280633 ) ) ;
#39990=CARTESIAN_POINT ( 'NONE',  ( 3.310556943749999981, 15.58864905735837247, -113.4349391362328134 ) ) ;
#39993=CARTESIAN_POINT ( 'NONE',  ( -3.500000000000002220, 15.47927405783633503, -127.5713974700441042 ) ) ;
#39994=CARTESIAN_POINT ( 'NONE',  ( 1.655278471874998436, 14.63297358603753828, -38.43077246956613635 ) ) ;
#39995=CARTESIAN_POINT ( 'NONE',  ( 1.655278471874998436, 14.63297358603754361, -68.51827246956612782 ) ) ;
#39996=CARTESIAN_POINT ( 'NONE',  ( 2.474675557024783212E-16, 21.54145188432740099, -118.2109808024215170 ) ) ;
#39997=EDGE_CURVE ( 'NONE', #24772, #22382, #34224, .T. ) ;
#39998=CARTESIAN_POINT ( 'NONE',  ( 3.310556943750001313, 17.50000000000002132, -104.2641058028994649 ) ) ;
#39999=CARTESIAN_POINT ( 'NONE',  ( 3.500000000000000000, 15.47927405783632437, -60.23806413671076143 ) ) ;
#40001=CARTESIAN_POINT ( 'NONE',  ( 0.000000000000000000, 17.50000000000002487, -149.5231586289125687 ) ) ;
#40003=CARTESIAN_POINT ( 'NONE',  ( -3.500000000000002220, 15.47927405783632615, -71.87764746908817415 ) ) ;
#40004=CARTESIAN_POINT ( 'NONE',  ( 1.750000000000001110, 20.53108891324555429, -100.2943141357548456 ) ) ;
#40005=CARTESIAN_POINT ( 'NONE',  ( 3.310556943749999981, 15.58864905735836182, -30.34743913623280775 ) ) ;
#40006=CARTESIAN_POINT ( 'NONE',  ( 3.310556943750001313, 17.50000000000001776, -91.35160580289947063 ) ) ;
#40007=CARTESIAN_POINT ( 'NONE',  ( -3.500000000000000888, 19.52072594216370760, -57.73806413671076143 ) ) ;
#40008=CARTESIAN_POINT ( 'NONE',  ( 3.310556943749999981, 15.58864905735837247, -110.4349391362328134 ) ) ;
#40009=CARTESIAN_POINT ( 'NONE',  ( -3.310556943750000425, 19.41135094264166128, -44.93493913623280633 ) ) ;
#40011=CARTESIAN_POINT ( 'NONE',  ( 3.500000000000001332, 19.52072594216371826, -127.3776474690881741 ) ) ;
#40016=DIRECTION ( 'NONE',  ( -0.000000000000000000, 1.259100132267607459E-16, -1.000000000000000000 ) ) ;
#40017=CARTESIAN_POINT ( 'NONE',  ( 3.310556943749999981, 15.58864905735836892, -93.34743913623280775 ) ) ;
#40018=( BOUNDED_CURVE ( )  B_SPLINE_CURVE ( 2, ( #25646, #11814, #12234, #12024, #22025, #34999, #22437, #5862, #8627 ),
 .UNSPECIFIED., .F., .F. ) 
 B_SPLINE_CURVE_WITH_KNOTS ( ( 3, 2, 2, 2, 3 ),
 ( 0.2937500000000000111, 0.2944444444444444531, 0.2958333333333333370, 0.2972222222222222210, 0.2979166666666666630 ),
 .UNSPECIFIED. ) 
 CURVE ( )  GEOMETRIC_REPRESENTATION_ITEM ( )  RATIONAL_B_SPLINE_CURVE ( ( 0.9330127018922194093, 0.9330127018922194093, 1.000000000000000000, 0.8660254037844387076, 1.000000000000000000, 0.8660254037844387076, 1.000000000000000000, 0.9330127018922194093, 0.9330127018922194093 ) ) 
 REPRESENTATION_ITEM ( '' )  );
#40019=CARTESIAN_POINT ( 'NONE',  ( -0.9378221735089291577, 21.00000000000001066, -36.86007260463891555 ) ) ;
#40024=LINE ( 'NONE', #4715, #14852 ) ;
#40025=ORIENTED_EDGE ( 'NONE', *, *, #27436, .F. ) ;
#40029=FACE_OUTER_BOUND ( 'NONE', #6340, .T. ) ;
#40038=CARTESIAN_POINT ( 'NONE',  ( -1.655278471874999990, 20.36702641396249902, -140.9307724695661364 ) ) ;
#40039=LINE ( 'NONE', #4523, #5562 ) ;
#40041=DIRECTION ( 'NONE',  ( -0.000000000000000000, 1.259100132267607459E-16, -1.000000000000000000 ) ) ;
#40042=CARTESIAN_POINT ( 'NONE',  ( 3.310556943749999981, 15.58864905735837425, -132.4349391362327992 ) ) ;
#40043=CARTESIAN_POINT ( 'NONE',  ( -3.500000000000002220, 15.47927405783632082, -26.87764746908817770 ) ) ;
#40045=CARTESIAN_POINT ( 'NONE',  ( 3.500000000000001776, 19.52072594216372181, -141.0713974700441042 ) ) ;
#40047=EDGE_CURVE ( 'NONE', #31756, #40297, #2426, .T. ) ;
#40049=CARTESIAN_POINT ( 'NONE',  ( -3.500000000000001332, 17.50000000000002487, -131.9609808024214885 ) ) ;
#40050=CARTESIAN_POINT ( 'NONE',  ( 3.310556943750001313, 19.41135094264166838, -119.1807724695661364 ) ) ;
#40053=CARTESIAN_POINT ( 'NONE',  ( 1.749999999999998224, 14.46891108675448123, -85.62764746908817415 ) ) ;
#40055=CARTESIAN_POINT ( 'NONE',  ( 3.310556943749999981, 15.58864905735836182, -52.34743913623281486 ) ) ;
#40057=CARTESIAN_POINT ( 'NONE',  ( 3.310556943749999981, 15.58864905735837070, -106.4349391362327992 ) ) ;
#40058=CARTESIAN_POINT ( 'NONE',  ( 3.500000000000000000, 15.47927405783632082, -38.54431413575484555 ) ) ;
#40061=CARTESIAN_POINT ( 'NONE',  ( -7.022189441860112050E-16, 13.67729811471672896, -130.6016058028994564 ) ) ;
#40062=ADVANCED_FACE ( 'NONE', ( #32567 ), #16019, .T. ) ;
#40065=CARTESIAN_POINT ( 'NONE',  ( 1.750000000000001110, 20.53108891324555429, -82.98806413671074722 ) ) ;
#40067=CARTESIAN_POINT ( 'NONE',  ( -3.310556943750002645, 15.58864905735836892, -64.76827246956614204 ) ) ;
#40069=( BOUNDED_CURVE ( )  B_SPLINE_CURVE ( 2, ( #4330, #937, #29638, #30061, #10291, #23260, #17098, #13689, #13902 ),
 .UNSPECIFIED., .F., .T. ) 
 B_SPLINE_CURVE_WITH_KNOTS ( ( 3, 2, 2, 2, 3 ),
 ( 0.2229166666666666796, 0.2236111111111111216, 0.2250000000000000056, 0.2263888888888888895, 0.2270833333333333315 ),
 .UNSPECIFIED. ) 
 CURVE ( )  GEOMETRIC_REPRESENTATION_ITEM ( )  RATIONAL_B_SPLINE_CURVE ( ( 0.9330127018922194093, 0.9330127018922207416, 1.000000000000000000, 0.8660254037844387076, 1.000000000000000000, 0.8660254037844387076, 1.000000000000000000, 0.9330127018922194093, 0.9330127018922194093 ) ) 
 REPRESENTATION_ITEM ( '' )  );
#40070=CARTESIAN_POINT ( 'NONE',  ( 1.655278471875001101, 20.36702641396249192, -81.18493913623279923 ) ) ;
#40071=LINE ( 'NONE', #24759, #24360 ) ;
#40075=CARTESIAN_POINT ( 'NONE',  ( 1.655278471875001101, 20.36702641396248481, -44.09743913623280775 ) ) ;
#40076=CARTESIAN_POINT ( 'NONE',  ( -7.022189441860112050E-16, 13.67729811471672541, -100.5141058028994792 ) ) ;
#40079=ORIENTED_EDGE ( 'NONE', *, *, #5842, .T. ) ;
#40083=CARTESIAN_POINT ( 'NONE',  ( 3.310556943750001313, 19.41135094264166128, -51.18077246956613635 ) ) ;
#40084=ORIENTED_EDGE ( 'NONE', *, *, #11157, .F. ) ;
#40086=CARTESIAN_POINT ( 'NONE',  ( -3.500000000000000000, 19.52072594216370405, -43.73806413671076143 ) ) ;
#40093=CARTESIAN_POINT ( 'NONE',  ( 1.749999999999998224, 14.46891108675447590, -45.62764746908818125 ) ) ;
#40095=CARTESIAN_POINT ( 'NONE',  ( -1.750000000000002220, 14.46891108675448656, -110.4880641367107614 ) ) ;
#40097=CARTESIAN_POINT ( 'NONE',  ( -3.310556943750000425, 19.41135094264165772, -29.93493913623279568 ) ) ;
#40098=CARTESIAN_POINT ( 'NONE',  ( 4.648177544792955347E-16, 21.00000000000001421, -53.21098080242150274 ) ) ;
#40099=CARTESIAN_POINT ( 'NONE',  ( -3.310556943750002645, 15.58864905735837247, -83.76827246956612782 ) ) ;
#40100=CARTESIAN_POINT ( 'NONE',  ( 3.310556943750001313, 17.50000000000002487, -132.2641058028994507 ) ) ;
#40105=CARTESIAN_POINT ( 'NONE',  ( 1.655278471874998436, 14.63297358603755072, -128.5182724695661136 ) ) ;
#40106=DIRECTION ( 'NONE',  ( -0.000000000000000000, 1.259100132267607459E-16, -1.000000000000000000 ) ) ;
#40107=CARTESIAN_POINT ( 'NONE',  ( 1.655278471875001101, 20.36702641396249192, -86.09743913623279354 ) ) ;
#40108=FACE_OUTER_BOUND ( 'NONE', #12129, .T. ) ;
#40109=CARTESIAN_POINT ( 'NONE',  ( 1.750000000000001110, 20.53108891324554719, -24.98806413671077209 ) ) ;
#40110=CARTESIAN_POINT ( 'NONE',  ( -3.500000000000002220, 15.47927405783632615, -71.57139747004410424 ) ) ;
#40111=CARTESIAN_POINT ( 'NONE',  ( -7.022189441860112050E-16, 13.67729811471672186, -55.60160580289947063 ) ) ;
#40113=CARTESIAN_POINT ( 'NONE',  ( 4.648177544792955347E-16, 21.00000000000001421, -67.90473080337741862 ) ) ;
#40115=CARTESIAN_POINT ( 'NONE',  ( 3.310556943750001313, 19.41135094264166483, -80.26827246956614204 ) ) ;
#40116=CARTESIAN_POINT ( 'NONE',  ( -3.310556943750000425, 19.41135094264167549, -140.9349391362327708 ) ) ;
#40118=CARTESIAN_POINT ( 'NONE',  ( -3.310556943750000425, 19.41135094264166838, -108.8474391362328220 ) ) ;
#40119=CARTESIAN_POINT ( 'NONE',  ( -1.655278471874999990, 20.36702641396249192, -74.93077246956613635 ) ) ;
#40123=CARTESIAN_POINT ( 'NONE',  ( -7.022189441860112050E-16, 13.67729811471672541, -96.60160580289947063 ) ) ;
#40124=CARTESIAN_POINT ( 'NONE',  ( 1.750000000000001110, 20.53108891324555429, -99.98806413671077564 ) ) ;
#40126=CYLINDRICAL_SURFACE ( 'NONE', #33337, 3.499999999999999556 ) ;
#40129=CARTESIAN_POINT ( 'NONE',  ( -7.022189441860112050E-16, 13.67729811471672186, -63.51410580289947205 ) ) ;
#40130=CARTESIAN_POINT ( 'NONE',  ( -1.394453263437886604E-15, 14.00000000000002132, -115.4047308033774186 ) ) ;
#40131=CARTESIAN_POINT ( 'NONE',  ( 3.310556943750001313, 17.50000000000002132, -115.2641058028994792 ) ) ;
#40132=CARTESIAN_POINT ( 'NONE',  ( 3.500000000000001332, 17.50000000000001066, -36.46098080242150985 ) ) ;
#40135=EDGE_CURVE ( 'NONE', #31790, #24436, #25163, .T. ) ;
#40139=CARTESIAN_POINT ( 'NONE',  ( 3.500000000000000000, 15.47927405783632082, -33.54431413575484555 ) ) ;
#40140=CARTESIAN_POINT ( 'NONE',  ( 3.310556943750001313, 17.50000000000001421, -68.26410580289947916 ) ) ;
#40141=ORIENTED_EDGE ( 'NONE', *, *, #31503, .F. ) ;
#40142=EDGE_LOOP ( 'NONE', ( #16975, #18359, #4631, #1484 ) ) ;
#40143=AXIS2_PLACEMENT_3D ( 'NONE', #17170, #26325, #19720 ) ;
#40144=CARTESIAN_POINT ( 'NONE',  ( 0.000000000000000000, 21.00000000000002487, -149.5231586289125687 ) ) ;
#40145=CARTESIAN_POINT ( 'NONE',  ( 1.750000000000001110, 20.53108891324555429, -83.29431413575483134 ) ) ;
#40149=LINE ( 'NONE', #33565, #39803 ) ;
#40150=CARTESIAN_POINT ( 'NONE',  ( 3.310556943749999981, 15.58864905735837425, -135.3474391362328220 ) ) ;
#40151=CARTESIAN_POINT ( 'NONE',  ( -3.500000000000001332, 17.50000000000002132, -115.9609808024215027 ) ) ;
#40153=CARTESIAN_POINT ( 'NONE',  ( 3.310556943750001313, 19.41135094264165772, -46.26827246956613493 ) ) ;
#40155=CARTESIAN_POINT ( 'NONE',  ( 3.310556943750001313, 19.41135094264165772, -40.26827246956612782 ) ) ;
#40156=CARTESIAN_POINT ( 'NONE',  ( 2.340729813953370519E-16, 21.32270188528331190, -96.10160580289945642 ) ) ;
#40157=EDGE_CURVE ( 'NONE', #41331, #37609, #6631, .T. ) ;
#40160=CARTESIAN_POINT ( 'NONE',  ( 1.655278471874998436, 14.63297358603753651, -25.43077246956613990 ) ) ;
#40162=CARTESIAN_POINT ( 'NONE',  ( -3.500000000000002220, 15.47927405783632970, -97.87764746908815994 ) ) ;
#40163=CARTESIAN_POINT ( 'NONE',  ( 3.500000000000000000, 15.47927405783633503, -132.5443141357548598 ) ) ;
#40165=CARTESIAN_POINT ( 'NONE',  ( -3.500000000000000888, 19.52072594216371115, -87.73806413671074722 ) ) ;
#40166=CARTESIAN_POINT ( 'NONE',  ( 3.310556943750001313, 17.50000000000001421, -67.35160580289947063 ) ) ;
#40170=CARTESIAN_POINT ( 'NONE',  ( -1.749999999999999778, 20.53108891324555074, -49.12764746908818125 ) ) ;
#40172=CARTESIAN_POINT ( 'NONE',  ( 0.000000000000000000, 17.50000000000002487, -149.5231586289125687 ) ) ;
#40173=DIRECTION ( 'NONE',  ( 0.000000000000000000, 1.000000000000000000, 0.000000000000000000 ) ) ;
#40174=ORIENTED_EDGE ( 'NONE', *, *, #21601, .F. ) ;
#40175=CARTESIAN_POINT ( 'NONE',  ( 3.500000000000001332, 17.50000000000002132, -116.1547308033774328 ) ) ;
#40177=CARTESIAN_POINT ( 'NONE',  ( 1.655278471875001101, 20.36702641396248481, -24.18493913623280633 ) ) ;
#40178=FACE_OUTER_BOUND ( 'NONE', #34074, .T. ) ;
#40180=CYLINDRICAL_SURFACE ( 'NONE', #32743, 3.499999999999999556 ) ;
#40182=CARTESIAN_POINT ( 'NONE',  ( -1.655278471874999990, 20.36702641396249192, -75.93077246956613635 ) ) ;
#40184=EDGE_CURVE ( 'NONE', #41707, #30090, #19802, .T. ) ;
#40185=CARTESIAN_POINT ( 'NONE',  ( 0.9378221735089281585, 14.00000000000002309, -127.3600726046389155 ) ) ;
#40186=CARTESIAN_POINT ( 'NONE',  ( 0.9378221735089281585, 14.00000000000001776, -90.36007260463890134 ) ) ;
#40188=ORIENTED_EDGE ( 'NONE', *, *, #17976, .T. ) ;
#40189=CARTESIAN_POINT ( 'NONE',  ( -3.500000000000002220, 15.47927405783633503, -120.5713974700441042 ) ) ;
#40190=CARTESIAN_POINT ( 'NONE',  ( -3.310556943750002645, 15.58864905735837247, -85.68077246956613635 ) ) ;
#40191=ORIENTED_EDGE ( 'NONE', *, *, #32630, .F. ) ;
#40192=ORIENTED_EDGE ( 'NONE', *, *, #6204, .T. ) ;
#40193=( BOUNDED_CURVE ( )  B_SPLINE_CURVE ( 2, ( #4393, #17371, #11196, #10983, #18351, #23970, #21750, #7799, #20774 ),
 .UNSPECIFIED., .F., .T. ) 
 B_SPLINE_CURVE_WITH_KNOTS ( ( 3, 2, 2, 2, 3 ),
 ( 0.7854166666666666519, 0.7861111111111110938, 0.7874999999999999778, 0.7888888888888888618, 0.7895833333333333037 ),
 .UNSPECIFIED. ) 
 CURVE ( )  GEOMETRIC_REPRESENTATION_ITEM ( )  RATIONAL_B_SPLINE_CURVE ( ( 0.9330127018922194093, 0.9330127018922194093, 1.000000000000000000, 0.8660254037844387076, 1.000000000000000000, 0.8660254037844387076, 1.000000000000000000, 0.9330127018922194093, 0.9330127018922194093 ) ) 
 REPRESENTATION_ITEM ( '' )  );
#40197=ORIENTED_EDGE ( 'NONE', *, *, #8171, .T. ) ;
#40199=CARTESIAN_POINT ( 'NONE',  ( -1.655278471874999990, 20.36702641396248836, -55.01827246956612782 ) ) ;
#40200=CARTESIAN_POINT ( 'NONE',  ( 3.310556943750001313, 17.50000000000002132, -112.3516058028994564 ) ) ;
#40202=EDGE_CURVE ( 'NONE', #27445, #28207, #40515, .T. ) ;
#40203=CARTESIAN_POINT ( 'NONE',  ( -3.500000000000000888, 19.52072594216371826, -127.7380641367107756 ) ) ;
#40206=CARTESIAN_POINT ( 'NONE',  ( -1.655278471875002211, 14.63297358603754006, -38.59743913623281486 ) ) ;
#40207=CARTESIAN_POINT ( 'NONE',  ( 1.655278471875001101, 20.36702641396248836, -65.18493913623279923 ) ) ;
#40208=CARTESIAN_POINT ( 'NONE',  ( -7.424026671074350129E-16, 13.45854811567263987, -113.7109808024215170 ) ) ;
#40209=CARTESIAN_POINT ( 'NONE',  ( 2.340729813953370519E-16, 21.32270188528331190, -97.01410580289947916 ) ) ;
#40211=CARTESIAN_POINT ( 'NONE',  ( -1.394453263437886604E-15, 14.00000000000000711, -25.71098080242150630 ) ) ;
#40212=CARTESIAN_POINT ( 'NONE',  ( -3.500000000000002220, 15.47927405783632793, -70.57139747004409003 ) ) ;
#40214=CARTESIAN_POINT ( 'NONE',  ( 1.750000000000001110, 20.53108891324555074, -71.29431413575483134 ) ) ;
#40215=DIRECTION ( 'NONE',  ( 0.000000000000000000, 1.000000000000000000, 0.000000000000000000 ) ) ;
#40216=CARTESIAN_POINT ( 'NONE',  ( -1.655278471874999990, 20.36702641396248481, -33.93077246956615056 ) ) ;
#40217=CARTESIAN_POINT ( 'NONE',  ( -3.310556943750002645, 15.58864905735837247, -90.76827246956614204 ) ) ;
#40218=CARTESIAN_POINT ( 'NONE',  ( 3.500000000000000000, 15.47927405783632260, -58.23806413671075433 ) ) ;
#40219=CARTESIAN_POINT ( 'NONE',  ( 1.750000000000001110, 20.53108891324555429, -92.29431413575484555 ) ) ;
#40220=CARTESIAN_POINT ( 'NONE',  ( -1.655278471874999990, 20.36702641396249547, -113.0182724695661278 ) ) ;
#40221=CARTESIAN_POINT ( 'NONE',  ( -3.310556943750000425, 19.41135094264166128, -35.93493913623279923 ) ) ;
#40224=AXIS2_PLACEMENT_3D ( 'NONE', #38033, #21867, #24865 ) ;
#40229=CARTESIAN_POINT ( 'NONE',  ( -1.655278471875002211, 14.63297358603754716, -94.59743913623280775 ) ) ;
#40236=DIRECTION ( 'NONE',  ( -0.000000000000000000, 1.259100132267607459E-16, -1.000000000000000000 ) ) ;
#40240=EDGE_LOOP ( 'NONE', ( #16191, #14461, #40821, #36409 ) ) ;
#40242=EDGE_CURVE ( 'NONE', #14818, #28459, #32844, .T. ) ;
#40244=EDGE_CURVE ( 'NONE', #37569, #4567, #11130, .T. ) ;
#40248=CYLINDRICAL_SURFACE ( 'NONE', #9041, 3.499999999999999556 ) ;
#40250=CARTESIAN_POINT ( 'NONE',  ( 3.310556943750001313, 17.50000000000002487, -140.2641058028994792 ) ) ;
#40252=CARTESIAN_POINT ( 'NONE',  ( 0.9378221735089300459, 21.00000000000001421, -68.25563900116002003 ) ) ;
#40253=ADVANCED_FACE ( 'NONE', ( #15196 ), #34543, .T. ) ;
#40254=AXIS2_PLACEMENT_3D ( 'NONE', #41533, #28958, #41954 ) ;
#40256=CARTESIAN_POINT ( 'NONE',  ( -1.655278471874999990, 20.36702641396249547, -129.0182724695661136 ) ) ;
#40257=CARTESIAN_POINT ( 'NONE',  ( 2.340729813953370519E-16, 21.32270188528330834, -58.10160580289947063 ) ) ;
#40260=CARTESIAN_POINT ( 'NONE',  ( -1.750000000000002220, 14.46891108675449011, -139.4880641367107614 ) ) ;
#40263=CARTESIAN_POINT ( 'NONE',  ( 2.474675557024783212E-16, 21.54145188432740810, -133.2109808024214885 ) ) ;
#40264=CARTESIAN_POINT ( 'NONE',  ( -3.310556943750001313, 17.50000000000002132, -110.7641058028994649 ) ) ;
#40266=( BOUNDED_CURVE ( )  B_SPLINE_CURVE ( 2, ( #24906, #4912, #8311, #6330, #11700, #34465, #37865, #21082, #34055 ),
 .UNSPECIFIED., .F., .T. ) 
 B_SPLINE_CURVE_WITH_KNOTS ( ( 3, 2, 2, 2, 3 ),
 ( 0.7770833333333333481, 0.7777777777777777901, 0.7791666666666666741, 0.7805555555555555580, 0.7812500000000000000 ),
 .UNSPECIFIED. ) 
 CURVE ( )  GEOMETRIC_REPRESENTATION_ITEM ( )  RATIONAL_B_SPLINE_CURVE ( ( 0.9330127018922194093, 0.9330127018922194093, 1.000000000000000000, 0.8660254037844387076, 1.000000000000000000, 0.8660254037844387076, 1.000000000000000000, 0.9330127018922194093, 0.9330127018922194093 ) ) 
 REPRESENTATION_ITEM ( '' )  );
#40268=CARTESIAN_POINT ( 'NONE',  ( 3.500000000000001332, 17.50000000000001776, -85.46098080242151696 ) ) ;
#40269=CARTESIAN_POINT ( 'NONE',  ( -3.500000000000001332, 17.50000000000001421, -69.65473080337743284 ) ) ;
#40270=CARTESIAN_POINT ( 'NONE',  ( -7.022189441860112050E-16, 13.67729811471671653, -50.51410580289946495 ) ) ;
#40271=CARTESIAN_POINT ( 'NONE',  ( -3.310556943750002645, 15.58864905735837425, -108.7682724695661420 ) ) ;
#40273=CARTESIAN_POINT ( 'NONE',  ( -3.500000000000002220, 15.47927405783632793, -79.87764746908817415 ) ) ;
#40275=CARTESIAN_POINT ( 'NONE',  ( -0.9378221735089310451, 14.00000000000002132, -88.75563900116004845 ) ) ;
#40276=CARTESIAN_POINT ( 'NONE',  ( 2.340729813953370519E-16, 21.32270188528331900, -127.1016058028994706 ) ) ;
#40279=CARTESIAN_POINT ( 'NONE',  ( -1.394453263437886604E-15, 14.00000000000001776, -83.40473080337743284 ) ) ;
#40280=CARTESIAN_POINT ( 'NONE',  ( 0.000000000000000000, 21.00000000000002487, -149.5231586289125687 ) ) ;
#40281=CARTESIAN_POINT ( 'NONE',  ( 1.655278471875001101, 20.36702641396248836, -57.18493913623279212 ) ) ;
#40282=ORIENTED_EDGE ( 'NONE', *, *, #41454, .T. ) ;
#40283=CARTESIAN_POINT ( 'NONE',  ( -3.310556943750000425, 19.41135094264166838, -79.93493913623278502 ) ) ;
#40288=CARTESIAN_POINT ( 'NONE',  ( -1.655278471874999990, 20.36702641396248481, -41.93077246956614346 ) ) ;
#40291=CARTESIAN_POINT ( 'NONE',  ( -3.310556943750002645, 15.58864905735837425, -102.6807724695661364 ) ) ;
#40292=LINE ( 'NONE', #28146, #33884 ) ;
#40296=CARTESIAN_POINT ( 'NONE',  ( 1.655278471875001101, 20.36702641396248836, -55.09743913623281486 ) ) ;
#40297=VERTEX_POINT ( 'NONE', #5405 ) ;
#40300=CARTESIAN_POINT ( 'NONE',  ( -3.500000000000001332, 17.50000000000001066, -43.65473080337743994 ) ) ;
#40301=CARTESIAN_POINT ( 'NONE',  ( 0.9378221735089281585, 14.00000000000002309, -125.3600726046389155 ) ) ;
#40304=ADVANCED_FACE ( 'NONE', ( #28158 ), #37947, .T. ) ;
#40307=CARTESIAN_POINT ( 'NONE',  ( -3.500000000000001332, 17.50000000000001066, -44.96098080242151696 ) ) ;
#40308=CARTESIAN_POINT ( 'NONE',  ( 4.648177544792955347E-16, 21.00000000000001066, -39.90473080337742573 ) ) ;
#40309=CARTESIAN_POINT ( 'NONE',  ( 4.648177544792955347E-16, 21.00000000000002132, -118.9047308033774328 ) ) ;
#40313=CARTESIAN_POINT ( 'NONE',  ( 3.310556943749999981, 15.58864905735836182, -27.43493913623279212 ) ) ;
#40314=CARTESIAN_POINT ( 'NONE',  ( 0.9378221735089281585, 14.00000000000002132, -122.3600726046389155 ) ) ;
#40316=CARTESIAN_POINT ( 'NONE',  ( -3.310556943750002645, 15.58864905735837780, -131.6807724695661364 ) ) ;
#40321=( BOUNDED_CURVE ( )  B_SPLINE_CURVE ( 2, ( #12286, #28867, #2930, #31642, #2508, #8674, #11652, #25270, #21647 ),
 .UNSPECIFIED., .F., .F. ) 
 B_SPLINE_CURVE_WITH_KNOTS ( ( 3, 2, 2, 2, 3 ),
 ( 0.02708333333333333426, 0.02777777777777777624, 0.02916666666666666713, 0.03055555555555555455, 0.03125000000000000000 ),
 .UNSPECIFIED. ) 
 CURVE ( )  GEOMETRIC_REPRESENTATION_ITEM ( )  RATIONAL_B_SPLINE_CURVE ( ( 0.9330127018922194093, 0.9330127018922195203, 1.000000000000000000, 0.8660254037844387076, 1.000000000000000000, 0.8660254037844387076, 1.000000000000000000, 0.9330127018922191873, 0.9330127018922194093 ) ) 
 REPRESENTATION_ITEM ( '' )  );
#40322=CARTESIAN_POINT ( 'NONE',  ( 1.655278471875001101, 20.36702641396249547, -125.1849391362327992 ) ) ;
#40324=CARTESIAN_POINT ( 'NONE',  ( -1.655278471875002211, 14.63297358603754716, -88.59743913623280775 ) ) ;
#40325=CARTESIAN_POINT ( 'NONE',  ( 3.500000000000001332, 19.52072594216370405, -46.07139747004410424 ) ) ;
#40326=VECTOR ( 'NONE', #25531, 1000.000000000000000 ) ;
#40328=CARTESIAN_POINT ( 'NONE',  ( 2.340729813953370519E-16, 21.32270188528332255, -143.1016058028994564 ) ) ;
#40329=CARTESIAN_POINT ( 'NONE',  ( -1.749999999999999778, 20.53108891324555074, -70.82139747004409003 ) ) ;
#40330=CARTESIAN_POINT ( 'NONE',  ( -3.310556943750001313, 17.50000000000001421, -53.85160580289946353 ) ) ;
#40332=CARTESIAN_POINT ( 'NONE',  ( -1.750000000000002220, 14.46891108675448123, -67.48806413671076143 ) ) ;
#40334=CARTESIAN_POINT ( 'NONE',  ( 1.655278471875001101, 20.36702641396249192, -76.18493913623279923 ) ) ;
#40335=CARTESIAN_POINT ( 'NONE',  ( -3.310556943750000425, 19.41135094264167549, -139.9349391362327992 ) ) ;
#40336=ADVANCED_FACE ( 'NONE', ( #21991 ), #1801, .T. ) ;
#40338=CARTESIAN_POINT ( 'NONE',  ( 1.655278471875001101, 20.36702641396249547, -106.0974391362328078 ) ) ;
#40339=CARTESIAN_POINT ( 'NONE',  ( -1.655278471875002211, 14.63297358603754539, -73.59743913623280775 ) ) ;
#40340=ORIENTED_EDGE ( 'NONE', *, *, #1981, .T. ) ;
#40341=CARTESIAN_POINT ( 'NONE',  ( 2.340729813953370519E-16, 21.32270188528331190, -97.10160580289945642 ) ) ;
#40343=CARTESIAN_POINT ( 'NONE',  ( 0.9378221735089300459, 21.00000000000001776, -91.25563900116003424 ) ) ;
#40344=CARTESIAN_POINT ( 'NONE',  ( 4.286263797015737581E-16, 14.00000000000002487, -149.5231586289125687 ) ) ;
#40345=LINE ( 'NONE', #30766, #8957 ) ;
#40346=CARTESIAN_POINT ( 'NONE',  ( -7.022189441860112050E-16, 13.67729811471671830, -53.51410580289947205 ) ) ;
#40347=CARTESIAN_POINT ( 'NONE',  ( -1.655278471874999990, 20.36702641396249547, -118.9307724695661364 ) ) ;
#40348=CARTESIAN_POINT ( 'NONE',  ( 0.000000000000000000, 21.00000000000002487, -149.5231586289125687 ) ) ;
#40349=VERTEX_POINT ( 'NONE', #11571 ) ;
#40351=ORIENTED_EDGE ( 'NONE', *, *, #16123, .T. ) ;
#40354=LINE ( 'NONE', #30356, #1544 ) ;
#40355=CARTESIAN_POINT ( 'NONE',  ( -7.022189441860112050E-16, 13.67729811471672186, -69.51410580289946495 ) ) ;
#40359=CARTESIAN_POINT ( 'NONE',  ( 3.500000000000000000, 15.47927405783633326, -112.2380641367107472 ) ) ;
#40362=VECTOR ( 'NONE', #39429, 1000.000000000000000 ) ;
#40364=EDGE_LOOP ( 'NONE', ( #41605, #15713, #18012, #31609 ) ) ;
#40366=CARTESIAN_POINT ( 'NONE',  ( 3.310556943749999981, 15.58864905735837425, -136.3474391362328220 ) ) ;
#40368=CARTESIAN_POINT ( 'NONE',  ( -3.310556943750002645, 15.58864905735836714, -46.76827246956613493 ) ) ;
#40369=CARTESIAN_POINT ( 'NONE',  ( -3.310556943750001313, 17.50000000000001066, -34.85160580289946353 ) ) ;
#40370=CARTESIAN_POINT ( 'NONE',  ( -1.655278471875002211, 14.63297358603754894, -98.68493913623279923 ) ) ;
#40371=EDGE_CURVE ( 'NONE', #17229, #11372, #27158, .T. ) ;
#40373=CARTESIAN_POINT ( 'NONE',  ( 3.310556943749999981, 15.58864905735837780, -137.4349391362327992 ) ) ;
#40374=FACE_OUTER_BOUND ( 'NONE', #29512, .T. ) ;
#40375=CARTESIAN_POINT ( 'NONE',  ( 1.749999999999998224, 14.46891108675448301, -96.62764746908817415 ) ) ;
#40376=CARTESIAN_POINT ( 'NONE',  ( 4.648177544792955347E-16, 21.00000000000001776, -97.90473080337743284 ) ) ;
#40377=CARTESIAN_POINT ( 'NONE',  ( 1.750000000000001110, 20.53108891324555429, -83.98806413671076143 ) ) ;
#40379=CARTESIAN_POINT ( 'NONE',  ( -3.310556943750000425, 19.41135094264166483, -68.93493913623279923 ) ) ;
#40383=CARTESIAN_POINT ( 'NONE',  ( 7.367361408496833051E-14, 14.00000000000002132, -110.7109808024214743 ) ) ;
#40384=CARTESIAN_POINT ( 'NONE',  ( -3.500000000000002220, 15.47927405783632260, -47.87764746908818125 ) ) ;
#40385=CARTESIAN_POINT ( 'NONE',  ( -7.022189441860112050E-16, 13.67729811471672896, -117.5141058028994792 ) ) ;
#40386=DIRECTION ( 'NONE',  ( -0.000000000000000000, 1.259100132267607459E-16, -1.000000000000000000 ) ) ;
#40387=CYLINDRICAL_SURFACE ( 'NONE', #38974, 3.499999999999999556 ) ;
#40389=CARTESIAN_POINT ( 'NONE',  ( 3.500000000000001776, 19.52072594216371826, -114.0713974700441042 ) ) ;
#40390=CARTESIAN_POINT ( 'NONE',  ( -1.394453263437886604E-15, 14.00000000000001421, -55.40473080337743284 ) ) ;
#40395=CARTESIAN_POINT ( 'NONE',  ( -7.022189441860112050E-16, 13.67729811471672186, -75.51410580289946495 ) ) ;
#40398=EDGE_LOOP ( 'NONE', ( #37259, #41201, #20526, #40744 ) ) ;
#40400=CARTESIAN_POINT ( 'NONE',  ( -7.022189441860112050E-16, 13.67729811471672363, -83.51410580289947916 ) ) ;
#40401=ADVANCED_FACE ( 'NONE', ( #40926 ), #41147, .T. ) ;
#40406=CARTESIAN_POINT ( 'NONE',  ( 3.500000000000000000, 15.47927405783632970, -102.5443141357548456 ) ) ;
#40410=CARTESIAN_POINT ( 'NONE',  ( -3.310556943750001313, 17.50000000000001421, -47.85160580289946353 ) ) ;
#40411=CARTESIAN_POINT ( 'NONE',  ( -1.655278471875002211, 14.63297358603755072, -113.6849391362327992 ) ) ;
#40414=CARTESIAN_POINT ( 'NONE',  ( 3.500000000000001332, 17.50000000000002132, -122.1547308033774328 ) ) ;
#40416=CARTESIAN_POINT ( 'NONE',  ( -3.310556943750001313, 17.50000000000001066, -40.76410580289947916 ) ) ;
#40417=CARTESIAN_POINT ( 'NONE',  ( 1.655278471875001101, 20.36702641396248836, -64.18493913623279923 ) ) ;
#40418=CARTESIAN_POINT ( 'NONE',  ( -3.500000000000002220, 15.47927405783633503, -111.8776474690881741 ) ) ;
#40420=CARTESIAN_POINT ( 'NONE',  ( 3.310556943750001313, 19.41135094264166483, -97.18077246956613635 ) ) ;
#40423=CARTESIAN_POINT ( 'NONE',  ( -3.500000000000000888, 19.52072594216370760, -62.04431413575484555 ) ) ;
#40424=DIRECTION ( 'NONE',  ( 0.000000000000000000, 1.000000000000000000, 0.000000000000000000 ) ) ;
#40425=CARTESIAN_POINT ( 'NONE',  ( -1.655278471875002211, 14.63297358603754006, -32.59743913623280775 ) ) ;
#40426=CARTESIAN_POINT ( 'NONE',  ( -3.310556943750001313, 17.50000000000001776, -92.85160580289947063 ) ) ;
#40428=CARTESIAN_POINT ( 'NONE',  ( -1.749999999999999778, 20.53108891324555074, -52.82139747004409003 ) ) ;
#40429=CARTESIAN_POINT ( 'NONE',  ( 3.310556943750001313, 19.41135094264166838, -112.2682724695661420 ) ) ;
#40430=CARTESIAN_POINT ( 'NONE',  ( -7.022189441860112050E-16, 13.67729811471671653, -35.60160580289946353 ) ) ;
#40437=CARTESIAN_POINT ( 'NONE',  ( -3.310556943750001313, 17.50000000000001776, -92.76410580289947916 ) ) ;
#40441=VERTEX_POINT ( 'NONE', #39189 ) ;
#40442=AXIS2_PLACEMENT_3D ( 'NONE', #11131, #24112, #36650 ) ;
#40446=( BOUNDED_CURVE ( )  B_SPLINE_CURVE ( 2, ( #26293, #39239, #29888, #3729, #19274, #16104, #39454, #29046, #25872 ),
 .UNSPECIFIED., .F., .T. ) 
 B_SPLINE_CURVE_WITH_KNOTS ( ( 3, 2, 2, 2, 3 ),
 ( 0.8687500000000000222, 0.8694444444444444642, 0.8708333333333333481, 0.8722222222222222321, 0.8729166666666666741 ),
 .UNSPECIFIED. ) 
 CURVE ( )  GEOMETRIC_REPRESENTATION_ITEM ( )  RATIONAL_B_SPLINE_CURVE ( ( 0.9330127018922194093, 0.9330127018922194093, 1.000000000000000000, 0.8660254037844387076, 1.000000000000000000, 0.8660254037844387076, 1.000000000000000000, 0.9330127018922194093, 0.9330127018922194093 ) ) 
 REPRESENTATION_ITEM ( '' )  );
#40447=AXIS2_PLACEMENT_3D ( 'NONE', #15797, #18042, #14653 ) ;
#40448=CARTESIAN_POINT ( 'NONE',  ( 0.9378221735089281585, 14.00000000000001066, -46.66632260368298546 ) ) ;
#40454=DIRECTION ( 'NONE',  ( -0.000000000000000000, 1.259100132267607459E-16, -1.000000000000000000 ) ) ;
#40455=EDGE_CURVE ( 'NONE', #13398, #30046, #9506, .T. ) ;
#40463=CARTESIAN_POINT ( 'NONE',  ( -1.394453263437886604E-15, 14.00000000000001421, -71.40473080337743284 ) ) ;
#40464=CARTESIAN_POINT ( 'NONE',  ( -1.655278471875002211, 14.63297358603755427, -139.5974391362327935 ) ) ;
#40465=DIRECTION ( 'NONE',  ( -0.000000000000000000, 1.259100132267607459E-16, -1.000000000000000000 ) ) ;
#40466=CARTESIAN_POINT ( 'NONE',  ( -3.500000000000001332, 17.50000000000001421, -63.65473080337742573 ) ) ;
#40467=CARTESIAN_POINT ( 'NONE',  ( 2.340729813953370519E-16, 21.32270188528332255, -132.1016058028994564 ) ) ;
#40468=CARTESIAN_POINT ( 'NONE',  ( 1.655278471875001101, 20.36702641396248836, -57.18493913623279212 ) ) ;
#40469=ORIENTED_EDGE ( 'NONE', *, *, #2992, .T. ) ;
#40471=CARTESIAN_POINT ( 'NONE',  ( 2.474675557024783212E-16, 21.54145188432740810, -138.9047308033774470 ) ) ;
#40474=CARTESIAN_POINT ( 'NONE',  ( 3.500000000000001332, 17.50000000000002132, -127.4609808024215170 ) ) ;
#40475=CARTESIAN_POINT ( 'NONE',  ( 2.340729813953370519E-16, 21.32270188528331900, -112.0141058028994792 ) ) ;
#40478=CARTESIAN_POINT ( 'NONE',  ( 2.474675557024783212E-16, 21.54145188432739744, -81.21098080242151696 ) ) ;
#40479=EDGE_CURVE ( 'NONE', #5958, #39287, #2846, .T. ) ;
#40481=CARTESIAN_POINT ( 'NONE',  ( -7.022189441860112050E-16, 13.67729811471671653, -48.51410580289947205 ) ) ;
#40482=CARTESIAN_POINT ( 'NONE',  ( 1.655278471875001101, 20.36702641396249547, -108.1849391362327992 ) ) ;
#40483=CARTESIAN_POINT ( 'NONE',  ( -3.500000000000001332, 17.50000000000001776, -82.96098080242150274 ) ) ;
#40485=CARTESIAN_POINT ( 'NONE',  ( -1.394453263437886604E-15, 14.00000000000001776, -105.4047308033774186 ) ) ;
#40487=CARTESIAN_POINT ( 'NONE',  ( -3.310556943750000425, 19.41135094264166838, -125.9349391362327992 ) ) ;
#40490=CARTESIAN_POINT ( 'NONE',  ( -1.394453263437886604E-15, 14.00000000000001776, -86.40473080337743284 ) ) ;
#40491=CARTESIAN_POINT ( 'NONE',  ( -7.022189441860112050E-16, 13.67729811471671830, -60.60160580289945642 ) ) ;
#40493=CARTESIAN_POINT ( 'NONE',  ( 2.340729813953370519E-16, 21.32270188528331190, -83.10160580289947063 ) ) ;
#40495=CARTESIAN_POINT ( 'NONE',  ( 0.9378221735089300459, 21.00000000000001066, -29.94938900211595723 ) ) ;
#40496=CARTESIAN_POINT ( 'NONE',  ( 0.9378221735089300459, 21.00000000000001066, -44.25563900116002003 ) ) ;
#40499=CARTESIAN_POINT ( 'NONE',  ( -3.310556943750001313, 17.50000000000001066, -41.76410580289947916 ) ) ;
#40500=CARTESIAN_POINT ( 'NONE',  ( -3.310556943750000425, 19.41135094264166483, -96.84743913623282197 ) ) ;
#40502=EDGE_CURVE ( 'NONE', #10652, #31790, #20063, .T. ) ;
#40503=AXIS2_PLACEMENT_3D ( 'NONE', #22093, #40817, #18267 ) ;
#40505=ORIENTED_EDGE ( 'NONE', *, *, #37714, .F. ) ;
#40507=CARTESIAN_POINT ( 'NONE',  ( 3.310556943750001313, 17.50000000000001066, -46.26410580289947205 ) ) ;
#40509=ORIENTED_EDGE ( 'NONE', *, *, #5304, .T. ) ;
#40511=CARTESIAN_POINT ( 'NONE',  ( -3.500000000000000000, 19.52072594216371115, -96.04431413575484555 ) ) ;
#40513=CARTESIAN_POINT ( 'NONE',  ( -1.394453263437886604E-15, 14.00000000000001066, -38.71098080242150985 ) ) ;
#40515=LINE ( 'NONE', #24985, #22733 ) ;
#40516=CARTESIAN_POINT ( 'NONE',  ( -3.500000000000001332, 17.50000000000001066, -39.96098080242150985 ) ) ;
#40517=( BOUNDED_CURVE ( )  B_SPLINE_CURVE ( 2, ( #34889, #8730, #40854, #21704, #24495, #11708, #14910, #21501, #18520 ),
 .UNSPECIFIED., .F., .T. ) 
 B_SPLINE_CURVE_WITH_KNOTS ( ( 3, 2, 2, 2, 3 ),
 ( 0.08125000000000000278, 0.08194444444444444475, 0.08333333333333332871, 0.08472222222222222654, 0.08541666666666666852 ),
 .UNSPECIFIED. ) 
 CURVE ( )  GEOMETRIC_REPRESENTATION_ITEM ( )  RATIONAL_B_SPLINE_CURVE ( ( 0.9330127018922194093, 0.9330127018922194093, 1.000000000000000000, 0.8660254037844387076, 1.000000000000000000, 0.8660254037844387076, 1.000000000000000000, 0.9330127018922194093, 0.9330127018922194093 ) ) 
 REPRESENTATION_ITEM ( '' )  );
#40518=CARTESIAN_POINT ( 'NONE',  ( 3.500000000000001332, 17.50000000000001066, -23.46098080242150985 ) ) ;
#40520=CARTESIAN_POINT ( 'NONE',  ( 1.750000000000001110, 20.53108891324555785, -118.9880641367107614 ) ) ;
#40522=CARTESIAN_POINT ( 'NONE',  ( -1.655278471875002211, 14.63297358603754006, -26.68493913623279212 ) ) ;
#40523=CARTESIAN_POINT ( 'NONE',  ( 3.500000000000001332, 19.52072594216371826, -122.0713974700441042 ) ) ;
#40524=CARTESIAN_POINT ( 'NONE',  ( 3.310556943749999981, 15.58864905735837425, -126.3474391362328078 ) ) ;
#40528=CARTESIAN_POINT ( 'NONE',  ( 3.310556943750001313, 19.41135094264166838, -123.2682724695661278 ) ) ;
#40529=CARTESIAN_POINT ( 'NONE',  ( 4.648177544792955347E-16, 21.00000000000002487, -133.9047308033774186 ) ) ;
#40530=CARTESIAN_POINT ( 'NONE',  ( 3.500000000000001332, 17.50000000000001066, -37.15473080337743284 ) ) ;
#40531=CARTESIAN_POINT ( 'NONE',  ( 4.648177544792955347E-16, 21.00000000000001066, -35.21098080242151696 ) ) ;
#40532=CARTESIAN_POINT ( 'NONE',  ( 1.749999999999998224, 14.46891108675448656, -130.6276474690881741 ) ) ;
#40533=ADVANCED_FACE ( 'NONE', ( #11124 ), #20695, .T. ) ;
#40534=CARTESIAN_POINT ( 'NONE',  ( 1.655278471875001101, 20.36702641396249902, -142.1849391362327992 ) ) ;
#40535=CARTESIAN_POINT ( 'NONE',  ( 1.750000000000001110, 20.53108891324555074, -67.98806413671076143 ) ) ;
#40536=CARTESIAN_POINT ( 'NONE',  ( -3.310556943750002201, 15.58864905735836714, -52.76827246956612782 ) ) ;
#40538=CARTESIAN_POINT ( 'NONE',  ( 3.500000000000000000, 15.47927405783633503, -137.5443141357548598 ) ) ;
#40539=CARTESIAN_POINT ( 'NONE',  ( -3.310556943750001313, 17.50000000000001776, -75.85160580289945642 ) ) ;
#40541=CARTESIAN_POINT ( 'NONE',  ( -3.310556943750002201, 15.58864905735837425, -102.6807724695661364 ) ) ;
#40542=CARTESIAN_POINT ( 'NONE',  ( -3.310556943750002645, 15.58864905735837070, -77.68077246956615056 ) ) ;
#40544=CARTESIAN_POINT ( 'NONE',  ( 2.340729813953370519E-16, 21.32270188528331190, -94.10160580289947063 ) ) ;
#40546=CARTESIAN_POINT ( 'NONE',  ( 0.000000000000000000, 17.50000000000002487, -149.5231586289125687 ) ) ;
#40547=CARTESIAN_POINT ( 'NONE',  ( -3.500000000000002220, 15.47927405783632437, -51.87764746908816704 ) ) ;
#40548=EDGE_CURVE ( 'NONE', #39330, #34369, #30259, .T. ) ;
#40550=CARTESIAN_POINT ( 'NONE',  ( 3.310556943749999981, 15.58864905735836537, -55.34743913623281486 ) ) ;
#40551=CARTESIAN_POINT ( 'NONE',  ( -3.500000000000002220, 15.47927405783633503, -124.8776474690881457 ) ) ;
#40552=CARTESIAN_POINT ( 'NONE',  ( 3.310556943750001313, 17.50000000000002132, -110.2641058028994649 ) ) ;
#40553=CARTESIAN_POINT ( 'NONE',  ( 3.500000000000000000, 15.47927405783632793, -84.54431413575483134 ) ) ;
#40555=VERTEX_POINT ( 'NONE', #26439 ) ;
#40557=ORIENTED_EDGE ( 'NONE', *, *, #21246, .T. ) ;
#40559=CARTESIAN_POINT ( 'NONE',  ( -3.310556943750002645, 15.58864905735837070, -68.68077246956613635 ) ) ;
#40560=ORIENTED_EDGE ( 'NONE', *, *, #23653, .T. ) ;
#40561=ORIENTED_EDGE ( 'NONE', *, *, #36218, .F. ) ;
#40562=CARTESIAN_POINT ( 'NONE',  ( -0.9378221735089310451, 14.00000000000002309, -130.7556390011600342 ) ) ;
#40566=ORIENTED_EDGE ( 'NONE', *, *, #33137, .T. ) ;
#40568=CARTESIAN_POINT ( 'NONE',  ( 1.655278471875001101, 20.36702641396249547, -128.0974391362328220 ) ) ;
#40570=( BOUNDED_CURVE ( )  B_SPLINE_CURVE ( 2, ( #32708, #16155, #28889, #29092, #32298, #6351, #42092, #22934, #25926, #25507, #35702, #38677, #6137, #35492, #36108, #12947, #22300, #41885, #2950, #32083, #12734, #38890, #6765, #3571, #22725, #6982, #3164, #16564, #16356, #35899, #9972, #39092, #15940, #25715, #10171, #19739, #9549, #29517, #9767, #19322, #13362, #6566, #22508, #19531, #32502, #3370, #26343, #39291, #13152, #23140, #32918, #3785, #26137, #28675, #12523, #35274, #41668, #38472, #9336, #33778, #23580, #17407, #33979, #37179, #23786, #26977, #16976, #16770, #30367, #3994, #29731, #7834, #27395, #26767, #814, #13567, #10803, #13788, #24211, #1239, #8034, #14207, #39511, #40366, #10602, #14003, #11228, #36539, #33567, #29941, #7403, #39729, #14417, #7615, #27184, #40150, #20377, #17194, #33343, #30576, #11018, #4426, #39939, #4211, #24005, #4633, #17613, #36753, #36975, #20804, #21005, #20592, #30155, #10388, #1446, #33129, #593, #1032, #26553, #23362, #36325, #7196, #20170, #28214, #37378, #18653, #30787, #25243, #40988, #27801, #40772, #24835, #12258, #14631, #31197, #18437, #38207, #21210, #4837, #28005, #11626, #41203, #15258, #34183, #18019, #28421, #25038, #14832, #12045, #21415, #37585, #38001, #8439, #8861, #21835, #8649, #34808, #5253, #5041, #21621, #1853, #5677, #2481, #24621, #34392, #1648, #11422, #18228, #31617, #2057, #15467, #15042, #41410, #27600, #9071, #11837, #37793, #24412, #34597, #22048, #30997, #17815, #40568, #8236, #5459, #31406, #2274, #29047, #19064, #330, #35652, #26294, #32249, #15675, #29460, #12475, #6087, #38837, #22458, #117, #26083, #41836, #15893, #32653, #25873, #32451, #16305, #38629, #35438, #12688, #6712, #3318, #35849, #9713, #3518, #29245, #28837, #38423, #3115, #9494, #35224, #22253, #22674, #16105, #9286, #16509, #2690, #39041, #18855, #13310, #31818, #32034, #39240, #10121, #13099, #25460, #19683, #28632, #35021, #42043, #25667, #6298, #41620, #5884, #22883, #12896, #9926, #19275, #2901, #6515, #19483, #28237, #37606, #5484, #14441, #5274, #18460, #5064, #24854, #8668, #40794, #1872, #31019, #11246, #41222, #14853, #24228, #12066, #8461, #31427, #17632, #27822, #8884, #25059, #11647, #38020, #21855, #24643, #8257, #21440, #37401, #37813, #34414, #21642, #18044, #21026, #18248, #1669, #4654, #27618, #37198, #2080, #31219, #28028, #17834, #34002, #15064, #41007, #11858, #34618, #2294, #15278, #34204, #11443, #8053, #30598, #1466, #4856, #27416, #40385, #21233, #30808, #14655, #40586, #24433, #35463, #9739, #18878, #9519, #22481, #6323, #29271, #12281, #5904, #38653, #22274, #42065, #25897, #12712, #25690, #31844, #41645, #144, #28861, #22072, #9309, #19298, #6541, #16130, #32272, #3140, #32477, #29070, #15698, #38232, #32056, #38447, #35043, #3342, #2712, #12919, #15914, #9093, #16329, #2503, #38863, #18674, #13126, #31637, #28652, #26108, #22699, #2924, #15489, #41861, #12497, #25265, #25483, #39065, #6109, #28443, #9950, #35677, #19507, #34831, #35248, #19089, #5698, #41431, #4397, #13759, #39265, #357, #23113, #16537, #23756, #36294, #29487, #13537, #20139, #26524, #785, #39483, #36081, #10357, #29703, #23333, #17163, #30125, #7168, #36720, #3755, #13336, #20346, #39698, #4180, #6950, #10146, #16947, #29914, #36510, #10571, #23551, #40118, #1208, #26738, #33099, #19925, #22910, #7372, #32891, #3966, #33312, #6739, #35874, #1001, #14175, #13969, #39910, #16740, #26948, #10772, #7585, #3543, #17375, #566, #20560, #30335, #33535, #27152, #19712, #32681, #26318, #17786, #5432, #5012, #40338, #27574, #27771, #24805, #34367, #30970, #40742, #34154, #1621, #21387, #27976, #40957, #17993, #11597, #24592, #11200, #37557, #1827, #27365, #21595, #20778, #15012, #36941, #18409, #7803, #24184, #2244, #31379, #5225, #1414, #37767, #33748, #15224, #14806, #33950, #24382, #4602, #28186, #11809, #8410, #18201, #40541, #37154, #4808, #31169, #34569, #2030, #8622, #17581, #10987, #23975, #11397, #30546, #14388, #8006, #8205, #37351, #20976, #30758, #14600, #21178, #12019, #9845, #3865, #20033, #35775, #23215, #16844, #38968, #22593, #3031, #22804, #3238, #41962, #10246, #26415, #7053, #13430, #16024, #3647, #29166, #12810, #44, #16222, #19403, #13024, #35975, #6636, #37973, #19599, #9631, #18623, #6432, #32998, #26004, #41173, #8833, #32572, #13229, #25011, #28966, #21808, #3439, #35569, #34778, #25794, #38760, #31587, #32375, #5648, #459, #16431, #29378, #247, #26215, #16636, #39162, #6839, #23006, #10043, #19812, #32780, #36182, #29595, #39369, #37050, #4290, #20458, #24083, #33425, #11099, #7909, #33649, #20877, #30234, #33848, #1109, #1522, #40229, #27471, #36620, #7484, #13645, #36406, #26841, #4708, #17271, #17688, #14081, #11297, #10462, #30656, #27054, #40017, #7273, #29806, #1314, #17054, #671, #14500, #40437, #39812, #13861, #26627, #23872, #10676, #37251, #30445, #21083, #10887, #23441, #24280, #20245, #891, #4503, #23658, #17484, #30019, #36837, #7697, #8105, #20671, #27267, #34056, #14288, #4913, #39587, #33206, #4070, #18729, #8725, #15541, #28291, #31689, #34262, #21906, #1729, #12336, #14710, #5123, #9148, #25322, #41275, #8313, #2558, #27669, #38282, #11914, #40849, #11702, #37867, #22124, #40639, #2136, #31483, #5327, #1925, #24700, #25113, #41488, #21697, #28494, #11496, #18514, #35096, #18301, #38076, #34885, #24908, #17894, #21496, #5752, #5540, #12119, #8935, #30867, #28081, #24489, #37458, #34674, #21293, #18102, #15120, #34467, #2350, #8519, #31072, #31273, #37662, #41062, #14904, #27873, #15337, #19768, #16386, #38500, #3397, #22755, #29330, #19146, #35306, #21425, #12975, #19557, #35730, #6592, #23171, #26370, #25955, #16181, #6169, #5957, #32529, #32114, #18931, #38709, #31898, #2766, #199, #39322, #13181, #22961, #2979, #26167, #39119, #9998, #28703, #29549, #41915, #3194, #414, #12763, #35930, #15970, #25744, #28918, #9579, #13390, #38920, #22537, #35521, #6794, #32735, #3601, #9797, #16594, #29120, #6380, #10202, #15751, #41697, #12550, #25536, #9363, #22329, #19352, #32327, #10418, #19987, #36136, #36788, #27427, #7648, #11052, #20200, #10837, #23822, #20623, #16798, #17644, #29971, #33376, #30608, #845, #33602, #14037, #27009, #33160, #13818, #1476, #30188, #23395, #10632, #4461, #7868, #17442, #39971, #30400, #17227, #26800, #1272, #24035, #37006, #1062, #14240, #39539, #4025, #17008, #7228, #36358, #4663, #3818, #40182, #32951, #14451, #29760, #39763, #40395, #11256, #27219, #26582, #20836, #621, #7010, #33808, #23610, #13597, #36571, #7436, #20411, #4243, #31647, #40597, #24239, #5284, #5075, #17846, #37411, #11453, #1681, #24444, #30819, #25069, #37616, #14665, #2512, #27832, #28246, #11870, #18469, #5494, #34629, #8269, #21243, #5709, #2304, #34215, #31436, #40804, #14865, #15292, #11657, #41233, #12075, #28037, #24655, #38031, #8895, #8473, #21866, #34840, #18684, #31029, #1882, #8063, #27627, #18055, #15500, #21450, #28453, #34425, #41441, #4866, #37208, #18258, #31229, #2090, #21037, #37823, #15074, #34014, #41019, #24864, #8679, #21652, #19519, #28875, #2937, #6552, #15926, #35690, #32488, #16142, #3354, #12723, #16341, #25701, #26120, #22711, #9961, #19100, #32067, #38243, #18887, #9320, #29284, #41872, #155, #38665, #35886, #35053, #13137, #9533, #22493, #31855, #12291, #25908, #41654, #25274, #39079, #22921, #22287, #38457, #9104, #6335, #35259, #19724, #12932, #3554, #35475, #5918, #6750, #2723, #25495, #29079, #6122, #42076, #12511, #19309, #32285, #32692, #3152, #9750, #16548, #38875, #29499, #22084, #15708, #28661, #1218, #33323, #40129, #10782, #23343, #3767, #23561, #30135, #1012, #13980, #13548, #27163, #7813, #14186, #16751, #4407, #29925, #576, #797, #3976, #20151, #13770, #36732, #39710, #39276, #7382, #20788, #36520, #36306, #7179, #20357, #33758, #10157, #26749, #26958, #4611, #29714, #369, #4191, #33111, #36092, #26537, #39494, #19937, #10368, #6961, #20569, #17385, #17174, #17590, #16958, #30345, #39920, #7594, #23765, #33546, #10583, #10997, #23984, #36951, #13347, #26329, #23124, #32902, #37775, #5020, #34162, #8418, #21187, #30767, #18001, #37359, #30979, #24814, #8630, #1835, #2252, #40965, #28193, #8213, #14815, #14397, #37161, #27582, #34577, #27781, #2039, #5233, #31178, #5655, #8840, #37564, #40750, #1628, #30556, #15021, #17794, #1424, #21604, #41182, #40550, #14609, #27373, #24599, #11405, #37981, #18210, #27985, #11817, #11209, #12027, #24390, #11606, #25020, #21396, #5441, #34375, #18419, #31387, #21818, #15234, #34788, #40346, #24194, #8012, #20984, #33959, #4817, #35418, #41817, #9266, #29028, #35631, #6494, #12670, #6282, #19257, #32228, #31796, #3296, #26064, #32432, #35002, #22656, #6068, #18836, #2462, #5865, #9906, #39021, #42025, #9052, #16283, #15447, #22862, #25649, #41600, #12457, #38609, #35830, #28402, #2882, #3096, #18631, #2668, #31596, #25440, #12238, #15655, #28613, #38188, #38401, #25224, #19465, #32016, #22028, #22234, #15873, #28818, #35203, #13080, #22440, #29224, #19047, #41388, #16088, #12875, #9474, #25855, #99, #38819, #9695, #13919, #23278, #39431, #953, #10306, #30079, #26898, #10520, #39864, #7116, #23066, #23501, #3707, #10942, #4349, #13489, #26475, #32634, #13289, #16696, #10726, #36244, #23713, #20090, #30292, #29439, #36676, #33054, #3920, #26274, #29867, #23926, #6900, #16901, #7540, #17329, #29652, #32839, #3498, #734, #517, #14131, #7328, #40075, #13708, #308, #1163, #39220, #19873, #36464, #26687, #20514, #33485, #39649, #20298, #27107, #33266, #4130, #6693, #17115, #19662, #16488, #10102, #36034, #37728, #27730, #34531, #5187, #17744, #40288, #34114, #40499, #37112, #11159, #7965, #21557, #2200, #8584, #24142, #40909, #24342, #20934, #37313, #11357, #14560, #8165, #31131, #4972, #33707, #1787, #4764, #14345, #1582, #15180, #14769, #28145, #4559, #21141, #8372, #41133, #33905, #36895, #17953, #30717, #30500, #27534, #30930, #27324, #40699, #1370, #5389, #11556, #24548, #37515, #21352, #34324, #18162, #1988, #14970, #27937, #11767, #11979, #7758, #24764, #18368, #31338, #20731, #17535, #12189, #37933, #16036, #35580, #34948, #8999, #16235, #25598, #41974, #21975, #41762, #12616, #38558, #5604, #6444, #18790, #22188, #19414, #31750, #9425, #25181, #2620, #5817, #22603, #15819, #22391, #38140, #41551, #35368, #38771, #6230, #2832, #19206, #6021, #15604, #32179, #12822, #25805, #18997, #3042, #28975, #9640, #28562, #32386, #3248, #29176, #34738, #53, #8796, #24972, #21765, #41339, #18580, #31545, #2414, #15402, #28354, #12403, #25391, #31962, #38350, #9214, #28764, #35157, #22816, #39383, #20254, #470, #39175, #6852, #33217, #36632, #3877, #13873, #35785, #13656, #26853, #13443, #4083, #17064, #7066, #20470, #16648, #30032, #683, #7284, #39822, #26014, #23226, #17282, #33435, #20046, #7494, #30247, #10259, #29606, #33009, #3660, #13243, #26426, #19823, #36194, #902, #10686, #16856, #23669, #35984, #3450, #10473, #29820, #36418, #26225, #13035, #4300, #26637, #38979, #39598, #10054, #32790, #9859, #6647, #23454, #19611, #32585, #16440, #29390, #259, #23018, #8275, #34429, #41024, #28042, #21250, #38247, #5500, #28460, #14669, #11876, #5922, #22089, #37829, #25280, #18895, #24868, #5289, #21657, #1887, #18262, #8477, #31233, #38037, #8900, #15079, #15505, #12082, #41447, #21456, #2095, #27629, #34219, #40809, #5714, #8684, #18691, #34635, #9110 ),
 .UNSPECIFIED., .F., .T. ) 
 B_SPLINE_CURVE_WITH_KNOTS ( ( 3, 2, 2, 2, 2, 2, 2, 2, 2, 2, 2, 2, 2, 2, 2, 2, 2, 2, 2, 2, 2, 2, 2, 2, 2, 2, 2, 2, 2, 2, 2, 2, 2, 2, 2, 2, 2, 2, 2, 2, 2, 2, 2, 2, 2, 2, 2, 2, 2, 2, 2, 2, 2, 2, 2, 2, 2, 2, 2, 2, 2, 2, 2, 2, 2, 2, 2, 2, 2, 2, 2, 2, 2, 2, 2, 2, 2, 2, 2, 2, 2, 2, 2, 2, 2, 2, 2, 2, 2, 2, 2, 2, 2, 2, 2, 2, 2, 2, 2, 2, 2, 2, 2, 2, 2, 2, 2, 2, 2, 2, 2, 2, 2, 2, 2, 2, 2, 2, 2, 2, 2, 2, 2, 2, 2, 2, 2, 2, 2, 2, 2, 2, 2, 2, 2, 2, 2, 2, 2, 2, 2, 2, 2, 2, 2, 2, 2, 2, 2, 2, 2, 2, 2, 2, 2, 2, 2, 2, 2, 2, 2, 2, 2, 2, 2, 2, 2, 2, 2, 2, 2, 2, 2, 2, 2, 2, 2, 2, 2, 2, 2, 2, 2, 2, 2, 2, 2, 2, 2, 2, 2, 2, 2, 2, 2, 2, 2, 2, 2, 2, 2, 2, 2, 2, 2, 2, 2, 2, 2, 2, 2, 2, 2, 2, 2, 2, 2, 2, 2, 2, 2, 2, 2, 2, 2, 2, 2, 2, 2, 2, 2, 2, 2, 2, 2, 2, 2, 2, 2, 2, 2, 2, 2, 2, 2, 2, 2, 2, 2, 2, 2, 2, 2, 2, 2, 2, 2, 2, 2, 2, 2, 2, 2, 2, 2, 2, 2, 2, 2, 2, 2, 2, 2, 2, 2, 2, 2, 2, 2, 2, 2, 2, 2, 2, 2, 2, 2, 2, 2, 2, 2, 2, 2, 2, 2, 2, 2, 2, 2, 2, 2, 2, 2, 2, 2, 2, 2, 2, 2, 2, 2, 2, 2, 2, 2, 2, 2, 2, 2, 2, 2, 2, 2, 2, 2, 2, 2, 2, 2, 2, 2, 2, 2, 2, 2, 2, 2, 2, 2, 2, 2, 2, 2, 2, 2, 2, 2, 2, 2, 2, 2, 2, 2, 2, 2, 2, 2, 2, 2, 2, 2, 2, 2, 2, 2, 2, 2, 2, 2, 2, 2, 2, 2, 2, 2, 2, 2, 2, 2, 2, 2, 2, 2, 2, 2, 2, 2, 2, 2, 2, 2, 2, 2, 2, 2, 2, 2, 2, 2, 2, 2, 2, 2, 2, 2, 2, 2, 2, 2, 2, 2, 2, 2, 2, 2, 2, 2, 2, 2, 2, 2, 2, 2, 2, 2, 2, 2, 2, 2, 2, 2, 2, 2, 2, 2, 2, 2, 2, 2, 2, 2, 2, 2, 2, 2, 2, 2, 2, 2, 2, 2, 2, 2, 2, 2, 2, 2, 2, 2, 2, 2, 2, 2, 2, 2, 2, 2, 2, 2, 2, 2, 2, 2, 2, 2, 2, 2, 2, 2, 2, 2, 2, 2, 2, 2, 2, 2, 2, 2, 2, 2, 2, 2, 2, 2, 2, 2, 2, 2, 2, 2, 2, 2, 2, 2, 2, 2, 2, 2, 2, 2, 2, 2, 2, 2, 2, 2, 2, 2, 2, 2, 2, 2, 2, 2, 2, 2, 2, 2, 2, 2, 2, 2, 2, 2, 2, 2, 2, 2, 2, 2, 2, 2, 2, 2, 2, 2, 2, 2, 2, 2, 2, 2, 2, 2, 2, 2, 2, 2, 2, 2, 2, 2, 2, 2, 2, 2, 2, 2, 2, 2, 2, 2, 2, 2, 2, 2, 2, 2, 2, 2, 2, 2, 2, 2, 2, 2, 2, 2, 2, 2, 2, 2, 2, 2, 2, 2, 2, 2, 2, 2, 2, 2, 2, 2, 2, 2, 2, 2, 2, 2, 2, 2, 2, 2, 2, 2, 2, 2, 2, 2, 2, 2, 2, 2, 2, 2, 2, 2, 2, 2, 2, 2, 2, 2, 2, 2, 2, 2, 2, 2, 2, 2, 2, 2, 2, 2, 2, 2, 2, 2, 2, 2, 2, 2, 2, 2, 2, 2, 2, 2, 2, 2, 2, 2, 2, 2, 2, 2, 2, 2, 2, 2, 2, 2, 2, 2, 2, 2, 2, 2, 2, 2, 2, 2, 2, 2, 2, 2, 2, 2, 2, 2, 2, 2, 2, 2, 2, 2, 2, 2, 2, 2, 2, 2, 2, 2, 2, 2, 2, 2, 2, 2, 2, 2, 2, 2, 2, 2, 2, 3 ),
 ( 0.000000000000000000, 0.001388888888888888942, 0.002777777777777777884, 0.004166666666666666609, 0.005555555555555555768, 0.006944444444444444059, 0.008333333333333333218, 0.009722222222222222376, 0.01111111111111111154, 0.01250000000000000069, 0.01388888888888888812, 0.01527777777777777728, 0.01666666666666666644, 0.01805555555555555386, 0.01944444444444444475, 0.02083333333333333218, 0.02222222222222222307, 0.02361111111111111049, 0.02500000000000000139, 0.02638888888888888881, 0.02777777777777777624, 0.02916666666666666713, 0.03055555555555555455, 0.03194444444444444198, 0.03333333333333333287, 0.03472222222222222376, 0.03611111111111110772, 0.03749999999999999861, 0.03888888888888888951, 0.04027777777777778040, 0.04166666666666666435, 0.04305555555555555525, 0.04444444444444444614, 0.04583333333333333010, 0.04722222222222222099, 0.04861111111111111188, 0.05000000000000000278, 0.05138888888888888673, 0.05277777777777777762, 0.05416666666666666852, 0.05555555555555555247, 0.05694444444444444337, 0.05833333333333333426, 0.05972222222222222515, 0.06111111111111110911, 0.06250000000000000000, 0.06388888888888888395, 0.06527777777777778179, 0.06666666666666666574, 0.06805555555555554970, 0.06944444444444444753, 0.07083333333333333148, 0.07222222222222221544, 0.07361111111111111327, 0.07499999999999999722, 0.07638888888888889506, 0.07777777777777777901, 0.07916666666666666297, 0.08055555555555556080, 0.08194444444444444475, 0.08333333333333332871, 0.08472222222222222654, 0.08611111111111111049, 0.08749999999999999445, 0.08888888888888889228, 0.09027777777777777624, 0.09166666666666666019, 0.09305555555555555802, 0.09444444444444444198, 0.09583333333333333981, 0.09722222222222222376, 0.09861111111111110772, 0.1000000000000000056, 0.1013888888888888895, 0.1027777777777777735, 0.1041666666666666713, 0.1055555555555555552, 0.1069444444444444392, 0.1083333333333333370, 0.1097222222222222210, 0.1111111111111111049, 0.1125000000000000028, 0.1138888888888888867, 0.1152777777777777846, 0.1166666666666666685, 0.1180555555555555525, 0.1194444444444444503, 0.1208333333333333343, 0.1222222222222222182, 0.1236111111111111160, 0.1250000000000000000, 0.1263888888888888840, 0.1277777777777777679, 0.1291666666666666796, 0.1305555555555555636, 0.1319444444444444475, 0.1333333333333333315, 0.1347222222222222154, 0.1361111111111110994, 0.1375000000000000111, 0.1388888888888888951, 0.1402777777777777790, 0.1416666666666666630, 0.1430555555555555469, 0.1444444444444444309, 0.1458333333333333426, 0.1472222222222222265, 0.1486111111111111105, 0.1499999999999999944, 0.1513888888888888784, 0.1527777777777777901, 0.1541666666666666741, 0.1555555555555555580, 0.1569444444444444420, 0.1583333333333333259, 0.1597222222222222099, 0.1611111111111111216, 0.1625000000000000056, 0.1638888888888888895, 0.1652777777777777735, 0.1666666666666666574, 0.1680555555555555691, 0.1694444444444444531, 0.1708333333333333370, 0.1722222222222222210, 0.1736111111111111049, 0.1749999999999999889, 0.1763888888888889006, 0.1777777777777777846, 0.1791666666666666685, 0.1805555555555555525, 0.1819444444444444364, 0.1833333333333333204, 0.1847222222222222321, 0.1861111111111111160, 0.1875000000000000000, 0.1888888888888888840, 0.1902777777777777679, 0.1916666666666666796, 0.1930555555555555636, 0.1944444444444444475, 0.1958333333333333315, 0.1972222222222222154, 0.1986111111111110994, 0.2000000000000000111, 0.2013888888888888951, 0.2027777777777777790, 0.2041666666666666630, 0.2055555555555555469, 0.2069444444444444309, 0.2083333333333333426, 0.2097222222222222265, 0.2111111111111111105, 0.2124999999999999944, 0.2138888888888888784, 0.2152777777777777901, 0.2166666666666666741, 0.2180555555555555580, 0.2194444444444444420, 0.2208333333333333259, 0.2222222222222222099, 0.2236111111111111216, 0.2250000000000000056, 0.2263888888888888895, 0.2277777777777777735, 0.2291666666666666574, 0.2305555555555555691, 0.2319444444444444531, 0.2333333333333333370, 0.2347222222222222210, 0.2361111111111111049, 0.2374999999999999889, 0.2388888888888889006, 0.2402777777777777846, 0.2416666666666666685, 0.2430555555555555525, 0.2444444444444444364, 0.2458333333333333204, 0.2472222222222222321, 0.2486111111111111160, 0.2500000000000000000, 0.2513888888888888840, 0.2527777777777777679, 0.2541666666666666519, 0.2555555555555555358, 0.2569444444444444198, 0.2583333333333333592, 0.2597222222222222432, 0.2611111111111111271, 0.2625000000000000111, 0.2638888888888888951, 0.2652777777777777790, 0.2666666666666666630, 0.2680555555555555469, 0.2694444444444444309, 0.2708333333333333148, 0.2722222222222221988, 0.2736111111111111382, 0.2750000000000000222, 0.2763888888888889062, 0.2777777777777777901, 0.2791666666666666741, 0.2805555555555555580, 0.2819444444444444420, 0.2833333333333333259, 0.2847222222222222099, 0.2861111111111110938, 0.2874999999999999778, 0.2888888888888888618, 0.2902777777777778012, 0.2916666666666666852, 0.2930555555555555691, 0.2944444444444444531, 0.2958333333333333370, 0.2972222222222222210, 0.2986111111111111049, 0.2999999999999999889, 0.3013888888888888729, 0.3027777777777777568, 0.3041666666666666408, 0.3055555555555555802, 0.3069444444444444642, 0.3083333333333333481, 0.3097222222222222321, 0.3111111111111111160, 0.3125000000000000000, 0.3138888888888888840, 0.3152777777777777679, 0.3166666666666666519, 0.3180555555555555358, 0.3194444444444444198, 0.3208333333333333592, 0.3222222222222222432, 0.3236111111111111271, 0.3250000000000000111, 0.3263888888888888951, 0.3277777777777777790, 0.3291666666666666630, 0.3305555555555555469, 0.3319444444444444309, 0.3333333333333333148, 0.3347222222222221988, 0.3361111111111111382, 0.3375000000000000222, 0.3388888888888889062, 0.3402777777777777901, 0.3416666666666666741, 0.3430555555555555580, 0.3444444444444444420, 0.3458333333333333259, 0.3472222222222222099, 0.3486111111111110938, 0.3499999999999999778, 0.3513888888888888618, 0.3527777777777778012, 0.3541666666666666852, 0.3555555555555555691, 0.3569444444444444531, 0.3583333333333333370, 0.3597222222222222210, 0.3611111111111111049, 0.3624999999999999889, 0.3638888888888888729, 0.3652777777777777568, 0.3666666666666666408, 0.3680555555555555802, 0.3694444444444444642, 0.3708333333333333481, 0.3722222222222222321, 0.3736111111111111160, 0.3750000000000000000, 0.3763888888888888840, 0.3777777777777777679, 0.3791666666666666519, 0.3805555555555555358, 0.3819444444444444198, 0.3833333333333333592, 0.3847222222222222432, 0.3861111111111111271, 0.3875000000000000111, 0.3888888888888888951, 0.3902777777777777790, 0.3916666666666666630, 0.3930555555555555469, 0.3944444444444444309, 0.3958333333333333148, 0.3972222222222221988, 0.3986111111111111382, 0.4000000000000000222, 0.4013888888888889062, 0.4027777777777777901, 0.4041666666666666741, 0.4055555555555555580, 0.4069444444444444420, 0.4083333333333333259, 0.4097222222222222099, 0.4111111111111110938, 0.4124999999999999778, 0.4138888888888888618, 0.4152777777777778012, 0.4166666666666666852, 0.4180555555555555691, 0.4194444444444444531, 0.4208333333333333370, 0.4222222222222222210, 0.4236111111111111049, 0.4249999999999999889, 0.4263888888888888729, 0.4277777777777777568, 0.4291666666666666408, 0.4305555555555555802, 0.4319444444444444642, 0.4333333333333333481, 0.4347222222222222321, 0.4361111111111111160, 0.4375000000000000000, 0.4388888888888888840, 0.4402777777777777679, 0.4416666666666666519, 0.4430555555555555358, 0.4444444444444444198, 0.4458333333333333592, 0.4472222222222222432, 0.4486111111111111271, 0.4500000000000000111, 0.4513888888888888951, 0.4527777777777777790, 0.4541666666666666630, 0.4555555555555555469, 0.4569444444444444309, 0.4583333333333333148, 0.4597222222222221988, 0.4611111111111111382, 0.4625000000000000222, 0.4638888888888889062, 0.4652777777777777901, 0.4666666666666666741, 0.4680555555555555580, 0.4694444444444444420, 0.4708333333333333259, 0.4722222222222222099, 0.4736111111111110938, 0.4749999999999999778, 0.4763888888888888618, 0.4777777777777778012, 0.4791666666666666852, 0.4805555555555555691, 0.4819444444444444531, 0.4833333333333333370, 0.4847222222222222210, 0.4861111111111111049, 0.4874999999999999889, 0.4888888888888888729, 0.4902777777777777568, 0.4916666666666666408, 0.4930555555555555802, 0.4944444444444444642, 0.4958333333333333481, 0.4972222222222222321, 0.4986111111111111160, 0.5000000000000000000, 0.5013888888888888840, 0.5027777777777777679, 0.5041666666666666519, 0.5055555555555555358, 0.5069444444444444198, 0.5083333333333333037, 0.5097222222222221877, 0.5111111111111110716, 0.5124999999999999556, 0.5138888888888888395, 0.5152777777777777235, 0.5166666666666667185, 0.5180555555555556024, 0.5194444444444444864, 0.5208333333333333703, 0.5222222222222222543, 0.5236111111111111382, 0.5250000000000000222, 0.5263888888888889062, 0.5277777777777777901, 0.5291666666666666741, 0.5305555555555555580, 0.5319444444444444420, 0.5333333333333333259, 0.5347222222222222099, 0.5361111111111110938, 0.5374999999999999778, 0.5388888888888888618, 0.5402777777777777457, 0.5416666666666666297, 0.5430555555555555136, 0.5444444444444443976, 0.5458333333333332815, 0.5472222222222222765, 0.5486111111111111605, 0.5500000000000000444, 0.5513888888888889284, 0.5527777777777778123, 0.5541666666666666963, 0.5555555555555555802, 0.5569444444444444642, 0.5583333333333333481, 0.5597222222222222321, 0.5611111111111111160, 0.5625000000000000000, 0.5638888888888888840, 0.5652777777777777679, 0.5666666666666666519, 0.5680555555555555358, 0.5694444444444444198, 0.5708333333333333037, 0.5722222222222221877, 0.5736111111111110716, 0.5749999999999999556, 0.5763888888888888395, 0.5777777777777777235, 0.5791666666666667185, 0.5805555555555556024, 0.5819444444444444864, 0.5833333333333333703, 0.5847222222222222543, 0.5861111111111111382, 0.5875000000000000222, 0.5888888888888889062, 0.5902777777777777901, 0.5916666666666666741, 0.5930555555555555580, 0.5944444444444444420, 0.5958333333333333259, 0.5972222222222222099, 0.5986111111111110938, 0.5999999999999999778, 0.6013888888888888618, 0.6027777777777777457, 0.6041666666666666297, 0.6055555555555555136, 0.6069444444444443976, 0.6083333333333332815, 0.6097222222222222765, 0.6111111111111111605, 0.6125000000000000444, 0.6138888888888889284, 0.6152777777777778123, 0.6166666666666666963, 0.6180555555555555802, 0.6194444444444444642, 0.6208333333333333481, 0.6222222222222222321, 0.6236111111111111160, 0.6250000000000000000, 0.6263888888888888840, 0.6277777777777777679, 0.6291666666666666519, 0.6305555555555555358, 0.6319444444444444198, 0.6333333333333333037, 0.6347222222222221877, 0.6361111111111110716, 0.6374999999999999556, 0.6388888888888888395, 0.6402777777777777235, 0.6416666666666667185, 0.6430555555555556024, 0.6444444444444444864, 0.6458333333333333703, 0.6472222222222222543, 0.6486111111111111382, 0.6500000000000000222, 0.6513888888888889062, 0.6527777777777777901, 0.6541666666666666741, 0.6555555555555555580, 0.6569444444444444420, 0.6583333333333333259, 0.6597222222222222099, 0.6611111111111110938, 0.6624999999999999778, 0.6638888888888888618, 0.6652777777777777457, 0.6666666666666666297, 0.6680555555555555136, 0.6694444444444443976, 0.6708333333333332815, 0.6722222222222222765, 0.6736111111111111605, 0.6750000000000000444, 0.6763888888888889284, 0.6777777777777778123, 0.6791666666666666963, 0.6805555555555555802, 0.6819444444444444642, 0.6833333333333333481, 0.6847222222222222321, 0.6861111111111111160, 0.6875000000000000000, 0.6888888888888888840, 0.6902777777777777679, 0.6916666666666666519, 0.6930555555555555358, 0.6944444444444444198, 0.6958333333333333037, 0.6972222222222221877, 0.6986111111111110716, 0.6999999999999999556, 0.7013888888888888395, 0.7027777777777777235, 0.7041666666666667185, 0.7055555555555556024, 0.7069444444444444864, 0.7083333333333333703, 0.7097222222222222543, 0.7111111111111111382, 0.7125000000000000222, 0.7138888888888889062, 0.7152777777777777901, 0.7166666666666666741, 0.7180555555555555580, 0.7194444444444444420, 0.7208333333333333259, 0.7222222222222222099, 0.7236111111111110938, 0.7249999999999999778, 0.7263888888888888618, 0.7277777777777777457, 0.7291666666666666297, 0.7305555555555555136, 0.7319444444444443976, 0.7333333333333332815, 0.7347222222222222765, 0.7361111111111111605, 0.7375000000000000444, 0.7388888888888889284, 0.7402777777777778123, 0.7416666666666666963, 0.7430555555555555802, 0.7444444444444444642, 0.7458333333333333481, 0.7472222222222222321, 0.7486111111111111160, 0.7500000000000000000, 0.7513888888888888840, 0.7527777777777777679, 0.7541666666666666519, 0.7555555555555555358, 0.7569444444444444198, 0.7583333333333333037, 0.7597222222222221877, 0.7611111111111110716, 0.7624999999999999556, 0.7638888888888888395, 0.7652777777777777235, 0.7666666666666667185, 0.7680555555555556024, 0.7694444444444444864, 0.7708333333333333703, 0.7722222222222222543, 0.7736111111111111382, 0.7750000000000000222, 0.7763888888888889062, 0.7777777777777777901, 0.7791666666666666741, 0.7805555555555555580, 0.7819444444444444420, 0.7833333333333333259, 0.7847222222222222099, 0.7861111111111110938, 0.7874999999999999778, 0.7888888888888888618, 0.7902777777777777457, 0.7916666666666666297, 0.7930555555555555136, 0.7944444444444443976, 0.7958333333333332815, 0.7972222222222222765, 0.7986111111111111605, 0.8000000000000000444, 0.8013888888888889284, 0.8027777777777778123, 0.8041666666666666963, 0.8055555555555555802, 0.8069444444444444642, 0.8083333333333333481, 0.8097222222222222321, 0.8111111111111111160, 0.8125000000000000000, 0.8138888888888888840, 0.8152777777777777679, 0.8166666666666666519, 0.8180555555555555358, 0.8194444444444444198, 0.8208333333333333037, 0.8222222222222221877, 0.8236111111111110716, 0.8249999999999999556, 0.8263888888888888395, 0.8277777777777777235, 0.8291666666666667185, 0.8305555555555556024, 0.8319444444444444864, 0.8333333333333333703, 0.8347222222222222543, 0.8361111111111111382, 0.8375000000000000222, 0.8388888888888889062, 0.8402777777777777901, 0.8416666666666666741, 0.8430555555555555580, 0.8444444444444444420, 0.8458333333333333259, 0.8472222222222222099, 0.8486111111111110938, 0.8499999999999999778, 0.8513888888888888618, 0.8527777777777777457, 0.8541666666666666297, 0.8555555555555555136, 0.8569444444444443976, 0.8583333333333332815, 0.8597222222222222765, 0.8611111111111111605, 0.8625000000000000444, 0.8638888888888889284, 0.8652777777777778123, 0.8666666666666666963, 0.8680555555555555802, 0.8694444444444444642, 0.8708333333333333481, 0.8722222222222222321, 0.8736111111111111160, 0.8750000000000000000, 0.8763888888888888840, 0.8777777777777777679, 0.8791666666666666519, 0.8805555555555555358, 0.8819444444444444198, 0.8833333333333333037, 0.8847222222222221877, 0.8861111111111110716, 0.8874999999999999556, 0.8888888888888888395, 0.8902777777777777235, 0.8916666666666667185, 0.8930555555555556024, 0.8944444444444444864, 0.8958333333333333703, 0.8972222222222222543, 0.8986111111111111382, 0.9000000000000000222, 0.9013888888888889062, 0.9027777777777777901, 0.9041666666666666741, 0.9055555555555555580, 0.9069444444444444420, 0.9083333333333333259, 0.9097222222222222099, 0.9111111111111110938, 0.9124999999999999778, 0.9138888888888888618, 0.9152777777777777457, 0.9166666666666666297, 0.9180555555555555136, 0.9194444444444443976, 0.9208333333333332815, 0.9222222222222222765, 0.9236111111111111605, 0.9250000000000000444, 0.9263888888888889284, 0.9277777777777778123, 0.9291666666666666963, 0.9305555555555555802, 0.9319444444444444642, 0.9333333333333333481, 0.9347222222222222321, 0.9361111111111111160, 0.9375000000000000000, 0.9388888888888888840, 0.9402777777777777679, 0.9416666666666666519, 0.9430555555555555358, 0.9444444444444444198, 0.9458333333333333037, 0.9472222222222221877, 0.9486111111111110716, 0.9499999999999999556, 0.9513888888888888395, 0.9527777777777777235, 0.9541666666666667185, 0.9555555555555556024, 0.9569444444444444864, 0.9583333333333333703, 0.9597222222222222543, 0.9611111111111111382, 0.9625000000000000222, 0.9638888888888889062, 0.9652777777777777901, 0.9666666666666666741, 0.9680555555555555580, 0.9694444444444444420, 0.9708333333333333259, 0.9722222222222222099, 0.9736111111111110938, 0.9749999999999999778, 0.9763888888888888618, 0.9777777777777777457, 0.9791666666666666297, 0.9805555555555555136, 0.9819444444444443976, 0.9833333333333332815, 0.9847222222222222765, 0.9861111111111111605, 0.9875000000000000444, 0.9888888888888889284, 0.9902777777777778123, 0.9916666666666666963, 0.9930555555555555802, 0.9944444444444444642, 0.9958333333333333481, 0.9972222222222222321, 0.9986111111111111160, 1.000000000000000000 ),
 .UNSPECIFIED. ) 
 CURVE ( )  GEOMETRIC_REPRESENTATION_ITEM ( )  RATIONAL_B_SPLINE_CURVE ( ( 1.000000000000000000, 0.8660254037844387076, 1.000000000000000000, 0.8660254037844387076, 1.000000000000000000, 0.8660254037844387076, 1.000000000000000000, 0.8660254037844387076, 1.000000000000000000, 0.8660254037844387076, 1.000000000000000000, 0.8660254037844387076, 1.000000000000000000, 0.8660254037844387076, 1.000000000000000000, 0.8660254037844387076, 1.000000000000000000, 0.8660254037844387076, 1.000000000000000000, 0.8660254037844387076, 1.000000000000000000, 0.8660254037844387076, 1.000000000000000000, 0.8660254037844387076, 1.000000000000000000, 0.8660254037844387076, 1.000000000000000000, 0.8660254037844387076, 1.000000000000000000, 0.8660254037844387076, 1.000000000000000000, 0.8660254037844387076, 1.000000000000000000, 0.8660254037844387076, 1.000000000000000000, 0.8660254037844387076, 1.000000000000000000, 0.8660254037844387076, 1.000000000000000000, 0.8660254037844387076, 1.000000000000000000, 0.8660254037844387076, 1.000000000000000000, 0.8660254037844387076, 1.000000000000000000, 0.8660254037844387076, 1.000000000000000000, 0.8660254037844387076, 1.000000000000000000, 0.8660254037844387076, 1.000000000000000000, 0.8660254037844387076, 1.000000000000000000, 0.8660254037844387076, 1.000000000000000000, 0.8660254037844387076, 1.000000000000000000, 0.8660254037844387076, 1.000000000000000000, 0.8660254037844387076, 1.000000000000000000, 0.8660254037844387076, 1.000000000000000000, 0.8660254037844387076, 1.000000000000000000, 0.8660254037844387076, 1.000000000000000000, 0.8660254037844387076, 1.000000000000000000, 0.8660254037844387076, 1.000000000000000000, 0.8660254037844387076, 1.000000000000000000, 0.8660254037844387076, 1.000000000000000000, 0.8660254037844387076, 1.000000000000000000, 0.8660254037844387076, 1.000000000000000000, 0.8660254037844387076, 1.000000000000000000, 0.8660254037844387076, 1.000000000000000000, 0.8660254037844387076, 1.000000000000000000, 0.8660254037844387076, 1.000000000000000000, 0.8660254037844387076, 1.000000000000000000, 0.8660254037844387076, 1.000000000000000000, 0.8660254037844387076, 1.000000000000000000, 0.8660254037844387076, 1.000000000000000000, 0.8660254037844387076, 1.000000000000000000, 0.8660254037844387076, 1.000000000000000000, 0.8660254037844387076, 1.000000000000000000, 0.8660254037844387076, 1.000000000000000000, 0.8660254037844387076, 1.000000000000000000, 0.8660254037844387076, 1.000000000000000000, 0.8660254037844387076, 1.000000000000000000, 0.8660254037844387076, 1.000000000000000000, 0.8660254037844387076, 1.000000000000000000, 0.8660254037844387076, 1.000000000000000000, 0.8660254037844387076, 1.000000000000000000, 0.8660254037844387076, 1.000000000000000000, 0.8660254037844387076, 1.000000000000000000, 0.8660254037844387076, 1.000000000000000000, 0.8660254037844387076, 1.000000000000000000, 0.8660254037844387076, 1.000000000000000000, 0.8660254037844387076, 1.000000000000000000, 0.8660254037844387076, 1.000000000000000000, 0.8660254037844387076, 1.000000000000000000, 0.8660254037844387076, 1.000000000000000000, 0.8660254037844387076, 1.000000000000000000, 0.8660254037844387076, 1.000000000000000000, 0.8660254037844387076, 1.000000000000000000, 0.8660254037844387076, 1.000000000000000000, 0.8660254037844387076, 1.000000000000000000, 0.8660254037844387076, 1.000000000000000000, 0.8660254037844387076, 1.000000000000000000, 0.8660254037844387076, 1.000000000000000000, 0.8660254037844387076, 1.000000000000000000, 0.8660254037844387076, 1.000000000000000000, 0.8660254037844387076, 1.000000000000000000, 0.8660254037844387076, 1.000000000000000000, 0.8660254037844387076, 1.000000000000000000, 0.8660254037844387076, 1.000000000000000000, 0.8660254037844387076, 1.000000000000000000, 0.8660254037844387076, 1.000000000000000000, 0.8660254037844387076, 1.000000000000000000, 0.8660254037844387076, 1.000000000000000000, 0.8660254037844387076, 1.000000000000000000, 0.8660254037844387076, 1.000000000000000000, 0.8660254037844387076, 1.000000000000000000, 0.8660254037844387076, 1.000000000000000000, 0.8660254037844387076, 1.000000000000000000, 0.8660254037844387076, 1.000000000000000000, 0.8660254037844387076, 1.000000000000000000, 0.8660254037844387076, 1.000000000000000000, 0.8660254037844387076, 1.000000000000000000, 0.8660254037844387076, 1.000000000000000000, 0.8660254037844387076, 1.000000000000000000, 0.8660254037844387076, 1.000000000000000000, 0.8660254037844387076, 1.000000000000000000, 0.8660254037844387076, 1.000000000000000000, 0.8660254037844387076, 1.000000000000000000, 0.8660254037844387076, 1.000000000000000000, 0.8660254037844387076, 1.000000000000000000, 0.8660254037844387076, 1.000000000000000000, 0.8660254037844387076, 1.000000000000000000, 0.8660254037844387076, 1.000000000000000000, 0.8660254037844387076, 1.000000000000000000, 0.8660254037844387076, 1.000000000000000000, 0.8660254037844387076, 1.000000000000000000, 0.8660254037844387076, 1.000000000000000000, 0.8660254037844387076, 1.000000000000000000, 0.8660254037844387076, 1.000000000000000000, 0.8660254037844387076, 1.000000000000000000, 0.8660254037844387076, 1.000000000000000000, 0.8660254037844387076, 1.000000000000000000, 0.8660254037844387076, 1.000000000000000000, 0.8660254037844387076, 1.000000000000000000, 0.8660254037844387076, 1.000000000000000000, 0.8660254037844387076, 1.000000000000000000, 0.8660254037844387076, 1.000000000000000000, 0.8660254037844387076, 1.000000000000000000, 0.8660254037844387076, 1.000000000000000000, 0.8660254037844387076, 1.000000000000000000, 0.8660254037844387076, 1.000000000000000000, 0.8660254037844387076, 1.000000000000000000, 0.8660254037844387076, 1.000000000000000000, 0.8660254037844387076, 1.000000000000000000, 0.8660254037844387076, 1.000000000000000000, 0.8660254037844387076, 1.000000000000000000, 0.8660254037844387076, 1.000000000000000000, 0.8660254037844387076, 1.000000000000000000, 0.8660254037844387076, 1.000000000000000000, 0.8660254037844387076, 1.000000000000000000, 0.8660254037844387076, 1.000000000000000000, 0.8660254037844387076, 1.000000000000000000, 0.8660254037844387076, 1.000000000000000000, 0.8660254037844387076, 1.000000000000000000, 0.8660254037844387076, 1.000000000000000000, 0.8660254037844387076, 1.000000000000000000, 0.8660254037844387076, 1.000000000000000000, 0.8660254037844387076, 1.000000000000000000, 0.8660254037844387076, 1.000000000000000000, 0.8660254037844387076, 1.000000000000000000, 0.8660254037844387076, 1.000000000000000000, 0.8660254037844387076, 1.000000000000000000, 0.8660254037844387076, 1.000000000000000000, 0.8660254037844387076, 1.000000000000000000, 0.8660254037844387076, 1.000000000000000000, 0.8660254037844387076, 1.000000000000000000, 0.8660254037844387076, 1.000000000000000000, 0.8660254037844387076, 1.000000000000000000, 0.8660254037844387076, 1.000000000000000000, 0.8660254037844387076, 1.000000000000000000, 0.8660254037844387076, 1.000000000000000000, 0.8660254037844387076, 1.000000000000000000, 0.8660254037844387076, 1.000000000000000000, 0.8660254037844387076, 1.000000000000000000, 0.8660254037844387076, 1.000000000000000000, 0.8660254037844387076, 1.000000000000000000, 0.8660254037844387076, 1.000000000000000000, 0.8660254037844387076, 1.000000000000000000, 0.8660254037844387076, 1.000000000000000000, 0.8660254037844387076, 1.000000000000000000, 0.8660254037844387076, 1.000000000000000000, 0.8660254037844387076, 1.000000000000000000, 0.8660254037844387076, 1.000000000000000000, 0.8660254037844387076, 1.000000000000000000, 0.8660254037844387076, 1.000000000000000000, 0.8660254037844387076, 1.000000000000000000, 0.8660254037844387076, 1.000000000000000000, 0.8660254037844387076, 1.000000000000000000, 0.8660254037844387076, 1.000000000000000000, 0.8660254037844387076, 1.000000000000000000, 0.8660254037844387076, 1.000000000000000000, 0.8660254037844387076, 1.000000000000000000, 0.8660254037844387076, 1.000000000000000000, 0.8660254037844387076, 1.000000000000000000, 0.8660254037844387076, 1.000000000000000000, 0.8660254037844387076, 1.000000000000000000, 0.8660254037844387076, 1.000000000000000000, 0.8660254037844387076, 1.000000000000000000, 0.8660254037844387076, 1.000000000000000000, 0.8660254037844387076, 1.000000000000000000, 0.8660254037844387076, 1.000000000000000000, 0.8660254037844387076, 1.000000000000000000, 0.8660254037844387076, 1.000000000000000000, 0.8660254037844387076, 1.000000000000000000, 0.8660254037844387076, 1.000000000000000000, 0.8660254037844387076, 1.000000000000000000, 0.8660254037844387076, 1.000000000000000000, 0.8660254037844387076, 1.000000000000000000, 0.8660254037844387076, 1.000000000000000000, 0.8660254037844387076, 1.000000000000000000, 0.8660254037844387076, 1.000000000000000000, 0.8660254037844387076, 1.000000000000000000, 0.8660254037844387076, 1.000000000000000000, 0.8660254037844387076, 1.000000000000000000, 0.8660254037844387076, 1.000000000000000000, 0.8660254037844387076, 1.000000000000000000, 0.8660254037844387076, 1.000000000000000000, 0.8660254037844387076, 1.000000000000000000, 0.8660254037844387076, 1.000000000000000000, 0.8660254037844387076, 1.000000000000000000, 0.8660254037844387076, 1.000000000000000000, 0.8660254037844387076, 1.000000000000000000, 0.8660254037844387076, 1.000000000000000000, 0.8660254037844387076, 1.000000000000000000, 0.8660254037844387076, 1.000000000000000000, 0.8660254037844387076, 1.000000000000000000, 0.8660254037844387076, 1.000000000000000000, 0.8660254037844387076, 1.000000000000000000, 0.8660254037844387076, 1.000000000000000000, 0.8660254037844387076, 1.000000000000000000, 0.8660254037844387076, 1.000000000000000000, 0.8660254037844387076, 1.000000000000000000, 0.8660254037844387076, 1.000000000000000000, 0.8660254037844387076, 1.000000000000000000, 0.8660254037844387076, 1.000000000000000000, 0.8660254037844387076, 1.000000000000000000, 0.8660254037844387076, 1.000000000000000000, 0.8660254037844387076, 1.000000000000000000, 0.8660254037844387076, 1.000000000000000000, 0.8660254037844387076, 1.000000000000000000, 0.8660254037844387076, 1.000000000000000000, 0.8660254037844387076, 1.000000000000000000, 0.8660254037844387076, 1.000000000000000000, 0.8660254037844387076, 1.000000000000000000, 0.8660254037844387076, 1.000000000000000000, 0.8660254037844387076, 1.000000000000000000, 0.8660254037844387076, 1.000000000000000000, 0.8660254037844387076, 1.000000000000000000, 0.8660254037844387076, 1.000000000000000000, 0.8660254037844387076, 1.000000000000000000, 0.8660254037844387076, 1.000000000000000000, 0.8660254037844387076, 1.000000000000000000, 0.8660254037844387076, 1.000000000000000000, 0.8660254037844387076, 1.000000000000000000, 0.8660254037844387076, 1.000000000000000000, 0.8660254037844387076, 1.000000000000000000, 0.8660254037844387076, 1.000000000000000000, 0.8660254037844387076, 1.000000000000000000, 0.8660254037844387076, 1.000000000000000000, 0.8660254037844387076, 1.000000000000000000, 0.8660254037844387076, 1.000000000000000000, 0.8660254037844387076, 1.000000000000000000, 0.8660254037844387076, 1.000000000000000000, 0.8660254037844387076, 1.000000000000000000, 0.8660254037844387076, 1.000000000000000000, 0.8660254037844387076, 1.000000000000000000, 0.8660254037844387076, 1.000000000000000000, 0.8660254037844387076, 1.000000000000000000, 0.8660254037844387076, 1.000000000000000000, 0.8660254037844387076, 1.000000000000000000, 0.8660254037844387076, 1.000000000000000000, 0.8660254037844387076, 1.000000000000000000, 0.8660254037844387076, 1.000000000000000000, 0.8660254037844387076, 1.000000000000000000, 0.8660254037844387076, 1.000000000000000000, 0.8660254037844387076, 1.000000000000000000, 0.8660254037844387076, 1.000000000000000000, 0.8660254037844387076, 1.000000000000000000, 0.8660254037844387076, 1.000000000000000000, 0.8660254037844387076, 1.000000000000000000, 0.8660254037844387076, 1.000000000000000000, 0.8660254037844387076, 1.000000000000000000, 0.8660254037844387076, 1.000000000000000000, 0.8660254037844387076, 1.000000000000000000, 0.8660254037844387076, 1.000000000000000000, 0.8660254037844387076, 1.000000000000000000, 0.8660254037844387076, 1.000000000000000000, 0.8660254037844387076, 1.000000000000000000, 0.8660254037844387076, 1.000000000000000000, 0.8660254037844387076, 1.000000000000000000, 0.8660254037844387076, 1.000000000000000000, 0.8660254037844387076, 1.000000000000000000, 0.8660254037844387076, 1.000000000000000000, 0.8660254037844387076, 1.000000000000000000, 0.8660254037844387076, 1.000000000000000000, 0.8660254037844387076, 1.000000000000000000, 0.8660254037844387076, 1.000000000000000000, 0.8660254037844387076, 1.000000000000000000, 0.8660254037844387076, 1.000000000000000000, 0.8660254037844387076, 1.000000000000000000, 0.8660254037844387076, 1.000000000000000000, 0.8660254037844387076, 1.000000000000000000, 0.8660254037844387076, 1.000000000000000000, 0.8660254037844387076, 1.000000000000000000, 0.8660254037844387076, 1.000000000000000000, 0.8660254037844387076, 1.000000000000000000, 0.8660254037844387076, 1.000000000000000000, 0.8660254037844387076, 1.000000000000000000, 0.8660254037844387076, 1.000000000000000000, 0.8660254037844387076, 1.000000000000000000, 0.8660254037844387076, 1.000000000000000000, 0.8660254037844387076, 1.000000000000000000, 0.8660254037844387076, 1.000000000000000000, 0.8660254037844387076, 1.000000000000000000, 0.8660254037844387076, 1.000000000000000000, 0.8660254037844387076, 1.000000000000000000, 0.8660254037844387076, 1.000000000000000000, 0.8660254037844387076, 1.000000000000000000, 0.8660254037844387076, 1.000000000000000000, 0.8660254037844387076, 1.000000000000000000, 0.8660254037844387076, 1.000000000000000000, 0.8660254037844387076, 1.000000000000000000, 0.8660254037844387076, 1.000000000000000000, 0.8660254037844387076, 1.000000000000000000, 0.8660254037844387076, 1.000000000000000000, 0.8660254037844387076, 1.000000000000000000, 0.8660254037844387076, 1.000000000000000000, 0.8660254037844387076, 1.000000000000000000, 0.8660254037844387076, 1.000000000000000000, 0.8660254037844387076, 1.000000000000000000, 0.8660254037844387076, 1.000000000000000000, 0.8660254037844387076, 1.000000000000000000, 0.8660254037844387076, 1.000000000000000000, 0.8660254037844387076, 1.000000000000000000, 0.8660254037844387076, 1.000000000000000000, 0.8660254037844387076, 1.000000000000000000, 0.8660254037844387076, 1.000000000000000000, 0.8660254037844387076, 1.000000000000000000, 0.8660254037844387076, 1.000000000000000000, 0.8660254037844387076, 1.000000000000000000, 0.8660254037844387076, 1.000000000000000000, 0.8660254037844387076, 1.000000000000000000, 0.8660254037844387076, 1.000000000000000000, 0.8660254037844387076, 1.000000000000000000, 0.8660254037844387076, 1.000000000000000000, 0.8660254037844387076, 1.000000000000000000, 0.8660254037844387076, 1.000000000000000000, 0.8660254037844387076, 1.000000000000000000, 0.8660254037844387076, 1.000000000000000000, 0.8660254037844387076, 1.000000000000000000, 0.8660254037844387076, 1.000000000000000000, 0.8660254037844387076, 1.000000000000000000, 0.8660254037844387076, 1.000000000000000000, 0.8660254037844387076, 1.000000000000000000, 0.8660254037844387076, 1.000000000000000000, 0.8660254037844387076, 1.000000000000000000, 0.8660254037844387076, 1.000000000000000000, 0.8660254037844387076, 1.000000000000000000, 0.8660254037844387076, 1.000000000000000000, 0.8660254037844387076, 1.000000000000000000, 0.8660254037844387076, 1.000000000000000000, 0.8660254037844387076, 1.000000000000000000, 0.8660254037844387076, 1.000000000000000000, 0.8660254037844387076, 1.000000000000000000, 0.8660254037844387076, 1.000000000000000000, 0.8660254037844387076, 1.000000000000000000, 0.8660254037844387076, 1.000000000000000000, 0.8660254037844387076, 1.000000000000000000, 0.8660254037844387076, 1.000000000000000000, 0.8660254037844387076, 1.000000000000000000, 0.8660254037844387076, 1.000000000000000000, 0.8660254037844387076, 1.000000000000000000, 0.8660254037844387076, 1.000000000000000000, 0.8660254037844387076, 1.000000000000000000, 0.8660254037844387076, 1.000000000000000000, 0.8660254037844387076, 1.000000000000000000, 0.8660254037844387076, 1.000000000000000000, 0.8660254037844387076, 1.000000000000000000, 0.8660254037844387076, 1.000000000000000000, 0.8660254037844387076, 1.000000000000000000, 0.8660254037844387076, 1.000000000000000000, 0.8660254037844387076, 1.000000000000000000, 0.8660254037844387076, 1.000000000000000000, 0.8660254037844387076, 1.000000000000000000, 0.8660254037844387076, 1.000000000000000000, 0.8660254037844387076, 1.000000000000000000, 0.8660254037844387076, 1.000000000000000000, 0.8660254037844387076, 1.000000000000000000, 0.8660254037844387076, 1.000000000000000000, 0.8660254037844387076, 1.000000000000000000, 0.8660254037844387076, 1.000000000000000000, 0.8660254037844387076, 1.000000000000000000, 0.8660254037844387076, 1.000000000000000000, 0.8660254037844387076, 1.000000000000000000, 0.8660254037844387076, 1.000000000000000000, 0.8660254037844387076, 1.000000000000000000, 0.8660254037844387076, 1.000000000000000000, 0.8660254037844387076, 1.000000000000000000, 0.8660254037844387076, 1.000000000000000000, 0.8660254037844387076, 1.000000000000000000, 0.8660254037844387076, 1.000000000000000000, 0.8660254037844387076, 1.000000000000000000, 0.8660254037844387076, 1.000000000000000000, 0.8660254037844387076, 1.000000000000000000, 0.8660254037844387076, 1.000000000000000000, 0.8660254037844387076, 1.000000000000000000, 0.8660254037844387076, 1.000000000000000000, 0.8660254037844387076, 1.000000000000000000, 0.8660254037844387076, 1.000000000000000000, 0.8660254037844387076, 1.000000000000000000, 0.8660254037844387076, 1.000000000000000000, 0.8660254037844387076, 1.000000000000000000, 0.8660254037844387076, 1.000000000000000000, 0.8660254037844387076, 1.000000000000000000, 0.8660254037844387076, 1.000000000000000000, 0.8660254037844387076, 1.000000000000000000, 0.8660254037844387076, 1.000000000000000000, 0.8660254037844387076, 1.000000000000000000, 0.8660254037844387076, 1.000000000000000000, 0.8660254037844387076, 1.000000000000000000, 0.8660254037844387076, 1.000000000000000000, 0.8660254037844387076, 1.000000000000000000, 0.8660254037844387076, 1.000000000000000000, 0.8660254037844387076, 1.000000000000000000, 0.8660254037844387076, 1.000000000000000000, 0.8660254037844387076, 1.000000000000000000, 0.8660254037844387076, 1.000000000000000000, 0.8660254037844387076, 1.000000000000000000, 0.8660254037844387076, 1.000000000000000000, 0.8660254037844387076, 1.000000000000000000, 0.8660254037844387076, 1.000000000000000000, 0.8660254037844387076, 1.000000000000000000, 0.8660254037844387076, 1.000000000000000000, 0.8660254037844387076, 1.000000000000000000, 0.8660254037844387076, 1.000000000000000000, 0.8660254037844387076, 1.000000000000000000, 0.8660254037844387076, 1.000000000000000000, 0.8660254037844387076, 1.000000000000000000, 0.8660254037844387076, 1.000000000000000000, 0.8660254037844387076, 1.000000000000000000, 0.8660254037844387076, 1.000000000000000000, 0.8660254037844387076, 1.000000000000000000, 0.8660254037844387076, 1.000000000000000000, 0.8660254037844387076, 1.000000000000000000, 0.8660254037844387076, 1.000000000000000000, 0.8660254037844387076, 1.000000000000000000, 0.8660254037844387076, 1.000000000000000000, 0.8660254037844387076, 1.000000000000000000, 0.8660254037844387076, 1.000000000000000000, 0.8660254037844387076, 1.000000000000000000, 0.8660254037844387076, 1.000000000000000000, 0.8660254037844387076, 1.000000000000000000, 0.8660254037844387076, 1.000000000000000000, 0.8660254037844387076, 1.000000000000000000, 0.8660254037844387076, 1.000000000000000000, 0.8660254037844387076, 1.000000000000000000, 0.8660254037844387076, 1.000000000000000000, 0.8660254037844387076, 1.000000000000000000, 0.8660254037844387076, 1.000000000000000000, 0.8660254037844387076, 1.000000000000000000, 0.8660254037844387076, 1.000000000000000000, 0.8660254037844387076, 1.000000000000000000, 0.8660254037844387076, 1.000000000000000000, 0.8660254037844387076, 1.000000000000000000, 0.8660254037844387076, 1.000000000000000000, 0.8660254037844387076, 1.000000000000000000, 0.8660254037844387076, 1.000000000000000000, 0.8660254037844387076, 1.000000000000000000, 0.8660254037844387076, 1.000000000000000000, 0.8660254037844387076, 1.000000000000000000, 0.8660254037844387076, 1.000000000000000000, 0.8660254037844387076, 1.000000000000000000, 0.8660254037844387076, 1.000000000000000000, 0.8660254037844387076, 1.000000000000000000, 0.8660254037844387076, 1.000000000000000000, 0.8660254037844387076, 1.000000000000000000, 0.8660254037844387076, 1.000000000000000000, 0.8660254037844387076, 1.000000000000000000, 0.8660254037844387076, 1.000000000000000000, 0.8660254037844387076, 1.000000000000000000, 0.8660254037844387076, 1.000000000000000000, 0.8660254037844387076, 1.000000000000000000, 0.8660254037844387076, 1.000000000000000000, 0.8660254037844387076, 1.000000000000000000, 0.8660254037844387076, 1.000000000000000000, 0.8660254037844387076, 1.000000000000000000, 0.8660254037844387076, 1.000000000000000000, 0.8660254037844387076, 1.000000000000000000, 0.8660254037844387076, 1.000000000000000000, 0.8660254037844387076, 1.000000000000000000, 0.8660254037844387076, 1.000000000000000000, 0.8660254037844387076, 1.000000000000000000, 0.8660254037844387076, 1.000000000000000000, 0.8660254037844387076, 1.000000000000000000, 0.8660254037844387076, 1.000000000000000000, 0.8660254037844387076, 1.000000000000000000, 0.8660254037844387076, 1.000000000000000000, 0.8660254037844387076, 1.000000000000000000, 0.8660254037844387076, 1.000000000000000000, 0.8660254037844387076, 1.000000000000000000, 0.8660254037844387076, 1.000000000000000000, 0.8660254037844387076, 1.000000000000000000, 0.8660254037844387076, 1.000000000000000000, 0.8660254037844387076, 1.000000000000000000, 0.8660254037844387076, 1.000000000000000000, 0.8660254037844387076, 1.000000000000000000, 0.8660254037844387076, 1.000000000000000000, 0.8660254037844387076, 1.000000000000000000, 0.8660254037844387076, 1.000000000000000000, 0.8660254037844387076, 1.000000000000000000, 0.8660254037844387076, 1.000000000000000000, 0.8660254037844387076, 1.000000000000000000, 0.8660254037844387076, 1.000000000000000000, 0.8660254037844387076, 1.000000000000000000, 0.8660254037844387076, 1.000000000000000000, 0.8660254037844387076, 1.000000000000000000, 0.8660254037844387076, 1.000000000000000000, 0.8660254037844387076, 1.000000000000000000, 0.8660254037844387076, 1.000000000000000000, 0.8660254037844387076, 1.000000000000000000, 0.8660254037844387076, 1.000000000000000000, 0.8660254037844387076, 1.000000000000000000, 0.8660254037844387076, 1.000000000000000000, 0.8660254037844387076, 1.000000000000000000, 0.8660254037844387076, 1.000000000000000000, 0.8660254037844387076, 1.000000000000000000, 0.8660254037844387076, 1.000000000000000000, 0.8660254037844387076, 1.000000000000000000, 0.8660254037844387076, 1.000000000000000000, 0.8660254037844387076, 1.000000000000000000, 0.8660254037844387076, 1.000000000000000000, 0.8660254037844387076, 1.000000000000000000, 0.8660254037844387076, 1.000000000000000000, 0.8660254037844387076, 1.000000000000000000, 0.8660254037844387076, 1.000000000000000000, 0.8660254037844387076, 1.000000000000000000, 0.8660254037844387076, 1.000000000000000000, 0.8660254037844387076, 1.000000000000000000, 0.8660254037844387076, 1.000000000000000000, 0.8660254037844387076, 1.000000000000000000, 0.8660254037844387076, 1.000000000000000000, 0.8660254037844387076, 1.000000000000000000, 0.8660254037844387076, 1.000000000000000000, 0.8660254037844387076, 1.000000000000000000, 0.8660254037844387076, 1.000000000000000000, 0.8660254037844387076, 1.000000000000000000, 0.8660254037844387076, 1.000000000000000000, 0.8660254037844387076, 1.000000000000000000, 0.8660254037844387076, 1.000000000000000000, 0.8660254037844387076, 1.000000000000000000, 0.8660254037844387076, 1.000000000000000000, 0.8660254037844387076, 1.000000000000000000, 0.8660254037844387076, 1.000000000000000000, 0.8660254037844387076, 1.000000000000000000, 0.8660254037844387076, 1.000000000000000000, 0.8660254037844387076, 1.000000000000000000, 0.8660254037844387076, 1.000000000000000000, 0.8660254037844387076, 1.000000000000000000, 0.8660254037844387076, 1.000000000000000000, 0.8660254037844387076, 1.000000000000000000, 0.8660254037844387076, 1.000000000000000000, 0.8660254037844387076, 1.000000000000000000, 0.8660254037844387076, 1.000000000000000000, 0.8660254037844387076, 1.000000000000000000, 0.8660254037844387076, 1.000000000000000000, 0.8660254037844387076, 1.000000000000000000, 0.8660254037844387076, 1.000000000000000000, 0.8660254037844387076, 1.000000000000000000, 0.8660254037844387076, 1.000000000000000000, 0.8660254037844387076, 1.000000000000000000, 0.8660254037844387076, 1.000000000000000000, 0.8660254037844387076, 1.000000000000000000, 0.8660254037844387076, 1.000000000000000000, 0.8660254037844387076, 1.000000000000000000, 0.8660254037844387076, 1.000000000000000000, 0.8660254037844387076, 1.000000000000000000, 0.8660254037844387076, 1.000000000000000000, 0.8660254037844387076, 1.000000000000000000, 0.8660254037844387076, 1.000000000000000000, 0.8660254037844387076, 1.000000000000000000, 0.8660254037844387076, 1.000000000000000000, 0.8660254037844387076, 1.000000000000000000, 0.8660254037844387076, 1.000000000000000000, 0.8660254037844387076, 1.000000000000000000, 0.8660254037844387076, 1.000000000000000000, 0.8660254037844387076, 1.000000000000000000, 0.8660254037844387076, 1.000000000000000000, 0.8660254037844387076, 1.000000000000000000, 0.8660254037844387076, 1.000000000000000000, 0.8660254037844387076, 1.000000000000000000, 0.8660254037844387076, 1.000000000000000000, 0.8660254037844387076, 1.000000000000000000, 0.8660254037844387076, 1.000000000000000000, 0.8660254037844387076, 1.000000000000000000, 0.8660254037844387076, 1.000000000000000000, 0.8660254037844387076, 1.000000000000000000, 0.8660254037844387076, 1.000000000000000000, 0.8660254037844387076, 1.000000000000000000, 0.8660254037844387076, 1.000000000000000000, 0.8660254037844387076, 1.000000000000000000, 0.8660254037844387076, 1.000000000000000000, 0.8660254037844387076, 1.000000000000000000, 0.8660254037844387076, 1.000000000000000000, 0.8660254037844387076, 1.000000000000000000, 0.8660254037844387076, 1.000000000000000000, 0.8660254037844387076, 1.000000000000000000, 0.8660254037844387076, 1.000000000000000000, 0.8660254037844387076, 1.000000000000000000, 0.8660254037844387076, 1.000000000000000000, 0.8660254037844387076, 1.000000000000000000, 0.8660254037844387076, 1.000000000000000000, 0.8660254037844387076, 1.000000000000000000, 0.8660254037844387076, 1.000000000000000000, 0.8660254037844387076, 1.000000000000000000, 0.8660254037844387076, 1.000000000000000000, 0.8660254037844387076, 1.000000000000000000, 0.8660254037844387076, 1.000000000000000000, 0.8660254037844387076, 1.000000000000000000, 0.8660254037844387076, 1.000000000000000000, 0.8660254037844387076, 1.000000000000000000, 0.8660254037844387076, 1.000000000000000000, 0.8660254037844387076, 1.000000000000000000, 0.8660254037844387076, 1.000000000000000000, 0.8660254037844387076, 1.000000000000000000, 0.8660254037844387076, 1.000000000000000000, 0.8660254037844387076, 1.000000000000000000, 0.8660254037844387076, 1.000000000000000000, 0.8660254037844387076, 1.000000000000000000, 0.8660254037844387076, 1.000000000000000000, 0.8660254037844387076, 1.000000000000000000, 0.8660254037844387076, 1.000000000000000000, 0.8660254037844387076, 1.000000000000000000, 0.8660254037844387076, 1.000000000000000000, 0.8660254037844387076, 1.000000000000000000, 0.8660254037844387076, 1.000000000000000000, 0.8660254037844387076, 1.000000000000000000, 0.8660254037844387076, 1.000000000000000000, 0.8660254037844387076, 1.000000000000000000, 0.8660254037844387076, 1.000000000000000000, 0.8660254037844387076, 1.000000000000000000, 0.8660254037844387076, 1.000000000000000000, 0.8660254037844387076, 1.000000000000000000, 0.8660254037844387076, 1.000000000000000000, 0.8660254037844387076, 1.000000000000000000, 0.8660254037844387076, 1.000000000000000000, 0.8660254037844387076, 1.000000000000000000, 0.8660254037844387076, 1.000000000000000000, 0.8660254037844387076, 1.000000000000000000, 0.8660254037844387076, 1.000000000000000000, 0.8660254037844387076, 1.000000000000000000, 0.8660254037844387076, 1.000000000000000000, 0.8660254037844387076, 1.000000000000000000, 0.8660254037844387076, 1.000000000000000000, 0.8660254037844387076, 1.000000000000000000, 0.8660254037844387076, 1.000000000000000000, 0.8660254037844387076, 1.000000000000000000, 0.8660254037844387076, 1.000000000000000000, 0.8660254037844387076, 1.000000000000000000, 0.8660254037844387076, 1.000000000000000000, 0.8660254037844387076, 1.000000000000000000, 0.8660254037844387076, 1.000000000000000000, 0.8660254037844387076, 1.000000000000000000, 0.8660254037844387076, 1.000000000000000000, 0.8660254037844387076, 1.000000000000000000, 0.8660254037844387076, 1.000000000000000000, 0.8660254037844387076, 1.000000000000000000, 0.8660254037844387076, 1.000000000000000000, 0.8660254037844387076, 1.000000000000000000, 0.8660254037844387076, 1.000000000000000000, 0.8660254037844387076, 1.000000000000000000, 0.8660254037844387076, 1.000000000000000000, 0.8660254037844387076, 1.000000000000000000, 0.8660254037844387076, 1.000000000000000000, 0.8660254037844387076, 1.000000000000000000, 0.8660254037844387076, 1.000000000000000000, 0.8660254037844387076, 1.000000000000000000, 0.8660254037844387076, 1.000000000000000000, 0.8660254037844387076, 1.000000000000000000, 0.8660254037844387076, 1.000000000000000000, 0.8660254037844387076, 1.000000000000000000, 0.8660254037844387076, 1.000000000000000000, 0.8660254037844387076, 1.000000000000000000, 0.8660254037844387076, 1.000000000000000000, 0.8660254037844387076, 1.000000000000000000, 0.8660254037844387076, 1.000000000000000000, 0.8660254037844387076, 1.000000000000000000, 0.8660254037844387076, 1.000000000000000000, 0.8660254037844387076, 1.000000000000000000, 0.8660254037844387076, 1.000000000000000000, 0.8660254037844387076, 1.000000000000000000, 0.8660254037844387076, 1.000000000000000000, 0.8660254037844387076, 1.000000000000000000, 0.8660254037844387076, 1.000000000000000000, 0.8660254037844387076, 1.000000000000000000, 0.8660254037844387076, 1.000000000000000000, 0.8660254037844387076, 1.000000000000000000, 0.8660254037844387076, 1.000000000000000000, 0.8660254037844387076, 1.000000000000000000, 0.8660254037844387076, 1.000000000000000000, 0.8660254037844387076, 1.000000000000000000, 0.8660254037844387076, 1.000000000000000000, 0.8660254037844387076, 1.000000000000000000, 0.8660254037844387076, 1.000000000000000000, 0.8660254037844387076, 1.000000000000000000, 0.8660254037844387076, 1.000000000000000000, 0.8660254037844387076, 1.000000000000000000, 0.8660254037844387076, 1.000000000000000000, 0.8660254037844387076, 1.000000000000000000, 0.8660254037844387076, 1.000000000000000000, 0.8660254037844387076, 1.000000000000000000, 0.8660254037844387076, 1.000000000000000000, 0.8660254037844387076, 1.000000000000000000, 0.8660254037844387076, 1.000000000000000000, 0.8660254037844387076, 1.000000000000000000, 0.8660254037844387076, 1.000000000000000000, 0.8660254037844387076, 1.000000000000000000, 0.8660254037844387076, 1.000000000000000000, 0.8660254037844387076, 1.000000000000000000, 0.8660254037844387076, 1.000000000000000000, 0.8660254037844387076, 1.000000000000000000, 0.8660254037844387076, 1.000000000000000000, 0.8660254037844387076, 1.000000000000000000, 0.8660254037844387076, 1.000000000000000000, 0.8660254037844387076, 1.000000000000000000, 0.8660254037844387076, 1.000000000000000000, 0.8660254037844387076, 1.000000000000000000, 0.8660254037844387076, 1.000000000000000000, 0.8660254037844387076, 1.000000000000000000, 0.8660254037844387076, 1.000000000000000000, 0.8660254037844387076, 1.000000000000000000, 0.8660254037844387076, 1.000000000000000000, 0.8660254037844387076, 1.000000000000000000, 0.8660254037844387076, 1.000000000000000000, 0.8660254037844387076, 1.000000000000000000, 0.8660254037844387076, 1.000000000000000000, 0.8660254037844387076, 1.000000000000000000, 0.8660254037844387076, 1.000000000000000000, 0.8660254037844387076, 1.000000000000000000 ) ) 
 REPRESENTATION_ITEM ( '' )  );
#40571=CARTESIAN_POINT ( 'NONE',  ( -3.310556943750001313, 17.50000000000001776, -93.85160580289947063 ) ) ;
#40572=CARTESIAN_POINT ( 'NONE',  ( 3.310556943750001313, 17.50000000000002487, -142.2641058028994792 ) ) ;
#40574=CARTESIAN_POINT ( 'NONE',  ( -7.022189441860112050E-16, 13.67729811471672896, -140.6016058028994564 ) ) ;
#40575=CARTESIAN_POINT ( 'NONE',  ( 1.749999999999998224, 14.46891108675448478, -121.6276474690881741 ) ) ;
#40576=CARTESIAN_POINT ( 'NONE',  ( 1.750000000000001110, 20.53108891324555429, -96.29431413575484555 ) ) ;
#40577=CYLINDRICAL_SURFACE ( 'NONE', #3493, 3.499999999999999556 ) ;
#40579=CARTESIAN_POINT ( 'NONE',  ( 3.500000000000001332, 17.50000000000001776, -87.15473080337743284 ) ) ;
#40580=CARTESIAN_POINT ( 'NONE',  ( 2.340729813953370519E-16, 21.32270188528331190, -68.10160580289947063 ) ) ;
#40584=FACE_OUTER_BOUND ( 'NONE', #25139, .T. ) ;
#40585=CARTESIAN_POINT ( 'NONE',  ( -3.500000000000000888, 19.52072594216370760, -49.04431413575484555 ) ) ;
#40586=CARTESIAN_POINT ( 'NONE',  ( 3.310556943750001313, 19.41135094264166838, -117.1807724695661506 ) ) ;
#40587=CARTESIAN_POINT ( 'NONE',  ( -0.9378221735089310451, 14.00000000000001599, -79.44938900211592170 ) ) ;
#40588=CARTESIAN_POINT ( 'NONE',  ( -1.394453263437886604E-15, 14.00000000000001776, -103.7109808024215027 ) ) ;
#40590=CARTESIAN_POINT ( 'NONE',  ( -3.500000000000000888, 19.52072594216371826, -112.7380641367107614 ) ) ;
#40593=CARTESIAN_POINT ( 'NONE',  ( 0.000000000000000000, 17.50000000000002487, -149.5231586289125687 ) ) ;
#40594=EDGE_CURVE ( 'NONE', #32798, #23290, #7723, .T. ) ;
#40597=CARTESIAN_POINT ( 'NONE',  ( 3.310556943750001313, 17.50000000000001421, -74.26410580289947916 ) ) ;
#40598=CARTESIAN_POINT ( 'NONE',  ( -1.749999999999999778, 20.53108891324555429, -97.12764746908817415 ) ) ;
#40599=CARTESIAN_POINT ( 'NONE',  ( -1.394453263437886604E-15, 14.00000000000001066, -49.40473080337742573 ) ) ;
#40601=CARTESIAN_POINT ( 'NONE',  ( -1.750000000000002220, 14.46891108675448834, -132.7943141357548598 ) ) ;
#40602=CARTESIAN_POINT ( 'NONE',  ( 1.749999999999998224, 14.46891108675447235, -25.62764746908817415 ) ) ;
#40603=CARTESIAN_POINT ( 'NONE',  ( -1.655278471875002211, 14.63297358603754716, -83.59743913623279354 ) ) ;
#40609=VERTEX_POINT ( 'NONE', #10271 ) ;
#40610=LINE ( 'NONE', #11468, #7130 ) ;
#40611=CARTESIAN_POINT ( 'NONE',  ( -1.655278471875002211, 14.63297358603754184, -47.68493913623279923 ) ) ;
#40612=CARTESIAN_POINT ( 'NONE',  ( -7.022189441860112050E-16, 13.67729811471672718, -116.6016058028994564 ) ) ;
#40613=EDGE_LOOP ( 'NONE', ( #30294, #31538, #10380, #35351 ) ) ;
#40614=CARTESIAN_POINT ( 'NONE',  ( -1.655278471874999990, 20.36702641396248481, -34.93077246956615056 ) ) ;
#40615=CARTESIAN_POINT ( 'NONE',  ( 3.310556943750001313, 17.50000000000001421, -66.35160580289945642 ) ) ;
#40616=CARTESIAN_POINT ( 'NONE',  ( -1.749999999999999778, 20.53108891324555785, -112.1276474690881884 ) ) ;
#40618=CARTESIAN_POINT ( 'NONE',  ( -3.310556943750002645, 15.58864905735837425, -96.68077246956612214 ) ) ;
#40620=CARTESIAN_POINT ( 'NONE',  ( -3.500000000000001332, 17.50000000000002132, -124.6547308033774186 ) ) ;
#40621=CARTESIAN_POINT ( 'NONE',  ( -0.9378221735089291577, 21.00000000000001421, -56.86007260463890844 ) ) ;
#40624=CARTESIAN_POINT ( 'NONE',  ( 3.500000000000001776, 19.52072594216370760, -62.37764746908818125 ) ) ;
#40626=CARTESIAN_POINT ( 'NONE',  ( -1.655278471875002211, 14.63297358603754006, -33.59743913623280775 ) ) ;
#40627=CARTESIAN_POINT ( 'NONE',  ( -3.310556943750000425, 19.41135094264166483, -88.93493913623281344 ) ) ;
#40628=CARTESIAN_POINT ( 'NONE',  ( 2.474675557024783212E-16, 21.54145188432739388, -53.90473080337743994 ) ) ;
#40629=CYLINDRICAL_SURFACE ( 'NONE', #38248, 3.499999999999999556 ) ;
#40630=CARTESIAN_POINT ( 'NONE',  ( 3.310556943749999981, 15.58864905735837070, -106.4349391362328134 ) ) ;
#40631=CARTESIAN_POINT ( 'NONE',  ( -1.655278471875002211, 14.63297358603754006, -38.68493913623280633 ) ) ;
#40633=CARTESIAN_POINT ( 'NONE',  ( -1.394453263437886604E-15, 14.00000000000001421, -66.40473080337741862 ) ) ;
#40637=CARTESIAN_POINT ( 'NONE',  ( 4.648177544792955347E-16, 21.00000000000001776, -81.21098080242150274 ) ) ;
#40639=CARTESIAN_POINT ( 'NONE',  ( 1.655278471874998436, 14.63297358603754539, -88.43077246956613635 ) ) ;
#40642=ORIENTED_EDGE ( 'NONE', *, *, #16489, .T. ) ;
#40643=CARTESIAN_POINT ( 'NONE',  ( 4.648177544792955347E-16, 21.00000000000001776, -102.2109808024215027 ) ) ;
#40652=VECTOR ( 'NONE', #38034, 1000.000000000000000 ) ;
#40661=CARTESIAN_POINT ( 'NONE',  ( -3.310556943750001313, 17.50000000000002487, -137.7641058028994792 ) ) ;
#40662=CARTESIAN_POINT ( 'NONE',  ( -1.394453263437886604E-15, 14.00000000000002132, -133.7109808024214885 ) ) ;
#40663=CARTESIAN_POINT ( 'NONE',  ( 4.648177544792955347E-16, 21.00000000000001421, -54.21098080242150985 ) ) ;
#40664=CARTESIAN_POINT ( 'NONE',  ( 3.310556943750001313, 17.50000000000002132, -128.3516058028994564 ) ) ;
#40665=CARTESIAN_POINT ( 'NONE',  ( -3.310556943750000425, 19.41135094264166128, -55.93493913623279212 ) ) ;
#40666=ORIENTED_EDGE ( 'NONE', *, *, #41477, .T. ) ;
#40668=CARTESIAN_POINT ( 'NONE',  ( -3.500000000000000888, 19.52072594216372181, -134.7380641367107614 ) ) ;
#40670=CARTESIAN_POINT ( 'NONE',  ( 1.750000000000001110, 20.53108891324555785, -127.2943141357548456 ) ) ;
#40671=CARTESIAN_POINT ( 'NONE',  ( -1.655278471874999990, 20.36702641396249547, -113.9307724695661364 ) ) ;
#40676=CARTESIAN_POINT ( 'NONE',  ( -3.500000000000000888, 19.52072594216371115, -83.04431413575484555 ) ) ;
#40677=AXIS2_PLACEMENT_3D ( 'NONE', #2833, #15403, #3044 ) ;
#40678=( BOUNDED_CURVE ( )  B_SPLINE_CURVE ( 2, ( #36549, #17623, #37188, #40163, #36986, #1659, #14218, #4440, #17420 ),
 .UNSPECIFIED., .F., .F. ) 
 B_SPLINE_CURVE_WITH_KNOTS ( ( 3, 2, 2, 2, 3 ),
 ( 0.08958333333333333426, 0.09027777777777777624, 0.09166666666666666019, 0.09305555555555555802, 0.09375000000000000000 ),
 .UNSPECIFIED. ) 
 CURVE ( )  GEOMETRIC_REPRESENTATION_ITEM ( )  RATIONAL_B_SPLINE_CURVE ( ( 0.9330127018922194093, 0.9330127018922194093, 1.000000000000000000, 0.8660254037844387076, 1.000000000000000000, 0.8660254037844387076, 1.000000000000000000, 0.9330127018922194093, 0.9330127018922194093 ) ) 
 REPRESENTATION_ITEM ( '' )  );
#40680=CARTESIAN_POINT ( 'NONE',  ( 3.310556943749999981, 15.58864905735836182, -47.34743913623280775 ) ) ;
#40681=EDGE_CURVE ( 'NONE', #31346, #16907, #36207, .T. ) ;
#40682=CARTESIAN_POINT ( 'NONE',  ( -3.310556943750001313, 17.50000000000002132, -108.8516058028994564 ) ) ;
#40683=( BOUNDED_CURVE ( )  B_SPLINE_CURVE ( 2, ( #39527, #16014, #3229, #23380, #35138, #16995, #5799, #34, #38539 ),
 .UNSPECIFIED., .F., .T. ) 
 B_SPLINE_CURVE_WITH_KNOTS ( ( 3, 2, 2, 2, 3 ),
 ( 0.6229166666666666741, 0.6236111111111111160, 0.6250000000000000000, 0.6263888888888888840, 0.6270833333333333259 ),
 .UNSPECIFIED. ) 
 CURVE ( )  GEOMETRIC_REPRESENTATION_ITEM ( )  RATIONAL_B_SPLINE_CURVE ( ( 0.9330127018922194093, 0.9330127018922194093, 1.000000000000000000, 0.8660254037844387076, 1.000000000000000000, 0.8660254037844387076, 1.000000000000000000, 0.9330127018922194093, 0.9330127018922194093 ) ) 
 REPRESENTATION_ITEM ( '' )  );
#40684=CARTESIAN_POINT ( 'NONE',  ( 3.500000000000001332, 17.50000000000002132, -111.1547308033774328 ) ) ;
#40685=CARTESIAN_POINT ( 'NONE',  ( -3.500000000000000000, 19.52072594216370405, -42.73806413671076143 ) ) ;
#40686=CARTESIAN_POINT ( 'NONE',  ( -1.655278471874999990, 20.36702641396249547, -122.0182724695661278 ) ) ;
#40689=CARTESIAN_POINT ( 'NONE',  ( -1.394453263437886604E-15, 14.00000000000002132, -124.4047308033774044 ) ) ;
#40691=CARTESIAN_POINT ( 'NONE',  ( 1.655278471875001101, 20.36702641396248836, -58.18493913623279212 ) ) ;
#40693=CARTESIAN_POINT ( 'NONE',  ( -3.310556943750002201, 15.58864905735837070, -78.76827246956615625 ) ) ;
#40695=CARTESIAN_POINT ( 'NONE',  ( 4.648177544792955347E-16, 21.00000000000001066, -29.90473080337743639 ) ) ;
#40699=CARTESIAN_POINT ( 'NONE',  ( -3.310556943750002201, 15.58864905735836537, -38.68077246956613635 ) ) ;
#40705=CARTESIAN_POINT ( 'NONE',  ( 1.655278471875001101, 20.36702641396248836, -48.09743913623280775 ) ) ;
#40706=ORIENTED_EDGE ( 'NONE', *, *, #12134, .F. ) ;
#40707=VERTEX_POINT ( 'NONE', #20265 ) ;
#40710=CARTESIAN_POINT ( 'NONE',  ( 3.500000000000001776, 19.52072594216370405, -24.37764746908817415 ) ) ;
#40713=VERTEX_POINT ( 'NONE', #1131 ) ;
#40714=CARTESIAN_POINT ( 'NONE',  ( 4.648177544792955347E-16, 21.00000000000002132, -112.2109808024214743 ) ) ;
#40715=CARTESIAN_POINT ( 'NONE',  ( 3.500000000000000000, 15.47927405783632082, -36.54431413575484555 ) ) ;
#40716=CARTESIAN_POINT ( 'NONE',  ( 0.9378221735089281585, 14.00000000000001776, -86.66632260368298546 ) ) ;
#40720=CARTESIAN_POINT ( 'NONE',  ( 3.500000000000001332, 17.50000000000002487, -142.4609808024215170 ) ) ;
#40721=CARTESIAN_POINT ( 'NONE',  ( -0.9378221735089291577, 21.00000000000002132, -106.8600726046389298 ) ) ;
#40722=CARTESIAN_POINT ( 'NONE',  ( 2.340729813953370519E-16, 21.32270188528332255, -130.0141058028994507 ) ) ;
#40725=EDGE_CURVE ( 'NONE', #9158, #12038, #24420, .T. ) ;
#40726=CYLINDRICAL_SURFACE ( 'NONE', #38813, 3.499999999999999556 ) ;
#40728=CARTESIAN_POINT ( 'NONE',  ( 1.655278471875001101, 20.36702641396249547, -124.1849391362327992 ) ) ;
#40729=CARTESIAN_POINT ( 'NONE',  ( 1.750000000000001110, 20.53108891324556140, -133.9880641367107614 ) ) ;
#40730=CARTESIAN_POINT ( 'NONE',  ( 3.500000000000001332, 17.50000000000001066, -40.15473080337743284 ) ) ;
#40731=CARTESIAN_POINT ( 'NONE',  ( 1.749999999999998224, 14.46891108675448478, -115.3213974700440900 ) ) ;
#40732=CARTESIAN_POINT ( 'NONE',  ( -1.394453263437886604E-15, 14.00000000000002132, -130.7109808024214885 ) ) ;
#40733=CARTESIAN_POINT ( 'NONE',  ( -1.394453263437886604E-15, 14.00000000000001776, -89.40473080337741862 ) ) ;
#40734=CARTESIAN_POINT ( 'NONE',  ( 3.500000000000001332, 17.50000000000001421, -68.15473080337743284 ) ) ;
#40736=CARTESIAN_POINT ( 'NONE',  ( -3.310556943750000425, 19.41135094264166483, -53.93493913623280633 ) ) ;
#40738=CARTESIAN_POINT ( 'NONE',  ( -0.9378221735089291577, 21.00000000000001066, -41.86007260463891555 ) ) ;
#40739=CARTESIAN_POINT ( 'NONE',  ( 1.655278471874998436, 14.63297358603754361, -73.51827246956612782 ) ) ;
#40742=CARTESIAN_POINT ( 'NONE',  ( -1.655278471875002211, 14.63297358603754894, -105.5974391362328078 ) ) ;
#40743=CARTESIAN_POINT ( 'NONE',  ( 2.340729813953370519E-16, 21.32270188528330834, -72.01410580289947916 ) ) ;
#40744=ORIENTED_EDGE ( 'NONE', *, *, #20753, .F. ) ;
#40745=CARTESIAN_POINT ( 'NONE',  ( 3.310556943750001313, 17.50000000000001776, -98.35160580289947063 ) ) ;
#40747=CARTESIAN_POINT ( 'NONE',  ( -3.500000000000000000, 19.52072594216371115, -86.73806413671076143 ) ) ;
#40748=CARTESIAN_POINT ( 'NONE',  ( -1.750000000000002220, 14.46891108675448301, -81.48806413671076143 ) ) ;
#40750=CARTESIAN_POINT ( 'NONE',  ( 2.340729813953370519E-16, 21.32270188528331190, -56.01410580289947916 ) ) ;
#40752=CARTESIAN_POINT ( 'NONE',  ( -1.655278471874999990, 20.36702641396249547, -109.9307724695661506 ) ) ;
#40753=CARTESIAN_POINT ( 'NONE',  ( 4.648177544792955347E-16, 21.00000000000001066, -36.21098080242150985 ) ) ;
#40754=VECTOR ( 'NONE', #40386, 1000.000000000000000 ) ;
#40759=CARTESIAN_POINT ( 'NONE',  ( -0.9378221735089291577, 21.00000000000002132, -110.1663226036829855 ) ) ;
#40760=CARTESIAN_POINT ( 'NONE',  ( -3.310556943750000425, 19.41135094264166128, -60.84743913623280775 ) ) ;
#40761=( BOUNDED_CURVE ( )  B_SPLINE_CURVE ( 2, ( #1670, #27619, #7857, #4655, #14656, #39960, #1467, #40587, #7637 ),
 .UNSPECIFIED., .F., .F. ) 
 B_SPLINE_CURVE_WITH_KNOTS ( ( 3, 2, 2, 2, 3 ),
 ( 0.5270833333333333481, 0.5277777777777777901, 0.5291666666666666741, 0.5305555555555555580, 0.5312500000000000000 ),
 .UNSPECIFIED. ) 
 CURVE ( )  GEOMETRIC_REPRESENTATION_ITEM ( )  RATIONAL_B_SPLINE_CURVE ( ( 0.9330127018922194093, 0.9330127018922194093, 1.000000000000000000, 0.8660254037844387076, 1.000000000000000000, 0.8660254037844387076, 1.000000000000000000, 0.9330127018922194093, 0.9330127018922194093 ) ) 
 REPRESENTATION_ITEM ( '' )  );
#40762=ORIENTED_EDGE ( 'NONE', *, *, #35204, .T. ) ;
#40764=CARTESIAN_POINT ( 'NONE',  ( -1.394453263437886604E-15, 14.00000000000001066, -29.40473080337743284 ) ) ;
#40766=LINE ( 'NONE', #15036, #21313 ) ;
#40769=EDGE_CURVE ( 'NONE', #9113, #14819, #15475, .T. ) ;
#40770=ORIENTED_EDGE ( 'NONE', *, *, #872, .F. ) ;
#40771=CARTESIAN_POINT ( 'NONE',  ( -0.9378221735089308231, 21.00000000000002487, -143.1663226036829997 ) ) ;
#40772=CARTESIAN_POINT ( 'NONE',  ( 1.655278471874998436, 14.63297358603755072, -132.4307724695661364 ) ) ;
#40774=CARTESIAN_POINT ( 'NONE',  ( -1.394453263437886604E-15, 14.00000000000002132, -131.4047308033774186 ) ) ;
#40775=CARTESIAN_POINT ( 'NONE',  ( -7.022189441860112050E-16, 13.67729811471671475, -39.60160580289946353 ) ) ;
#40776=CARTESIAN_POINT ( 'NONE',  ( -1.655278471875002211, 14.63297358603754006, -34.68493913623279923 ) ) ;
#40777=EDGE_CURVE ( 'NONE', #41462, #30193, #21427, .T. ) ;
#40778=CARTESIAN_POINT ( 'NONE',  ( -7.022189441860112050E-16, 13.67729811471672363, -90.60160580289947063 ) ) ;
#40779=CARTESIAN_POINT ( 'NONE',  ( 2.340729813953370519E-16, 21.32270188528332255, -142.0141058028994792 ) ) ;
#40780=ORIENTED_EDGE ( 'NONE', *, *, #14712, .T. ) ;
#40782=CARTESIAN_POINT ( 'NONE',  ( 1.655278471874998436, 14.63297358603755249, -138.5182724695661420 ) ) ;
#40784=CARTESIAN_POINT ( 'NONE',  ( -1.750000000000002220, 14.46891108675448301, -94.79431413575484555 ) ) ;
#40785=CARTESIAN_POINT ( 'NONE',  ( -1.394453263437886604E-15, 14.00000000000001776, -87.40473080337743284 ) ) ;
#40786=CARTESIAN_POINT ( 'NONE',  ( 1.655278471875001101, 20.36702641396248836, -58.09743913623280065 ) ) ;
#40788=CARTESIAN_POINT ( 'NONE',  ( -7.424026671074350129E-16, 13.45854811567263631, -83.40473080337741862 ) ) ;
#40789=CARTESIAN_POINT ( 'NONE',  ( 3.310556943749999981, 15.58864905735836714, -71.43493913623278502 ) ) ;
#40791=CARTESIAN_POINT ( 'NONE',  ( 1.750000000000001110, 20.53108891324555429, -83.98806413671076143 ) ) ;
#40792=DIRECTION ( 'NONE',  ( -0.000000000000000000, 1.259100132267607459E-16, -1.000000000000000000 ) ) ;
#40793=CARTESIAN_POINT ( 'NONE',  ( 3.500000000000001776, 19.52072594216370760, -47.37764746908818125 ) ) ;
#40794=CARTESIAN_POINT ( 'NONE',  ( -1.655278471875002211, 14.63297358603755072, -121.5974391362328078 ) ) ;
#40795=FACE_OUTER_BOUND ( 'NONE', #25812, .T. ) ;
#40796=CARTESIAN_POINT ( 'NONE',  ( 3.500000000000001332, 19.52072594216371826, -103.3776474690881741 ) ) ;
#40797=ORIENTED_EDGE ( 'NONE', *, *, #4139, .F. ) ;
#40798=CARTESIAN_POINT ( 'NONE',  ( 3.500000000000000000, 15.47927405783632970, -114.2380641367107614 ) ) ;
#40800=CYLINDRICAL_SURFACE ( 'NONE', #22677, 3.499999999999999556 ) ;
#40804=CARTESIAN_POINT ( 'NONE',  ( 1.655278471875001101, 20.36702641396248836, -72.09743913623280775 ) ) ;
#40807=FACE_OUTER_BOUND ( 'NONE', #13663, .T. ) ;
#40808=ORIENTED_EDGE ( 'NONE', *, *, #2992, .F. ) ;
#40809=CARTESIAN_POINT ( 'NONE',  ( -3.310556943750002201, 15.58864905735836182, -23.68077246956613635 ) ) ;
#40810=EDGE_CURVE ( 'NONE', #1595, #19734, #26902, .T. ) ;
#40811=CARTESIAN_POINT ( 'NONE',  ( -0.9378221735089310451, 14.00000000000002309, -120.4493890021159643 ) ) ;
#40812=CARTESIAN_POINT ( 'NONE',  ( 1.655278471874998436, 14.63297358603754361, -79.43077246956615056 ) ) ;
#40815=( BOUNDED_CURVE ( )  B_SPLINE_CURVE ( 2, ( #10081, #29203, #19235, #26042, #79, #42002, #3072, #12851, #25833 ),
 .UNSPECIFIED., .F., .T. ) 
 B_SPLINE_CURVE_WITH_KNOTS ( ( 3, 2, 2, 2, 3 ),
 ( 0.8104166666666666741, 0.8111111111111111160, 0.8125000000000000000, 0.8138888888888888840, 0.8145833333333333259 ),
 .UNSPECIFIED. ) 
 CURVE ( )  GEOMETRIC_REPRESENTATION_ITEM ( )  RATIONAL_B_SPLINE_CURVE ( ( 0.9330127018922194093, 0.9330127018922194093, 1.000000000000000000, 0.8660254037844387076, 1.000000000000000000, 0.8660254037844387076, 1.000000000000000000, 0.9330127018922194093, 0.9330127018922194093 ) ) 
 REPRESENTATION_ITEM ( '' )  );
#40816=VECTOR ( 'NONE', #23943, 1000.000000000000000 ) ;
#40817=DIRECTION ( 'NONE',  ( -0.000000000000000000, 1.259100132267607459E-16, -1.000000000000000000 ) ) ;
#40820=CARTESIAN_POINT ( 'NONE',  ( 3.500000000000000000, 15.47927405783633503, -129.2380641367107614 ) ) ;
#40821=ORIENTED_EDGE ( 'NONE', *, *, #12348, .T. ) ;
#40822=DIRECTION ( 'NONE',  ( -0.000000000000000000, 1.259100132267607459E-16, -1.000000000000000000 ) ) ;
#40823=CARTESIAN_POINT ( 'NONE',  ( 2.340729813953370519E-16, 21.32270188528330834, -48.10160580289946353 ) ) ;
#40824=EDGE_CURVE ( 'NONE', #39330, #24198, #28501, .T. ) ;
#40825=CARTESIAN_POINT ( 'NONE',  ( -1.655278471875002211, 14.63297358603755072, -110.6849391362327992 ) ) ;
#40826=ORIENTED_EDGE ( 'NONE', *, *, #27235, .F. ) ;
#40827=CARTESIAN_POINT ( 'NONE',  ( -3.310556943750001313, 17.50000000000001066, -34.76410580289947205 ) ) ;
#40828=CARTESIAN_POINT ( 'NONE',  ( 3.310556943750001313, 19.41135094264166128, -62.26827246956614204 ) ) ;
#40829=CARTESIAN_POINT ( 'NONE',  ( 1.749999999999998224, 14.46891108675448478, -112.6276474690881884 ) ) ;
#40831=CARTESIAN_POINT ( 'NONE',  ( 1.655278471874998436, 14.63297358603754716, -98.43077246956613635 ) ) ;
#40832=FACE_OUTER_BOUND ( 'NONE', #38134, .T. ) ;
#40833=CARTESIAN_POINT ( 'NONE',  ( 4.648177544792955347E-16, 21.00000000000001421, -56.90473080337742573 ) ) ;
#40835=CARTESIAN_POINT ( 'NONE',  ( -3.500000000000001332, 17.50000000000001421, -65.96098080242150274 ) ) ;
#40837=CARTESIAN_POINT ( 'NONE',  ( -3.310556943750001313, 17.50000000000001066, -33.76410580289947205 ) ) ;
#40838=CARTESIAN_POINT ( 'NONE',  ( 3.500000000000000000, 15.47927405783632260, -55.23806413671077564 ) ) ;
#40839=CYLINDRICAL_SURFACE ( 'NONE', #16516, 3.499999999999999556 ) ;
#40840=CARTESIAN_POINT ( 'NONE',  ( -3.310556943750000425, 19.41135094264166838, -108.9349391362327992 ) ) ;
#40841=CARTESIAN_POINT ( 'NONE',  ( -3.310556943750002201, 15.58864905735836537, -39.76827246956612072 ) ) ;
#40847=LINE ( 'NONE', #25111, #10935 ) ;
#40849=CARTESIAN_POINT ( 'NONE',  ( -3.310556943750001313, 17.50000000000001776, -88.76410580289947916 ) ) ;
#40852=ORIENTED_EDGE ( 'NONE', *, *, #12052, .F. ) ;
#40854=CARTESIAN_POINT ( 'NONE',  ( 1.749999999999998224, 14.46891108675448656, -133.3213974700441042 ) ) ;
#40860=CARTESIAN_POINT ( 'NONE',  ( 4.648177544792955347E-16, 21.00000000000001776, -78.90473080337741862 ) ) ;
#40861=ORIENTED_EDGE ( 'NONE', *, *, #39950, .T. ) ;
#40868=EDGE_CURVE ( 'NONE', #16644, #37791, #6462, .T. ) ;
#40872=CARTESIAN_POINT ( 'NONE',  ( 2.340729813953370519E-16, 21.32270188528332255, -138.0141058028994507 ) ) ;
#40873=CARTESIAN_POINT ( 'NONE',  ( 0.9378221735089300459, 21.00000000000002487, -133.2556390011600342 ) ) ;
#40875=CARTESIAN_POINT ( 'NONE',  ( -0.9378221735089291577, 21.00000000000001421, -63.86007260463891555 ) ) ;
#40876=CARTESIAN_POINT ( 'NONE',  ( 3.310556943749999981, 15.58864905735837425, -124.4349391362327992 ) ) ;
#40877=CARTESIAN_POINT ( 'NONE',  ( -7.022189441860112050E-16, 13.67729811471671830, -55.60160580289947063 ) ) ;
#40878=ORIENTED_EDGE ( 'NONE', *, *, #19979, .F. ) ;
#40880=CARTESIAN_POINT ( 'NONE',  ( 3.500000000000000000, 15.47927405783633503, -138.2380641367107614 ) ) ;
#40882=CARTESIAN_POINT ( 'NONE',  ( 2.340729813953370519E-16, 21.32270188528331190, -84.10160580289945642 ) ) ;
#40883=CARTESIAN_POINT ( 'NONE',  ( -3.500000000000001332, 17.50000000000002487, -129.9609808024214885 ) ) ;
#40884=CARTESIAN_POINT ( 'NONE',  ( -3.310556943750002645, 15.58864905735837780, -114.6807724695661364 ) ) ;
#40889=CARTESIAN_POINT ( 'NONE',  ( 3.500000000000001776, 19.52072594216371115, -80.37764746908818836 ) ) ;
#40891=CARTESIAN_POINT ( 'NONE',  ( -1.655278471875002211, 14.63297358603754184, -47.59743913623280775 ) ) ;
#40892=CARTESIAN_POINT ( 'NONE',  ( 1.655278471874998436, 14.63297358603754716, -108.5182724695661420 ) ) ;
#40893=CARTESIAN_POINT ( 'NONE',  ( -0.9378221735089291577, 21.00000000000002487, -130.8600726046389013 ) ) ;
#40895=CARTESIAN_POINT ( 'NONE',  ( 4.286263797015737581E-16, 14.00000000000002487, -149.5231586289125687 ) ) ;
#40896=CARTESIAN_POINT ( 'NONE',  ( 3.310556943750001313, 17.50000000000002132, -124.3516058028994564 ) ) ;
#40899=CARTESIAN_POINT ( 'NONE',  ( -3.500000000000002220, 15.47927405783633326, -100.8776474690881599 ) ) ;
#40900=CARTESIAN_POINT ( 'NONE',  ( -1.655278471875002211, 14.63297358603754361, -59.68493913623279212 ) ) ;
#40903=CARTESIAN_POINT ( 'NONE',  ( 3.310556943750001313, 17.50000000000001421, -73.35160580289947063 ) ) ;
#40904=CARTESIAN_POINT ( 'NONE',  ( 0.000000000000000000, 17.50000000000002487, -149.5231586289125687 ) ) ;
#40906=DIRECTION ( 'NONE',  ( -0.000000000000000000, 1.259100132267607459E-16, -1.000000000000000000 ) ) ;
#40909=CARTESIAN_POINT ( 'NONE',  ( 1.655278471875001101, 20.36702641396248481, -41.09743913623280065 ) ) ;
#40911=EDGE_LOOP ( 'NONE', ( #34851, #14039, #25397, #15771 ) ) ;
#40917=CARTESIAN_POINT ( 'NONE',  ( -3.310556943750001313, 17.50000000000001066, -46.76410580289947205 ) ) ;
#40921=ORIENTED_EDGE ( 'NONE', *, *, #41666, .T. ) ;
#40923=FACE_OUTER_BOUND ( 'NONE', #27807, .T. ) ;
#40925=CARTESIAN_POINT ( 'NONE',  ( 0.9378221735089281585, 14.00000000000002132, -113.3600726046389155 ) ) ;
#40926=FACE_OUTER_BOUND ( 'NONE', #17838, .T. ) ;
#40927=CARTESIAN_POINT ( 'NONE',  ( 2.474675557024783212E-16, 21.54145188432739033, -37.21098080242150985 ) ) ;
#40929=CARTESIAN_POINT ( 'NONE',  ( -1.750000000000002220, 14.46891108675448123, -76.79431413575484555 ) ) ;
#40930=( BOUNDED_CURVE ( )  B_SPLINE_CURVE ( 2, ( #36968, #30990, #17807, #1438, #27594, #21203, #33771, #40562, #1847 ),
 .UNSPECIFIED., .F., .T. ) 
 B_SPLINE_CURVE_WITH_KNOTS ( ( 3, 2, 2, 2, 3 ),
 ( 0.1020833333333333315, 0.1027777777777777735, 0.1041666666666666713, 0.1055555555555555552, 0.1062499999999999972 ),
 .UNSPECIFIED. ) 
 CURVE ( )  GEOMETRIC_REPRESENTATION_ITEM ( )  RATIONAL_B_SPLINE_CURVE ( ( 0.9330127018922194093, 0.9330127018922194093, 1.000000000000000000, 0.8660254037844387076, 1.000000000000000000, 0.8660254037844387076, 1.000000000000000000, 0.9330127018922194093, 0.9330127018922194093 ) ) 
 REPRESENTATION_ITEM ( '' )  );
#40931=( BOUNDED_CURVE ( )  B_SPLINE_CURVE ( 2, ( #23725, #1175, #30303, #16915, #14143, #1381, #20743, #14357, #7340 ),
 .UNSPECIFIED., .F., .T. ) 
 B_SPLINE_CURVE_WITH_KNOTS ( ( 3, 2, 2, 2, 3 ),
 ( 0.4270833333333333148, 0.4277777777777777568, 0.4291666666666666408, 0.4305555555555555802, 0.4312500000000000222 ),
 .UNSPECIFIED. ) 
 CURVE ( )  GEOMETRIC_REPRESENTATION_ITEM ( )  RATIONAL_B_SPLINE_CURVE ( ( 0.9330127018922194093, 0.9330127018922194093, 1.000000000000000000, 0.8660254037844387076, 1.000000000000000000, 0.8660254037844387076, 1.000000000000000000, 0.9330127018922194093, 0.9330127018922194093 ) ) 
 REPRESENTATION_ITEM ( '' )  );
#40934=CARTESIAN_POINT ( 'NONE',  ( -3.500000000000002220, 15.47927405783633503, -142.8776474690881741 ) ) ;
#40936=CARTESIAN_POINT ( 'NONE',  ( 1.655278471875001101, 20.36702641396249547, -128.0974391362328220 ) ) ;
#40940=CARTESIAN_POINT ( 'NONE',  ( 0.000000000000000000, 17.49999999999998934, 153.5815388724490163 ) ) ;
#40941=CARTESIAN_POINT ( 'NONE',  ( -7.022189441860112050E-16, 13.67729811471672718, -120.6016058028994564 ) ) ;
#40943=CARTESIAN_POINT ( 'NONE',  ( 4.648177544792955347E-16, 21.00000000000002487, -140.9047308033773902 ) ) ;
#40944=CARTESIAN_POINT ( 'NONE',  ( -3.500000000000002220, 15.47927405783632082, -38.57139747004409003 ) ) ;
#40948=CARTESIAN_POINT ( 'NONE',  ( -7.022189441860112050E-16, 13.67729811471673074, -140.6016058028994564 ) ) ;
#40951=CARTESIAN_POINT ( 'NONE',  ( -3.310556943750001313, 17.50000000000001421, -47.85160580289946353 ) ) ;
#40953=CARTESIAN_POINT ( 'NONE',  ( -1.394453263437886604E-15, 14.00000000000002132, -114.4047308033774186 ) ) ;
#40955=CARTESIAN_POINT ( 'NONE',  ( 3.310556943750001313, 19.41135094264166483, -76.26827246956612782 ) ) ;
#40957=CARTESIAN_POINT ( 'NONE',  ( 3.310556943750001313, 19.41135094264166838, -105.1807724695661364 ) ) ;
#40958=CARTESIAN_POINT ( 'NONE',  ( -1.655278471875002211, 14.63297358603754539, -69.59743913623280775 ) ) ;
#40960=CARTESIAN_POINT ( 'NONE',  ( -1.655278471875002211, 14.63297358603754716, -88.68493913623279923 ) ) ;
#40962=CARTESIAN_POINT ( 'NONE',  ( 1.749999999999998224, 14.46891108675447768, -67.62764746908817415 ) ) ;
#40965=CARTESIAN_POINT ( 'NONE',  ( 3.310556943750001313, 17.50000000000001421, -57.26410580289947916 ) ) ;
#40966=CARTESIAN_POINT ( 'NONE',  ( -3.500000000000000000, 19.52072594216370405, -24.73806413671077209 ) ) ;
#40967=CARTESIAN_POINT ( 'NONE',  ( -1.655278471874999990, 20.36702641396249547, -111.9307724695661506 ) ) ;
#40972=ORIENTED_EDGE ( 'NONE', *, *, #18391, .F. ) ;
#40974=CARTESIAN_POINT ( 'NONE',  ( 3.310556943749999981, 15.58864905735836537, -65.34743913623282197 ) ) ;
#40976=VERTEX_POINT ( 'NONE', #37276 ) ;
#40977=ADVANCED_FACE ( 'NONE', ( #18328 ), #4937, .T. ) ;
#40978=EDGE_LOOP ( 'NONE', ( #7230, #41346, #20625, #34954 ) ) ;
#40980=LINE ( 'NONE', #34592, #39644 ) ;
#40986=CARTESIAN_POINT ( 'NONE',  ( 0.000000000000000000, 17.50000000000002487, -149.5231586289125687 ) ) ;
#40987=AXIS2_PLACEMENT_3D ( 'NONE', #41021, #12076, #2305 ) ;
#40988=CARTESIAN_POINT ( 'NONE',  ( -1.655278471875002211, 14.63297358603755249, -132.5974391362328220 ) ) ;
#40989=CARTESIAN_POINT ( 'NONE',  ( -1.749999999999999778, 20.53108891324555785, -128.8213974700441042 ) ) ;
#40990=CARTESIAN_POINT ( 'NONE',  ( 3.310556943750001313, 19.41135094264165772, -42.26827246956612782 ) ) ;
#40991=CARTESIAN_POINT ( 'NONE',  ( -3.310556943750000425, 19.41135094264165772, -34.93493913623279923 ) ) ;
#40992=CARTESIAN_POINT ( 'NONE',  ( -3.310556943750000425, 19.41135094264166483, -92.93493913623281344 ) ) ;
#40993=CARTESIAN_POINT ( 'NONE',  ( 2.474675557024783212E-16, 21.54145188432739033, -25.90473080337743284 ) ) ;
#40994=ORIENTED_EDGE ( 'NONE', *, *, #29730, .T. ) ;
#40996=CARTESIAN_POINT ( 'NONE',  ( -7.022189441860112050E-16, 13.67729811471672896, -136.6016058028994564 ) ) ;
#40999=CARTESIAN_POINT ( 'NONE',  ( -3.310556943750001313, 17.50000000000001421, -57.76410580289947916 ) ) ;
#41000=CARTESIAN_POINT ( 'NONE',  ( 0.9378221735089300459, 21.00000000000001776, -94.94938900211595012 ) ) ;
#41001=CARTESIAN_POINT ( 'NONE',  ( -3.500000000000000888, 19.52072594216371115, -84.73806413671074722 ) ) ;
#41002=CARTESIAN_POINT ( 'NONE',  ( -3.310556943750000425, 19.41135094264166483, -65.93493913623279923 ) ) ;
#41005=LINE ( 'NONE', #12494, #263 ) ;
#41006=CARTESIAN_POINT ( 'NONE',  ( -0.9378221735089310451, 14.00000000000001066, -47.75563900116002714 ) ) ;
#41007=CARTESIAN_POINT ( 'NONE',  ( -7.022189441860112050E-16, 13.67729811471672896, -118.5141058028994792 ) ) ;
#41011=ORIENTED_EDGE ( 'NONE', *, *, #25856, .T. ) ;
#41012=CARTESIAN_POINT ( 'NONE',  ( 1.749999999999998224, 14.46891108675448478, -111.3213974700441042 ) ) ;
#41013=CARTESIAN_POINT ( 'NONE',  ( -0.9378221735089310451, 14.00000000000001066, -28.44938900211594657 ) ) ;
#41015=EDGE_CURVE ( 'NONE', #36364, #31756, #22794, .T. ) ;
#41016=CARTESIAN_POINT ( 'NONE',  ( -1.394453263437886604E-15, 14.00000000000001421, -61.40473080337742573 ) ) ;
#41019=CARTESIAN_POINT ( 'NONE',  ( 3.310556943749999981, 15.58864905735836714, -69.34743913623280775 ) ) ;
#41020=( BOUNDED_CURVE ( )  B_SPLINE_CURVE ( 2, ( #270, #35996, #38781, #29615, #39393, #6862, #38988, #32191, #12833 ),
 .UNSPECIFIED., .F., .F. ) 
 B_SPLINE_CURVE_WITH_KNOTS ( ( 3, 2, 2, 2, 3 ),
 ( 0.9312500000000000222, 0.9319444444444444642, 0.9333333333333333481, 0.9347222222222222321, 0.9354166666666666741 ),
 .UNSPECIFIED. ) 
 CURVE ( )  GEOMETRIC_REPRESENTATION_ITEM ( )  RATIONAL_B_SPLINE_CURVE ( ( 0.9330127018922194093, 0.9330127018922194093, 1.000000000000000000, 0.8660254037844387076, 1.000000000000000000, 0.8660254037844387076, 1.000000000000000000, 0.9330127018922194093, 0.9330127018922194093 ) ) 
 REPRESENTATION_ITEM ( '' )  );
#41021=CARTESIAN_POINT ( 'NONE',  ( 0.000000000000000000, 17.50000000000002487, -149.5231586289125687 ) ) ;
#41022=ORIENTED_EDGE ( 'NONE', *, *, #37714, .T. ) ;
#41024=CARTESIAN_POINT ( 'NONE',  ( 3.310556943750001313, 19.41135094264166128, -26.18077246956613990 ) ) ;
#41027=CARTESIAN_POINT ( 'NONE',  ( -3.310556943750001313, 17.50000000000001776, -81.76410580289947916 ) ) ;
#41028=ORIENTED_EDGE ( 'NONE', *, *, #33113, .T. ) ;
#41029=ORIENTED_EDGE ( 'NONE', *, *, #31160, .F. ) ;
#41030=CARTESIAN_POINT ( 'NONE',  ( 0.000000000000000000, 17.50000000000002487, -149.5231586289125687 ) ) ;
#41031=EDGE_CURVE ( 'NONE', #3992, #31346, #25783, .T. ) ;
#41036=CARTESIAN_POINT ( 'NONE',  ( 3.310556943750001313, 19.41135094264166128, -47.26827246956614204 ) ) ;
#41037=CARTESIAN_POINT ( 'NONE',  ( -1.655278471875002211, 14.63297358603755072, -109.6849391362327992 ) ) ;
#41039=CARTESIAN_POINT ( 'NONE',  ( -1.655278471874999990, 20.36702641396248481, -31.93077246956614701 ) ) ;
#41041=CARTESIAN_POINT ( 'NONE',  ( 2.340729813953370519E-16, 21.32270188528330834, -59.10160580289947063 ) ) ;
#41042=CARTESIAN_POINT ( 'NONE',  ( -1.750000000000002220, 14.46891108675448656, -112.7943141357548456 ) ) ;
#41044=CARTESIAN_POINT ( 'NONE',  ( 3.310556943750001313, 19.41135094264166483, -96.18077246956612214 ) ) ;
#41045=CARTESIAN_POINT ( 'NONE',  ( 4.648177544792955347E-16, 21.00000000000001421, -47.21098080242149564 ) ) ;
#41048=CARTESIAN_POINT ( 'NONE',  ( -3.500000000000001332, 17.50000000000001421, -66.96098080242150274 ) ) ;
#41050=CARTESIAN_POINT ( 'NONE',  ( -3.310556943750001313, 17.50000000000001066, -26.76410580289947916 ) ) ;
#41051=CARTESIAN_POINT ( 'NONE',  ( 3.500000000000000000, 15.47927405783632082, -52.23806413671078275 ) ) ;
#41052=CARTESIAN_POINT ( 'NONE',  ( 4.648177544792955347E-16, 21.00000000000001776, -77.21098080242148853 ) ) ;
#41053=CARTESIAN_POINT ( 'NONE',  ( -1.655278471874999990, 20.36702641396249547, -106.0182724695661278 ) ) ;
#41054=EDGE_CURVE ( 'NONE', #28716, #33169, #16833, .T. ) ;
#41055=CARTESIAN_POINT ( 'NONE',  ( -3.310556943750000425, 19.41135094264166128, -38.93493913623280633 ) ) ;
#41060=FACE_OUTER_BOUND ( 'NONE', #35267, .T. ) ;
#41062=CARTESIAN_POINT ( 'NONE',  ( 3.310556943749999981, 15.58864905735836892, -85.34743913623279354 ) ) ;
#41063=CARTESIAN_POINT ( 'NONE',  ( 1.743066579297357930E-14, 14.00000000000002132, -135.4047308033774186 ) ) ;
#41067=( BOUNDED_CURVE ( )  B_SPLINE_CURVE ( 2, ( #45, #8990, #21963, #16025, #9202, #35148, #34937, #18781, #31739 ),
 .UNSPECIFIED., .F., .T. ) 
 B_SPLINE_CURVE_WITH_KNOTS ( ( 3, 2, 2, 2, 3 ),
 ( 0.6687499999999999556, 0.6694444444444443976, 0.6708333333333332815, 0.6722222222222222765, 0.6729166666666667185 ),
 .UNSPECIFIED. ) 
 CURVE ( )  GEOMETRIC_REPRESENTATION_ITEM ( )  RATIONAL_B_SPLINE_CURVE ( ( 0.9330127018922194093, 0.9330127018922194093, 1.000000000000000000, 0.8660254037844387076, 1.000000000000000000, 0.8660254037844387076, 1.000000000000000000, 0.9330127018922194093, 0.9330127018922194093 ) ) 
 REPRESENTATION_ITEM ( '' )  );
#41068=CARTESIAN_POINT ( 'NONE',  ( -1.749999999999999778, 20.53108891324555074, -50.82139747004409003 ) ) ;
#41069=AXIS2_PLACEMENT_3D ( 'NONE', #10635, #33810, #14040 ) ;
#41073=EDGE_CURVE ( 'NONE', #30668, #1116, #31240, .T. ) ;
#41077=CARTESIAN_POINT ( 'NONE',  ( 3.500000000000000000, 15.47927405783633326, -121.2380641367107756 ) ) ;
#41078=EDGE_LOOP ( 'NONE', ( #8774, #37522, #945, #42040 ) ) ;
#41083=FACE_OUTER_BOUND ( 'NONE', #37014, .T. ) ;
#41087=FACE_OUTER_BOUND ( 'NONE', #32348, .T. ) ;
#41089=CARTESIAN_POINT ( 'NONE',  ( 1.655278471874998436, 14.63297358603755249, -137.4307724695661364 ) ) ;
#41090=CARTESIAN_POINT ( 'NONE',  ( 3.500000000000000000, 15.47927405783632082, -38.23806413671076854 ) ) ;
#41092=CARTESIAN_POINT ( 'NONE',  ( 0.9378221735089300459, 21.00000000000001421, -54.25563900116004135 ) ) ;
#41093=CARTESIAN_POINT ( 'NONE',  ( 3.310556943749999981, 15.58864905735837425, -123.4349391362327992 ) ) ;
#41094=CARTESIAN_POINT ( 'NONE',  ( 1.655278471875001101, 20.36702641396248836, -55.18493913623280633 ) ) ;
#41097=CARTESIAN_POINT ( 'NONE',  ( 3.500000000000001776, 19.52072594216372181, -137.0713974700440758 ) ) ;
#41098=AXIS2_PLACEMENT_3D ( 'NONE', #42105, #25520, #12958 ) ;
#41100=CARTESIAN_POINT ( 'NONE',  ( -3.310556943750001313, 17.50000000000001776, -74.85160580289947063 ) ) ;
#41101=CARTESIAN_POINT ( 'NONE',  ( -1.750000000000002220, 14.46891108675448834, -130.7943141357548598 ) ) ;
#41103=CARTESIAN_POINT ( 'NONE',  ( 2.340729813953370519E-16, 21.32270188528331900, -113.0141058028994649 ) ) ;
#41106=EDGE_CURVE ( 'NONE', #5149, #6296, #39941, .T. ) ;
#41108=CARTESIAN_POINT ( 'NONE',  ( -3.500000000000002220, 15.47927405783632615, -77.87764746908817415 ) ) ;
#41109=CARTESIAN_POINT ( 'NONE',  ( -1.394453263437886604E-15, 14.00000000000001776, -103.4047308033774186 ) ) ;
#41110=CARTESIAN_POINT ( 'NONE',  ( 2.340729813953370519E-16, 21.32270188528330834, -49.01410580289947205 ) ) ;
#41111=CARTESIAN_POINT ( 'NONE',  ( -1.655278471874999990, 20.36702641396249547, -103.0182724695661278 ) ) ;
#41113=CARTESIAN_POINT ( 'NONE',  ( -1.394453263437886604E-15, 14.00000000000001066, -39.71098080242150985 ) ) ;
#41116=CARTESIAN_POINT ( 'NONE',  ( 1.655278471874998436, 14.63297358603755072, -123.5182724695661278 ) ) ;
#41120=CARTESIAN_POINT ( 'NONE',  ( 3.500000000000001332, 17.50000000000001066, -32.15473080337742573 ) ) ;
#41121=FACE_OUTER_BOUND ( 'NONE', #17855, .T. ) ;
#41122=ORIENTED_EDGE ( 'NONE', *, *, #25133, .T. ) ;
#41124=ORIENTED_EDGE ( 'NONE', *, *, #2216, .T. ) ;
#41125=CARTESIAN_POINT ( 'NONE',  ( -1.655278471875002211, 14.63297358603754539, -77.68493913623279923 ) ) ;
#41126=DIRECTION ( 'NONE',  ( 0.000000000000000000, 1.000000000000000000, 0.000000000000000000 ) ) ;
#41133=CARTESIAN_POINT ( 'NONE',  ( 1.655278471874998436, 14.63297358603753828, -39.43077246956613635 ) ) ;
#41138=CARTESIAN_POINT ( 'NONE',  ( -3.310556943750001313, 17.50000000000001421, -47.76410580289947205 ) ) ;
#41139=( BOUNDED_CURVE ( )  B_SPLINE_CURVE ( 2, ( #35158, #19207, #25807, #25182, #35581, #34739, #32180, #28563, #6445 ),
 .UNSPECIFIED., .F., .T. ) 
 B_SPLINE_CURVE_WITH_KNOTS ( ( 3, 2, 2, 2, 3 ),
 ( 0.2979166666666666630, 0.2986111111111111049, 0.2999999999999999889, 0.3013888888888888729, 0.3020833333333333148 ),
 .UNSPECIFIED. ) 
 CURVE ( )  GEOMETRIC_REPRESENTATION_ITEM ( )  RATIONAL_B_SPLINE_CURVE ( ( 0.9330127018922194093, 0.9330127018922194093, 1.000000000000000000, 0.8660254037844387076, 1.000000000000000000, 0.8660254037844387076, 1.000000000000000000, 0.9330127018922194093, 0.9330127018922194093 ) ) 
 REPRESENTATION_ITEM ( '' )  );
#41141=ORIENTED_EDGE ( 'NONE', *, *, #30349, .T. ) ;
#41143=CARTESIAN_POINT ( 'NONE',  ( -3.500000000000001332, 17.50000000000001066, -24.96098080242151340 ) ) ;
#41145=CARTESIAN_POINT ( 'NONE',  ( 1.750000000000001110, 20.53108891324555785, -112.9880641367107614 ) ) ;
#41146=VECTOR ( 'NONE', #35042, 1000.000000000000000 ) ;
#41147=CYLINDRICAL_SURFACE ( 'NONE', #4414, 3.499999999999999556 ) ;
#41148=CARTESIAN_POINT ( 'NONE',  ( 3.500000000000001776, 19.52072594216370405, -39.37764746908817415 ) ) ;
#41149=CARTESIAN_POINT ( 'NONE',  ( 1.749999999999998224, 14.46891108675448123, -86.62764746908817415 ) ) ;
#41150=ORIENTED_EDGE ( 'NONE', *, *, #5304, .F. ) ;
#41151=CARTESIAN_POINT ( 'NONE',  ( 0.9378221735089281585, 14.00000000000001599, -70.66632260368299967 ) ) ;
#41152=CARTESIAN_POINT ( 'NONE',  ( 4.286263797015737581E-16, 14.00000000000002487, -149.5231586289125687 ) ) ;
#41154=CARTESIAN_POINT ( 'NONE',  ( -3.310556943750001313, 17.50000000000001066, -24.85160580289946708 ) ) ;
#41155=CARTESIAN_POINT ( 'NONE',  ( -3.500000000000000000, 19.52072594216371115, -100.7380641367107756 ) ) ;
#41156=CARTESIAN_POINT ( 'NONE',  ( -3.310556943750002645, 15.58864905735837780, -127.6807724695661364 ) ) ;
#41159=CARTESIAN_POINT ( 'NONE',  ( -1.394453263437886604E-15, 14.00000000000001066, -29.40473080337743284 ) ) ;
#41160=CARTESIAN_POINT ( 'NONE',  ( -3.310556943750000425, 19.41135094264166838, -120.9349391362327992 ) ) ;
#41161=CYLINDRICAL_SURFACE ( 'NONE', #28868, 3.499999999999999556 ) ;
#41162=CARTESIAN_POINT ( 'NONE',  ( 1.750000000000001110, 20.53108891324554719, -35.98806413671076854 ) ) ;
#41163=CARTESIAN_POINT ( 'NONE',  ( 0.9378221735089281585, 14.00000000000002132, -115.3600726046389155 ) ) ;
#41165=CARTESIAN_POINT ( 'NONE',  ( -1.655278471874999990, 20.36702641396249902, -139.0182724695661420 ) ) ;
#41166=CARTESIAN_POINT ( 'NONE',  ( 1.750000000000001110, 20.53108891324554719, -29.29431413575483845 ) ) ;
#41167=EDGE_CURVE ( 'NONE', #23350, #18376, #19562, .T. ) ;
#41168=CARTESIAN_POINT ( 'NONE',  ( 1.655278471875001101, 20.36702641396248836, -48.18493913623279923 ) ) ;
#41170=CARTESIAN_POINT ( 'NONE',  ( 1.750000000000001110, 20.53108891324555785, -104.2943141357548456 ) ) ;
#41171=CARTESIAN_POINT ( 'NONE',  ( -1.655278471875002211, 14.63297358603754539, -72.68493913623279923 ) ) ;
#41173=CARTESIAN_POINT ( 'NONE',  ( 3.310556943750001313, 19.41135094264166838, -98.18077246956613635 ) ) ;
#41174=CARTESIAN_POINT ( 'NONE',  ( -3.310556943750000425, 19.41135094264166128, -69.84743913623280775 ) ) ;
#41175=ORIENTED_EDGE ( 'NONE', *, *, #18764, .T. ) ;
#41176=CARTESIAN_POINT ( 'NONE',  ( 1.655278471875001101, 20.36702641396249192, -93.18493913623279923 ) ) ;
#41177=AXIS2_PLACEMENT_3D ( 'NONE', #12831, #25815, #9650 ) ;
#41179=CARTESIAN_POINT ( 'NONE',  ( -1.394453263437886604E-15, 14.00000000000002132, -113.7109808024214885 ) ) ;
#41180=CARTESIAN_POINT ( 'NONE',  ( -3.500000000000000000, 19.52072594216371115, -85.04431413575483134 ) ) ;
#41182=CARTESIAN_POINT ( 'NONE',  ( 1.655278471874998436, 14.63297358603754184, -55.43077246956613635 ) ) ;
#41183=CARTESIAN_POINT ( 'NONE',  ( -1.750000000000002220, 14.46891108675449011, -137.4880641367107614 ) ) ;
#41184=CARTESIAN_POINT ( 'NONE',  ( -7.022189441860112050E-16, 13.67729811471672718, -109.5141058028994792 ) ) ;
#41185=CARTESIAN_POINT ( 'NONE',  ( -3.500000000000000000, 19.52072594216371115, -101.7380641367107756 ) ) ;
#41186=ORIENTED_EDGE ( 'NONE', *, *, #11891, .T. ) ;
#41187=ORIENTED_EDGE ( 'NONE', *, *, #3512, .F. ) ;
#41191=CARTESIAN_POINT ( 'NONE',  ( -1.655278471875002211, 14.63297358603754361, -65.59743913623280775 ) ) ;
#41195=( BOUNDED_CURVE ( )  B_SPLINE_CURVE ( 2, ( #20001, #20426, #32966, #16811, #33390, #637, #20212, #33174, #4256 ),
 .UNSPECIFIED., .F., .T. ) 
 B_SPLINE_CURVE_WITH_KNOTS ( ( 3, 2, 2, 2, 3 ),
 ( 0.2312500000000000111, 0.2319444444444444531, 0.2333333333333333370, 0.2347222222222222210, 0.2354166666666666630 ),
 .UNSPECIFIED. ) 
 CURVE ( )  GEOMETRIC_REPRESENTATION_ITEM ( )  RATIONAL_B_SPLINE_CURVE ( ( 0.9330127018922194093, 0.9330127018922194093, 1.000000000000000000, 0.8660254037844387076, 1.000000000000000000, 0.8660254037844387076, 1.000000000000000000, 0.9330127018922194093, 0.9330127018922194093 ) ) 
 REPRESENTATION_ITEM ( '' )  );
#41198=EDGE_CURVE ( 'NONE', #12728, #9113, #18447, .T. ) ;
#41200=LINE ( 'NONE', #41407, #41457 ) ;
#41201=ORIENTED_EDGE ( 'NONE', *, *, #41811, .T. ) ;
#41203=CARTESIAN_POINT ( 'NONE',  ( -7.022189441860112050E-16, 13.67729811471672896, -131.5141058028994507 ) ) ;
#41204=CARTESIAN_POINT ( 'NONE',  ( -1.750000000000002220, 14.46891108675448834, -128.4880641367107614 ) ) ;
#41205=VECTOR ( 'NONE', #26762, 1000.000000000000000 ) ;
#41206=CARTESIAN_POINT ( 'NONE',  ( 1.655278471875001101, 20.36702641396248481, -42.18493913623279212 ) ) ;
#41207=CARTESIAN_POINT ( 'NONE',  ( 2.340729813953370519E-16, 21.32270188528330479, -33.10160580289945642 ) ) ;
#41208=CARTESIAN_POINT ( 'NONE',  ( -1.655278471874999990, 20.36702641396249192, -92.01827246956611361 ) ) ;
#41209=CARTESIAN_POINT ( 'NONE',  ( 3.310556943750001313, 19.41135094264167549, -143.1807724695661364 ) ) ;
#41212=CARTESIAN_POINT ( 'NONE',  ( -1.655278471874999990, 20.36702641396249902, -138.0182724695661420 ) ) ;
#41213=CARTESIAN_POINT ( 'NONE',  ( -3.500000000000000000, 19.52072594216371115, -84.04431413575483134 ) ) ;
#41214=CARTESIAN_POINT ( 'NONE',  ( 1.750000000000001110, 20.53108891324555429, -86.98806413671076143 ) ) ;
#41215=CARTESIAN_POINT ( 'NONE',  ( 0.9378221735089630196, 14.00000000000003730, -95.36007260463891555 ) ) ;
#41217=CARTESIAN_POINT ( 'NONE',  ( 2.474675557024783212E-16, 21.54145188432739744, -78.90473080337743284 ) ) ;
#41219=CARTESIAN_POINT ( 'NONE',  ( -3.500000000000000000, 19.52072594216371826, -137.0443141357548598 ) ) ;
#41220=CARTESIAN_POINT ( 'NONE',  ( 1.749999999999998224, 14.46891108675447590, -47.62764746908818125 ) ) ;
#41221=CARTESIAN_POINT ( 'NONE',  ( -1.749999999999999778, 20.53108891324555074, -60.12764746908817415 ) ) ;
#41222=CARTESIAN_POINT ( 'NONE',  ( 3.310556943750001313, 17.50000000000002132, -121.2641058028994792 ) ) ;
#41223=CARTESIAN_POINT ( 'NONE',  ( -1.394453263437886604E-15, 14.00000000000001066, -39.71098080242150985 ) ) ;
#41224=CARTESIAN_POINT ( 'NONE',  ( 1.750000000000001110, 20.53108891324555074, -61.98806413671076143 ) ) ;
#41225=ORIENTED_EDGE ( 'NONE', *, *, #30557, .T. ) ;
#41227=CARTESIAN_POINT ( 'NONE',  ( -3.500000000000001332, 17.50000000000002132, -107.6547308033774186 ) ) ;
#41233=CARTESIAN_POINT ( 'NONE',  ( -3.310556943750001313, 17.50000000000001421, -71.76410580289947916 ) ) ;
#41234=CYLINDRICAL_SURFACE ( 'NONE', #40987, 3.499999999999999556 ) ;
#41235=CARTESIAN_POINT ( 'NONE',  ( 3.500000000000000000, 15.47927405783632082, -46.54431413575483845 ) ) ;
#41237=VERTEX_POINT ( 'NONE', #27640 ) ;
#41238=LINE ( 'NONE', #11663, #2202 ) ;
#41239=DIRECTION ( 'NONE',  ( -0.000000000000000000, 1.259100132267607459E-16, -1.000000000000000000 ) ) ;
#41240=CARTESIAN_POINT ( 'NONE',  ( -3.310556943750000425, 19.41135094264166483, -80.84743913623280775 ) ) ;
#41241=VERTEX_POINT ( 'NONE', #14877 ) ;
#41243=CARTESIAN_POINT ( 'NONE',  ( -7.460324959392693302E-14, 21.00000000000002132, -102.9047308033774044 ) ) ;
#41245=DIRECTION ( 'NONE',  ( -0.000000000000000000, 1.259100132267607459E-16, -1.000000000000000000 ) ) ;
#41246=EDGE_CURVE ( 'NONE', #29810, #32548, #40610, .T. ) ;
#41248=CARTESIAN_POINT ( 'NONE',  ( -3.310556943750002645, 15.58864905735836714, -48.76827246956614204 ) ) ;
#41249=CARTESIAN_POINT ( 'NONE',  ( -7.022189441860112050E-16, 13.67729811471672541, -107.6016058028994706 ) ) ;
#41250=ORIENTED_EDGE ( 'NONE', *, *, #26378, .T. ) ;
#41251=CARTESIAN_POINT ( 'NONE',  ( -3.310556943750002645, 15.58864905735836537, -34.68077246956615056 ) ) ;
#41252=CARTESIAN_POINT ( 'NONE',  ( 3.310556943749999981, 15.58864905735836537, -61.43493913623279212 ) ) ;
#41253=CARTESIAN_POINT ( 'NONE',  ( -3.500000000000000888, 19.52072594216371826, -107.0443141357548456 ) ) ;
#41255=CARTESIAN_POINT ( 'NONE',  ( 3.310556943750001313, 19.41135094264166483, -90.18077246956615056 ) ) ;
#41256=CARTESIAN_POINT ( 'NONE',  ( -3.500000000000002220, 15.47927405783632970, -97.57139747004410424 ) ) ;
#41257=ADVANCED_FACE ( 'NONE', ( #5299 ), #33821, .T. ) ;
#41258=DIRECTION ( 'NONE',  ( 0.000000000000000000, -0.4999999999999998890, 0.8660254037844385966 ) ) ;
#41259=CARTESIAN_POINT ( 'NONE',  ( 0.9378221735089300459, 21.00000000000001776, -84.94938900211595012 ) ) ;
#41261=CARTESIAN_POINT ( 'NONE',  ( -1.750000000000002220, 14.46891108675447946, -62.79431413575483845 ) ) ;
#41263=CARTESIAN_POINT ( 'NONE',  ( -3.310556943750000425, 19.41135094264165772, -25.84743913623280065 ) ) ;
#41264=EDGE_CURVE ( 'NONE', #39728, #5960, #27846, .T. ) ;
#41265=CARTESIAN_POINT ( 'NONE',  ( -1.749999999999999778, 20.53108891324555074, -55.82139747004409713 ) ) ;
#41266=CARTESIAN_POINT ( 'NONE',  ( -3.500000000000000000, 19.52072594216370405, -46.04431413575483845 ) ) ;
#41267=CARTESIAN_POINT ( 'NONE',  ( 3.310556943750001313, 17.50000000000002132, -105.3516058028994564 ) ) ;
#41268=CARTESIAN_POINT ( 'NONE',  ( -1.655278471875002211, 14.63297358603754006, -31.68493913623279923 ) ) ;
#41275=CARTESIAN_POINT ( 'NONE',  ( 3.310556943750001313, 17.50000000000001776, -89.26410580289947916 ) ) ;
#41277=ORIENTED_EDGE ( 'NONE', *, *, #25320, .F. ) ;
#41279=CARTESIAN_POINT ( 'NONE',  ( 1.749999999999998224, 14.46891108675447946, -74.62764746908817415 ) ) ;
#41280=ORIENTED_EDGE ( 'NONE', *, *, #29206, .F. ) ;
#41283=CARTESIAN_POINT ( 'NONE',  ( 3.310556943750001313, 17.50000000000001776, -96.26410580289946495 ) ) ;
#41295=DIRECTION ( 'NONE',  ( -0.000000000000000000, 1.259100132267607459E-16, -1.000000000000000000 ) ) ;
#41296=EDGE_CURVE ( 'NONE', #23290, #2470, #33105, .T. ) ;
#41297=CARTESIAN_POINT ( 'NONE',  ( -1.655278471875002211, 14.63297358603755427, -137.5974391362328220 ) ) ;
#41298=CARTESIAN_POINT ( 'NONE',  ( -3.500000000000001332, 17.50000000000002487, -132.6547308033774186 ) ) ;
#41301=CARTESIAN_POINT ( 'NONE',  ( -1.394453263437886604E-15, 14.00000000000001776, -101.7109808024215027 ) ) ;
#41302=CARTESIAN_POINT ( 'NONE',  ( -3.310556943750002645, 15.58864905735837780, -126.7682724695661420 ) ) ;
#41303=CARTESIAN_POINT ( 'NONE',  ( -3.310556943750002645, 15.58864905735836714, -49.76827246956613493 ) ) ;
#41304=VERTEX_POINT ( 'NONE', #28053 ) ;
#41306=CARTESIAN_POINT ( 'NONE',  ( 3.500000000000001332, 17.50000000000002487, -136.1547308033774186 ) ) ;
#41309=CARTESIAN_POINT ( 'NONE',  ( 3.310556943750001313, 19.41135094264166483, -77.26827246956614204 ) ) ;
#41310=CARTESIAN_POINT ( 'NONE',  ( 1.750000000000001110, 20.53108891324555785, -129.2943141357548313 ) ) ;
#41311=CARTESIAN_POINT ( 'NONE',  ( -7.022189441860112050E-16, 13.67729811471672541, -108.5141058028994649 ) ) ;
#41312=ADVANCED_FACE ( 'NONE', ( #34646 ), #20848, .T. ) ;
#41313=DIRECTION ( 'NONE',  ( -0.000000000000000000, 1.259100132267607459E-16, -1.000000000000000000 ) ) ;
#41316=CARTESIAN_POINT ( 'NONE',  ( -1.749999999999999778, 20.53108891324555429, -83.12764746908818836 ) ) ;
#41317=CARTESIAN_POINT ( 'NONE',  ( 0.9378221735088952959, 21.00000000000004263, -102.9493890021159501 ) ) ;
#41318=CARTESIAN_POINT ( 'NONE',  ( -1.655278471875002211, 14.63297358603754184, -44.59743913623280775 ) ) ;
#41319=CARTESIAN_POINT ( 'NONE',  ( 3.310556943750001313, 17.50000000000001776, -100.3516058028994706 ) ) ;
#41322=CARTESIAN_POINT ( 'NONE',  ( -3.310556943750001313, 17.50000000000002132, -123.8516058028994564 ) ) ;
#41327=CARTESIAN_POINT ( 'NONE',  ( -3.500000000000002220, 15.47927405783632615, -57.57139747004410424 ) ) ;
#41330=AXIS2_PLACEMENT_3D ( 'NONE', #2362, #12130, #41925 ) ;
#41331=VERTEX_POINT ( 'NONE', #5511 ) ;
#41332=CARTESIAN_POINT ( 'NONE',  ( 3.310556943750001313, 19.41135094264166483, -74.26827246956612782 ) ) ;
#41337=DIRECTION ( 'NONE',  ( -0.000000000000000000, 1.259100132267607459E-16, -1.000000000000000000 ) ) ;
#41339=CARTESIAN_POINT ( 'NONE',  ( -3.310556943750001313, 17.50000000000001066, -32.76410580289947205 ) ) ;
#41343=ADVANCED_FACE ( 'NONE', ( #1699 ), #31246, .T. ) ;
#41345=CARTESIAN_POINT ( 'NONE',  ( -1.655278471874999990, 20.36702641396248836, -47.93077246956614346 ) ) ;
#41346=ORIENTED_EDGE ( 'NONE', *, *, #23088, .T. ) ;
#41349=CARTESIAN_POINT ( 'NONE',  ( 3.500000000000001332, 17.50000000000001066, -23.46098080242150985 ) ) ;
#41351=CARTESIAN_POINT ( 'NONE',  ( 1.749999999999998224, 14.46891108675447768, -63.32139747004410424 ) ) ;
#41352=CARTESIAN_POINT ( 'NONE',  ( 3.500000000000000000, 15.47927405783633326, -112.5443141357548740 ) ) ;
#41353=CARTESIAN_POINT ( 'NONE',  ( 3.500000000000001776, 19.52072594216370405, -32.37764746908818125 ) ) ;
#41355=CARTESIAN_POINT ( 'NONE',  ( 3.500000000000001332, 17.50000000000001421, -70.46098080242151696 ) ) ;
#41357=CARTESIAN_POINT ( 'NONE',  ( 4.286263797015737581E-16, 14.00000000000002487, -149.5231586289125687 ) ) ;
#41359=CARTESIAN_POINT ( 'NONE',  ( -1.749999999999999778, 20.53108891324556140, -143.1276474690881741 ) ) ;
#41360=FACE_OUTER_BOUND ( 'NONE', #9602, .T. ) ;
#41361=CARTESIAN_POINT ( 'NONE',  ( 3.310556943749999981, 15.58864905735837425, -127.3474391362328078 ) ) ;
#41366=CARTESIAN_POINT ( 'NONE',  ( 3.500000000000001332, 19.52072594216370405, -24.07139747004409358 ) ) ;
#41367=CARTESIAN_POINT ( 'NONE',  ( 3.310556943749999981, 15.58864905735837247, -117.4349391362327850 ) ) ;
#41369=CARTESIAN_POINT ( 'NONE',  ( 3.500000000000001776, 19.52072594216370405, -37.07139747004409003 ) ) ;
#41370=DIRECTION ( 'NONE',  ( -0.000000000000000000, 1.259100132267607459E-16, -1.000000000000000000 ) ) ;
#41372=CARTESIAN_POINT ( 'NONE',  ( -3.310556943750001313, 17.50000000000002487, -137.8516058028994564 ) ) ;
#41375=CARTESIAN_POINT ( 'NONE',  ( 1.655278471874998436, 14.63297358603754006, -48.51827246956613493 ) ) ;
#41377=CARTESIAN_POINT ( 'NONE',  ( 4.648177544792955347E-16, 21.00000000000001421, -73.21098080242151696 ) ) ;
#41378=CARTESIAN_POINT ( 'NONE',  ( 3.310556943750001313, 19.41135094264166128, -68.26827246956612782 ) ) ;
#41380=CARTESIAN_POINT ( 'NONE',  ( -7.022189441860112050E-16, 13.67729811471672186, -72.51410580289946495 ) ) ;
#41381=ORIENTED_EDGE ( 'NONE', *, *, #12432, .T. ) ;
#41382=VERTEX_POINT ( 'NONE', #27442 ) ;
#41383=CARTESIAN_POINT ( 'NONE',  ( 3.310556943749999981, 15.58864905735836892, -93.43493913623281344 ) ) ;
#41385=CARTESIAN_POINT ( 'NONE',  ( -1.394453263437886604E-15, 14.00000000000001066, -49.71098080242150274 ) ) ;
#41386=CARTESIAN_POINT ( 'NONE',  ( -1.750000000000002220, 14.46891108675448478, -105.7943141357548313 ) ) ;
#41387=CARTESIAN_POINT ( 'NONE',  ( -0.9378221735089310451, 14.00000000000001599, -69.75563900116003424 ) ) ;
#41388=CARTESIAN_POINT ( 'NONE',  ( 3.310556943749999981, 15.58864905735836182, -48.34743913623281486 ) ) ;
#41389=( BOUNDED_CURVE ( )  B_SPLINE_CURVE ( 2, ( #40113, #20554, #10982, #23969, #36936, #7367, #40332, #33307, #8202 ),
 .UNSPECIFIED., .F., .T. ) 
 B_SPLINE_CURVE_WITH_KNOTS ( ( 3, 2, 2, 2, 3 ),
 ( 0.6270833333333333259, 0.6277777777777777679, 0.6291666666666666519, 0.6305555555555555358, 0.6312499999999999778 ),
 .UNSPECIFIED. ) 
 CURVE ( )  GEOMETRIC_REPRESENTATION_ITEM ( )  RATIONAL_B_SPLINE_CURVE ( ( 0.9330127018922194093, 0.9330127018922194093, 1.000000000000000000, 0.8660254037844387076, 1.000000000000000000, 0.8660254037844387076, 1.000000000000000000, 0.9330127018922194093, 0.9330127018922194093 ) ) 
 REPRESENTATION_ITEM ( '' )  );
#41391=DIRECTION ( 'NONE',  ( -0.000000000000000000, 1.259100132267607459E-16, -1.000000000000000000 ) ) ;
#41392=CARTESIAN_POINT ( 'NONE',  ( -3.310556943750001313, 17.50000000000002132, -112.7641058028994792 ) ) ;
#41393=CARTESIAN_POINT ( 'NONE',  ( 0.9378221735089281585, 14.00000000000002132, -96.36007260463890134 ) ) ;
#41398=ORIENTED_EDGE ( 'NONE', *, *, #37303, .F. ) ;
#41400=CARTESIAN_POINT ( 'NONE',  ( 1.655278471875001101, 20.36702641396248836, -63.09743913623280775 ) ) ;
#41403=CARTESIAN_POINT ( 'NONE',  ( 4.648177544792955347E-16, 21.00000000000002132, -103.9047308033774186 ) ) ;
#41407=CARTESIAN_POINT ( 'NONE',  ( 0.000000000000000000, 21.00000000000002487, -149.5231586289125687 ) ) ;
#41410=CARTESIAN_POINT ( 'NONE',  ( -1.655278471874999990, 20.36702641396249547, -128.9307724695661364 ) ) ;
#41412=CARTESIAN_POINT ( 'NONE',  ( 1.655278471874998436, 14.63297358603754006, -41.51827246956612782 ) ) ;
#41413=CARTESIAN_POINT ( 'NONE',  ( 3.310556943750001313, 17.50000000000001066, -30.35160580289947418 ) ) ;
#41414=CARTESIAN_POINT ( 'NONE',  ( 3.310556943750001313, 17.50000000000001776, -94.35160580289947063 ) ) ;
#41415=CARTESIAN_POINT ( 'NONE',  ( -1.655278471874999990, 20.36702641396249902, -142.9307724695661364 ) ) ;
#41419=CARTESIAN_POINT ( 'NONE',  ( -1.655278471874999990, 20.36702641396249902, -135.0182724695661420 ) ) ;
#41422=DIRECTION ( 'NONE',  ( -0.000000000000000000, 1.259100132267607459E-16, -1.000000000000000000 ) ) ;
#41424=CARTESIAN_POINT ( 'NONE',  ( 3.500000000000001332, 17.50000000000001776, -78.15473080337741862 ) ) ;
#41425=CARTESIAN_POINT ( 'NONE',  ( -3.310556943750000425, 19.41135094264166483, -63.93493913623279923 ) ) ;
#41428=CYLINDRICAL_SURFACE ( 'NONE', #1676, 3.499999999999999556 ) ;
#41429=CARTESIAN_POINT ( 'NONE',  ( 3.310556943749999981, 15.58864905735836892, -92.43493913623279923 ) ) ;
#41431=CARTESIAN_POINT ( 'NONE',  ( -3.310556943750001313, 17.50000000000002132, -111.7641058028994649 ) ) ;
#41433=VERTEX_POINT ( 'NONE', #18903 ) ;
#41435=CARTESIAN_POINT ( 'NONE',  ( -3.500000000000001332, 17.50000000000002132, -109.6547308033774328 ) ) ;
#41436=CARTESIAN_POINT ( 'NONE',  ( -3.500000000000000000, 19.52072594216370405, -28.73806413671076143 ) ) ;
#41439=CARTESIAN_POINT ( 'NONE',  ( 4.648177544792955347E-16, 21.00000000000001066, -32.90473080337742573 ) ) ;
#41441=CARTESIAN_POINT ( 'NONE',  ( 3.310556943750001313, 19.41135094264166483, -70.18077246956613635 ) ) ;
#41443=CARTESIAN_POINT ( 'NONE',  ( 4.648177544792955347E-16, 21.00000000000002132, -111.9047308033774186 ) ) ;
#41444=( BOUNDED_CURVE ( )  B_SPLINE_CURVE ( 2, ( #25281, #25501, #5715, #2313, #12083, #38466, #41879, #9111, #19110 ),
 .UNSPECIFIED., .F., .F. ) 
 B_SPLINE_CURVE_WITH_KNOTS ( ( 3, 2, 2, 2, 3 ),
 ( 0.3187499999999999778, 0.3194444444444444198, 0.3208333333333333592, 0.3222222222222222432, 0.3229166666666666852 ),
 .UNSPECIFIED. ) 
 CURVE ( )  GEOMETRIC_REPRESENTATION_ITEM ( )  RATIONAL_B_SPLINE_CURVE ( ( 0.9330127018922194093, 0.9330127018922194093, 1.000000000000000000, 0.8660254037844387076, 1.000000000000000000, 0.8660254037844387076, 1.000000000000000000, 0.9330127018922194093, 0.9330127018922194093 ) ) 
 REPRESENTATION_ITEM ( '' )  );
#41447=CARTESIAN_POINT ( 'NONE',  ( 1.655278471875001101, 20.36702641396248481, -24.09743913623281486 ) ) ;
#41449=CARTESIAN_POINT ( 'NONE',  ( 1.655278471874998436, 14.63297358603754361, -78.43077246956615056 ) ) ;
#41450=EDGE_LOOP ( 'NONE', ( #14677, #12408, #1280, #36593 ) ) ;
#41451=ORIENTED_EDGE ( 'NONE', *, *, #10436, .T. ) ;
#41452=VECTOR ( 'NONE', #27523, 1000.000000000000000 ) ;
#41453=CARTESIAN_POINT ( 'NONE',  ( -1.749999999999999778, 20.53108891324555074, -53.82139747004409713 ) ) ;
#41454=EDGE_CURVE ( 'NONE', #16103, #33816, #28677, .T. ) ;
#41457=VECTOR ( 'NONE', #9282, 1000.000000000000000 ) ;
#41458=EDGE_CURVE ( 'NONE', #12815, #21111, #14107, .T. ) ;
#41459=CARTESIAN_POINT ( 'NONE',  ( -1.749999999999999778, 20.53108891324555429, -89.82139747004410424 ) ) ;
#41460=CARTESIAN_POINT ( 'NONE',  ( 1.655278471874998436, 14.63297358603754006, -41.51827246956612782 ) ) ;
#41461=CARTESIAN_POINT ( 'NONE',  ( -3.310556943750002645, 15.58864905735837780, -109.7682724695661278 ) ) ;
#41462=VERTEX_POINT ( 'NONE', #35494 ) ;
#41463=CARTESIAN_POINT ( 'NONE',  ( -7.022189441860112050E-16, 13.67729811471671475, -33.51410580289947205 ) ) ;
#41464=CARTESIAN_POINT ( 'NONE',  ( -3.310556943750001313, 17.50000000000001421, -59.85160580289947063 ) ) ;
#41465=CARTESIAN_POINT ( 'NONE',  ( -3.500000000000000888, 19.52072594216371826, -105.0443141357548313 ) ) ;
#41467=CARTESIAN_POINT ( 'NONE',  ( 1.655278471875001101, 20.36702641396249192, -94.09743913623280775 ) ) ;
#41468=CARTESIAN_POINT ( 'NONE',  ( -7.424026671074350129E-16, 13.45854811567263809, -97.40473080337743284 ) ) ;
#41473=CARTESIAN_POINT ( 'NONE',  ( 1.749999999999998224, 14.46891108675447768, -60.62764746908818125 ) ) ;
#41474=VECTOR ( 'NONE', #31271, 1000.000000000000000 ) ;
#41476=CARTESIAN_POINT ( 'NONE',  ( 3.310556943750001313, 17.50000000000001066, -26.26410580289947916 ) ) ;
#41477=EDGE_CURVE ( 'NONE', #11917, #36671, #6353, .T. ) ;
#41478=CARTESIAN_POINT ( 'NONE',  ( -1.750000000000002220, 14.46891108675447768, -47.48806413671076143 ) ) ;
#41480=CARTESIAN_POINT ( 'NONE',  ( -7.022189441860112050E-16, 13.67729811471672541, -106.6016058028994564 ) ) ;
#41481=CARTESIAN_POINT ( 'NONE',  ( 2.340729813953370519E-16, 21.32270188528330834, -33.10160580289946353 ) ) ;
#41488=CARTESIAN_POINT ( 'NONE',  ( -3.310556943750000425, 19.41135094264166838, -87.84743913623279354 ) ) ;
#41491=CARTESIAN_POINT ( 'NONE',  ( -3.500000000000002220, 15.47927405783633326, -101.8776474690881741 ) ) ;
#41492=CARTESIAN_POINT ( 'NONE',  ( -0.9378221735089310451, 14.00000000000001066, -50.44938900211595012 ) ) ;
#41493=ORIENTED_EDGE ( 'NONE', *, *, #35900, .T. ) ;
#41496=CARTESIAN_POINT ( 'NONE',  ( -1.655278471875002211, 14.63297358603754716, -94.59743913623280775 ) ) ;
#41501=CARTESIAN_POINT ( 'NONE',  ( 4.648177544792955347E-16, 21.00000000000002487, -139.2109808024214885 ) ) ;
#41506=EDGE_CURVE ( 'NONE', #19314, #9822, #16157, .T. ) ;
#41507=ADVANCED_FACE ( 'NONE', ( #34856 ), #2528, .T. ) ;
#41508=ORIENTED_EDGE ( 'NONE', *, *, #15656, .F. ) ;
#41511=CARTESIAN_POINT ( 'NONE',  ( 1.750000000000001110, 20.53108891324555785, -129.2943141357548313 ) ) ;
#41512=EDGE_CURVE ( 'NONE', #11127, #15800, #3787, .T. ) ;
#41513=CARTESIAN_POINT ( 'NONE',  ( 1.655278471875001101, 20.36702641396249902, -139.0974391362327935 ) ) ;
#41516=CARTESIAN_POINT ( 'NONE',  ( 3.310556943749999981, 15.58864905735837425, -125.4349391362327992 ) ) ;
#41517=CARTESIAN_POINT ( 'NONE',  ( 3.310556943750001313, 19.41135094264166128, -48.26827246956613493 ) ) ;
#41518=ORIENTED_EDGE ( 'NONE', *, *, #8488, .F. ) ;
#41519=CARTESIAN_POINT ( 'NONE',  ( 3.500000000000000000, 15.47927405783633503, -136.2380641367107614 ) ) ;
#41520=VECTOR ( 'NONE', #34760, 1000.000000000000000 ) ;
#41522=CARTESIAN_POINT ( 'NONE',  ( 3.310556943749999981, 15.58864905735836714, -77.43493913623279923 ) ) ;
#41523=CARTESIAN_POINT ( 'NONE',  ( 2.474675557024783212E-16, 21.54145188432740099, -125.2109808024215170 ) ) ;
#41524=CARTESIAN_POINT ( 'NONE',  ( 3.310556943749999981, 15.58864905735837247, -109.3474391362328220 ) ) ;
#41525=CARTESIAN_POINT ( 'NONE',  ( -7.022189441860112050E-16, 13.67729811471671297, -23.60160580289946708 ) ) ;
#41528=CARTESIAN_POINT ( 'NONE',  ( 3.500000000000001332, 17.50000000000001776, -76.46098080242150274 ) ) ;
#41529=CARTESIAN_POINT ( 'NONE',  ( -7.022189441860112050E-16, 13.67729811471671653, -42.51410580289947916 ) ) ;
#41530=CARTESIAN_POINT ( 'NONE',  ( -3.310556943750002645, 15.58864905735837425, -100.7682724695661278 ) ) ;
#41531=CARTESIAN_POINT ( 'NONE',  ( -0.9378221735089310451, 14.00000000000002309, -113.7556390011600342 ) ) ;
#41532=CARTESIAN_POINT ( 'NONE',  ( -7.424026671074350129E-16, 13.45854811567263454, -64.40473080337743284 ) ) ;
#41533=CARTESIAN_POINT ( 'NONE',  ( 0.000000000000000000, 17.50000000000002487, -149.5231586289125687 ) ) ;
#41535=CARTESIAN_POINT ( 'NONE',  ( -3.310556943750000425, 19.41135094264166838, -120.9349391362327992 ) ) ;
#41536=CARTESIAN_POINT ( 'NONE',  ( -3.500000000000002220, 15.47927405783632970, -91.87764746908817415 ) ) ;
#41539=CARTESIAN_POINT ( 'NONE',  ( 4.286263797015737581E-16, 14.00000000000002487, -149.5231586289125687 ) ) ;
#41540=CARTESIAN_POINT ( 'NONE',  ( -0.9378221735089291577, 21.00000000000001421, -71.86007260463891555 ) ) ;
#41544=CARTESIAN_POINT ( 'NONE',  ( 3.310556943750001313, 17.50000000000001776, -77.35160580289945642 ) ) ;
#41548=EDGE_CURVE ( 'NONE', #27029, #21810, #8136, .T. ) ;
#41551=CARTESIAN_POINT ( 'NONE',  ( -3.310556943750001313, 17.50000000000001066, -34.76410580289947205 ) ) ;
#41554=ORIENTED_EDGE ( 'NONE', *, *, #28841, .T. ) ;
#41556=EDGE_CURVE ( 'NONE', #27997, #12774, #25542, .T. ) ;
#41559=EDGE_LOOP ( 'NONE', ( #35897, #37013, #6224, #10426 ) ) ;
#41561=CARTESIAN_POINT ( 'NONE',  ( -1.750000000000002220, 14.46891108675448656, -114.7943141357548313 ) ) ;
#41564=( BOUNDED_CURVE ( )  B_SPLINE_CURVE ( 2, ( #15166, #33744, #24180, #4598, #20341, #17157, #4174, #20972, #37150 ),
 .UNSPECIFIED., .F., .F. ) 
 B_SPLINE_CURVE_WITH_KNOTS ( ( 3, 2, 2, 2, 3 ),
 ( 0.3687500000000000222, 0.3694444444444444642, 0.3708333333333333481, 0.3722222222222222321, 0.3729166666666666741 ),
 .UNSPECIFIED. ) 
 CURVE ( )  GEOMETRIC_REPRESENTATION_ITEM ( )  RATIONAL_B_SPLINE_CURVE ( ( 0.9330127018922194093, 0.9330127018922194093, 1.000000000000000000, 0.8660254037844387076, 1.000000000000000000, 0.8660254037844387076, 1.000000000000000000, 0.9330127018922194093, 0.9330127018922194093 ) ) 
 REPRESENTATION_ITEM ( '' )  );
#41566=CARTESIAN_POINT ( 'NONE',  ( 3.500000000000001332, 17.50000000000001066, -35.46098080242150985 ) ) ;
#41567=CARTESIAN_POINT ( 'NONE',  ( -3.500000000000001332, 17.50000000000001421, -65.96098080242150274 ) ) ;
#41568=CARTESIAN_POINT ( 'NONE',  ( 4.648177544792955347E-16, 21.00000000000001421, -70.21098080242150274 ) ) ;
#41569=CARTESIAN_POINT ( 'NONE',  ( 0.9378221735089300459, 21.00000000000001776, -96.25563900116003424 ) ) ;
#41571=CARTESIAN_POINT ( 'NONE',  ( -7.424026671074350129E-16, 13.45854811567264164, -139.7109808024215170 ) ) ;
#41573=CARTESIAN_POINT ( 'NONE',  ( 2.340729813953370519E-16, 21.32270188528331900, -126.0141058028994792 ) ) ;
#41577=CARTESIAN_POINT ( 'NONE',  ( 3.500000000000000000, 15.47927405783632793, -98.54431413575484555 ) ) ;
#41579=CARTESIAN_POINT ( 'NONE',  ( -3.310556943750002645, 15.58864905735837780, -115.7682724695661278 ) ) ;
#41581=CARTESIAN_POINT ( 'NONE',  ( -3.500000000000000888, 19.52072594216370405, -31.73806413671076143 ) ) ;
#41582=CARTESIAN_POINT ( 'NONE',  ( -0.9378221735089291577, 21.00000000000002132, -109.1663226036829855 ) ) ;
#41584=CARTESIAN_POINT ( 'NONE',  ( 1.655278471874998436, 14.63297358603755249, -140.5182724695661420 ) ) ;
#41586=FACE_OUTER_BOUND ( 'NONE', #37576, .T. ) ;
#41587=CARTESIAN_POINT ( 'NONE',  ( 3.310556943750001313, 17.50000000000001421, -49.35160580289946353 ) ) ;
#41590=CARTESIAN_POINT ( 'NONE',  ( -1.655278471875002211, 14.63297358603754539, -71.68493913623278502 ) ) ;
#41592=CARTESIAN_POINT ( 'NONE',  ( -1.655278471874999990, 20.36702641396248836, -69.93077246956613635 ) ) ;
#41594=CARTESIAN_POINT ( 'NONE',  ( -3.310556943750001313, 17.50000000000001776, -90.85160580289947063 ) ) ;
#41596=CARTESIAN_POINT ( 'NONE',  ( 3.500000000000001332, 17.50000000000001421, -67.46098080242150274 ) ) ;
#41600=CARTESIAN_POINT ( 'NONE',  ( -3.310556943750002201, 15.58864905735836714, -50.68077246956613635 ) ) ;
#41603=CARTESIAN_POINT ( 'NONE',  ( 3.310556943749999981, 15.58864905735837070, -106.3474391362328078 ) ) ;
#41605=ORIENTED_EDGE ( 'NONE', *, *, #6369, .F. ) ;
#41610=EDGE_CURVE ( 'NONE', #1435, #36297, #37464, .T. ) ;
#41611=CARTESIAN_POINT ( 'NONE',  ( 3.310556943750001313, 17.50000000000001421, -62.26410580289947205 ) ) ;
#41612=ORIENTED_EDGE ( 'NONE', *, *, #32136, .T. ) ;
#41613=VERTEX_POINT ( 'NONE', #3573 ) ;
#41614=CARTESIAN_POINT ( 'NONE',  ( 4.648177544792955347E-16, 21.00000000000001421, -51.21098080242150274 ) ) ;
#41617=LINE ( 'NONE', #15254, #3406 ) ;
#41619=LINE ( 'NONE', #9070, #11947 ) ;
#41620=CARTESIAN_POINT ( 'NONE',  ( 1.655278471875001101, 20.36702641396249547, -123.0974391362328078 ) ) ;
#41622=CARTESIAN_POINT ( 'NONE',  ( -3.310556943750001313, 17.50000000000001066, -40.85160580289947063 ) ) ;
#41623=CARTESIAN_POINT ( 'NONE',  ( 2.340729813953370519E-16, 21.32270188528330479, -27.10160580289947063 ) ) ;
#41625=CARTESIAN_POINT ( 'NONE',  ( -3.310556943750000425, 19.41135094264166483, -85.93493913623278502 ) ) ;
#41626=CARTESIAN_POINT ( 'NONE',  ( -1.655278471874999990, 20.36702641396249902, -137.9307724695661364 ) ) ;
#41631=CARTESIAN_POINT ( 'NONE',  ( -1.655278471874999990, 20.36702641396249902, -132.0182724695661420 ) ) ;
#41632=CARTESIAN_POINT ( 'NONE',  ( -3.500000000000001332, 17.50000000000001776, -83.96098080242150274 ) ) ;
#41635=CARTESIAN_POINT ( 'NONE',  ( -1.750000000000002220, 14.46891108675448656, -122.4880641367107614 ) ) ;
#41637=CARTESIAN_POINT ( 'NONE',  ( -1.750000000000002220, 14.46891108675448123, -78.48806413671076143 ) ) ;
#41638=CARTESIAN_POINT ( 'NONE',  ( -3.310556943750000425, 19.41135094264166483, -62.93493913623279923 ) ) ;
#41641=CARTESIAN_POINT ( 'NONE',  ( 7.785697387528201340E-15, 14.00000000000002487, -136.7109808024214885 ) ) ;
#41642=CARTESIAN_POINT ( 'NONE',  ( -0.9378221735089310451, 14.00000000000001599, -58.44938900211595012 ) ) ;
#41643=CARTESIAN_POINT ( 'NONE',  ( 3.310556943750001313, 19.41135094264166483, -83.26827246956614204 ) ) ;
#41644=CARTESIAN_POINT ( 'NONE',  ( -1.749999999999999778, 20.53108891324555785, -116.8213974700440900 ) ) ;
#41645=CARTESIAN_POINT ( 'NONE',  ( -3.310556943750002201, 15.58864905735837780, -115.6807724695661364 ) ) ;
#41647=ORIENTED_EDGE ( 'NONE', *, *, #21423, .T. ) ;
#41648=CARTESIAN_POINT ( 'NONE',  ( 2.474675557024783212E-16, 21.54145188432740099, -109.9047308033774186 ) ) ;
#41649=CARTESIAN_POINT ( 'NONE',  ( 4.286263797015737581E-16, 14.00000000000002487, -149.5231586289125687 ) ) ;
#41651=CARTESIAN_POINT ( 'NONE',  ( -1.394453263437886604E-15, 14.00000000000001776, -82.40473080337743284 ) ) ;
#41652=CARTESIAN_POINT ( 'NONE',  ( -3.500000000000000000, 19.52072594216370405, -27.04431413575483845 ) ) ;
#41654=CARTESIAN_POINT ( 'NONE',  ( 3.310556943749999981, 15.58864905735836537, -66.34743913623280775 ) ) ;
#41655=CARTESIAN_POINT ( 'NONE',  ( 3.500000000000001332, 17.50000000000001421, -59.46098080242151696 ) ) ;
#41657=CARTESIAN_POINT ( 'NONE',  ( -3.500000000000002220, 15.47927405783633503, -125.5713974700440900 ) ) ;
#41661=CARTESIAN_POINT ( 'NONE',  ( 4.648177544792955347E-16, 21.00000000000001066, -45.21098080242150985 ) ) ;
#41663=CARTESIAN_POINT ( 'NONE',  ( -7.022189441860112050E-16, 13.67729811471672363, -81.51410580289946495 ) ) ;
#41664=EDGE_LOOP ( 'NONE', ( #20519, #18570, #2151, #14622 ) ) ;
#41666=EDGE_CURVE ( 'NONE', #13827, #21956, #11999, .T. ) ;
#41668=CARTESIAN_POINT ( 'NONE',  ( -1.655278471875002211, 14.63297358603755427, -138.5974391362327935 ) ) ;
#41669=CARTESIAN_POINT ( 'NONE',  ( -1.750000000000002220, 14.46891108675447768, -51.48806413671076854 ) ) ;
#41670=CARTESIAN_POINT ( 'NONE',  ( -0.9378221735089310451, 14.00000000000002309, -113.4493890021159643 ) ) ;
#41671=CARTESIAN_POINT ( 'NONE',  ( 3.310556943750001313, 17.50000000000001066, -42.35160580289947063 ) ) ;
#41672=CARTESIAN_POINT ( 'NONE',  ( -1.655278471875002211, 14.63297358603754894, -105.6849391362327992 ) ) ;
#41674=CARTESIAN_POINT ( 'NONE',  ( -7.022189441860112050E-16, 13.67729811471671475, -29.51410580289948982 ) ) ;
#41676=CARTESIAN_POINT ( 'NONE',  ( 3.310556943749999981, 15.58864905735836537, -59.43493913623279923 ) ) ;
#41677=CARTESIAN_POINT ( 'NONE',  ( -3.500000000000001332, 17.50000000000002132, -105.9609808024215027 ) ) ;
#41679=CARTESIAN_POINT ( 'NONE',  ( 3.500000000000001332, 17.50000000000001776, -99.15473080337743284 ) ) ;
#41683=CARTESIAN_POINT ( 'NONE',  ( -3.500000000000002220, 15.47927405783632437, -58.87764746908817415 ) ) ;
#41685=CARTESIAN_POINT ( 'NONE',  ( -3.310556943750002645, 15.58864905735836537, -28.68077246956614346 ) ) ;
#41686=( BOUNDED_CURVE ( )  B_SPLINE_CURVE ( 2, ( #10584, #17795, #30346, #23562, #7595, #14188, #1219, #36521, #11406 ),
 .UNSPECIFIED., .F., .T. ) 
 B_SPLINE_CURVE_WITH_KNOTS ( ( 3, 2, 2, 2, 3 ),
 ( 0.2520833333333333259, 0.2527777777777777679, 0.2541666666666666519, 0.2555555555555555358, 0.2562499999999999778 ),
 .UNSPECIFIED. ) 
 CURVE ( )  GEOMETRIC_REPRESENTATION_ITEM ( )  RATIONAL_B_SPLINE_CURVE ( ( 0.9330127018922194093, 0.9330127018922194093, 1.000000000000000000, 0.8660254037844387076, 1.000000000000000000, 0.8660254037844387076, 1.000000000000000000, 0.9330127018922194093, 0.9330127018922194093 ) ) 
 REPRESENTATION_ITEM ( '' )  );
#41687=CARTESIAN_POINT ( 'NONE',  ( -3.500000000000001332, 17.50000000000001421, -47.65473080337742573 ) ) ;
#41689=CARTESIAN_POINT ( 'NONE',  ( -1.655278471874999990, 20.36702641396248481, -34.01827246956613493 ) ) ;
#41692=CARTESIAN_POINT ( 'NONE',  ( 1.750000000000001110, 20.53108891324555074, -49.98806413671076854 ) ) ;
#41697=CARTESIAN_POINT ( 'NONE',  ( 3.310556943750001313, 17.50000000000001776, -80.26410580289946495 ) ) ;
#41698=CARTESIAN_POINT ( 'NONE',  ( 4.648177544792955347E-16, 21.00000000000001066, -25.90473080337743284 ) ) ;
#41700=CARTESIAN_POINT ( 'NONE',  ( -1.394453263437886604E-15, 14.00000000000001066, -37.71098080242150985 ) ) ;
#41701=CARTESIAN_POINT ( 'NONE',  ( 0.9378221735089281585, 14.00000000000001599, -80.66632260368298546 ) ) ;
#41705=CARTESIAN_POINT ( 'NONE',  ( 3.310556943750001313, 19.41135094264166483, -93.18077246956613635 ) ) ;
#41707=VERTEX_POINT ( 'NONE', #15625 ) ;
#41709=ORIENTED_EDGE ( 'NONE', *, *, #34727, .T. ) ;
#41712=CYLINDRICAL_SURFACE ( 'NONE', #32603, 3.499999999999999556 ) ;
#41716=EDGE_CURVE ( 'NONE', #16691, #4203, #34473, .T. ) ;
#41717=CARTESIAN_POINT ( 'NONE',  ( -1.750000000000002220, 14.46891108675448834, -127.4880641367107614 ) ) ;
#41718=CYLINDRICAL_SURFACE ( 'NONE', #21461, 3.499999999999999556 ) ;
#41719=ADVANCED_FACE ( 'NONE', ( #31565 ), #12423, .T. ) ;
#41720=CARTESIAN_POINT ( 'NONE',  ( 2.340729813953370519E-16, 21.32270188528332255, -131.0141058028994792 ) ) ;
#41721=CARTESIAN_POINT ( 'NONE',  ( 3.500000000000001332, 19.52072594216371826, -141.3776474690881741 ) ) ;
#41723=CARTESIAN_POINT ( 'NONE',  ( 3.500000000000001332, 17.50000000000001066, -28.46098080242151340 ) ) ;
#41724=CARTESIAN_POINT ( 'NONE',  ( 3.310556943749999981, 15.58864905735837425, -126.4349391362327992 ) ) ;
#41725=CARTESIAN_POINT ( 'NONE',  ( 1.655278471874998436, 14.63297358603754006, -49.51827246956613493 ) ) ;
#41727=CARTESIAN_POINT ( 'NONE',  ( 1.750000000000001110, 20.53108891324556140, -130.9880641367107614 ) ) ;
#41729=CARTESIAN_POINT ( 'NONE',  ( 1.655278471874998436, 14.63297358603754361, -76.51827246956612782 ) ) ;
#41730=CARTESIAN_POINT ( 'NONE',  ( -3.500000000000002220, 15.47927405783633503, -123.8776474690881884 ) ) ;
#41731=CARTESIAN_POINT ( 'NONE',  ( 1.655278471874998436, 14.63297358603754716, -105.4307724695661364 ) ) ;
#41732=DIRECTION ( 'NONE',  ( -0.000000000000000000, 1.259100132267607459E-16, -1.000000000000000000 ) ) ;
#41736=CARTESIAN_POINT ( 'NONE',  ( 1.749999999999998224, 14.46891108675447946, -74.62764746908817415 ) ) ;
#41738=CARTESIAN_POINT ( 'NONE',  ( -3.310556943750002645, 15.58864905735836714, -40.68077246956613635 ) ) ;
#41739=CARTESIAN_POINT ( 'NONE',  ( -3.310556943750001313, 17.50000000000001776, -99.85160580289947063 ) ) ;
#41742=CARTESIAN_POINT ( 'NONE',  ( -3.500000000000002220, 15.47927405783632437, -62.57139747004409713 ) ) ;
#41745=CARTESIAN_POINT ( 'NONE',  ( 3.310556943749999981, 15.58864905735837247, -115.4349391362327708 ) ) ;
#41746=CARTESIAN_POINT ( 'NONE',  ( -0.9378221735089291577, 21.00000000000001066, -28.16632260368299256 ) ) ;
#41750=CARTESIAN_POINT ( 'NONE',  ( 1.749999999999998224, 14.46891108675448301, -107.6276474690881741 ) ) ;
#41753=ORIENTED_EDGE ( 'NONE', *, *, #20466, .T. ) ;
#41754=CARTESIAN_POINT ( 'NONE',  ( 2.340729813953370519E-16, 21.32270188528331190, -76.10160580289945642 ) ) ;
#41757=VECTOR ( 'NONE', #25998, 1000.000000000000000 ) ;
#41758=CARTESIAN_POINT ( 'NONE',  ( -0.9378221735089310451, 14.00000000000002132, -102.4493890021159359 ) ) ;
#41762=CARTESIAN_POINT ( 'NONE',  ( 3.310556943750001313, 19.41135094264166128, -36.18077246956613635 ) ) ;
#41767=CARTESIAN_POINT ( 'NONE',  ( -1.394453263437886604E-15, 14.00000000000001776, -96.71098080242150274 ) ) ;
#41770=CARTESIAN_POINT ( 'NONE',  ( 0.9378221735089281585, 14.00000000000001776, -90.66632260368299967 ) ) ;
#41772=AXIS2_PLACEMENT_3D ( 'NONE', #19386, #32358, #30001 ) ;
#41773=CARTESIAN_POINT ( 'NONE',  ( 1.750000000000001110, 20.53108891324556140, -140.2943141357548313 ) ) ;
#41774=CARTESIAN_POINT ( 'NONE',  ( 1.750000000000001110, 20.53108891324555785, -118.9880641367107614 ) ) ;
#41776=CARTESIAN_POINT ( 'NONE',  ( -3.500000000000000888, 19.52072594216370405, -33.04431413575484555 ) ) ;
#41780=EDGE_CURVE ( 'NONE', #29815, #28708, #14420, .T. ) ;
#41781=VECTOR ( 'NONE', #34982, 1000.000000000000000 ) ;
#41782=CARTESIAN_POINT ( 'NONE',  ( 1.749999999999998224, 14.46891108675448834, -142.6276474690881741 ) ) ;
#41784=CARTESIAN_POINT ( 'NONE',  ( 3.500000000000000000, 15.47927405783633503, -136.5443141357548598 ) ) ;
#41785=EDGE_CURVE ( 'NONE', #14818, #6760, #33570, .T. ) ;
#41787=CARTESIAN_POINT ( 'NONE',  ( 1.655278471874998436, 14.63297358603754894, -121.4307724695661364 ) ) ;
#41789=ORIENTED_EDGE ( 'NONE', *, *, #33436, .F. ) ;
#41791=CARTESIAN_POINT ( 'NONE',  ( 4.648177544792955347E-16, 21.00000000000001421, -73.90473080337743284 ) ) ;
#41792=CARTESIAN_POINT ( 'NONE',  ( -3.500000000000002220, 15.47927405783632793, -91.87764746908818836 ) ) ;
#41794=CARTESIAN_POINT ( 'NONE',  ( 3.310556943750001313, 19.41135094264166128, -58.18077246956614346 ) ) ;
#41795=CARTESIAN_POINT ( 'NONE',  ( -3.310556943750001313, 17.50000000000002132, -116.8516058028994706 ) ) ;
#41796=LINE ( 'NONE', #29207, #20039 ) ;
#41797=CARTESIAN_POINT ( 'NONE',  ( 2.474675557024783212E-16, 21.54145188432739033, -32.90473080337742573 ) ) ;
#41798=DIRECTION ( 'NONE',  ( -0.000000000000000000, 1.259100132267607459E-16, -1.000000000000000000 ) ) ;
#41800=CARTESIAN_POINT ( 'NONE',  ( -3.310556943750000425, 19.41135094264167549, -137.9349391362327708 ) ) ;
#41802=CARTESIAN_POINT ( 'NONE',  ( -1.749999999999999778, 20.53108891324555074, -66.82139747004409003 ) ) ;
#41803=CARTESIAN_POINT ( 'NONE',  ( 2.340729813953370519E-16, 21.32270188528331190, -49.10160580289946353 ) ) ;
#41806=CARTESIAN_POINT ( 'NONE',  ( 3.310556943750001313, 17.50000000000001421, -70.35160580289947063 ) ) ;
#41808=CARTESIAN_POINT ( 'NONE',  ( -1.655278471874999990, 20.36702641396248836, -63.93077246956614346 ) ) ;
#41810=CARTESIAN_POINT ( 'NONE',  ( -1.655278471874999990, 20.36702641396249192, -89.01827246956612782 ) ) ;
#41811=EDGE_CURVE ( 'NONE', #25967, #26790, #9019, .T. ) ;
#41815=CARTESIAN_POINT ( 'NONE',  ( -0.9378221735089291577, 21.00000000000001776, -85.16632260368298546 ) ) ;
#41816=CARTESIAN_POINT ( 'NONE',  ( -1.749999999999999778, 20.53108891324555074, -70.12764746908817415 ) ) ;
#41817=CARTESIAN_POINT ( 'NONE',  ( -1.655278471874999990, 20.36702641396248836, -52.93077246956613635 ) ) ;
#41819=CARTESIAN_POINT ( 'NONE',  ( -3.310556943750001313, 17.50000000000002132, -105.7641058028994649 ) ) ;
#41820=CARTESIAN_POINT ( 'NONE',  ( -1.749999999999999778, 20.53108891324554719, -36.12764746908816704 ) ) ;
#41825=EDGE_LOOP ( 'NONE', ( #21400, #18372, #17131, #14135 ) ) ;
#41827=CARTESIAN_POINT ( 'NONE',  ( 2.340729813953370519E-16, 21.32270188528330834, -59.01410580289947916 ) ) ;
#41828=VERTEX_POINT ( 'NONE', #27188 ) ;
#41829=EDGE_LOOP ( 'NONE', ( #5195, #22650, #29159, #582 ) ) ;
#41831=CARTESIAN_POINT ( 'NONE',  ( 0.9378221735089281585, 14.00000000000001243, -55.66632260368299256 ) ) ;
#41834=ORIENTED_EDGE ( 'NONE', *, *, #118, .T. ) ;
#41836=CARTESIAN_POINT ( 'NONE',  ( -7.022189441860112050E-16, 13.67729811471672896, -126.5141058028994507 ) ) ;
#41839=CARTESIAN_POINT ( 'NONE',  ( 3.310556943750001313, 17.50000000000001066, -37.35160580289946353 ) ) ;
#41841=CARTESIAN_POINT ( 'NONE',  ( -1.655278471874999990, 20.36702641396248481, -28.01827246956613138 ) ) ;
#41842=CARTESIAN_POINT ( 'NONE',  ( -3.310556943750001313, 17.50000000000001776, -87.85160580289947063 ) ) ;
#41843=CARTESIAN_POINT ( 'NONE',  ( -1.655278471874999990, 20.36702641396249902, -138.9307724695661364 ) ) ;
#41846=CARTESIAN_POINT ( 'NONE',  ( 4.648177544792955347E-16, 21.00000000000002132, -113.9047308033774186 ) ) ;
#41847=CARTESIAN_POINT ( 'NONE',  ( -3.310556943750002645, 15.58864905735837780, -130.7682724695661420 ) ) ;
#41849=CARTESIAN_POINT ( 'NONE',  ( 1.750000000000001110, 20.53108891324555074, -56.29431413575483845 ) ) ;
#41850=CARTESIAN_POINT ( 'NONE',  ( -1.394453263437886604E-15, 14.00000000000001066, -28.40473080337742928 ) ) ;
#41851=CARTESIAN_POINT ( 'NONE',  ( 0.000000000000000000, 21.00000000000002487, -149.5231586289125687 ) ) ;
#41853=CARTESIAN_POINT ( 'NONE',  ( -3.500000000000001332, 17.50000000000001776, -78.65473080337743284 ) ) ;
#41855=CARTESIAN_POINT ( 'NONE',  ( -3.310556943750002201, 15.58864905735836892, -66.76827246956612782 ) ) ;
#41858=CARTESIAN_POINT ( 'NONE',  ( 0.000000000000000000, 21.00000000000002487, -149.5231586289125687 ) ) ;
#41859=CARTESIAN_POINT ( 'NONE',  ( -3.310556943750001313, 17.50000000000001776, -84.85160580289947063 ) ) ;
#41861=CARTESIAN_POINT ( 'NONE',  ( -1.655278471874999990, 20.36702641396249547, -112.9307724695661364 ) ) ;
#41862=CARTESIAN_POINT ( 'NONE',  ( 0.9378221735089300459, 21.00000000000001066, -34.25563900116002714 ) ) ;
#41865=CARTESIAN_POINT ( 'NONE',  ( -7.424026671074350129E-16, 13.45854811567263987, -110.4047308033774186 ) ) ;
#41868=CARTESIAN_POINT ( 'NONE',  ( -3.500000000000001332, 17.50000000000001421, -67.96098080242150274 ) ) ;
#41872=CARTESIAN_POINT ( 'NONE',  ( 3.310556943750001313, 17.50000000000001421, -67.26410580289947916 ) ) ;
#41874=CARTESIAN_POINT ( 'NONE',  ( -7.022189441860112050E-16, 13.67729811471672718, -123.5141058028994649 ) ) ;
#41875=CARTESIAN_POINT ( 'NONE',  ( -1.394453263437886604E-15, 14.00000000000001421, -71.40473080337743284 ) ) ;
#41877=ORIENTED_EDGE ( 'NONE', *, *, #27436, .T. ) ;
#41879=CARTESIAN_POINT ( 'NONE',  ( -1.750000000000002220, 14.46891108675448478, -104.7943141357548313 ) ) ;
#41880=CARTESIAN_POINT ( 'NONE',  ( 2.340729813953370519E-16, 21.32270188528331190, -76.01410580289947916 ) ) ;
#41882=ORIENTED_EDGE ( 'NONE', *, *, #28272, .T. ) ;
#41885=CARTESIAN_POINT ( 'NONE',  ( -3.310556943750000425, 19.41135094264167549, -141.8474391362327935 ) ) ;
#41887=CARTESIAN_POINT ( 'NONE',  ( 4.648177544792955347E-16, 21.00000000000002132, -113.9047308033774186 ) ) ;
#41888=CARTESIAN_POINT ( 'NONE',  ( -1.655278471874999990, 20.36702641396248481, -43.01827246956613493 ) ) ;
#41889=CARTESIAN_POINT ( 'NONE',  ( -1.655278471874999990, 20.36702641396249192, -102.0182724695661278 ) ) ;
#41892=( BOUNDED_CURVE ( )  B_SPLINE_CURVE ( 2, ( #39543, #23399, #36362, #30192, #33164, #27013, #37210, #5287, #8273 ),
 .UNSPECIFIED., .F., .F. ) 
 B_SPLINE_CURVE_WITH_KNOTS ( ( 3, 2, 2, 2, 3 ),
 ( 0.8187499999999999778, 0.8194444444444444198, 0.8208333333333333037, 0.8222222222222221877, 0.8229166666666666297 ),
 .UNSPECIFIED. ) 
 CURVE ( )  GEOMETRIC_REPRESENTATION_ITEM ( )  RATIONAL_B_SPLINE_CURVE ( ( 0.9330127018922194093, 0.9330127018922194093, 1.000000000000000000, 0.8660254037844387076, 1.000000000000000000, 0.8660254037844387076, 1.000000000000000000, 0.9330127018922194093, 0.9330127018922194093 ) ) 
 REPRESENTATION_ITEM ( '' )  );
#41893=CARTESIAN_POINT ( 'NONE',  ( -1.655278471875002211, 14.63297358603754006, -28.59743913623280420 ) ) ;
#41895=CARTESIAN_POINT ( 'NONE',  ( -1.749999999999999778, 20.53108891324555785, -106.1276474690881741 ) ) ;
#41898=CARTESIAN_POINT ( 'NONE',  ( -3.500000000000000888, 19.52072594216371115, -95.73806413671074722 ) ) ;
#41899=EDGE_CURVE ( 'NONE', #15782, #27445, #28259, .T. ) ;
#41900=CARTESIAN_POINT ( 'NONE',  ( 4.648177544792955347E-16, 21.00000000000002132, -108.9047308033774328 ) ) ;
#41903=CARTESIAN_POINT ( 'NONE',  ( -1.750000000000002220, 14.46891108675447946, -58.79431413575483845 ) ) ;
#41904=CARTESIAN_POINT ( 'NONE',  ( 4.648177544792955347E-16, 21.00000000000001421, -47.21098080242149564 ) ) ;
#41905=CARTESIAN_POINT ( 'NONE',  ( -3.310556943750001313, 17.50000000000001066, -24.76410580289947916 ) ) ;
#41906=CARTESIAN_POINT ( 'NONE',  ( 1.750000000000001110, 20.53108891324555074, -47.98806413671076143 ) ) ;
#41907=CARTESIAN_POINT ( 'NONE',  ( 4.648177544792955347E-16, 21.00000000000002132, -106.2109808024215027 ) ) ;
#41908=CARTESIAN_POINT ( 'NONE',  ( -3.310556943750000425, 19.41135094264166128, -32.93493913623279923 ) ) ;
#41911=CARTESIAN_POINT ( 'NONE',  ( 3.500000000000000000, 15.47927405783632082, -50.23806413671076854 ) ) ;
#41915=CARTESIAN_POINT ( 'NONE',  ( 1.655278471875001101, 20.36702641396249192, -82.09743913623279354 ) ) ;
#41916=CARTESIAN_POINT ( 'NONE',  ( -0.9378221735089310451, 14.00000000000000888, -25.44938900211595012 ) ) ;
#41917=ORIENTED_EDGE ( 'NONE', *, *, #12080, .T. ) ;
#41918=FACE_OUTER_BOUND ( 'NONE', #39170, .T. ) ;
#41919=CARTESIAN_POINT ( 'NONE',  ( 3.500000000000001332, 17.50000000000001776, -87.46098080242151696 ) ) ;
#41920=ORIENTED_EDGE ( 'NONE', *, *, #9863, .T. ) ;
#41923=CARTESIAN_POINT ( 'NONE',  ( -3.310556943750001313, 17.50000000000001776, -93.76410580289947916 ) ) ;
#41924=ORIENTED_EDGE ( 'NONE', *, *, #41106, .T. ) ;
#41925=DIRECTION ( 'NONE',  ( 0.000000000000000000, 1.000000000000000000, 0.000000000000000000 ) ) ;
#41930=ORIENTED_EDGE ( 'NONE', *, *, #1692, .F. ) ;
#41931=CARTESIAN_POINT ( 'NONE',  ( 0.000000000000000000, 17.50000000000002487, -149.5231586289125687 ) ) ;
#41932=CYLINDRICAL_SURFACE ( 'NONE', #18065, 3.499999999999999556 ) ;
#41933=CARTESIAN_POINT ( 'NONE',  ( 3.310556943750001313, 19.41135094264167549, -133.1807724695661364 ) ) ;
#41934=ORIENTED_EDGE ( 'NONE', *, *, #5423, .T. ) ;
#41935=CARTESIAN_POINT ( 'NONE',  ( 1.750000000000001110, 20.53108891324556140, -138.9880641367107614 ) ) ;
#41936=CARTESIAN_POINT ( 'NONE',  ( 1.655278471874998436, 14.63297358603754894, -122.5182724695661278 ) ) ;
#41937=CARTESIAN_POINT ( 'NONE',  ( -1.655278471875002211, 14.63297358603754184, -50.68493913623279923 ) ) ;
#41938=ORIENTED_EDGE ( 'NONE', *, *, #28510, .F. ) ;
#41939=CARTESIAN_POINT ( 'NONE',  ( 3.500000000000000000, 15.47927405783633503, -130.2380641367107614 ) ) ;
#41940=( BOUNDED_CURVE ( )  B_SPLINE_CURVE ( 2, ( #31899, #34469, #12764, #38284, #2560 ),
 .UNSPECIFIED., .F., .T. ) 
 B_SPLINE_CURVE_WITH_KNOTS ( ( 3, 2, 3 ),
 ( 0.9979166666666666741, 0.9986111111111111160, 1.000000000000000000 ),
 .UNSPECIFIED. ) 
 CURVE ( )  GEOMETRIC_REPRESENTATION_ITEM ( )  RATIONAL_B_SPLINE_CURVE ( ( 0.9330127018922194093, 0.9330127018922194093, 1.000000000000000000, 0.8660254037844387076, 1.000000000000000000 ) ) 
 REPRESENTATION_ITEM ( '' )  );
#41942=CARTESIAN_POINT ( 'NONE',  ( 3.310556943750001313, 17.50000000000001776, -79.35160580289945642 ) ) ;
#41943=CARTESIAN_POINT ( 'NONE',  ( 3.500000000000001332, 17.50000000000002132, -125.4609808024215170 ) ) ;
#41944=CARTESIAN_POINT ( 'NONE',  ( 3.310556943750001313, 19.41135094264166838, -108.1807724695661506 ) ) ;
#41945=CARTESIAN_POINT ( 'NONE',  ( 1.749999999999998224, 14.46891108675448123, -81.32139747004410424 ) ) ;
#41948=CARTESIAN_POINT ( 'NONE',  ( -3.500000000000002220, 15.47927405783632615, -74.87764746908817415 ) ) ;
#41949=CARTESIAN_POINT ( 'NONE',  ( -1.394453263437886604E-15, 14.00000000000001776, -101.4047308033774186 ) ) ;
#41950=CARTESIAN_POINT ( 'NONE',  ( -3.310556943750000425, 19.41135094264165772, -40.84743913623280775 ) ) ;
#41951=CARTESIAN_POINT ( 'NONE',  ( -3.310556943750001313, 17.50000000000001776, -101.8516058028994706 ) ) ;
#41952=CARTESIAN_POINT ( 'NONE',  ( 3.500000000000001332, 19.52072594216370760, -73.37764746908817415 ) ) ;
#41953=CARTESIAN_POINT ( 'NONE',  ( 2.474675557024783212E-16, 21.54145188432739388, -65.90473080337743284 ) ) ;
#41954=DIRECTION ( 'NONE',  ( 0.000000000000000000, 1.000000000000000000, 0.000000000000000000 ) ) ;
#41956=CARTESIAN_POINT ( 'NONE',  ( -1.655278471875002211, 14.63297358603755072, -116.6849391362327850 ) ) ;
#41957=DIRECTION ( 'NONE',  ( -0.000000000000000000, 1.259100132267607459E-16, -1.000000000000000000 ) ) ;
#41960=CARTESIAN_POINT ( 'NONE',  ( 0.9378221735089281585, 14.00000000000000888, -32.36007260463890844 ) ) ;
#41962=CARTESIAN_POINT ( 'NONE',  ( 2.340729813953370519E-16, 21.32270188528331190, -100.0141058028994792 ) ) ;
#41963=CARTESIAN_POINT ( 'NONE',  ( -1.394453263437886604E-15, 14.00000000000001066, -52.40473080337743284 ) ) ;
#41964=EDGE_CURVE ( 'NONE', #12311, #29973, #7019, .T. ) ;
#41966=ORIENTED_EDGE ( 'NONE', *, *, #18158, .F. ) ;
#41967=CARTESIAN_POINT ( 'NONE',  ( -1.394453263437886604E-15, 14.00000000000001066, -28.71098080242150985 ) ) ;
#41968=EDGE_CURVE ( 'NONE', #40349, #3232, #4037, .T. ) ;
#41969=CARTESIAN_POINT ( 'NONE',  ( 3.500000000000000000, 15.47927405783632082, -48.23806413671076143 ) ) ;
#41970=CARTESIAN_POINT ( 'NONE',  ( -3.500000000000001332, 17.50000000000002132, -102.6547308033774186 ) ) ;
#41971=CARTESIAN_POINT ( 'NONE',  ( 4.648177544792955347E-16, 21.00000000000002487, -133.9047308033774186 ) ) ;
#41974=CARTESIAN_POINT ( 'NONE',  ( 3.310556943749999981, 15.58864905735836182, -36.34743913623281486 ) ) ;
#41979=CARTESIAN_POINT ( 'NONE',  ( -3.500000000000001332, 17.50000000000002487, -138.6547308033774186 ) ) ;
#41984=CARTESIAN_POINT ( 'NONE',  ( -3.500000000000000000, 19.52072594216371826, -119.7380641367107756 ) ) ;
#41985=CARTESIAN_POINT ( 'NONE',  ( -1.749999999999999778, 20.53108891324555785, -116.8213974700440900 ) ) ;
#41987=CARTESIAN_POINT ( 'NONE',  ( -1.655278471874999990, 20.36702641396249902, -138.0182724695661420 ) ) ;
#41988=CARTESIAN_POINT ( 'NONE',  ( -1.750000000000002220, 14.46891108675447590, -34.79431413575484555 ) ) ;
#41990=CARTESIAN_POINT ( 'NONE',  ( -3.500000000000000000, 19.52072594216370760, -66.04431413575484555 ) ) ;
#41992=EDGE_CURVE ( 'NONE', #31245, #37404, #30130, .T. ) ;
#41993=CARTESIAN_POINT ( 'NONE',  ( 3.500000000000000000, 15.47927405783633503, -142.5443141357548313 ) ) ;
#41995=CARTESIAN_POINT ( 'NONE',  ( -3.500000000000001332, 17.50000000000002487, -138.9609808024214885 ) ) ;
#41996=CARTESIAN_POINT ( 'NONE',  ( 0.000000000000000000, 17.50000000000002487, -149.5231586289125687 ) ) ;
#41997=CARTESIAN_POINT ( 'NONE',  ( -3.310556943750000425, 19.41135094264166838, -123.8474391362327935 ) ) ;
#42000=CARTESIAN_POINT ( 'NONE',  ( -3.500000000000002220, 15.47927405783632970, -81.87764746908818836 ) ) ;
#42001=CARTESIAN_POINT ( 'NONE',  ( -3.500000000000000888, 19.52072594216371115, -91.04431413575484555 ) ) ;
#42002=CARTESIAN_POINT ( 'NONE',  ( -3.500000000000002220, 15.47927405783632437, -45.57139747004409003 ) ) ;
#42003=CARTESIAN_POINT ( 'NONE',  ( -1.655278471875002211, 14.63297358603754361, -60.59743913623280775 ) ) ;
#42004=CARTESIAN_POINT ( 'NONE',  ( -3.310556943750000425, 19.41135094264166838, -115.9349391362327850 ) ) ;
#42005=DIRECTION ( 'NONE',  ( -0.000000000000000000, 1.259100132267607459E-16, -1.000000000000000000 ) ) ;
#42006=CARTESIAN_POINT ( 'NONE',  ( 3.500000000000001776, 19.52072594216370405, -32.07139747004410424 ) ) ;
#42007=CARTESIAN_POINT ( 'NONE',  ( 4.648177544792955347E-16, 21.00000000000002132, -109.2109808024215170 ) ) ;
#42009=CARTESIAN_POINT ( 'NONE',  ( 3.310556943749999981, 15.58864905735837425, -131.4349391362327992 ) ) ;
#42012=CARTESIAN_POINT ( 'NONE',  ( -3.310556943750002201, 15.58864905735836714, -40.76827246956612782 ) ) ;
#42014=CARTESIAN_POINT ( 'NONE',  ( 2.340729813953370519E-16, 21.32270188528330834, -70.10160580289945642 ) ) ;
#42016=CARTESIAN_POINT ( 'NONE',  ( -3.310556943750000425, 19.41135094264166128, -66.84743913623280775 ) ) ;
#42018=ORIENTED_EDGE ( 'NONE', *, *, #23364, .T. ) ;
#42019=CARTESIAN_POINT ( 'NONE',  ( 3.310556943749999981, 15.58864905735836892, -87.43493913623281344 ) ) ;
#42020=EDGE_CURVE ( 'NONE', #22103, #39717, #38822, .T. ) ;
#42022=CYLINDRICAL_SURFACE ( 'NONE', #21103, 3.499999999999999556 ) ;
#42023=DIRECTION ( 'NONE',  ( 0.000000000000000000, 1.000000000000000000, 0.000000000000000000 ) ) ;
#42024=CARTESIAN_POINT ( 'NONE',  ( -1.394453263437886604E-15, 14.00000000000001776, -85.40473080337743284 ) ) ;
#42025=CARTESIAN_POINT ( 'NONE',  ( 3.310556943750001313, 19.41135094264166483, -51.18077246956613635 ) ) ;
#42027=CARTESIAN_POINT ( 'NONE',  ( 3.310556943750001313, 17.50000000000002132, -107.2641058028994649 ) ) ;
#42029=VERTEX_POINT ( 'NONE', #26033 ) ;
#42033=CARTESIAN_POINT ( 'NONE',  ( -1.655278471874999990, 20.36702641396248836, -57.93077246956614346 ) ) ;
#42034=ORIENTED_EDGE ( 'NONE', *, *, #41811, .F. ) ;
#42035=ORIENTED_EDGE ( 'NONE', *, *, #10684, .T. ) ;
#42039=DIRECTION ( 'NONE',  ( -0.000000000000000000, 1.259100132267607459E-16, -1.000000000000000000 ) ) ;
#42040=ORIENTED_EDGE ( 'NONE', *, *, #22527, .F. ) ;
#42041=EDGE_CURVE ( 'NONE', #23073, #19172, #1074, .T. ) ;
#42042=CARTESIAN_POINT ( 'NONE',  ( 1.750000000000001110, 20.53108891324556140, -143.2943141357548313 ) ) ;
#42043=CARTESIAN_POINT ( 'NONE',  ( 3.310556943749999981, 15.58864905735837425, -123.3474391362328078 ) ) ;
#42044=CARTESIAN_POINT ( 'NONE',  ( 3.500000000000000000, 15.47927405783632793, -94.54431413575484555 ) ) ;
#42045=EDGE_CURVE ( 'NONE', #17813, #41613, #5403, .T. ) ;
#42047=CARTESIAN_POINT ( 'NONE',  ( -3.310556943750000425, 19.41135094264165772, -35.93493913623279923 ) ) ;
#42048=CARTESIAN_POINT ( 'NONE',  ( -7.022189441860112050E-16, 13.67729811471671297, -25.60160580289946708 ) ) ;
#42049=CARTESIAN_POINT ( 'NONE',  ( -1.655278471874999990, 20.36702641396249192, -87.01827246956612782 ) ) ;
#42050=CARTESIAN_POINT ( 'NONE',  ( -3.310556943750000425, 19.41135094264167549, -137.8474391362328220 ) ) ;
#42053=CARTESIAN_POINT ( 'NONE',  ( -3.310556943750001313, 17.50000000000002487, -134.8516058028994564 ) ) ;
#42057=CARTESIAN_POINT ( 'NONE',  ( 2.474675557024783212E-16, 21.54145188432739744, -81.90473080337743284 ) ) ;
#42058=CARTESIAN_POINT ( 'NONE',  ( -3.310556943750001313, 17.50000000000001421, -56.85160580289947063 ) ) ;
#42062=CARTESIAN_POINT ( 'NONE',  ( -3.310556943750002645, 15.58864905735837247, -85.76827246956612782 ) ) ;
#42064=VECTOR ( 'NONE', #30719, 1000.000000000000000 ) ;
#42065=CARTESIAN_POINT ( 'NONE',  ( 1.655278471875001101, 20.36702641396249547, -116.0974391362327935 ) ) ;
#42066=CARTESIAN_POINT ( 'NONE',  ( -3.310556943750001313, 17.50000000000001776, -82.76410580289947916 ) ) ;
#42069=CARTESIAN_POINT ( 'NONE',  ( -3.500000000000002220, 15.47927405783633503, -110.5713974700440900 ) ) ;
#42070=( BOUNDED_CURVE ( )  B_SPLINE_CURVE ( 2, ( #12683, #41831, #22878, #6294, #16503, #12890, #6913, #3312, #113 ),
 .UNSPECIFIED., .F., .T. ) 
 B_SPLINE_CURVE_WITH_KNOTS ( ( 3, 2, 2, 2, 3 ),
 ( 0.7312499999999999556, 0.7319444444444443976, 0.7333333333333332815, 0.7347222222222222765, 0.7354166666666667185 ),
 .UNSPECIFIED. ) 
 CURVE ( )  GEOMETRIC_REPRESENTATION_ITEM ( )  RATIONAL_B_SPLINE_CURVE ( ( 0.9330127018922194093, 0.9330127018922194093, 1.000000000000000000, 0.8660254037844387076, 1.000000000000000000, 0.8660254037844387076, 1.000000000000000000, 0.9330127018922194093, 0.9330127018922194093 ) ) 
 REPRESENTATION_ITEM ( '' )  );
#42072=CARTESIAN_POINT ( 'NONE',  ( 4.648177544792955347E-16, 21.00000000000002487, -131.9047308033774186 ) ) ;
#42073=CARTESIAN_POINT ( 'NONE',  ( 0.000000000000000000, 21.00000000000002487, -149.5231586289125687 ) ) ;
#42076=CARTESIAN_POINT ( 'NONE',  ( -3.310556943750001313, 17.50000000000001421, -64.76410580289946495 ) ) ;
#42078=CARTESIAN_POINT ( 'NONE',  ( -3.310556943750000425, 19.41135094264166838, -122.8474391362328220 ) ) ;
#42079=LINE ( 'NONE', #5919, #36583 ) ;
#42080=EDGE_CURVE ( 'NONE', #35835, #8868, #9769, .T. ) ;
#42086=DIRECTION ( 'NONE',  ( -0.000000000000000000, 1.259100132267607459E-16, -1.000000000000000000 ) ) ;
#42087=CARTESIAN_POINT ( 'NONE',  ( -3.310556943750001313, 17.50000000000001776, -74.76410580289947916 ) ) ;
#42092=CARTESIAN_POINT ( 'NONE',  ( -3.310556943750001313, 17.50000000000002487, -142.7641058028994792 ) ) ;
#42093=CARTESIAN_POINT ( 'NONE',  ( -3.500000000000002220, 15.47927405783632437, -51.57139747004408292 ) ) ;
#42096=CARTESIAN_POINT ( 'NONE',  ( 3.310556943749999981, 15.58864905735836182, -41.43493913623279212 ) ) ;
#42097=CARTESIAN_POINT ( 'NONE',  ( -7.022189441860112050E-16, 13.67729811471672541, -103.6016058028994564 ) ) ;
#42099=CARTESIAN_POINT ( 'NONE',  ( -3.310556943750000425, 19.41135094264165772, -30.84743913623280775 ) ) ;
#42100=CARTESIAN_POINT ( 'NONE',  ( -0.9378221735089310451, 14.00000000000002309, -111.7556390011600200 ) ) ;
#42101=CARTESIAN_POINT ( 'NONE',  ( 2.474675557024783212E-16, 21.54145188432740099, -108.2109808024215027 ) ) ;
#42104=CARTESIAN_POINT ( 'NONE',  ( -3.500000000000000888, 19.52072594216371115, -96.73806413671076143 ) ) ;
#42105=CARTESIAN_POINT ( 'NONE',  ( 0.000000000000000000, 17.50000000000002487, -149.5231586289125687 ) ) ;
#42108=CARTESIAN_POINT ( 'NONE',  ( -1.749999999999999778, 20.53108891324555074, -60.12764746908817415 ) ) ;
#42109=CARTESIAN_POINT ( 'NONE',  ( -1.750000000000002220, 14.46891108675447768, -46.79431413575483845 ) ) ;
#42110=CARTESIAN_POINT ( 'NONE',  ( -1.394453263437886604E-15, 14.00000000000000711, -24.71098080242150985 ) ) ;
#42111=CARTESIAN_POINT ( 'NONE',  ( 2.474675557024783212E-16, 21.54145188432739388, -48.90473080337742573 ) ) ;
#42113=CARTESIAN_POINT ( 'NONE',  ( 3.310556943750001313, 17.50000000000001066, -30.35160580289947418 ) ) ;
#42116=CARTESIAN_POINT ( 'NONE',  ( 0.000000000000000000, 21.00000000000002487, -149.5231586289125687 ) ) ;
#42153=COLOUR_RGB('Black',0.12,0.14,0.17);
#42154=FILL_AREA_STYLE_COLOUR('',#42153);
#42155=FILL_AREA_STYLE('',(#42154));
#42156=SURFACE_STYLE_FILL_AREA(#42155);
#42157=SURFACE_SIDE_STYLE('',(#42156));
#42158=SURFACE_STYLE_USAGE(.BOTH.,#42157);
#42159=PRESENTATION_STYLE_ASSIGNMENT((#42158));
ENDSEC;
END-ISO-10303-21;
